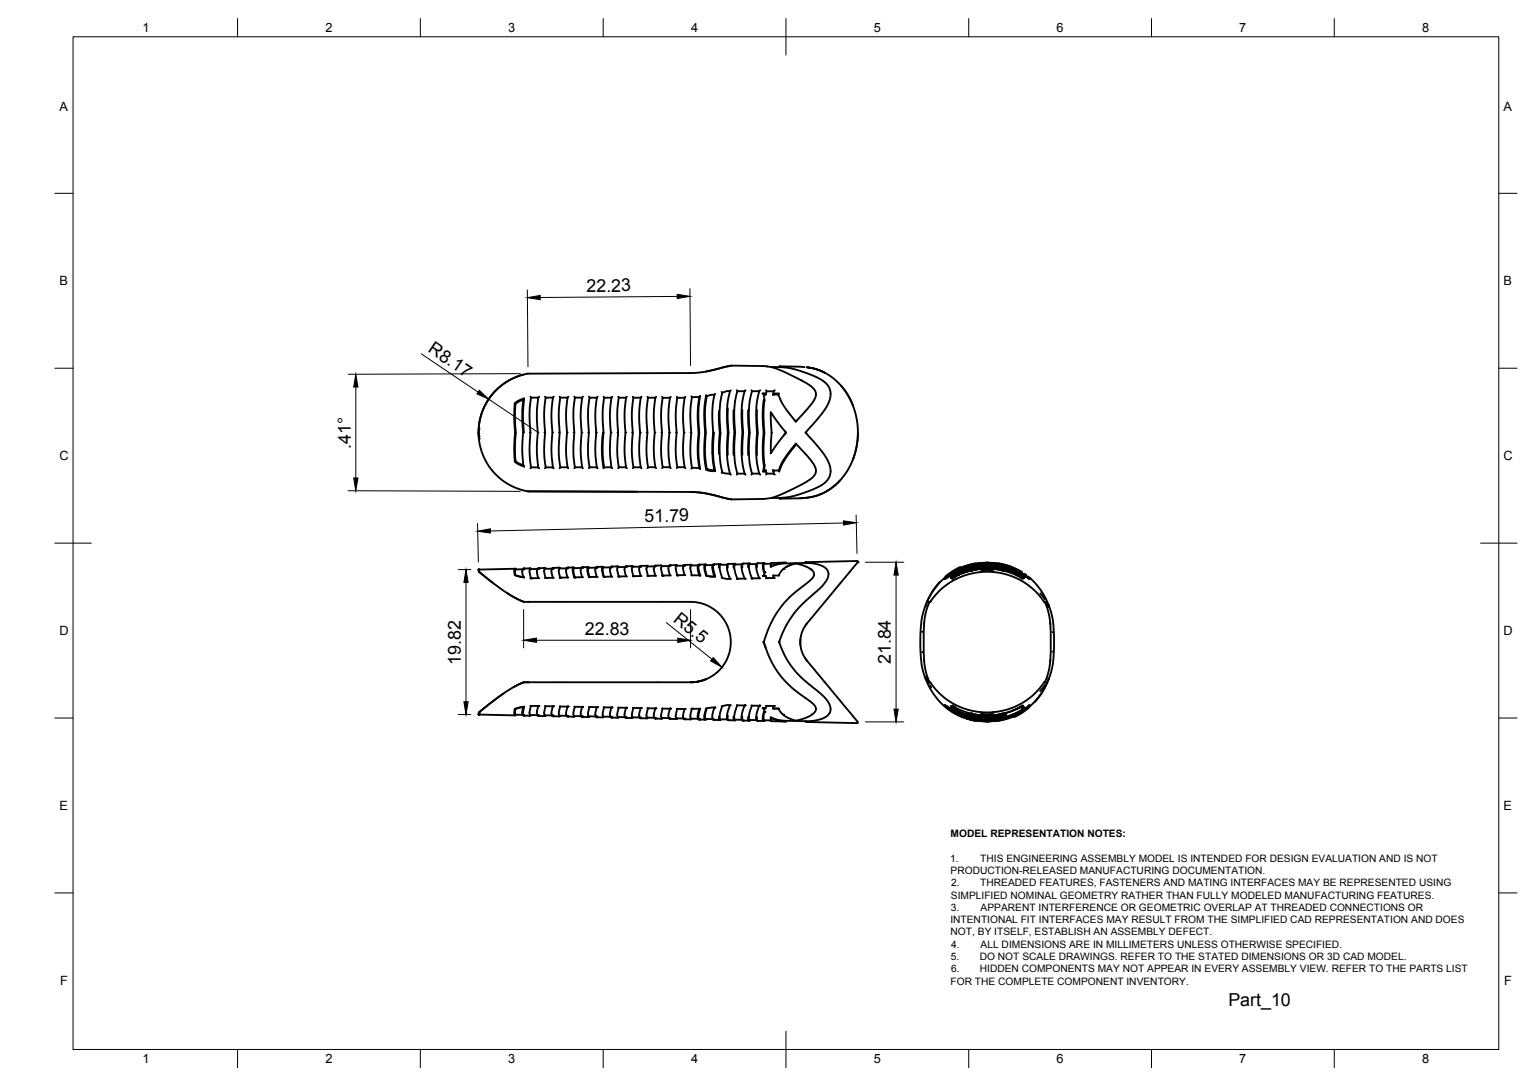
ISO-10303-21;
HEADER;
/* Generated by software containing ST-Developer
 * from STEP Tools, Inc. (www.steptools.com) 
 */

FILE_DESCRIPTION(
/* description */ ('STEP AP242 Edition 2'),
/* implementation_level */ '2;1');

FILE_NAME(
/* name */ 'Part_10.step',
/* time_stamp */ '2026-10-06T10:11:12-07:00',
/* author */ (''),
/* organization */ (''),
/* preprocessor_version */ 'ST-DEVELOPER v20.2',
/* originating_system */ 'Autodesk Translation Framework v15.15.0.0',
/* authorisation */ '');

FILE_SCHEMA (('AUTOMOTIVE_DESIGN { 1 0 10303 214 3 1 1 }'));
ENDSEC;

DATA;
#10=MECHANICAL_DESIGN_GEOMETRIC_PRESENTATION_REPRESENTATION('',(#1786),#54580);
#71=ELLIPSE('',#18547,0.0043287679400298,0.000195921240702569);
#131=CONICAL_SURFACE('',#18530,0.00265391324380841,1.37712278252772);
#132=CONICAL_SURFACE('',#18588,3.48610109958525E-5,0.141830950521549);
#133=CONICAL_SURFACE('',#18589,3.48394090574724E-5,0.141829837312193);
#134=CONICAL_SURFACE('',#18592,3.48609373749775E-5,0.141830787231043);
#135=CONICAL_SURFACE('',#18599,3.48393253777631E-5,0.141829687868949);
#136=CONICAL_SURFACE('',#18616,0.0026288792428795,1.38153808164484);
#137=CONICAL_SURFACE('',#18636,0.00265359345896356,1.37715118560564);
#138=CONICAL_SURFACE('',#18637,0.00263026865692114,1.38147192931234);
#139=CONICAL_SURFACE('',#18655,0.00614051900660571,0.733182632957209);
#140=CONICAL_SURFACE('',#18656,0.00592688725800199,0.772003379135275);
#143=SPHERICAL_SURFACE('',#18577,0.0001);
#144=SPHERICAL_SURFACE('',#18591,0.0001);
#145=SPHERICAL_SURFACE('',#18594,0.0001);
#146=SPHERICAL_SURFACE('',#18598,0.0001);
#147=SPHERICAL_SURFACE('',#18605,0.0001);
#148=SPHERICAL_SURFACE('',#18609,0.0001);
#192=TOROIDAL_SURFACE('',#18561,43.0172655815845,43.0171612476028);
#193=TOROIDAL_SURFACE('',#18562,43.0192266270189,43.0191222943202);
#194=TOROIDAL_SURFACE('',#18565,0.00931146593211752,9.99931797011151E-5);
#195=TOROIDAL_SURFACE('',#18566,0.00931142924739271,9.99898356076873E-5);
#196=TOROIDAL_SURFACE('',#18569,43.0172619393224,43.0171576053291);
#197=TOROIDAL_SURFACE('',#18572,43.0192273884314,43.0191230557219);
#198=TOROIDAL_SURFACE('',#18575,0.00408904168337188,9.99937992667749E-5);
#199=TOROIDAL_SURFACE('',#18576,0.00408904168282665,9.99937992622037E-5);
#200=TOROIDAL_SURFACE('',#18579,0.00806904972011834,0.0001);
#201=TOROIDAL_SURFACE('',#18596,0.00806904972011834,0.0001);
#202=TOROIDAL_SURFACE('',#18607,0.00806904972011834,0.0001);
#203=TOROIDAL_SURFACE('',#18610,0.00408913544960028,0.000100040268464404);
#204=TOROIDAL_SURFACE('',#18615,0.0040891354500689,0.000100040268460989);
#205=TOROIDAL_SURFACE('',#18659,0.00836123117893049,0.00010366855176599);
#206=TOROIDAL_SURFACE('',#18684,0.00815612470458011,0.000103667398436053);
#207=TOROIDAL_SURFACE('',#18687,0.00871025103595541,0.000103662944645038);
#208=TOROIDAL_SURFACE('',#18688,0.00850695260093233,0.000103538344715324);
#209=TOROIDAL_SURFACE('',#18689,0.00871017740815006,0.000103662875721332);
#210=TOROIDAL_SURFACE('',#18690,0.00836086459677531,0.00010366849218277);
#211=TOROIDAL_SURFACE('',#18717,0.00815633290592581,0.00010366728866353);
#212=TOROIDAL_SURFACE('',#18720,0.00864670349933223,0.000103665652215068);
#213=TOROIDAL_SURFACE('',#18721,0.00850751186664759,0.00010353842958418);
#214=TOROIDAL_SURFACE('',#18722,0.00867809676383051,0.000103667225081647);
#215=TOROIDAL_SURFACE('',#18723,0.000528332315378602,0.000103512489509189);
#216=TOROIDAL_SURFACE('',#18724,0.00917182682012945,9.99999869507318E-5);
#217=TOROIDAL_SURFACE('',#18725,0.0040475617622906,9.99881997863187E-5);
#218=TOROIDAL_SURFACE('',#18727,0.00904061800886142,0.000100004225353136);
#219=TOROIDAL_SURFACE('',#18728,0.00360779826836622,9.99961776029768E-5);
#220=TOROIDAL_SURFACE('',#18729,0.0052330922254768,9.99920638411154E-5);
#221=TOROIDAL_SURFACE('',#18730,0.000732704479508413,0.000103581963632023);
#222=TOROIDAL_SURFACE('',#18731,0.0091590450963941,9.99999843261172E-5);
#223=TOROIDAL_SURFACE('',#18733,0.00915567105502713,9.99999896646458E-5);
#224=TOROIDAL_SURFACE('',#18734,0.00389212279884052,9.99966861379351E-5);
#225=TOROIDAL_SURFACE('',#18735,0.00357438694091518,9.99963100583166E-5);
#226=TOROIDAL_SURFACE('',#18736,0.00915654585560002,9.9999989426787E-5);
#227=TOROIDAL_SURFACE('',#18738,0.009161034600788,9.9999985180343E-5);
#228=TOROIDAL_SURFACE('',#18739,0.000584574123278554,0.000103503607413102);
#229=TOROIDAL_SURFACE('',#18740,0.00392317197798013,9.99876820615925E-5);
#230=TOROIDAL_SURFACE('',#18741,0.00339615673268595,9.99957943856544E-5);
#231=TOROIDAL_SURFACE('',#18742,0.00916833013124114,9.99999895548281E-5);
#232=TOROIDAL_SURFACE('',#18744,0.00475797702577389,9.99904037368119E-5);
#233=TOROIDAL_SURFACE('',#18745,0.00917126548676907,9.99999867155255E-5);
#234=TOROIDAL_SURFACE('',#18746,0.00060192390944549,0.000103561614538704);
#325=B_SPLINE_SURFACE_WITH_KNOTS('',3,3,((#25845,#25846,#25847,#25848),
(#25849,#25850,#25851,#25852),(#25853,#25854,#25855,#25856),(#25857,#25858,
#25859,#25860),(#25861,#25862,#25863,#25864),(#25865,#25866,#25867,#25868),
(#25869,#25870,#25871,#25872),(#25873,#25874,#25875,#25876),(#25877,#25878,
#25879,#25880),(#25881,#25882,#25883,#25884),(#25885,#25886,#25887,#25888),
(#25889,#25890,#25891,#25892),(#25893,#25894,#25895,#25896),(#25897,#25898,
#25899,#25900),(#25901,#25902,#25903,#25904),(#25905,#25906,#25907,#25908),
(#25909,#25910,#25911,#25912),(#25913,#25914,#25915,#25916),(#25917,#25918,
#25919,#25920),(#25921,#25922,#25923,#25924),(#25925,#25926,#25927,#25928),
(#25929,#25930,#25931,#25932),(#25933,#25934,#25935,#25936),(#25937,#25938,
#25939,#25940),(#25941,#25942,#25943,#25944),(#25945,#25946,#25947,#25948),
(#25949,#25950,#25951,#25952),(#25953,#25954,#25955,#25956),(#25957,#25958,
#25959,#25960),(#25961,#25962,#25963,#25964),(#25965,#25966,#25967,#25968),
(#25969,#25970,#25971,#25972),(#25973,#25974,#25975,#25976),(#25977,#25978,
#25979,#25980),(#25981,#25982,#25983,#25984),(#25985,#25986,#25987,#25988),
(#25989,#25990,#25991,#25992),(#25993,#25994,#25995,#25996),(#25997,#25998,
#25999,#26000)),.UNSPECIFIED.,.T.,.F.,.F.,(4,1,1,1,1,1,1,1,1,1,1,1,1,1,
1,1,1,1,1,1,1,1,1,1,1,1,1,1,1,1,1,1,1,1,1,1,4),(4,4),(-1.,-0.9921875,-0.984375,
-0.96875,-0.9375,-0.921875,-0.90625,-0.875,-0.84375,-0.8125,-0.78125,-0.75,
-0.6875,-0.625,-0.59375,-0.5625,-0.53125,-0.515625,-0.5,-0.4921875,-0.484375,
-0.46875,-0.4375,-0.421875,-0.40625,-0.375,-0.34375,-0.3125,-0.28125,-0.25,
-0.1875,-0.125,-0.09375,-0.0625,-0.03125,-0.015625,0.),(0.0970446199077052,
0.967246564070376),.UNSPECIFIED.);
#326=B_SPLINE_SURFACE_WITH_KNOTS('',3,1,((#26093,#26094),(#26095,#26096),
(#26097,#26098),(#26099,#26100),(#26101,#26102),(#26103,#26104),(#26105,
#26106),(#26107,#26108),(#26109,#26110),(#26111,#26112),(#26113,#26114),
(#26115,#26116),(#26117,#26118),(#26119,#26120),(#26121,#26122),(#26123,
#26124),(#26125,#26126),(#26127,#26128),(#26129,#26130),(#26131,#26132),
(#26133,#26134),(#26135,#26136),(#26137,#26138),(#26139,#26140),(#26141,
#26142),(#26143,#26144),(#26145,#26146),(#26147,#26148),(#26149,#26150),
(#26151,#26152),(#26153,#26154),(#26155,#26156)),.UNSPECIFIED.,.T.,.F.,
 .F.,(4,1,2,1,1,1,1,1,1,1,2,1,1,1,2,1,1,1,1,1,1,1,3,1,4),(2,2),(-0.962123410396902,
-0.943185115595354,-0.924246820793805,-0.871215968194179,-0.818185115594553,
-0.765154262994927,-0.712123410395301,-0.659092557795675,-0.606061705196049,
-0.553030852596423,-0.499999999996798,-0.481061705196237,-0.462123410395676,
-0.443185115595116,-0.424246820794555,-0.371215968195236,-0.318185115595916,
-0.265154262996597,-0.212123410397278,-0.159092557797958,-0.106061705198639,
-0.0530308525993189,0.,0.0189382948015488,0.0378765896030977),(0.785837404066612,
0.964086943478034),.UNSPECIFIED.);
#327=B_SPLINE_SURFACE_WITH_KNOTS('',3,1,((#26801,#26802),(#26803,#26804),
(#26805,#26806),(#26807,#26808),(#26809,#26810),(#26811,#26812),(#26813,
#26814),(#26815,#26816),(#26817,#26818),(#26819,#26820),(#26821,#26822),
(#26823,#26824),(#26825,#26826),(#26827,#26828),(#26829,#26830),(#26831,
#26832),(#26833,#26834),(#26835,#26836),(#26837,#26838),(#26839,#26840),
(#26841,#26842),(#26843,#26844),(#26845,#26846),(#26847,#26848),(#26849,
#26850),(#26851,#26852),(#26853,#26854),(#26855,#26856),(#26857,#26858),
(#26859,#26860),(#26861,#26862),(#26863,#26864),(#26865,#26866)),
 .UNSPECIFIED.,.T.,.F.,.F.,(4,1,1,1,1,3,1,1,1,2,1,1,1,1,1,1,1,2,1,1,1,2,
1,1,1,4),(2,2),(-0.237377771779514,-0.212123410397278,-0.159092557797958,
-0.106061705198639,-0.0530308525993189,0.,0.0189382948015488,0.0378765896030977,
0.0568148844046463,0.0757531792061952,0.128784031805821,0.181814884405447,
0.234845737005073,0.287876589604699,0.340907442204325,0.393938294803951,
0.446969147403577,0.500000000003202,0.518938294803763,0.537876589604324,
0.556814884404884,0.575753179205445,0.628784031804764,0.681814884404084,
0.734845737003403,0.762622228220486),(0.0953842576150604,0.872111738883991),
 .UNSPECIFIED.);
#328=B_SPLINE_SURFACE_WITH_KNOTS('',3,3,((#29129,#29130,#29131,#29132),
(#29133,#29134,#29135,#29136),(#29137,#29138,#29139,#29140),(#29141,#29142,
#29143,#29144),(#29145,#29146,#29147,#29148),(#29149,#29150,#29151,#29152),
(#29153,#29154,#29155,#29156),(#29157,#29158,#29159,#29160),(#29161,#29162,
#29163,#29164),(#29165,#29166,#29167,#29168),(#29169,#29170,#29171,#29172),
(#29173,#29174,#29175,#29176),(#29177,#29178,#29179,#29180),(#29181,#29182,
#29183,#29184),(#29185,#29186,#29187,#29188),(#29189,#29190,#29191,#29192),
(#29193,#29194,#29195,#29196),(#29197,#29198,#29199,#29200),(#29201,#29202,
#29203,#29204),(#29205,#29206,#29207,#29208),(#29209,#29210,#29211,#29212),
(#29213,#29214,#29215,#29216),(#29217,#29218,#29219,#29220),(#29221,#29222,
#29223,#29224),(#29225,#29226,#29227,#29228),(#29229,#29230,#29231,#29232),
(#29233,#29234,#29235,#29236),(#29237,#29238,#29239,#29240),(#29241,#29242,
#29243,#29244),(#29245,#29246,#29247,#29248),(#29249,#29250,#29251,#29252),
(#29253,#29254,#29255,#29256),(#29257,#29258,#29259,#29260),(#29261,#29262,
#29263,#29264),(#29265,#29266,#29267,#29268)),.UNSPECIFIED.,.T.,.F.,.F.,
(4,1,1,1,1,1,1,1,1,1,1,1,1,1,1,1,1,1,1,1,1,1,1,1,1,1,1,1,1,1,1,1,4),(4,
4),(-1.,-0.984375,-0.96875,-0.9375,-0.921875,-0.90625,-0.875,-0.84375,-0.8125,
-0.75,-0.6875,-0.625,-0.59375,-0.5625,-0.53125,-0.515625,-0.5,-0.484375,
-0.46875,-0.4375,-0.421875,-0.40625,-0.375,-0.34375,-0.3125,-0.25,-0.1875,
-0.125,-0.09375,-0.0625,-0.03125,-0.015625,0.),(0.748401658952503,0.903433079647334),
 .UNSPECIFIED.);
#329=B_SPLINE_SURFACE_WITH_KNOTS('',3,3,((#30017,#30018,#30019,#30020),
(#30021,#30022,#30023,#30024),(#30025,#30026,#30027,#30028),(#30029,#30030,
#30031,#30032),(#30033,#30034,#30035,#30036),(#30037,#30038,#30039,#30040),
(#30041,#30042,#30043,#30044),(#30045,#30046,#30047,#30048),(#30049,#30050,
#30051,#30052),(#30053,#30054,#30055,#30056),(#30057,#30058,#30059,#30060),
(#30061,#30062,#30063,#30064),(#30065,#30066,#30067,#30068),(#30069,#30070,
#30071,#30072),(#30073,#30074,#30075,#30076),(#30077,#30078,#30079,#30080),
(#30081,#30082,#30083,#30084),(#30085,#30086,#30087,#30088),(#30089,#30090,
#30091,#30092),(#30093,#30094,#30095,#30096),(#30097,#30098,#30099,#30100),
(#30101,#30102,#30103,#30104),(#30105,#30106,#30107,#30108),(#30109,#30110,
#30111,#30112),(#30113,#30114,#30115,#30116),(#30117,#30118,#30119,#30120),
(#30121,#30122,#30123,#30124),(#30125,#30126,#30127,#30128),(#30129,#30130,
#30131,#30132),(#30133,#30134,#30135,#30136),(#30137,#30138,#30139,#30140),
(#30141,#30142,#30143,#30144),(#30145,#30146,#30147,#30148),(#30149,#30150,
#30151,#30152),(#30153,#30154,#30155,#30156)),.UNSPECIFIED.,.T.,.F.,.F.,
(4,1,1,1,1,1,1,1,1,1,1,1,1,1,1,1,1,1,1,1,1,1,1,1,1,1,1,1,1,1,1,1,4),(4,
4),(1.,1.015625,1.03125,1.0625,1.078125,1.09375,1.125,1.15625,1.1875,1.25,
1.3125,1.375,1.40625,1.4375,1.46875,1.484375,1.5,1.515625,1.53125,1.5625,
1.578125,1.59375,1.625,1.65625,1.6875,1.75,1.8125,1.875,1.90625,1.9375,
1.96875,1.984375,2.),(0.748401658952503,0.903433079647334),
 .UNSPECIFIED.);
#330=B_SPLINE_SURFACE_WITH_KNOTS('',3,1,((#30336,#30337),(#30338,#30339),
(#30340,#30341),(#30342,#30343),(#30344,#30345),(#30346,#30347),(#30348,
#30349),(#30350,#30351),(#30352,#30353),(#30354,#30355),(#30356,#30357),
(#30358,#30359),(#30360,#30361),(#30362,#30363),(#30364,#30365),(#30366,
#30367),(#30368,#30369),(#30370,#30371),(#30372,#30373),(#30374,#30375),
(#30376,#30377),(#30378,#30379),(#30380,#30381),(#30382,#30383),(#30384,
#30385),(#30386,#30387),(#30388,#30389),(#30390,#30391),(#30392,#30393),
(#30394,#30395)),.UNSPECIFIED.,.T.,.F.,.F.,(4,1,1,1,2,1,1,1,1,1,1,1,2,1,
1,1,2,1,1,1,1,1,1,1,4),(2,2),(1.,1.01893829480155,1.0378765896031,1.05681488440465,
1.0757531792062,1.12878403180582,1.18181488440545,1.23484573700507,1.2878765896047,
1.34090744220433,1.39393829480395,1.44696914740358,1.5000000000032,1.51893829480376,
1.53787658960432,1.55681488440488,1.57575317920544,1.62878403180476,1.68181488440408,
1.7348457370034,1.78787658960272,1.84090744220204,1.89393829480136,1.94696914740068,
2.),(0.0953842576150604,0.872111738883991),.UNSPECIFIED.);
#331=B_SPLINE_SURFACE_WITH_KNOTS('',3,1,((#34950,#34951),(#34952,#34953),
(#34954,#34955),(#34956,#34957),(#34958,#34959),(#34960,#34961),(#34962,
#34963),(#34964,#34965),(#34966,#34967),(#34968,#34969),(#34970,#34971),
(#34972,#34973),(#34974,#34975),(#34976,#34977),(#34978,#34979),(#34980,
#34981),(#34982,#34983),(#34984,#34985),(#34986,#34987),(#34988,#34989),
(#34990,#34991),(#34992,#34993),(#34994,#34995),(#34996,#34997),(#34998,
#34999),(#35000,#35001),(#35002,#35003),(#35004,#35005),(#35006,#35007),
(#35008,#35009)),.UNSPECIFIED.,.T.,.F.,.F.,(4,1,1,1,2,1,1,1,1,1,1,1,2,1,
1,1,2,1,1,1,1,1,1,1,4),(2,2),(1.,1.01893829480155,1.0378765896031,1.05681488440465,
1.0757531792062,1.12878403180582,1.18181488440545,1.23484573700507,1.2878765896047,
1.34090744220433,1.39393829480395,1.44696914740358,1.5000000000032,1.51893829480376,
1.53787658960432,1.55681488440488,1.57575317920544,1.62878403180476,1.68181488440408,
1.7348457370034,1.78787658960272,1.84090744220204,1.89393829480136,1.94696914740068,
2.),(0.785837404066612,0.964086943478034),.UNSPECIFIED.);
#332=B_SPLINE_SURFACE_WITH_KNOTS('',1,3,((#35025,#35026,#35027,#35028,#35029,
#35030,#35031,#35032,#35033,#35034,#35035,#35036,#35037,#35038,#35039,#35040,
#35041,#35042,#35043,#35044),(#35045,#35046,#35047,#35048,#35049,#35050,
#35051,#35052,#35053,#35054,#35055,#35056,#35057,#35058,#35059,#35060,#35061,
#35062,#35063,#35064),(#35065,#35066,#35067,#35068,#35069,#35070,#35071,
#35072,#35073,#35074,#35075,#35076,#35077,#35078,#35079,#35080,#35081,#35082,
#35083,#35084)),.UNSPECIFIED.,.F.,.F.,.F.,(2,1,2),(4,2,2,2,2,2,2,2,2,4),
(0.,1.,1.005),(0.999268187708551,0.99938964839267,0.999511718705164,0.999633789017659,
0.999694824173906,0.999755859330153,0.999877929642648,0.999908447220771,
0.999938964798895,0.999999999955142),.UNSPECIFIED.);
#333=B_SPLINE_SURFACE_WITH_KNOTS('',3,3,((#35229,#35230,#35231,#35232),
(#35233,#35234,#35235,#35236),(#35237,#35238,#35239,#35240),(#35241,#35242,
#35243,#35244),(#35245,#35246,#35247,#35248),(#35249,#35250,#35251,#35252),
(#35253,#35254,#35255,#35256),(#35257,#35258,#35259,#35260),(#35261,#35262,
#35263,#35264),(#35265,#35266,#35267,#35268),(#35269,#35270,#35271,#35272),
(#35273,#35274,#35275,#35276),(#35277,#35278,#35279,#35280),(#35281,#35282,
#35283,#35284),(#35285,#35286,#35287,#35288),(#35289,#35290,#35291,#35292),
(#35293,#35294,#35295,#35296),(#35297,#35298,#35299,#35300),(#35301,#35302,
#35303,#35304),(#35305,#35306,#35307,#35308),(#35309,#35310,#35311,#35312),
(#35313,#35314,#35315,#35316),(#35317,#35318,#35319,#35320),(#35321,#35322,
#35323,#35324),(#35325,#35326,#35327,#35328),(#35329,#35330,#35331,#35332),
(#35333,#35334,#35335,#35336),(#35337,#35338,#35339,#35340),(#35341,#35342,
#35343,#35344),(#35345,#35346,#35347,#35348),(#35349,#35350,#35351,#35352),
(#35353,#35354,#35355,#35356),(#35357,#35358,#35359,#35360),(#35361,#35362,
#35363,#35364),(#35365,#35366,#35367,#35368),(#35369,#35370,#35371,#35372),
(#35373,#35374,#35375,#35376),(#35377,#35378,#35379,#35380),(#35381,#35382,
#35383,#35384)),.UNSPECIFIED.,.T.,.F.,.F.,(4,1,1,1,1,1,1,1,1,1,1,1,1,1,
1,1,1,1,1,1,1,1,1,1,1,1,1,1,1,1,1,1,1,1,1,1,4),(4,4),(0.,0.0078125,0.015625,
0.03125,0.0625,0.078125,0.09375,0.125,0.15625,0.1875,0.21875,0.25,0.3125,
0.375,0.40625,0.4375,0.46875,0.484375,0.5,0.5078125,0.515625,0.53125,0.5625,
0.578125,0.59375,0.625,0.65625,0.6875,0.71875,0.75,0.8125,0.875,0.90625,
0.9375,0.96875,0.984375,1.),(0.0970446199077052,0.967246564070376),
 .UNSPECIFIED.);
#334=B_SPLINE_SURFACE_WITH_KNOTS('',3,3,((#37152,#37153,#37154,#37155),
(#37156,#37157,#37158,#37159),(#37160,#37161,#37162,#37163),(#37164,#37165,
#37166,#37167),(#37168,#37169,#37170,#37171),(#37172,#37173,#37174,#37175),
(#37176,#37177,#37178,#37179),(#37180,#37181,#37182,#37183),(#37184,#37185,
#37186,#37187),(#37188,#37189,#37190,#37191),(#37192,#37193,#37194,#37195),
(#37196,#37197,#37198,#37199),(#37200,#37201,#37202,#37203),(#37204,#37205,
#37206,#37207),(#37208,#37209,#37210,#37211),(#37212,#37213,#37214,#37215),
(#37216,#37217,#37218,#37219),(#37220,#37221,#37222,#37223),(#37224,#37225,
#37226,#37227),(#37228,#37229,#37230,#37231),(#37232,#37233,#37234,#37235),
(#37236,#37237,#37238,#37239),(#37240,#37241,#37242,#37243),(#37244,#37245,
#37246,#37247),(#37248,#37249,#37250,#37251),(#37252,#37253,#37254,#37255),
(#37256,#37257,#37258,#37259),(#37260,#37261,#37262,#37263),(#37264,#37265,
#37266,#37267),(#37268,#37269,#37270,#37271),(#37272,#37273,#37274,#37275),
(#37276,#37277,#37278,#37279),(#37280,#37281,#37282,#37283),(#37284,#37285,
#37286,#37287),(#37288,#37289,#37290,#37291)),.UNSPECIFIED.,.T.,.F.,.F.,
(4,1,1,1,1,1,1,1,1,1,1,1,1,1,1,1,1,1,1,1,1,1,1,1,1,1,1,1,1,1,1,1,4),(4,
4),(0.,0.015625,0.03125,0.0625,0.078125,0.09375,0.125,0.15625,0.1875,0.25,
0.3125,0.375,0.40625,0.4375,0.46875,0.484375,0.5,0.515625,0.53125,0.5625,
0.578125,0.59375,0.625,0.65625,0.6875,0.75,0.8125,0.875,0.90625,0.9375,
0.96875,0.984375,1.),(0.748401658952503,0.903433079647334),
 .UNSPECIFIED.);
#335=B_SPLINE_SURFACE_WITH_KNOTS('',3,3,((#44797,#44798,#44799,#44800,#44801),
(#44802,#44803,#44804,#44805,#44806),(#44807,#44808,#44809,#44810,#44811),
(#44812,#44813,#44814,#44815,#44816),(#44817,#44818,#44819,#44820,#44821),
(#44822,#44823,#44824,#44825,#44826),(#44827,#44828,#44829,#44830,#44831),
(#44832,#44833,#44834,#44835,#44836),(#44837,#44838,#44839,#44840,#44841)),
 .UNSPECIFIED.,.F.,.F.,.F.,(4,1,1,1,1,1,4),(4,1,4),(0.00214678110273797,
0.00328311417485291,0.00393151580676355,0.00522831907058484,0.00652512233440613,
0.00717352396631677,0.00830134515056596),(-0.00760700162757571,0.496196499186212,
1.0043667759093),.UNSPECIFIED.);
#336=B_SPLINE_SURFACE_WITH_KNOTS('',3,3,((#44958,#44959,#44960,#44961,#44962),
(#44963,#44964,#44965,#44966,#44967),(#44968,#44969,#44970,#44971,#44972),
(#44973,#44974,#44975,#44976,#44977),(#44978,#44979,#44980,#44981,#44982),
(#44983,#44984,#44985,#44986,#44987),(#44988,#44989,#44990,#44991,#44992),
(#44993,#44994,#44995,#44996,#44997),(#44998,#44999,#45000,#45001,#45002)),
 .UNSPECIFIED.,.F.,.F.,.F.,(4,1,1,1,1,1,4),(4,1,4),(0.0021509040335451,
0.00328755319845632,0.00393613508633228,0.0052332988620842,0.00653046263783612,
0.00717904452571208,0.0083071902285716),(-0.00767667710147584,0.496161661449262,
1.00435471660804),.UNSPECIFIED.);
#365=B_SPLINE_CURVE_WITH_KNOTS('',3,(#26003,#26004,#26005,#26006),
 .UNSPECIFIED.,.F.,.F.,(4,4),(0.668250521172189,0.843615509259931),
 .UNSPECIFIED.);
#366=B_SPLINE_CURVE_WITH_KNOTS('',3,(#26008,#26009,#26010,#26011,#26012,
#26013,#26014,#26015,#26016,#26017,#26018,#26019,#26020,#26021,#26022,#26023,
#26024,#26025,#26026),.UNSPECIFIED.,.F.,.F.,(4,3,3,3,3,3,4),(0.0111833063008374,
0.0121008630969431,0.0122880406507484,0.0132009415603016,0.0135642406067081,
0.0154010984870185,0.0176012552434354),.UNSPECIFIED.);
#367=B_SPLINE_CURVE_WITH_KNOTS('',3,(#26028,#26029,#26030,#26031,#26032,
#26033,#26034,#26035,#26036,#26037,#26038,#26039,#26040,#26041,#26042,#26043,
#26044,#26045,#26046,#26047,#26048,#26049,#26050,#26051,#26052,#26053,#26054,
#26055),.UNSPECIFIED.,.F.,.F.,(4,3,3,3,3,3,3,3,3,4),(1.06517613933674E-8,
0.0625,0.125,0.15625,0.1875,0.25,0.375,0.5,0.75,0.99999998854857),
 .UNSPECIFIED.);
#368=B_SPLINE_CURVE_WITH_KNOTS('',3,(#26057,#26058,#26059,#26060,#26061,
#26062,#26063),.UNSPECIFIED.,.F.,.F.,(4,1,1,1,4),(2.92983445734476E-17,
0.00266695458268161,0.00533390916536319,0.00800086374804478,0.0106678183307264),
 .UNSPECIFIED.);
#369=B_SPLINE_CURVE_WITH_KNOTS('',3,(#26065,#26066,#26067,#26068),
 .UNSPECIFIED.,.F.,.F.,(4,4),(0.102324395314902,0.960851822466372),
 .UNSPECIFIED.);
#370=B_SPLINE_CURVE_WITH_KNOTS('',3,(#26070,#26071,#26072,#26073,#26074,
#26075,#26076,#26077,#26078,#26079,#26080,#26081,#26082,#26083,#26084,#26085,
#26086,#26087,#26088,#26089,#26090,#26091),.UNSPECIFIED.,.F.,.F.,(4,3,3,
3,3,3,3,4),(0.0158713903754465,0.0168306242499723,0.0187006936110803,0.0205707629721883,
0.0224303222343527,0.0224408323332963,0.0261809710555123,0.0299211047587188),
 .UNSPECIFIED.);
#371=B_SPLINE_CURVE_WITH_KNOTS('',1,(#26159,#26160),.UNSPECIFIED.,.F.,.F.,
(2,2),(-0.843561641779046,-0.803664345351663),.UNSPECIFIED.);
#372=B_SPLINE_CURVE_WITH_KNOTS('',3,(#26162,#26163,#26164,#26165),
 .UNSPECIFIED.,.F.,.F.,(4,4),(0.,0.0677982128913682),.UNSPECIFIED.);
#373=B_SPLINE_CURVE_WITH_KNOTS('',3,(#26167,#26168,#26169,#26170,#26171,
#26172,#26173,#26174,#26175,#26176,#26177,#26178,#26179,#26180,#26181,#26182,
#26183,#26184,#26185,#26186,#26187,#26188,#26189,#26190,#26191,#26192,#26193,
#26194,#26195,#26196,#26197,#26198,#26199,#26200,#26201,#26202,#26203,#26204,
#26205,#26206,#26207,#26208,#26209,#26210,#26211,#26212,#26213,#26214,#26215,
#26216,#26217,#26218,#26219,#26220,#26221,#26222,#26223,#26224,#26225,#26226,
#26227,#26228,#26229,#26230,#26231,#26232,#26233,#26234,#26235,#26236,#26237,
#26238,#26239,#26240,#26241,#26242,#26243,#26244,#26245,#26246,#26247,#26248,
#26249,#26250,#26251,#26252,#26253,#26254,#26255,#26256,#26257,#26258,#26259,
#26260,#26261,#26262,#26263,#26264,#26265,#26266,#26267,#26268,#26269,#26270,
#26271,#26272,#26273,#26274,#26275,#26276,#26277,#26278,#26279,#26280,#26281,
#26282,#26283,#26284,#26285,#26286,#26287,#26288,#26289,#26290,#26291,#26292,
#26293,#26294,#26295,#26296,#26297,#26298,#26299,#26300,#26301,#26302,#26303,
#26304,#26305,#26306,#26307,#26308,#26309,#26310,#26311,#26312,#26313,#26314,
#26315,#26316,#26317,#26318,#26319,#26320,#26321,#26322,#26323,#26324,#26325,
#26326,#26327,#26328,#26329,#26330,#26331,#26332,#26333,#26334,#26335,#26336,
#26337,#26338,#26339,#26340,#26341,#26342,#26343,#26344,#26345,#26346,#26347,
#26348,#26349,#26350),.UNSPECIFIED.,.F.,.F.,(4,3,3,3,3,3,3,3,3,3,3,3,3,
3,3,3,3,3,3,3,3,3,3,3,3,3,3,3,3,3,3,3,3,3,3,3,3,3,3,3,3,3,3,3,3,3,3,3,3,
3,3,3,3,3,3,3,3,3,3,3,3,4),(2.23112281381123E-7,0.03125,0.046875,0.0546875,
0.0625,0.0703125,0.078125,0.09375,0.109375,0.125,0.128101322996236,0.140625,
0.15625,0.171875,0.1875,0.203125,0.21875,0.234375,0.25,0.261882944458568,
0.265625,0.28125,0.3125,0.34375,0.359375,0.375,0.385783882951856,0.390625,
0.40625,0.4375,0.5,0.50039038538168,0.5625,0.59375,0.609375,0.614591279201434,
0.625,0.640625,0.65625,0.6875,0.71875,0.734375,0.73855596574661,0.75,0.765625,
0.78125,0.796875,0.8125,0.828125,0.84375,0.859375,0.872372445270951,0.875,
0.890625,0.90625,0.921875,0.9296875,0.9375,0.9453125,0.953125,0.96875,0.999999779165919),
 .UNSPECIFIED.);
#374=B_SPLINE_CURVE_WITH_KNOTS('',3,(#26352,#26353,#26354,#26355,#26356),
 .UNSPECIFIED.,.F.,.F.,(4,1,4),(0.,0.5,1.),.UNSPECIFIED.);
#375=B_SPLINE_CURVE_WITH_KNOTS('',3,(#26358,#26359,#26360,#26361,#26362,
#26363,#26364,#26365,#26366,#26367,#26368,#26369,#26370,#26371,#26372,#26373,
#26374,#26375,#26376,#26377,#26378,#26379,#26380,#26381,#26382,#26383,#26384,
#26385,#26386,#26387,#26388,#26389,#26390,#26391,#26392,#26393,#26394,#26395,
#26396,#26397,#26398,#26399,#26400,#26401,#26402,#26403,#26404,#26405,#26406,
#26407,#26408,#26409,#26410,#26411,#26412,#26413,#26414,#26415,#26416,#26417,
#26418,#26419,#26420,#26421,#26422,#26423,#26424,#26425,#26426,#26427,#26428,
#26429,#26430,#26431,#26432,#26433,#26434,#26435,#26436,#26437,#26438,#26439,
#26440,#26441,#26442,#26443,#26444,#26445,#26446,#26447,#26448,#26449,#26450,
#26451,#26452,#26453,#26454,#26455,#26456,#26457,#26458,#26459,#26460,#26461,
#26462,#26463,#26464,#26465,#26466,#26467,#26468,#26469,#26470,#26471,#26472,
#26473,#26474,#26475,#26476,#26477,#26478,#26479,#26480,#26481,#26482,#26483,
#26484,#26485,#26486,#26487,#26488,#26489,#26490,#26491,#26492,#26493,#26494,
#26495,#26496,#26497,#26498,#26499,#26500,#26501,#26502,#26503,#26504,#26505,
#26506,#26507,#26508,#26509,#26510,#26511,#26512,#26513,#26514,#26515,#26516,
#26517,#26518,#26519,#26520,#26521,#26522,#26523,#26524,#26525,#26526,#26527,
#26528,#26529,#26530,#26531,#26532,#26533,#26534,#26535,#26536,#26537,#26538,
#26539,#26540,#26541),.UNSPECIFIED.,.F.,.F.,(4,3,3,3,3,3,3,3,3,3,3,3,3,
3,3,3,3,3,3,3,3,3,3,3,3,3,3,3,3,3,3,3,3,3,3,3,3,3,3,3,3,3,3,3,3,3,3,3,3,
3,3,3,3,3,3,3,3,3,3,3,3,4),(2.23106010072049E-7,0.03125,0.046875,0.0546875,
0.0625,0.0703125,0.078125,0.09375,0.109375,0.125,0.128101110916128,0.140625,
0.15625,0.171875,0.1875,0.203125,0.21875,0.234375,0.25,0.261882369249052,
0.265625,0.28125,0.3125,0.34375,0.359375,0.375,0.385783798958653,0.390625,
0.40625,0.4375,0.5,0.500390522344446,0.5625,0.59375,0.609375,0.614591477860909,
0.625,0.640625,0.65625,0.6875,0.71875,0.734375,0.738556592284746,0.75,0.765625,
0.78125,0.796875,0.8125,0.828125,0.84375,0.859375,0.872372659350468,0.875,
0.890625,0.90625,0.921875,0.9296875,0.9375,0.9453125,0.953125,0.96875,0.999999779172077),
 .UNSPECIFIED.);
#376=B_SPLINE_CURVE_WITH_KNOTS('',3,(#26543,#26544,#26545,#26546),
 .UNSPECIFIED.,.F.,.F.,(4,4),(0.499948130219197,1.),.UNSPECIFIED.);
#377=B_SPLINE_CURVE_WITH_KNOTS('',1,(#26548,#26549),.UNSPECIFIED.,.F.,.F.,
(2,2),(-0.831634677873798,-0.786894219517676),.UNSPECIFIED.);
#378=B_SPLINE_CURVE_WITH_KNOTS('',3,(#26551,#26552,#26553,#26554,#26555,
#26556,#26557,#26558,#26559,#26560,#26561,#26562,#26563,#26564,#26565,#26566,
#26567,#26568,#26569,#26570,#26571,#26572,#26573,#26574,#26575,#26576,#26577,
#26578,#26579,#26580,#26581,#26582,#26583,#26584,#26585,#26586,#26587,#26588,
#26589),.UNSPECIFIED.,.F.,.F.,(4,1,1,1,1,1,1,1,1,1,1,1,1,1,1,1,1,1,1,1,
1,1,1,1,1,1,1,1,1,1,1,1,1,1,1,1,4),(0.,0.015625,0.03125,0.046875,0.0625,
0.09375,0.125,0.15625,0.1875,0.25,0.28125,0.296875,0.3125,0.328125,0.34375,
0.359375,0.3671875,0.37109375,0.375,0.37890625,0.3828125,0.390625,0.3984375,
0.40625,0.4140625,0.421875,0.4296875,0.4375,0.4453125,0.453125,0.46875,
0.484375,0.5,0.515625,0.53125,0.5625,0.625),.UNSPECIFIED.);
#379=B_SPLINE_CURVE_WITH_KNOTS('',3,(#26591,#26592,#26593,#26594,#26595,
#26596,#26597,#26598,#26599,#26600,#26601,#26602,#26603,#26604,#26605,#26606,
#26607,#26608,#26609,#26610,#26611,#26612),.UNSPECIFIED.,.F.,.F.,(4,1,1,
1,1,1,1,1,1,1,1,1,1,1,1,1,1,1,1,4),(0.625,0.6875,0.71875,0.75,0.78125,0.796875,
0.8125,0.828125,0.84375,0.859375,0.875,0.890625,0.90625,0.921875,0.9296875,
0.9375,0.9453125,0.953125,0.96875,1.),.UNSPECIFIED.);
#380=B_SPLINE_CURVE_WITH_KNOTS('',3,(#26614,#26615,#26616,#26617,#26618,
#26619,#26620,#26621,#26622,#26623,#26624,#26625,#26626,#26627,#26628,#26629,
#26630,#26631,#26632,#26633,#26634,#26635,#26636,#26637,#26638,#26639,#26640,
#26641,#26642,#26643,#26644,#26645,#26646,#26647,#26648,#26649,#26650,#26651,
#26652,#26653,#26654,#26655,#26656,#26657,#26658,#26659,#26660,#26661,#26662,
#26663,#26664,#26665,#26666,#26667,#26668,#26669,#26670,#26671,#26672,#26673,
#26674,#26675,#26676,#26677),.UNSPECIFIED.,.F.,.F.,(4,1,1,1,1,1,1,1,1,1,
1,1,1,1,1,1,1,1,1,1,1,1,1,1,1,1,1,1,1,1,1,1,1,1,1,1,1,1,1,1,1,1,1,1,1,1,
1,1,1,1,1,1,1,1,1,1,1,1,1,1,1,4),(1.77187976368624E-6,0.03125,0.046875,
0.0546875,0.0625,0.0703125,0.078125,0.09375,0.109375,0.125,0.140625,0.15625,
0.171875,0.1875,0.203125,0.21875,0.234375,0.25,0.265625,0.28125,0.3125,
0.375,0.40625,0.4375,0.46875,0.484375,0.5,0.515625,0.53125,0.546875,0.5546875,
0.5625,0.5703125,0.578125,0.59375,0.6015625,0.609375,0.6171875,0.62109375,
0.625,0.62890625,0.6328125,0.640625,0.65625,0.671875,0.6875,0.703125,0.71875,
0.75,0.8125,0.84375,0.859375,0.875,0.90625,0.921875,0.9375,0.953125,0.9609375,
0.96875,0.9765625,0.984375,0.999999998713145),.UNSPECIFIED.);
#381=B_SPLINE_CURVE_WITH_KNOTS('',3,(#26679,#26680,#26681,#26682,#26683,
#26684,#26685,#26686,#26687,#26688,#26689,#26690),.UNSPECIFIED.,.F.,.F.,
(4,1,1,1,1,1,1,1,1,4),(0.,0.015625,0.0234375,0.03125,0.0390625,0.046875,
0.0625,0.078125,0.09375,0.124710011167853),.UNSPECIFIED.);
#382=B_SPLINE_CURVE_WITH_KNOTS('',3,(#26692,#26693,#26694,#26695,#26696,
#26697,#26698,#26699,#26700,#26701,#26702,#26703,#26704,#26705,#26706,#26707,
#26708,#26709,#26710,#26711,#26712,#26713,#26714,#26715,#26716,#26717,#26718,
#26719,#26720,#26721,#26722,#26723,#26724,#26725,#26726,#26727,#26728,#26729,
#26730,#26731),.UNSPECIFIED.,.F.,.F.,(4,1,1,1,1,1,1,1,1,1,1,1,1,1,1,1,1,
1,1,1,1,1,1,1,1,1,1,1,1,1,1,1,1,1,1,1,1,4),(0.124710011167853,0.125,0.15625,
0.1875,0.21875,0.25,0.28125,0.296875,0.3125,0.328125,0.34375,0.359375,0.3671875,
0.375,0.3828125,0.390625,0.40625,0.4140625,0.421875,0.4296875,0.43359375,
0.4375,0.44140625,0.4453125,0.453125,0.4609375,0.46875,0.484375,0.5,0.515625,
0.53125,0.5625,0.59375,0.625,0.6875,0.71875,0.75,0.756387532860041),
 .UNSPECIFIED.);
#383=B_SPLINE_CURVE_WITH_KNOTS('',3,(#26733,#26734,#26735,#26736,#26737,
#26738,#26739,#26740,#26741,#26742,#26743,#26744,#26745,#26746,#26747,#26748,
#26749,#26750,#26751),.UNSPECIFIED.,.F.,.F.,(4,1,1,1,1,1,1,1,1,1,1,1,1,
1,1,1,4),(0.756387532860041,0.78125,0.796875,0.8125,0.828125,0.84375,0.859375,
0.875,0.890625,0.90625,0.921875,0.9296875,0.9375,0.9453125,0.953125,0.96875,
1.),.UNSPECIFIED.);
#384=B_SPLINE_CURVE_WITH_KNOTS('',3,(#26752,#26753,#26754,#26755,#26756,
#26757,#26758,#26759,#26760,#26761,#26762,#26763,#26764,#26765,#26766,#26767,
#26768,#26769,#26770,#26771,#26772,#26773,#26774,#26775,#26776,#26777,#26778,
#26779,#26780,#26781,#26782,#26783,#26784,#26785,#26786,#26787,#26788,#26789,
#26790,#26791,#26792,#26793,#26794,#26795,#26796,#26797,#26798,#26799,#26800),
 .UNSPECIFIED.,.F.,.F.,(4,1,1,1,1,1,1,1,1,1,1,1,1,1,1,1,1,1,1,1,1,1,1,1,
1,1,1,1,1,1,1,1,1,1,1,1,1,1,1,1,1,1,1,1,1,1,4),(5.26782351439448E-6,0.03125,
0.0625,0.09375,0.109375,0.125,0.140625,0.15625,0.171875,0.1875,0.203125,
0.21875,0.25,0.28125,0.3125,0.375,0.40625,0.4375,0.46875,0.484375,0.5,0.515625,
0.5234375,0.53125,0.5390625,0.546875,0.5546875,0.55859375,0.5625,0.56640625,
0.5703125,0.578125,0.5859375,0.59375,0.609375,0.6171875,0.625,0.6328125,
0.640625,0.65625,0.671875,0.6875,0.703125,0.71875,0.75,0.8125,0.867768400737492),
 .UNSPECIFIED.);
#385=B_SPLINE_CURVE_WITH_KNOTS('',1,(#26869,#26870),.UNSPECIFIED.,.F.,.F.,
(2,2),(-0.762686810518316,-0.668179912465779),.UNSPECIFIED.);
#386=B_SPLINE_CURVE_WITH_KNOTS('',3,(#26872,#26873,#26874,#26875,#26876,
#26877,#26878,#26879,#26880,#26881,#26882,#26883,#26884,#26885,#26886,#26887,
#26888,#26889,#26890,#26891,#26892,#26893,#26894,#26895,#26896,#26897,#26898,
#26899,#26900,#26901,#26902,#26903,#26904,#26905,#26906,#26907,#26908,#26909,
#26910,#26911,#26912,#26913),.UNSPECIFIED.,.F.,.F.,(4,1,1,1,1,1,1,1,1,1,
1,1,1,1,1,1,1,1,1,1,1,1,1,1,1,1,1,1,1,1,1,1,1,1,1,1,1,1,1,4),(0.142413158676735,
0.1875,0.25,0.3125,0.34375,0.375,0.40625,0.4375,0.46875,0.484375,0.5,0.515625,
0.53125,0.5625,0.578125,0.59375,0.609375,0.625,0.640625,0.65625,0.671875,
0.6875,0.703125,0.71875,0.75,0.765625,0.78125,0.796875,0.8125,0.828125,
0.84375,0.859375,0.875,0.890625,0.90625,0.921875,0.9375,0.953125,0.96875,
1.),.UNSPECIFIED.);
#387=B_SPLINE_CURVE_WITH_KNOTS('',3,(#26915,#26916,#26917,#26918,#26919,
#26920,#26921,#26922,#26923,#26924,#26925,#26926,#26927,#26928,#26929,#26930,
#26931,#26932,#26933,#26934,#26935,#26936,#26937,#26938,#26939,#26940,#26941,
#26942),.UNSPECIFIED.,.F.,.F.,(4,3,3,3,3,3,3,3,3,4),(0.,0.0625,0.125,0.1875,
0.25,0.3125,0.375,0.4375,0.475532550545482,0.483433722321772),
 .UNSPECIFIED.);
#388=B_SPLINE_CURVE_WITH_KNOTS('',3,(#26944,#26945,#26946,#26947,#26948,
#26949,#26950,#26951,#26952,#26953,#26954,#26955,#26956,#26957,#26958,#26959,
#26960,#26961,#26962,#26963,#26964,#26965,#26966,#26967,#26968,#26969,#26970,
#26971,#26972,#26973,#26974,#26975,#26976,#26977),.UNSPECIFIED.,.F.,.F.,
(4,3,3,3,3,3,3,3,3,3,3,4),(0.483433722321772,0.5,0.5625,0.625,0.6875,0.75,
0.8125,0.84375,0.875,0.90625,0.9375,0.999990394166022),.UNSPECIFIED.);
#389=B_SPLINE_CURVE_WITH_KNOTS('',3,(#26979,#26980,#26981,#26982,#26983,
#26984,#26985,#26986,#26987,#26988,#26989,#26990,#26991,#26992,#26993,#26994,
#26995,#26996,#26997,#26998,#26999,#27000,#27001,#27002,#27003),
 .UNSPECIFIED.,.F.,.F.,(4,3,3,3,3,3,3,3,4),(3.51665398735729E-9,0.125,0.25,
0.375,0.5,0.5625,0.625,0.75,0.99894251312119),.UNSPECIFIED.);
#390=B_SPLINE_CURVE_WITH_KNOTS('',3,(#27009,#27010,#27011,#27012,#27013,
#27014,#27015,#27016,#27017,#27018),.UNSPECIFIED.,.F.,.F.,(4,3,3,4),(0.,
0.25,0.5,1.),.UNSPECIFIED.);
#391=B_SPLINE_CURVE_WITH_KNOTS('',3,(#27020,#27021,#27022,#27023,#27024,
#27025,#27026),.UNSPECIFIED.,.F.,.F.,(4,3,4),(0.0269518367147259,0.5,1.),
 .UNSPECIFIED.);
#392=B_SPLINE_CURVE_WITH_KNOTS('',3,(#27028,#27029,#27030,#27031),
 .UNSPECIFIED.,.F.,.F.,(4,4),(0.,0.0269518367147259),.UNSPECIFIED.);
#393=B_SPLINE_CURVE_WITH_KNOTS('',3,(#27033,#27034,#27035,#27036,#27037,
#27038,#27039,#27040,#27041,#27042,#27043,#27044,#27045,#27046,#27047,#27048,
#27049,#27050,#27051,#27052,#27053,#27054,#27055,#27056,#27057,#27058,#27059,
#27060),.UNSPECIFIED.,.F.,.F.,(4,3,3,3,3,3,3,3,3,4),(0.,0.25,0.375,0.5,
0.5625,0.625,0.6875,0.75,0.875,1.),.UNSPECIFIED.);
#394=B_SPLINE_CURVE_WITH_KNOTS('',3,(#27062,#27063,#27064,#27065,#27066,
#27067,#27068,#27069,#27070,#27071,#27072,#27073,#27074),.UNSPECIFIED.,
 .F.,.F.,(4,3,3,3,4),(0.,0.125,0.25,0.270263701077272,0.364903448065341),
 .UNSPECIFIED.);
#395=B_SPLINE_CURVE_WITH_KNOTS('',3,(#27076,#27077,#27078,#27079,#27080,
#27081,#27082,#27083,#27084,#27085,#27086,#27087,#27088,#27089,#27090,#27091,
#27092,#27093,#27094,#27095,#27096,#27097),.UNSPECIFIED.,.F.,.F.,(4,3,3,
3,3,3,3,4),(0.364903448065341,0.5,0.625,0.6875,0.75,0.8125,0.875,1.),
 .UNSPECIFIED.);
#396=B_SPLINE_CURVE_WITH_KNOTS('',3,(#27099,#27100,#27101,#27102,#27103,
#27104,#27105,#27106,#27107,#27108,#27109,#27110,#27111,#27112,#27113,#27114),
 .UNSPECIFIED.,.F.,.F.,(4,3,3,3,3,4),(8.50485119671489E-5,0.125,0.1875,
0.25,0.3125,0.339613136872108),.UNSPECIFIED.);
#397=B_SPLINE_CURVE_WITH_KNOTS('',1,(#27116,#27117),.UNSPECIFIED.,.F.,.F.,
(2,2),(-0.747935545358406,-0.734608691980728),.UNSPECIFIED.);
#398=B_SPLINE_CURVE_WITH_KNOTS('',3,(#27119,#27120,#27121,#27122,#27123,
#27124,#27125,#27126,#27127,#27128),.UNSPECIFIED.,.F.,.F.,(4,1,1,1,1,1,
1,4),(0.742143863244383,0.75,0.8125,0.84375,0.875,0.90625,0.9375,1.),
 .UNSPECIFIED.);
#399=B_SPLINE_CURVE_WITH_KNOTS('',3,(#27130,#27131,#27132,#27133,#27134,
#27135,#27136,#27137,#27138,#27139,#27140),.UNSPECIFIED.,.F.,.F.,(4,1,1,
1,1,1,1,1,4),(2.19745662600075E-7,0.0625,0.09375,0.125,0.15625,0.1875,0.25,
0.375,0.499885453205276),.UNSPECIFIED.);
#400=B_SPLINE_CURVE_WITH_KNOTS('',3,(#27142,#27143,#27144,#27145,#27146,
#27147,#27148,#27149,#27150,#27151,#27152,#27153),.UNSPECIFIED.,.F.,.F.,
(4,1,1,1,1,1,1,1,1,4),(0.5,0.625,0.6875,0.75,0.8125,0.84375,0.875,0.90625,
0.9375,0.999977328601928),.UNSPECIFIED.);
#401=B_SPLINE_CURVE_WITH_KNOTS('',3,(#27157,#27158,#27159,#27160,#27161,
#27162,#27163,#27164,#27165,#27166,#27167,#27168),.UNSPECIFIED.,.F.,.F.,
(4,1,1,1,1,1,1,1,1,4),(0.,0.0625,0.09375,0.125,0.15625,0.1875,0.25,0.3125,
0.375,0.5),.UNSPECIFIED.);
#402=B_SPLINE_CURVE_WITH_KNOTS('',3,(#27170,#27171,#27172,#27173,#27174,
#27175,#27176,#27177,#27178,#27179,#27180),.UNSPECIFIED.,.F.,.F.,(4,1,1,
1,1,1,1,1,4),(0.5,0.625,0.75,0.8125,0.84375,0.875,0.90625,0.9375,1.),
 .UNSPECIFIED.);
#403=B_SPLINE_CURVE_WITH_KNOTS('',3,(#27182,#27183,#27184,#27185,#27186,
#27187,#27188,#27189,#27190,#27191),.UNSPECIFIED.,.F.,.F.,(4,1,1,1,1,1,
1,4),(7.21673521508086E-6,0.0625,0.09375,0.125,0.15625,0.1875,0.25,0.257506245398161),
 .UNSPECIFIED.);
#404=B_SPLINE_CURVE_WITH_KNOTS('',1,(#27193,#27194),.UNSPECIFIED.,.F.,.F.,
(2,2),(-0.714609893047583,-0.701287175823169),.UNSPECIFIED.);
#405=B_SPLINE_CURVE_WITH_KNOTS('',3,(#27196,#27197,#27198,#27199,#27200,
#27201,#27202,#27203,#27204,#27205),.UNSPECIFIED.,.F.,.F.,(4,1,1,1,1,1,
1,4),(0.742719765959379,0.75,0.8125,0.84375,0.875,0.90625,0.9375,1.),
 .UNSPECIFIED.);
#406=B_SPLINE_CURVE_WITH_KNOTS('',3,(#27207,#27208,#27209,#27210,#27211,
#27212,#27213,#27214,#27215,#27216,#27217),.UNSPECIFIED.,.F.,.F.,(4,1,1,
1,1,1,1,1,4),(2.44735148634498E-7,0.0625,0.09375,0.125,0.15625,0.1875,0.25,
0.375,0.499888365983082),.UNSPECIFIED.);
#407=B_SPLINE_CURVE_WITH_KNOTS('',3,(#27219,#27220,#27221,#27222,#27223,
#27224,#27225,#27226,#27227,#27228,#27229,#27230),.UNSPECIFIED.,.F.,.F.,
(4,1,1,1,1,1,1,1,1,4),(0.5,0.625,0.6875,0.75,0.8125,0.84375,0.875,0.90625,
0.9375,1.),.UNSPECIFIED.);
#408=B_SPLINE_CURVE_WITH_KNOTS('',3,(#27234,#27235,#27236,#27237,#27238,
#27239,#27240,#27241,#27242,#27243,#27244,#27245),.UNSPECIFIED.,.F.,.F.,
(4,1,1,1,1,1,1,1,1,4),(0.,0.0625,0.09375,0.125,0.15625,0.1875,0.25,0.3125,
0.375,0.5),.UNSPECIFIED.);
#409=B_SPLINE_CURVE_WITH_KNOTS('',3,(#27247,#27248,#27249,#27250,#27251,
#27252,#27253,#27254,#27255,#27256,#27257),.UNSPECIFIED.,.F.,.F.,(4,1,1,
1,1,1,1,1,4),(0.5,0.625,0.75,0.8125,0.84375,0.875,0.90625,0.9375,1.),
 .UNSPECIFIED.);
#410=B_SPLINE_CURVE_WITH_KNOTS('',3,(#27259,#27260,#27261,#27262,#27263,
#27264,#27265,#27266,#27267,#27268),.UNSPECIFIED.,.F.,.F.,(4,1,1,1,1,1,
1,4),(6.46805633295331E-6,0.0625,0.09375,0.125,0.15625,0.1875,0.25,0.256944255797255),
 .UNSPECIFIED.);
#411=B_SPLINE_CURVE_WITH_KNOTS('',1,(#27270,#27271),.UNSPECIFIED.,.F.,.F.,
(2,2),(-0.681288387796028,-0.667963314640389),.UNSPECIFIED.);
#412=B_SPLINE_CURVE_WITH_KNOTS('',3,(#27273,#27274,#27275,#27276,#27277,
#27278,#27279,#27280,#27281,#27282),.UNSPECIFIED.,.F.,.F.,(4,1,1,1,1,1,
1,4),(0.743178274051315,0.75,0.8125,0.84375,0.875,0.90625,0.9375,1.),
 .UNSPECIFIED.);
#413=B_SPLINE_CURVE_WITH_KNOTS('',3,(#27284,#27285,#27286,#27287,#27288,
#27289,#27290,#27291,#27292,#27293,#27294),.UNSPECIFIED.,.F.,.F.,(4,1,1,
1,1,1,1,1,4),(1.8821041512382E-7,0.0625,0.09375,0.125,0.15625,0.1875,0.25,
0.375,0.499902076873613),.UNSPECIFIED.);
#414=B_SPLINE_CURVE_WITH_KNOTS('',3,(#27296,#27297,#27298,#27299,#27300,
#27301,#27302,#27303,#27304,#27305,#27306,#27307),.UNSPECIFIED.,.F.,.F.,
(4,1,1,1,1,1,1,1,1,4),(0.5,0.625,0.6875,0.75,0.8125,0.84375,0.875,0.90625,
0.9375,1.),.UNSPECIFIED.);
#415=B_SPLINE_CURVE_WITH_KNOTS('',3,(#27309,#27310,#27311,#27312,#27313,
#27314,#27315,#27316,#27317,#27318,#27319,#27320,#27321,#27322,#27323,#27324,
#27325,#27326,#27327,#27328,#27329,#27330,#27331,#27332,#27333,#27334,#27335,
#27336,#27337,#27338,#27339),.UNSPECIFIED.,.F.,.F.,(4,3,3,3,3,3,3,3,3,3,
4),(0.000195514036727322,0.0625,0.125,0.1875,0.25,0.375,0.5,0.625,0.75,
0.875,0.999997646068875),.UNSPECIFIED.);
#416=B_SPLINE_CURVE_WITH_KNOTS('',3,(#27341,#27342,#27343,#27344,#27345,
#27346,#27347,#27348,#27349,#27350,#27351,#27352,#27353),.UNSPECIFIED.,
 .F.,.F.,(4,1,1,1,1,1,1,1,1,1,4),(0.,0.0625,0.09375,0.125,0.15625,0.1875,
0.25,0.3125,0.375,0.5,0.500672802403104),.UNSPECIFIED.);
#417=B_SPLINE_CURVE_WITH_KNOTS('',3,(#27355,#27356,#27357,#27358,#27359,
#27360,#27361,#27362,#27363,#27364,#27365),.UNSPECIFIED.,.F.,.F.,(4,1,1,
1,1,1,1,1,4),(0.500672802403104,0.625,0.75,0.8125,0.84375,0.875,0.90625,
0.9375,0.999999779246756),.UNSPECIFIED.);
#418=B_SPLINE_CURVE_WITH_KNOTS('',3,(#27367,#27368,#27369,#27370,#27371,
#27372,#27373,#27374,#27375,#27376),.UNSPECIFIED.,.F.,.F.,(4,1,1,1,1,1,
1,4),(0.,0.0625,0.09375,0.125,0.15625,0.1875,0.25,0.271066582727647),
 .UNSPECIFIED.);
#419=B_SPLINE_CURVE_WITH_KNOTS('',1,(#27378,#27379),.UNSPECIFIED.,.F.,.F.,
(2,2),(-0.647962203600483,-0.634635368538325),.UNSPECIFIED.);
#420=B_SPLINE_CURVE_WITH_KNOTS('',3,(#27381,#27382,#27383,#27384,#27385,
#27386,#27387,#27388,#27389,#27390),.UNSPECIFIED.,.F.,.F.,(4,1,1,1,1,1,
1,4),(0.71355566892686,0.75,0.8125,0.84375,0.875,0.90625,0.9375,1.),
 .UNSPECIFIED.);
#421=B_SPLINE_CURVE_WITH_KNOTS('',3,(#27392,#27393,#27394,#27395),
 .UNSPECIFIED.,.F.,.F.,(4,4),(0.951039109725656,0.999996744713042),
 .UNSPECIFIED.);
#422=B_SPLINE_CURVE_WITH_KNOTS('',3,(#27397,#27398,#27399,#27400,#27401,
#27402,#27403,#27404,#27405,#27406,#27407,#27408,#27409,#27410,#27411,#27412,
#27413,#27414,#27415,#27416,#27417,#27418,#27419,#27420,#27421,#27422,#27423,
#27424),.UNSPECIFIED.,.F.,.F.,(4,3,3,3,3,3,3,3,3,4),(0.584078652551858,
0.59375,0.625,0.6875,0.71875,0.75,0.78125,0.8125,0.875,0.951039109725656),
 .UNSPECIFIED.);
#423=B_SPLINE_CURVE_WITH_KNOTS('',3,(#27426,#27427,#27428,#27429,#27430,
#27431,#27432,#27433,#27434,#27435,#27436,#27437,#27438,#27439,#27440,#27441,
#27442,#27443,#27444,#27445,#27446,#27447,#27448,#27449,#27450,#27451,#27452,
#27453,#27454,#27455,#27456,#27457,#27458,#27459,#27460,#27461,#27462,#27463,
#27464,#27465,#27466,#27467,#27468,#27469,#27470,#27471,#27472,#27473,#27474),
 .UNSPECIFIED.,.F.,.F.,(4,3,3,3,3,3,3,3,3,3,3,3,3,3,3,3,4),(0.125,0.15625,
0.1875,0.21875,0.25,0.3125,0.375,0.40625,0.434649092523259,0.4375,0.46875,
0.484375,0.5,0.515625,0.53125,0.5625,0.584078652551858),.UNSPECIFIED.);
#424=B_SPLINE_CURVE_WITH_KNOTS('',3,(#27476,#27477,#27478,#27479,#27480,
#27481,#27482),.UNSPECIFIED.,.F.,.F.,(4,3,4),(1.0214071444072E-5,0.0625,
0.125),.UNSPECIFIED.);
#425=B_SPLINE_CURVE_WITH_KNOTS('',3,(#27484,#27485,#27486,#27487,#27488,
#27489,#27490,#27491),.UNSPECIFIED.,.F.,.F.,(4,1,1,1,1,4),(7.73334121881107E-5,
0.0625,0.125,0.25,0.375,0.499602040488809),.UNSPECIFIED.);
#426=B_SPLINE_CURVE_WITH_KNOTS('',3,(#27493,#27494,#27495,#27496,#27497,
#27498,#27499),.UNSPECIFIED.,.F.,.F.,(4,1,1,1,4),(0.5,0.625,0.75,0.875,
0.999994675291189),.UNSPECIFIED.);
#427=B_SPLINE_CURVE_WITH_KNOTS('',3,(#27501,#27502,#27503,#27504,#27505,
#27506,#27507,#27508,#27509,#27510,#27511,#27512,#27513,#27514,#27515,#27516,
#27517,#27518,#27519,#27520,#27521,#27522,#27523,#27524,#27525,#27526,#27527,
#27528),.UNSPECIFIED.,.F.,.F.,(4,3,3,3,3,3,3,3,3,4),(0.,0.0625,0.09375,
0.125,0.15625,0.1875,0.25,0.375,0.5,0.500630475285163),.UNSPECIFIED.);
#428=B_SPLINE_CURVE_WITH_KNOTS('',3,(#27530,#27531,#27532,#27533,#27534,
#27535,#27536,#27537,#27538,#27539,#27540,#27541,#27542,#27543,#27544,#27545,
#27546,#27547,#27548,#27549,#27550,#27551,#27552,#27553,#27554),
 .UNSPECIFIED.,.F.,.F.,(4,3,3,3,3,3,3,3,4),(0.500630475285163,0.625,0.6875,
0.71875,0.75,0.78125,0.8125,0.875,0.999999745637335),.UNSPECIFIED.);
#429=B_SPLINE_CURVE_WITH_KNOTS('',3,(#27556,#27557,#27558,#27559,#27560,
#27561,#27562,#27563,#27564,#27565,#27566,#27567,#27568,#27569,#27570,#27571,
#27572,#27573,#27574),.UNSPECIFIED.,.F.,.F.,(4,3,3,3,3,3,4),(0.,0.125,0.1875,
0.21875,0.25,0.28125,0.295540353636982),.UNSPECIFIED.);
#430=B_SPLINE_CURVE_WITH_KNOTS('',1,(#27576,#27577),.UNSPECIFIED.,.F.,.F.,
(2,2),(-0.614701012907286,-0.601354554659112),.UNSPECIFIED.);
#431=B_SPLINE_CURVE_WITH_KNOTS('',3,(#27579,#27580,#27581,#27582,#27583,
#27584,#27585,#27586,#27587,#27588,#27589,#27590,#27591,#27592,#27593,#27594,
#27595,#27596,#27597),.UNSPECIFIED.,.F.,.F.,(4,3,3,3,3,3,4),(0.699974107082008,
0.71875,0.75,0.78125,0.8125,0.875,0.999999882359552),.UNSPECIFIED.);
#432=B_SPLINE_CURVE_WITH_KNOTS('',3,(#27599,#27600,#27601,#27602,#27603,
#27604,#27605,#27606,#27607,#27608,#27609,#27610,#27611,#27612,#27613,#27614,
#27615,#27616,#27617,#27618,#27619,#27620,#27621,#27622,#27623),
 .UNSPECIFIED.,.F.,.F.,(4,3,3,3,3,3,3,3,4),(0.,0.125,0.1875,0.21875,0.25,
0.28125,0.3125,0.375,0.5),.UNSPECIFIED.);
#433=B_SPLINE_CURVE_WITH_KNOTS('',3,(#27625,#27626,#27627,#27628,#27629,
#27630,#27631,#27632,#27633,#27634,#27635,#27636,#27637,#27638,#27639,#27640,
#27641,#27642,#27643,#27644,#27645,#27646,#27647,#27648,#27649,#27650,#27651,
#27652),.UNSPECIFIED.,.F.,.F.,(4,3,3,3,3,3,3,3,3,4),(0.5,0.625,0.636099191630217,
0.75,0.8125,0.84375,0.875,0.90625,0.9375,1.),.UNSPECIFIED.);
#434=B_SPLINE_CURVE_WITH_KNOTS('',3,(#27656,#27657,#27658,#27659,#27660,
#27661,#27662,#27663,#27664,#27665,#27666,#27667,#27668,#27669,#27670,#27671,
#27672,#27673,#27674),.UNSPECIFIED.,.F.,.F.,(4,1,1,1,1,1,1,1,1,1,1,1,1,
1,1,1,4),(0.,0.0625,0.09375,0.125,0.15625,0.1875,0.25,0.375,0.5,0.625,0.6875,
0.71875,0.75,0.78125,0.8125,0.875,0.9999997812994),.UNSPECIFIED.);
#435=B_SPLINE_CURVE_WITH_KNOTS('',3,(#27676,#27677,#27678,#27679,#27680,
#27681,#27682,#27683,#27684),.UNSPECIFIED.,.F.,.F.,(4,1,1,1,1,1,4),(0.,
0.125,0.1875,0.21875,0.25,0.28125,0.302671489156909),.UNSPECIFIED.);
#436=B_SPLINE_CURVE_WITH_KNOTS('',1,(#27686,#27687),.UNSPECIFIED.,.F.,.F.,
(2,2),(-0.581356766185651,-0.567943718980148),.UNSPECIFIED.);
#437=B_SPLINE_CURVE_WITH_KNOTS('',3,(#27689,#27690,#27691,#27692,#27693,
#27694,#27695,#27696,#27697,#27698,#27699,#27700,#27701,#27702,#27703,#27704,
#27705,#27706,#27707,#27708,#27709,#27710),.UNSPECIFIED.,.F.,.F.,(4,3,3,
3,3,3,3,4),(0.690961556714303,0.75,0.8125,0.84375,0.875,0.90625,0.9375,
1.),.UNSPECIFIED.);
#438=B_SPLINE_CURVE_WITH_KNOTS('',3,(#27712,#27713,#27714,#27715,#27716,
#27717,#27718,#27719,#27720,#27721,#27722,#27723,#27724,#27725,#27726,#27727,
#27728,#27729,#27730,#27731,#27732,#27733,#27734,#27735,#27736,#27737,#27738,
#27739,#27740,#27741,#27742,#27743,#27744,#27745,#27746,#27747,#27748,#27749,
#27750,#27751,#27752,#27753,#27754,#27755,#27756,#27757,#27758,#27759,#27760,
#27761,#27762,#27763,#27764,#27765,#27766,#27767,#27768,#27769),
 .UNSPECIFIED.,.F.,.F.,(4,3,3,3,3,3,3,3,3,3,3,3,3,3,3,3,3,3,3,4),(8.74756603760378E-8,
0.0625,0.09375,0.125,0.15625,0.1875,0.25,0.3125,0.375,0.5,0.625,0.653701494884754,
0.6875,0.75,0.8125,0.84375,0.875,0.90625,0.9375,0.999999836811042),
 .UNSPECIFIED.);
#439=B_SPLINE_CURVE_WITH_KNOTS('',3,(#27773,#27774,#27775,#27776,#27777,
#27778,#27779,#27780,#27781,#27782,#27783,#27784,#27785,#27786,#27787,#27788,
#27789,#27790,#27791,#27792,#27793),.UNSPECIFIED.,.F.,.F.,(4,1,1,1,1,1,
1,1,1,1,1,1,1,1,1,1,1,1,4),(2.76904502469975E-7,0.0625,0.09375,0.125,0.15625,
0.1875,0.25,0.3125,0.375,0.5,0.625,0.6875,0.75,0.8125,0.84375,0.875,0.90625,
0.9375,0.999999617215634),.UNSPECIFIED.);
#440=B_SPLINE_CURVE_WITH_KNOTS('',3,(#27795,#27796,#27797,#27798,#27799,
#27800,#27801,#27802,#27803,#27804),.UNSPECIFIED.,.F.,.F.,(4,1,1,1,1,1,
1,4),(0.,0.0625,0.09375,0.125,0.15625,0.1875,0.25,0.308404661026527),
 .UNSPECIFIED.);
#441=B_SPLINE_CURVE_WITH_KNOTS('',1,(#27806,#27807),.UNSPECIFIED.,.F.,.F.,
(2,2),(-0.547952025403732,-0.534632217745046),.UNSPECIFIED.);
#442=B_SPLINE_CURVE_WITH_KNOTS('',3,(#27809,#27810,#27811,#27812,#27813,
#27814,#27815,#27816,#27817,#27818,#27819,#27820,#27821,#27822,#27823,#27824,
#27825,#27826,#27827,#27828,#27829,#27830),.UNSPECIFIED.,.F.,.F.,(4,3,3,
3,3,3,3,4),(0.691764098829342,0.75,0.8125,0.84375,0.875,0.90625,0.9375,
1.),.UNSPECIFIED.);
#443=B_SPLINE_CURVE_WITH_KNOTS('',3,(#27832,#27833,#27834,#27835,#27836,
#27837,#27838,#27839,#27840,#27841,#27842,#27843,#27844,#27845,#27846,#27847,
#27848,#27849,#27850,#27851,#27852,#27853,#27854,#27855,#27856,#27857,#27858,
#27859,#27860,#27861,#27862,#27863,#27864,#27865,#27866,#27867,#27868,#27869,
#27870,#27871,#27872,#27873,#27874,#27875,#27876,#27877,#27878,#27879,#27880,
#27881,#27882,#27883,#27884,#27885,#27886,#27887,#27888,#27889),
 .UNSPECIFIED.,.F.,.F.,(4,3,3,3,3,3,3,3,3,3,3,3,3,3,3,3,3,3,3,4),(6.60130104707959E-8,
0.0625,0.09375,0.125,0.15625,0.1875,0.25,0.3125,0.375,0.5,0.625,0.651822706730315,
0.6875,0.75,0.8125,0.84375,0.875,0.90625,0.9375,0.999999831175229),
 .UNSPECIFIED.);
#444=B_SPLINE_CURVE_WITH_KNOTS('',3,(#27893,#27894,#27895,#27896,#27897,
#27898,#27899,#27900,#27901,#27902,#27903,#27904,#27905,#27906,#27907,#27908,
#27909,#27910,#27911,#27912,#27913),.UNSPECIFIED.,.F.,.F.,(4,1,1,1,1,1,
1,1,1,1,1,1,1,1,1,1,1,1,4),(2.85246569633639E-7,0.0625,0.09375,0.125,0.15625,
0.1875,0.25,0.3125,0.375,0.5,0.625,0.6875,0.75,0.8125,0.84375,0.875,0.90625,
0.9375,0.999999654885251),.UNSPECIFIED.);
#445=B_SPLINE_CURVE_WITH_KNOTS('',3,(#27915,#27916,#27917,#27918,#27919,
#27920,#27921,#27922,#27923,#27924),.UNSPECIFIED.,.F.,.F.,(4,1,1,1,1,1,
1,4),(0.,0.0625,0.09375,0.125,0.15625,0.1875,0.25,0.307485444826301),
 .UNSPECIFIED.);
#446=B_SPLINE_CURVE_WITH_KNOTS('',1,(#27926,#27927),.UNSPECIFIED.,.F.,.F.,
(2,2),(-0.514641034236103,-0.501321659607129),.UNSPECIFIED.);
#447=B_SPLINE_CURVE_WITH_KNOTS('',3,(#27929,#27930,#27931,#27932,#27933,
#27934,#27935,#27936,#27937,#27938),.UNSPECIFIED.,.F.,.F.,(4,1,1,1,1,1,
1,4),(0.692733007429323,0.75,0.8125,0.84375,0.875,0.90625,0.9375,1.),
 .UNSPECIFIED.);
#448=B_SPLINE_CURVE_WITH_KNOTS('',3,(#27940,#27941,#27942,#27943,#27944,
#27945,#27946,#27947,#27948,#27949,#27950,#27951,#27952,#27953,#27954,#27955,
#27956,#27957,#27958,#27959,#27960,#27961,#27962,#27963,#27964,#27965,#27966,
#27967,#27968,#27969,#27970,#27971,#27972,#27973,#27974,#27975,#27976,#27977,
#27978,#27979,#27980,#27981,#27982,#27983,#27984,#27985,#27986,#27987,#27988,
#27989,#27990,#27991,#27992,#27993,#27994,#27995,#27996,#27997),
 .UNSPECIFIED.,.F.,.F.,(4,3,3,3,3,3,3,3,3,3,3,3,3,3,3,3,3,3,3,4),(3.79295315668372E-8,
0.0625,0.09375,0.125,0.15625,0.1875,0.25,0.3125,0.375,0.5,0.625,0.64975298249665,
0.6875,0.75,0.8125,0.84375,0.875,0.90625,0.9375,0.999999823692408),
 .UNSPECIFIED.);
#449=B_SPLINE_CURVE_WITH_KNOTS('',3,(#28001,#28002,#28003,#28004,#28005,
#28006,#28007,#28008,#28009,#28010,#28011,#28012,#28013,#28014,#28015,#28016,
#28017,#28018,#28019,#28020,#28021),.UNSPECIFIED.,.F.,.F.,(4,1,1,1,1,1,
1,1,1,1,1,1,1,1,1,1,1,1,4),(2.85268618544073E-7,0.0625,0.09375,0.125,0.15625,
0.1875,0.25,0.3125,0.375,0.5,0.625,0.6875,0.75,0.8125,0.84375,0.875,0.90625,
0.9375,0.999999714317637),.UNSPECIFIED.);
#450=B_SPLINE_CURVE_WITH_KNOTS('',3,(#28023,#28024,#28025,#28026,#28027,
#28028,#28029,#28030,#28031,#28032),.UNSPECIFIED.,.F.,.F.,(4,1,1,1,1,1,
1,4),(0.,0.0625,0.09375,0.125,0.15625,0.1875,0.25,0.306675627321796),
 .UNSPECIFIED.);
#451=B_SPLINE_CURVE_WITH_KNOTS('',1,(#28034,#28035),.UNSPECIFIED.,.F.,.F.,
(2,2),(-0.481330907823224,-0.468014532967897),.UNSPECIFIED.);
#452=B_SPLINE_CURVE_WITH_KNOTS('',3,(#28037,#28038,#28039,#28040,#28041,
#28042,#28043,#28044,#28045,#28046),.UNSPECIFIED.,.F.,.F.,(4,1,1,1,1,1,
1,4),(0.693739351488113,0.75,0.8125,0.84375,0.875,0.90625,0.9375,1.),
 .UNSPECIFIED.);
#453=B_SPLINE_CURVE_WITH_KNOTS('',3,(#28048,#28049,#28050,#28051,#28052,
#28053,#28054,#28055,#28056,#28057,#28058,#28059,#28060,#28061,#28062,#28063,
#28064,#28065,#28066,#28067,#28068,#28069,#28070,#28071,#28072,#28073,#28074,
#28075,#28076,#28077,#28078,#28079,#28080,#28081,#28082,#28083,#28084,#28085,
#28086,#28087,#28088,#28089,#28090,#28091,#28092,#28093,#28094,#28095,#28096,
#28097,#28098,#28099,#28100,#28101,#28102,#28103,#28104,#28105),
 .UNSPECIFIED.,.F.,.F.,(4,3,3,3,3,3,3,3,3,3,3,3,3,3,3,3,3,3,3,4),(2.59941942783721E-8,
0.0625,0.09375,0.125,0.15625,0.1875,0.25,0.3125,0.375,0.5,0.625,0.647786928436969,
0.6875,0.75,0.8125,0.84375,0.875,0.90625,0.9375,0.999999815530093),
 .UNSPECIFIED.);
#454=B_SPLINE_CURVE_WITH_KNOTS('',3,(#28109,#28110,#28111,#28112,#28113,
#28114,#28115,#28116,#28117,#28118,#28119,#28120,#28121,#28122,#28123,#28124,
#28125,#28126,#28127,#28128,#28129),.UNSPECIFIED.,.F.,.F.,(4,1,1,1,1,1,
1,1,1,1,1,1,1,1,1,1,1,1,4),(2.82907565420154E-7,0.0625,0.09375,0.125,0.15625,
0.1875,0.25,0.3125,0.375,0.5,0.625,0.6875,0.75,0.8125,0.84375,0.875,0.90625,
0.9375,0.99999978184527),.UNSPECIFIED.);
#455=B_SPLINE_CURVE_WITH_KNOTS('',3,(#28131,#28132,#28133,#28134,#28135,
#28136,#28137,#28138,#28139,#28140),.UNSPECIFIED.,.F.,.F.,(4,1,1,1,1,1,
1,4),(0.,0.0625,0.09375,0.125,0.15625,0.1875,0.25,0.305513267453618),
 .UNSPECIFIED.);
#456=B_SPLINE_CURVE_WITH_KNOTS('',1,(#28142,#28143),.UNSPECIFIED.,.F.,.F.,
(2,2),(-0.448026172671341,-0.434710029955949),.UNSPECIFIED.);
#457=B_SPLINE_CURVE_WITH_KNOTS('',3,(#28145,#28146,#28147,#28148,#28149,
#28150,#28151,#28152,#28153,#28154),.UNSPECIFIED.,.F.,.F.,(4,1,1,1,1,1,
1,4),(0.69476673108169,0.75,0.8125,0.84375,0.875,0.90625,0.9375,1.),
 .UNSPECIFIED.);
#458=B_SPLINE_CURVE_WITH_KNOTS('',3,(#28156,#28157,#28158,#28159,#28160,
#28161,#28162,#28163,#28164,#28165,#28166,#28167,#28168,#28169,#28170,#28171,
#28172,#28173,#28174,#28175,#28176),.UNSPECIFIED.,.F.,.F.,(4,1,1,1,1,1,
1,1,1,1,1,1,1,1,1,1,1,1,4),(1.10928375193975E-8,0.0625,0.09375,0.125,0.15625,
0.1875,0.25,0.3125,0.375,0.5,0.625,0.6875,0.75,0.8125,0.84375,0.875,0.90625,
0.9375,0.999999806606368),.UNSPECIFIED.);
#459=B_SPLINE_CURVE_WITH_KNOTS('',3,(#28180,#28181,#28182,#28183,#28184,
#28185,#28186,#28187,#28188,#28189,#28190,#28191,#28192,#28193,#28194,#28195,
#28196,#28197,#28198,#28199,#28200),.UNSPECIFIED.,.F.,.F.,(4,1,1,1,1,1,
1,1,1,1,1,1,1,1,1,1,1,1,4),(2.78980747991976E-7,0.0625,0.09375,0.125,0.15625,
0.1875,0.25,0.3125,0.375,0.5,0.625,0.6875,0.75,0.8125,0.84375,0.875,0.90625,
0.9375,0.99999982218199),.UNSPECIFIED.);
#460=B_SPLINE_CURVE_WITH_KNOTS('',3,(#28202,#28203,#28204,#28205,#28206,
#28207,#28208,#28209,#28210,#28211),.UNSPECIFIED.,.F.,.F.,(4,1,1,1,1,1,
1,4),(0.,0.0625,0.09375,0.125,0.15625,0.1875,0.25,0.304441335563685),
 .UNSPECIFIED.);
#461=B_SPLINE_CURVE_WITH_KNOTS('',1,(#28213,#28214),.UNSPECIFIED.,.F.,.F.,
(2,2),(-0.414721936888564,-0.401409886337017),.UNSPECIFIED.);
#462=B_SPLINE_CURVE_WITH_KNOTS('',3,(#28216,#28217,#28218,#28219,#28220,
#28221,#28222,#28223,#28224,#28225,#28226,#28227,#28228,#28229,#28230,#28231),
 .UNSPECIFIED.,.F.,.F.,(4,3,3,3,3,4),(0.694959544378405,0.75,0.8125,0.84375,
0.875,0.999999985529887),.UNSPECIFIED.);
#463=B_SPLINE_CURVE_WITH_KNOTS('',3,(#28233,#28234,#28235,#28236,#28237,
#28238,#28239,#28240,#28241,#28242,#28243,#28244,#28245,#28246,#28247,#28248,
#28249,#28250,#28251,#28252,#28253),.UNSPECIFIED.,.F.,.F.,(4,1,1,1,1,1,
1,1,1,1,1,1,1,1,1,1,1,1,4),(0.,0.0625,0.09375,0.125,0.15625,0.1875,0.25,
0.3125,0.375,0.5,0.625,0.6875,0.75,0.8125,0.84375,0.875,0.90625,0.9375,
0.99999979724297),.UNSPECIFIED.);
#464=B_SPLINE_CURVE_WITH_KNOTS('',3,(#28257,#28258,#28259,#28260,#28261,
#28262),.UNSPECIFIED.,.F.,.F.,(4,2,4),(-0.386843013885963,-0.22816224008248,
-0.000106862707127469),.UNSPECIFIED.);
#465=B_SPLINE_CURVE_WITH_KNOTS('',3,(#28264,#28265,#28266,#28267,#28268,
#28269,#28270,#28271,#28272),.UNSPECIFIED.,.F.,.F.,(4,1,1,1,1,1,4),(0.,
0.125,0.1875,0.21875,0.25,0.28125,0.302853998408664),.UNSPECIFIED.);
#466=B_SPLINE_CURVE_WITH_KNOTS('',1,(#28274,#28275),.UNSPECIFIED.,.F.,.F.,
(2,2),(-0.38141833719901,-0.368114143248423),.UNSPECIFIED.);
#467=B_SPLINE_CURVE_WITH_KNOTS('',3,(#28277,#28278,#28279,#28280,#28281,
#28282,#28283,#28284,#28285,#28286,#28287,#28288,#28289,#28290,#28291,#28292,
#28293,#28294,#28295),.UNSPECIFIED.,.F.,.F.,(4,3,3,3,3,3,4),(0.697655525115426,
0.71875,0.75,0.78125,0.8125,0.875,1.),.UNSPECIFIED.);
#468=B_SPLINE_CURVE_WITH_KNOTS('',3,(#28297,#28298,#28299,#28300,#28301,
#28302,#28303,#28304,#28305,#28306,#28307,#28308,#28309,#28310,#28311,#28312,
#28313,#28314,#28315,#28316,#28317,#28318,#28319,#28320,#28321,#28322,#28323,
#28324,#28325,#28326,#28327,#28328,#28329,#28330,#28331,#28332,#28333,#28334,
#28335,#28336,#28337,#28338,#28339,#28340,#28341,#28342,#28343,#28344,#28345,
#28346,#28347,#28348),.UNSPECIFIED.,.F.,.F.,(4,3,3,3,3,3,3,3,3,3,3,3,3,
3,3,3,3,4),(3.40252582782886E-8,0.125,0.1875,0.21875,0.25,0.28125,0.3125,
0.375,0.5,0.625,0.641085058040362,0.75,0.8125,0.84375,0.875,0.90625,0.9375,
0.999999822300934),.UNSPECIFIED.);
#469=B_SPLINE_CURVE_WITH_KNOTS('',3,(#28352,#28353,#28354,#28355,#28356,
#28357,#28358,#28359,#28360,#28361,#28362,#28363,#28364,#28365,#28366,#28367,
#28368,#28369,#28370,#28371,#28372,#28373,#28374,#28375,#28376,#28377,#28378,
#28379,#28380,#28381,#28382,#28383,#28384,#28385,#28386,#28387,#28388,#28389,
#28390,#28391,#28392,#28393,#28394,#28395,#28396,#28397,#28398,#28399,#28400,
#28401,#28402,#28403),.UNSPECIFIED.,.F.,.F.,(4,3,3,3,3,3,3,3,3,3,3,3,3,
3,3,3,3,4),(0.,0.0625,0.09375,0.125,0.15625,0.1875,0.25,0.360119793928473,
0.375,0.5,0.625,0.6875,0.71875,0.75,0.78125,0.8125,0.875,1.),
 .UNSPECIFIED.);
#470=B_SPLINE_CURVE_WITH_KNOTS('',3,(#28405,#28406,#28407,#28408,#28409,
#28410,#28411,#28412,#28413),.UNSPECIFIED.,.F.,.F.,(4,1,1,1,1,1,4),(0.,
0.125,0.1875,0.21875,0.25,0.28125,0.301839172550323),.UNSPECIFIED.);
#471=B_SPLINE_CURVE_WITH_KNOTS('',1,(#28415,#28416),.UNSPECIFIED.,.F.,.F.,
(2,2),(-0.348122442733603,-0.334802618107589),.UNSPECIFIED.);
#472=B_SPLINE_CURVE_WITH_KNOTS('',3,(#28418,#28419,#28420,#28421,#28422,
#28423,#28424,#28425,#28426,#28427,#28428,#28429,#28430,#28431,#28432,#28433,
#28434,#28435,#28436),.UNSPECIFIED.,.F.,.F.,(4,3,3,3,3,3,4),(0.698643471576761,
0.71875,0.75,0.78125,0.8125,0.875,1.),.UNSPECIFIED.);
#473=B_SPLINE_CURVE_WITH_KNOTS('',3,(#28438,#28439,#28440,#28441,#28442,
#28443,#28444,#28445,#28446,#28447,#28448,#28449,#28450,#28451,#28452,#28453,
#28454,#28455,#28456,#28457,#28458,#28459,#28460,#28461,#28462,#28463,#28464,
#28465,#28466,#28467,#28468,#28469,#28470,#28471,#28472,#28473,#28474,#28475,
#28476,#28477,#28478,#28479,#28480,#28481,#28482,#28483,#28484,#28485,#28486,
#28487,#28488,#28489),.UNSPECIFIED.,.F.,.F.,(4,3,3,3,3,3,3,3,3,3,3,3,3,
3,3,3,3,4),(6.90927897239085E-8,0.125,0.1875,0.21875,0.25,0.28125,0.3125,
0.375,0.5,0.625,0.639344739454029,0.75,0.8125,0.84375,0.875,0.90625,0.9375,
0.999999825004712),.UNSPECIFIED.);
#474=B_SPLINE_CURVE_WITH_KNOTS('',3,(#28493,#28494,#28495,#28496,#28497,
#28498,#28499,#28500,#28501,#28502,#28503,#28504,#28505,#28506,#28507,#28508,
#28509,#28510,#28511,#28512,#28513,#28514,#28515,#28516,#28517,#28518,#28519,
#28520,#28521,#28522,#28523,#28524,#28525,#28526,#28527,#28528,#28529,#28530,
#28531,#28532,#28533,#28534,#28535,#28536,#28537,#28538,#28539,#28540,#28541,
#28542,#28543,#28544),.UNSPECIFIED.,.F.,.F.,(4,3,3,3,3,3,3,3,3,3,3,3,3,
3,3,3,3,4),(1.74218079178612E-7,0.0625,0.09375,0.125,0.15625,0.1875,0.25,
0.361910921352633,0.375,0.5,0.625,0.6875,0.71875,0.75,0.78125,0.8125,0.875,
1.),.UNSPECIFIED.);
#475=B_SPLINE_CURVE_WITH_KNOTS('',3,(#28546,#28547,#28548,#28549,#28550,
#28551,#28552,#28553,#28554),.UNSPECIFIED.,.F.,.F.,(4,1,1,1,1,1,4),(0.,
0.125,0.1875,0.21875,0.25,0.28125,0.300810905459472),.UNSPECIFIED.);
#476=B_SPLINE_CURVE_WITH_KNOTS('',1,(#28556,#28557),.UNSPECIFIED.,.F.,.F.,
(2,2),(-0.314810126318466,-0.30149018112365),.UNSPECIFIED.);
#477=B_SPLINE_CURVE_WITH_KNOTS('',3,(#28559,#28560,#28561,#28562,#28563,
#28564,#28565,#28566,#28567,#28568,#28569,#28570,#28571,#28572,#28573,#28574,
#28575,#28576,#28577),.UNSPECIFIED.,.F.,.F.,(4,3,3,3,3,3,4),(0.699678783356034,
0.71875,0.75,0.78125,0.8125,0.875,1.),.UNSPECIFIED.);
#478=B_SPLINE_CURVE_WITH_KNOTS('',3,(#28579,#28580,#28581,#28582,#28583,
#28584,#28585,#28586,#28587,#28588,#28589,#28590,#28591,#28592,#28593,#28594,
#28595,#28596,#28597,#28598,#28599,#28600,#28601,#28602,#28603,#28604,#28605,
#28606,#28607,#28608,#28609,#28610,#28611,#28612,#28613,#28614,#28615,#28616,
#28617,#28618,#28619,#28620,#28621,#28622,#28623,#28624,#28625,#28626,#28627,
#28628,#28629,#28630),.UNSPECIFIED.,.F.,.F.,(4,3,3,3,3,3,3,3,3,3,3,3,3,
3,3,3,3,4),(7.65381569237967E-8,0.125,0.1875,0.21875,0.25,0.28125,0.3125,
0.375,0.5,0.625,0.637564576525894,0.75,0.8125,0.84375,0.875,0.90625,0.9375,
0.999999824573213),.UNSPECIFIED.);
#479=B_SPLINE_CURVE_WITH_KNOTS('',3,(#28634,#28635,#28636,#28637,#28638,
#28639,#28640,#28641,#28642,#28643,#28644,#28645,#28646,#28647,#28648,#28649,
#28650,#28651,#28652),.UNSPECIFIED.,.F.,.F.,(4,1,1,1,1,1,1,1,1,1,1,1,1,
1,1,1,4),(2.68538809727287E-7,0.0625,0.09375,0.125,0.15625,0.1875,0.25,
0.375,0.5,0.625,0.6875,0.71875,0.75,0.78125,0.8125,0.875,1.),
 .UNSPECIFIED.);
#480=B_SPLINE_CURVE_WITH_KNOTS('',3,(#28654,#28655,#28656,#28657,#28658,
#28659,#28660,#28661,#28662),.UNSPECIFIED.,.F.,.F.,(4,1,1,1,1,1,4),(1.72862727219145E-8,
0.125,0.1875,0.21875,0.25,0.28125,0.299787333569703),.UNSPECIFIED.);
#481=B_SPLINE_CURVE_WITH_KNOTS('',1,(#28664,#28665),.UNSPECIFIED.,.F.,.F.,
(2,2),(-0.281497700229318,-0.268175969207313),.UNSPECIFIED.);
#482=B_SPLINE_CURVE_WITH_KNOTS('',3,(#28667,#28668,#28669,#28670,#28671,
#28672,#28673,#28674,#28675,#28676,#28677,#28678,#28679,#28680,#28681,#28682,
#28683,#28684,#28685),.UNSPECIFIED.,.F.,.F.,(4,3,3,3,3,3,4),(0.700679367798627,
0.71875,0.75,0.78125,0.8125,0.875,0.999999976169426),.UNSPECIFIED.);
#483=B_SPLINE_CURVE_WITH_KNOTS('',3,(#28687,#28688,#28689,#28690,#28691,
#28692,#28693,#28694,#28695,#28696,#28697,#28698,#28699,#28700,#28701,#28702,
#28703,#28704,#28705,#28706,#28707,#28708,#28709,#28710,#28711,#28712,#28713,
#28714,#28715,#28716,#28717,#28718,#28719,#28720,#28721,#28722,#28723,#28724,
#28725,#28726,#28727,#28728,#28729,#28730,#28731,#28732,#28733,#28734,#28735,
#28736,#28737,#28738),.UNSPECIFIED.,.F.,.F.,(4,3,3,3,3,3,3,3,3,3,3,3,3,
3,3,3,3,4),(0.,0.125,0.1875,0.21875,0.25,0.28125,0.3125,0.375,0.5,0.625,
0.635605727697318,0.75,0.8125,0.84375,0.875,0.90625,0.9375,0.999999821937738),
 .UNSPECIFIED.);
#484=B_SPLINE_CURVE_WITH_KNOTS('',3,(#28742,#28743,#28744,#28745,#28746,
#28747,#28748,#28749,#28750,#28751,#28752,#28753,#28754,#28755,#28756,#28757,
#28758,#28759,#28760),.UNSPECIFIED.,.F.,.F.,(4,1,1,1,1,1,1,1,1,1,1,1,1,
1,1,1,4),(0.,0.0625,0.09375,0.125,0.15625,0.1875,0.25,0.375,0.5,0.625,0.6875,
0.71875,0.75,0.78125,0.8125,0.875,1.),.UNSPECIFIED.);
#485=B_SPLINE_CURVE_WITH_KNOTS('',3,(#28762,#28763,#28764,#28765,#28766,
#28767,#28768,#28769,#28770),.UNSPECIFIED.,.F.,.F.,(4,1,1,1,1,1,4),(4.65545680163139E-9,
0.125,0.1875,0.21875,0.25,0.28125,0.298831604432797),.UNSPECIFIED.);
#486=B_SPLINE_CURVE_WITH_KNOTS('',1,(#28772,#28773),.UNSPECIFIED.,.F.,.F.,
(2,2),(-0.24818047819294,-0.234857897987038),.UNSPECIFIED.);
#487=B_SPLINE_CURVE_WITH_KNOTS('',3,(#28775,#28776,#28777,#28778,#28779,
#28780,#28781,#28782,#28783,#28784,#28785,#28786,#28787,#28788,#28789,#28790,
#28791,#28792,#28793),.UNSPECIFIED.,.F.,.F.,(4,3,3,3,3,3,4),(0.701590233395244,
0.71875,0.75,0.78125,0.8125,0.875,0.99999997963134),.UNSPECIFIED.);
#488=B_SPLINE_CURVE_WITH_KNOTS('',3,(#28795,#28796,#28797,#28798,#28799,
#28800,#28801,#28802,#28803,#28804,#28805,#28806,#28807,#28808,#28809,#28810,
#28811,#28812,#28813,#28814,#28815,#28816,#28817,#28818,#28819,#28820,#28821,
#28822,#28823,#28824,#28825,#28826,#28827,#28828,#28829,#28830,#28831,#28832,
#28833,#28834,#28835,#28836,#28837,#28838,#28839,#28840,#28841,#28842,#28843,
#28844,#28845,#28846),.UNSPECIFIED.,.F.,.F.,(4,3,3,3,3,3,3,3,3,3,3,3,3,
3,3,3,3,4),(0.,0.125,0.1875,0.21875,0.25,0.28125,0.3125,0.375,0.5,0.625,
0.633652818087256,0.75,0.8125,0.84375,0.875,0.90625,0.9375,0.99999982127163),
 .UNSPECIFIED.);
#489=B_SPLINE_CURVE_WITH_KNOTS('',3,(#28850,#28851,#28852,#28853,#28854,
#28855,#28856,#28857,#28858,#28859,#28860,#28861,#28862,#28863,#28864,#28865,
#28866,#28867,#28868),.UNSPECIFIED.,.F.,.F.,(4,1,1,1,1,1,1,1,1,1,1,1,1,
1,1,1,4),(2.60020861133173E-7,0.0625,0.09375,0.125,0.15625,0.1875,0.25,
0.375,0.5,0.625,0.6875,0.71875,0.75,0.78125,0.8125,0.875,0.999999902697824),
 .UNSPECIFIED.);
#490=B_SPLINE_CURVE_WITH_KNOTS('',3,(#28870,#28871,#28872,#28873,#28874,
#28875,#28876,#28877,#28878),.UNSPECIFIED.,.F.,.F.,(4,1,1,1,1,1,4),(0.,
0.125,0.1875,0.21875,0.25,0.28125,0.298021461655708),.UNSPECIFIED.);
#491=B_SPLINE_CURVE_WITH_KNOTS('',1,(#28880,#28881),.UNSPECIFIED.,.F.,.F.,
(2,2),(-0.214862684454297,-0.201578551331348),.UNSPECIFIED.);
#492=B_SPLINE_CURVE_WITH_KNOTS('',3,(#28883,#28884,#28885,#28886,#28887,
#28888,#28889,#28890,#28891,#28892,#28893,#28894,#28895,#28896,#28897,#28898,
#28899,#28900,#28901),.UNSPECIFIED.,.F.,.F.,(4,3,3,3,3,3,4),(0.0574863041974119,
0.125,0.1875,0.21875,0.25,0.28125,0.293194800091934),.UNSPECIFIED.);
#493=B_SPLINE_CURVE_WITH_KNOTS('',3,(#28903,#28904,#28905,#28906),
 .UNSPECIFIED.,.F.,.F.,(4,4),(6.86640626528075E-6,0.0574863041974119),
 .UNSPECIFIED.);
#494=B_SPLINE_CURVE_WITH_KNOTS('',3,(#28908,#28909,#28910,#28911,#28912,
#28913,#28914,#28915,#28916,#28917,#28918,#28919,#28920,#28921,#28922,#28923,
#28924,#28925,#28926,#28927,#28928,#28929,#28930,#28931,#28932,#28933,#28934,
#28935,#28936,#28937,#28938,#28939,#28940,#28941,#28942,#28943,#28944,#28945,
#28946,#28947,#28948,#28949,#28950,#28951,#28952,#28953,#28954,#28955,#28956,
#28957,#28958,#28959),.UNSPECIFIED.,.F.,.F.,(4,3,3,3,3,3,3,3,3,3,3,3,3,
3,3,3,3,4),(0.,0.125,0.1875,0.21875,0.25,0.28125,0.3125,0.375,0.5,0.625,
0.66804399378711,0.75,0.8125,0.84375,0.875,0.90625,0.9375,0.999999677104164),
 .UNSPECIFIED.);
#495=B_SPLINE_CURVE_WITH_KNOTS('',3,(#28961,#28962,#28963,#28964,#28965,
#28966,#28967,#28968,#28969),.UNSPECIFIED.,.F.,.F.,(4,1,1,1,1,1,4),(0.,
0.125,0.1875,0.25,0.3125,0.375,0.499188038144574),.UNSPECIFIED.);
#496=B_SPLINE_CURVE_WITH_KNOTS('',3,(#28971,#28972,#28973,#28974,#28975,
#28976,#28977,#28978,#28979),.UNSPECIFIED.,.F.,.F.,(4,1,1,1,1,1,4),(0.499188038144574,
0.5,0.625,0.75,0.875,0.9375,0.998196008235996),.UNSPECIFIED.);
#497=B_SPLINE_CURVE_WITH_KNOTS('',3,(#28981,#28982,#28983,#28984,#28985,
#28986,#28987,#28988,#28989,#28990,#28991,#28992,#28993,#28994,#28995,#28996,
#28997,#28998,#28999,#29000,#29001,#29002,#29003,#29004,#29005,#29006,#29007,
#29008,#29009,#29010,#29011,#29012,#29013,#29014,#29015,#29016,#29017,#29018,
#29019,#29020,#29021,#29022,#29023,#29024,#29025,#29026,#29027,#29028,#29029),
 .UNSPECIFIED.,.F.,.F.,(4,3,3,3,3,3,3,3,3,3,3,3,3,3,3,3,4),(0.,0.125,0.1875,
0.21875,0.25,0.28125,0.3125,0.375,0.4375,0.5,0.5625,0.625,0.6875,0.75,0.809462341510482,
0.875,1.),.UNSPECIFIED.);
#498=B_SPLINE_CURVE_WITH_KNOTS('',3,(#29031,#29032,#29033,#29034,#29035,
#29036,#29037,#29038,#29039,#29040,#29041,#29042,#29043,#29044,#29045,#29046,
#29047,#29048,#29049,#29050,#29051,#29052),.UNSPECIFIED.,.F.,.F.,(4,3,3,
3,3,3,3,4),(0.626108993264048,0.6875,0.71875,0.75,0.78125,0.8125,0.875,
0.999993195039302),.UNSPECIFIED.);
#499=B_SPLINE_CURVE_WITH_KNOTS('',1,(#29054,#29055),.UNSPECIFIED.,.F.,.F.,
(2,2),(-0.181505671215862,-0.1040158100396),.UNSPECIFIED.);
#500=B_SPLINE_CURVE_WITH_KNOTS('',3,(#29057,#29058,#29059,#29060),
 .UNSPECIFIED.,.F.,.F.,(4,4),(0.915239918615735,1.),.UNSPECIFIED.);
#501=B_SPLINE_CURVE_WITH_KNOTS('',3,(#29062,#29063,#29064,#29065),
 .UNSPECIFIED.,.F.,.F.,(4,4),(0.75,1.),.UNSPECIFIED.);
#502=B_SPLINE_CURVE_WITH_KNOTS('',3,(#29067,#29068,#29069,#29070,#29071,
#29072,#29073,#29074,#29075,#29076,#29077,#29078,#29079),.UNSPECIFIED.,
 .F.,.F.,(4,3,3,3,4),(6.7281280280231E-5,0.25,0.375,0.5,0.75),
 .UNSPECIFIED.);
#503=B_SPLINE_CURVE_WITH_KNOTS('',3,(#29081,#29082,#29083,#29084),
 .UNSPECIFIED.,.F.,.F.,(4,4),(0.380644930253737,0.999995028027359),
 .UNSPECIFIED.);
#504=B_SPLINE_CURVE_WITH_KNOTS('',3,(#29086,#29087,#29088,#29089),
 .UNSPECIFIED.,.F.,.F.,(4,4),(0.,0.380644930253737),.UNSPECIFIED.);
#505=B_SPLINE_CURVE_WITH_KNOTS('',3,(#29091,#29092,#29093,#29094,#29095,
#29096,#29097,#29098,#29099,#29100,#29101,#29102,#29103,#29104,#29105,#29106,
#29107),.UNSPECIFIED.,.F.,.F.,(4,1,1,1,1,1,1,1,1,1,1,1,1,1,4),(0.,0.125,
0.1875,0.25,0.3125,0.375,0.4375,0.5,0.625,0.6875,0.75,0.8125,0.875,0.9375,
0.999999571178552),.UNSPECIFIED.);
#506=B_SPLINE_CURVE_WITH_KNOTS('',3,(#29109,#29110,#29111,#29112),
 .UNSPECIFIED.,.F.,.F.,(4,4),(0.,1.),.UNSPECIFIED.);
#507=B_SPLINE_CURVE_WITH_KNOTS('',3,(#29113,#29114,#29115,#29116,#29117,
#29118,#29119,#29120,#29121,#29122,#29123,#29124,#29125,#29126,#29127,#29128),
 .UNSPECIFIED.,.F.,.F.,(4,3,3,3,3,4),(0.,0.0575860235571798,0.125,0.25,
0.3125,0.364118167489102),.UNSPECIFIED.);
#508=B_SPLINE_CURVE_WITH_KNOTS('',3,(#29271,#29272,#29273,#29274),
 .UNSPECIFIED.,.F.,.F.,(4,4),(-0.801761649289337,-0.764530975504951),
 .UNSPECIFIED.);
#509=B_SPLINE_CURVE_WITH_KNOTS('',3,(#29276,#29277,#29278,#29279,#29280,
#29281,#29282,#29283,#29284,#29285,#29286,#29287,#29288,#29289,#29290,#29291,
#29292,#29293,#29294,#29295,#29296,#29297,#29298,#29299,#29300,#29301,#29302,
#29303,#29304,#29305,#29306,#29307,#29308,#29309,#29310,#29311,#29312,#29313,
#29314,#29315,#29316,#29317,#29318,#29319,#29320,#29321,#29322,#29323,#29324,
#29325,#29326,#29327,#29328,#29329,#29330),.UNSPECIFIED.,.F.,.F.,(4,3,3,
3,3,3,3,3,3,3,3,3,3,3,3,3,3,3,4),(3.7275728618467E-8,0.00213268712132415,
0.00241015582328363,0.00361523373492544,0.00482031164656725,0.00602538955820906,
0.00666926365661724,0.00723046746985087,0.00843554538149267,0.00883404960601883,
0.00964062329313448,0.0108457012047763,0.0115672277245366,0.0120507791164181,
0.0143099259775042,0.0144609349397017,0.0155427936599299,0.0156660128513435,
0.0167172049195214),.UNSPECIFIED.);
#510=B_SPLINE_CURVE_WITH_KNOTS('',3,(#29332,#29333,#29334,#29335,#29336,
#29337,#29338,#29339,#29340,#29341,#29342,#29343,#29344,#29345,#29346,#29347,
#29348,#29349),.UNSPECIFIED.,.F.,.F.,(4,2,2,2,2,2,2,2,4),(0.,0.125,0.25,
0.375,0.5,0.625,0.75,0.875,1.),.UNSPECIFIED.);
#511=B_SPLINE_CURVE_WITH_KNOTS('',3,(#29351,#29352,#29353,#29354,#29355,
#29356,#29357,#29358,#29359,#29360,#29361,#29362,#29363,#29364,#29365,#29366,
#29367,#29368,#29369,#29370,#29371,#29372,#29373,#29374,#29375,#29376,#29377,
#29378,#29379,#29380,#29381,#29382,#29383,#29384,#29385,#29386,#29387,#29388,
#29389,#29390,#29391,#29392,#29393,#29394,#29395,#29396,#29397,#29398,#29399,
#29400,#29401,#29402,#29403,#29404,#29405,#29406,#29407,#29408,#29409,#29410,
#29411,#29412,#29413,#29414,#29415,#29416,#29417,#29418,#29419,#29420),
 .UNSPECIFIED.,.F.,.F.,(4,3,3,3,3,3,3,3,3,3,3,3,3,3,3,3,3,3,3,3,3,3,3,4),
(1.08058869667645E-7,0.000426646628827551,0.00122648046975059,0.00145211381056247,
0.0024529609387835,0.00255429073838069,0.00367944140781642,0.00374167552846414,
0.00490592187684933,0.0050104433434355,0.00735888281491516,0.0079238714718458,
0.00858536328394808,0.00981184375298099,0.010715819001823,0.0110383242220139,
0.0122648046910468,0.0128618444900144,0.0134912851600797,0.0147177656291127,
0.0159442460981456,0.0171707265671785,0.0174912668652558,0.0196236713267414),
 .UNSPECIFIED.);
#512=B_SPLINE_CURVE_WITH_KNOTS('',3,(#29422,#29423,#29424,#29425,#29426,
#29427,#29428,#29429,#29430,#29431,#29432,#29433,#29434,#29435,#29436,#29437,
#29438,#29439,#29440,#29441,#29442,#29443,#29444,#29445,#29446,#29447,#29448,
#29449,#29450,#29451,#29452,#29453,#29454,#29455,#29456,#29457,#29458,#29459,
#29460,#29461),.UNSPECIFIED.,.F.,.F.,(4,3,3,3,3,3,3,3,3,3,3,3,3,4),(0.0138309084487971,
0.0141209324226746,0.0144279092144626,0.0147348860062506,0.0147783505908347,
0.0153488395898266,0.0158093047775086,0.0158956420001989,0.0159765831464712,
0.0160205263564273,0.0171907003405545,0.0172599467341181,0.0178046539241305,
0.019646491834798),.UNSPECIFIED.);
#513=B_SPLINE_CURVE_WITH_KNOTS('',3,(#29463,#29464,#29465,#29466),
 .UNSPECIFIED.,.F.,.F.,(4,4),(-0.900360708476172,-0.86499516359624),
 .UNSPECIFIED.);
#514=B_SPLINE_CURVE_WITH_KNOTS('',3,(#29468,#29469,#29470,#29471,#29472,
#29473,#29474),.UNSPECIFIED.,.F.,.F.,(4,1,1,1,4),(3.72393009463586E-10,
0.00112032596633615,0.00224065181164156,0.00336097765694698,0.00404745390640756),
 .UNSPECIFIED.);
#515=B_SPLINE_CURVE_WITH_KNOTS('',3,(#29476,#29477,#29478,#29479,#29480,
#29481,#29482,#29483,#29484,#29485,#29486,#29487,#29488,#29489,#29490,#29491,
#29492,#29493,#29494,#29495,#29496,#29497,#29498,#29499,#29500,#29501,#29502,
#29503,#29504,#29505,#29506,#29507,#29508,#29509),.UNSPECIFIED.,.F.,.F.,
(4,3,3,3,3,3,3,3,3,3,3,4),(1.56135529065312E-9,0.000149014693064497,0.000707813936974023,
0.00112691336990617,0.00118870219951449,0.00128407565725572,0.0023842116687026,
0.00241586779852081,0.00298026419553942,0.00357631672237625,0.00364795327462914,
0.00380005432105398),.UNSPECIFIED.);
#516=B_SPLINE_CURVE_WITH_KNOTS('',3,(#29511,#29512,#29513,#29514),
 .UNSPECIFIED.,.F.,.F.,(4,4),(-0.788485824448602,-0.75173722881735),
 .UNSPECIFIED.);
#517=B_SPLINE_CURVE_WITH_KNOTS('',3,(#29516,#29517,#29518,#29519,#29520,
#29521,#29522,#29523,#29524,#29525),.UNSPECIFIED.,.F.,.F.,(4,3,3,4),(3.52393154467455E-8,
0.00220719129062706,0.00226386756700581,0.00462327622956672),
 .UNSPECIFIED.);
#518=B_SPLINE_CURVE_WITH_KNOTS('',3,(#29527,#29528,#29529,#29530,#29531,
#29532,#29533,#29534,#29535,#29536),.UNSPECIFIED.,.F.,.F.,(4,3,3,4),(7.932060984575E-15,
0.00157881831260296,0.00235387237808879,0.00470771557316006),
 .UNSPECIFIED.);
#519=B_SPLINE_CURVE_WITH_KNOTS('',3,(#29538,#29539,#29540,#29541,#29542,
#29543,#29544,#29545),.UNSPECIFIED.,.F.,.F.,(4,2,2,4),(7.02291898378891E-6,
0.0451293601147105,0.0692682469770136,0.0896084138988641),.UNSPECIFIED.);
#520=B_SPLINE_CURVE_WITH_KNOTS('',3,(#29547,#29548,#29549,#29550,#29551,
#29552),.UNSPECIFIED.,.F.,.F.,(4,2,4),(0.00040201242378087,0.0139583175638981,
0.0275208583776574),.UNSPECIFIED.);
#521=B_SPLINE_CURVE_WITH_KNOTS('',3,(#29554,#29555,#29556,#29557,#29558,
#29559),.UNSPECIFIED.,.F.,.F.,(4,2,4),(6.53624102621552E-6,0.0289149570250049,
0.0574752936489782),.UNSPECIFIED.);
#522=B_SPLINE_CURVE_WITH_KNOTS('',3,(#29561,#29562,#29563,#29564,#29565,
#29566),.UNSPECIFIED.,.F.,.F.,(4,2,4),(-0.100164676307967,-0.0501603860011391,
-0.000310269947608522),.UNSPECIFIED.);
#523=B_SPLINE_CURVE_WITH_KNOTS('',3,(#29568,#29569,#29570,#29571,#29572,
#29573),.UNSPECIFIED.,.F.,.F.,(4,2,4),(0.000156968191344601,0.0294034008226515,
0.0586209359117642),.UNSPECIFIED.);
#524=B_SPLINE_CURVE_WITH_KNOTS('',3,(#29575,#29576,#29577,#29578,#29579,
#29580),.UNSPECIFIED.,.F.,.F.,(4,2,4),(5.32014841871761E-5,0.0390048636397492,
0.0777949467112503),.UNSPECIFIED.);
#525=B_SPLINE_CURVE_WITH_KNOTS('',3,(#29582,#29583,#29584,#29585,#29586,
#29587,#29588,#29589,#29590,#29591,#29592,#29593,#29594),.UNSPECIFIED.,
 .F.,.F.,(4,3,3,3,4),(8.67361737988404E-19,7.42016414987991E-5,0.00236271426147704,
0.00354407139221556,0.00472542852295408),.UNSPECIFIED.);
#526=B_SPLINE_CURVE_WITH_KNOTS('',3,(#29596,#29597,#29598,#29599,#29600,
#29601,#29602,#29603,#29604,#29605,#29606,#29607,#29608,#29609,#29610,#29611,
#29612,#29613,#29614,#29615,#29616,#29617,#29618,#29619,#29620,#29621,#29622,
#29623,#29624,#29625,#29626,#29627,#29628,#29629,#29630,#29631,#29632,#29633,
#29634,#29635,#29636,#29637,#29638,#29639,#29640,#29641,#29642,#29643,#29644,
#29645,#29646,#29647,#29648,#29649,#29650,#29651,#29652,#29653,#29654,#29655,
#29656,#29657,#29658,#29659,#29660,#29661,#29662,#29663,#29664,#29665,#29666,
#29667,#29668),.UNSPECIFIED.,.F.,.F.,(4,3,3,3,3,3,3,3,3,3,3,3,3,3,3,3,3,
3,3,3,3,3,3,3,4),(0.,7.75161947677991E-5,0.00111757680617575,0.00223515361235151,
0.00335273041852726,0.00391151882161514,0.00447030722470301,0.00499947827886225,
0.00502909562779089,0.00558788403087876,0.00670546083705452,0.00745503820642138,
0.00782303764323027,0.00894061444940602,0.0104502859150961,0.0111757680617575,
0.0130679753464858,0.013410921674109,0.0142514928999412,0.0145284984802848,
0.0153723205684816,0.0156460752864605,0.0164339145851788,0.0174532669379536,
0.017881228898812),.UNSPECIFIED.);
#527=B_SPLINE_CURVE_WITH_KNOTS('',3,(#29670,#29671,#29672,#29673,#29674,
#29675,#29676,#29677,#29678,#29679,#29680,#29681,#29682,#29683,#29684,#29685,
#29686,#29687,#29688,#29689,#29690,#29691,#29692,#29693,#29694,#29695,#29696,
#29697,#29698,#29699,#29700,#29701,#29702,#29703,#29704,#29705,#29706,#29707,
#29708,#29709,#29710,#29711,#29712,#29713,#29714,#29715,#29716,#29717,#29718,
#29719,#29720,#29721,#29722,#29723,#29724,#29725,#29726,#29727,#29728,#29729,
#29730,#29731,#29732,#29733),.UNSPECIFIED.,.F.,.F.,(4,3,3,3,3,3,3,3,3,3,
3,3,3,3,3,3,3,3,3,3,3,4),(0.,0.00158828845524716,0.0021893200599713,0.00264594734442174,
0.00328398008995695,0.00375597387774578,0.0043786401199426,0.00615520482571866,
0.0065679601799139,0.0087572802398852,0.0088668805883462,0.00985194026987085,
0.0109466002998565,0.011634371002562,0.0120412603298422,0.012588590344835,
0.0131359203598278,0.0142305803898135,0.0153252404197991,0.016220768789973,
0.0164199004497848,0.0175145604797704),.UNSPECIFIED.);
#528=B_SPLINE_CURVE_WITH_KNOTS('',3,(#29735,#29736,#29737,#29738,#29739,
#29740,#29741,#29742,#29743,#29744,#29745,#29746,#29747,#29748,#29749,#29750,
#29751,#29752,#29753,#29754,#29755,#29756,#29757,#29758,#29759,#29760,#29761,
#29762,#29763,#29764,#29765,#29766,#29767,#29768,#29769,#29770,#29771),
 .UNSPECIFIED.,.F.,.F.,(4,3,3,3,3,3,3,3,3,3,3,3,4),(0.,0.000297867429863575,
0.000744668574658938,0.000968069147056619,0.00110064938673372,0.0011914697194543,
0.00178720457918146,0.00193613829411324,0.00234224251489775,0.00238293943890861,
0.00297867429863576,0.00359302587272938,0.00476587887781721),
 .UNSPECIFIED.);
#529=B_SPLINE_CURVE_WITH_KNOTS('',3,(#29773,#29774,#29775,#29776,#29777,
#29778),.UNSPECIFIED.,.F.,.F.,(4,2,4),(0.000112668959181985,0.0394878781786619,
0.0787740170229608),.UNSPECIFIED.);
#530=B_SPLINE_CURVE_WITH_KNOTS('',3,(#29782,#29783,#29784,#29785,#29786,
#29787),.UNSPECIFIED.,.F.,.F.,(4,2,4),(4.69002654761246E-6,0.050001342311006,
0.0999913387878795),.UNSPECIFIED.);
#531=B_SPLINE_CURVE_WITH_KNOTS('',3,(#29791,#29792,#29793,#29794,#29795,
#29796),.UNSPECIFIED.,.F.,.F.,(4,2,4),(0.000695999025172847,0.013935683082129,
0.0269158957041709),.UNSPECIFIED.);
#532=B_SPLINE_CURVE_WITH_KNOTS('',3,(#29798,#29799,#29800,#29801,#29802,
#29803,#29804,#29805),.UNSPECIFIED.,.F.,.F.,(4,2,2,4),(4.60554727665049E-5,
0.0201218316749581,0.0440109401186668,0.0887346835144923),.UNSPECIFIED.);
#533=B_SPLINE_CURVE_WITH_KNOTS('',3,(#29807,#29808,#29809,#29810,#29811,
#29812,#29813),.UNSPECIFIED.,.F.,.F.,(4,3,4),(3.18003771205116E-15,0.0023582377455569,
0.00470691707255086),.UNSPECIFIED.);
#534=B_SPLINE_CURVE_WITH_KNOTS('',3,(#29815,#29816,#29817,#29818,#29819,
#29820,#29821,#29822,#29823,#29824),.UNSPECIFIED.,.F.,.F.,(4,3,3,4),(3.44289573972157E-8,
0.00232495486867497,0.00307076742172914,0.00464990715460391),
 .UNSPECIFIED.);
#535=B_SPLINE_CURVE_WITH_KNOTS('',3,(#29826,#29827,#29828,#29829,#29830,
#29831,#29832,#29833),.UNSPECIFIED.,.F.,.F.,(4,2,2,4),(6.42183317534942E-6,
0.04781967269061,0.0732367945616579,0.0950553531959799),.UNSPECIFIED.);
#536=B_SPLINE_CURVE_WITH_KNOTS('',3,(#29835,#29836,#29837,#29838,#29839,
#29840),.UNSPECIFIED.,.F.,.F.,(4,2,4),(0.000374884371361637,0.0150232472508783,
0.0297168549388432),.UNSPECIFIED.);
#537=B_SPLINE_CURVE_WITH_KNOTS('',3,(#29842,#29843,#29844,#29845,#29846,
#29847),.UNSPECIFIED.,.F.,.F.,(4,2,4),(6.13317120454564E-6,0.0290789797557169,
0.0578659870050568),.UNSPECIFIED.);
#538=B_SPLINE_CURVE_WITH_KNOTS('',3,(#29849,#29850,#29851,#29852,#29853,
#29854),.UNSPECIFIED.,.F.,.F.,(4,2,4),(1.00018224971625E-5,0.0500087821938493,
0.10001293618161),.UNSPECIFIED.);
#539=B_SPLINE_CURVE_WITH_KNOTS('',3,(#29856,#29857,#29858,#29859,#29860,
#29861),.UNSPECIFIED.,.F.,.F.,(4,2,4),(7.53330920655929E-6,0.0293896381172448,
0.0587097736963051),.UNSPECIFIED.);
#540=B_SPLINE_CURVE_WITH_KNOTS('',3,(#29863,#29864,#29865,#29866,#29867,
#29868),.UNSPECIFIED.,.F.,.F.,(4,2,4),(8.20230271009787E-5,0.0377809065926269,
0.0755399468969054),.UNSPECIFIED.);
#541=B_SPLINE_CURVE_WITH_KNOTS('',3,(#29870,#29871,#29872,#29873,#29874,
#29875),.UNSPECIFIED.,.F.,.F.,(4,1,1,4),(0.,0.00119697920627212,0.00239395841254424,
0.00478791682508848),.UNSPECIFIED.);
#542=B_SPLINE_CURVE_WITH_KNOTS('',3,(#29876,#29877,#29878,#29879,#29880,
#29881,#29882,#29883,#29884,#29885,#29886,#29887,#29888,#29889,#29890,#29891),
 .UNSPECIFIED.,.F.,.F.,(4,1,1,1,1,1,1,1,1,1,1,1,1,4),(0.00248265578786311,
0.00329931417081839,0.00439908556096978,0.00659862834127257,0.00879817112157535,
0.00989794251172675,0.0109977139018781,0.0120974852920295,0.0126473709871052,
0.0131972566821809,0.0142970280723323,0.0153967994624837,0.0164965708526351,
0.0175963422427865),.UNSPECIFIED.);
#543=B_SPLINE_CURVE_WITH_KNOTS('',3,(#29894,#29895,#29896,#29897,#29898,
#29899),.UNSPECIFIED.,.F.,.F.,(4,2,4),(-0.351103621180421,-0.184658836618039,
-0.000144336259837594),.UNSPECIFIED.);
#544=B_SPLINE_CURVE_WITH_KNOTS('',3,(#29901,#29902,#29903,#29904,#29905,
#29906,#29907,#29908),.UNSPECIFIED.,.F.,.F.,(4,2,2,4),(0.00013573500535706,
0.152913187988002,0.221936523531357,0.281794792544631),.UNSPECIFIED.);
#545=B_SPLINE_CURVE_WITH_KNOTS('',3,(#29910,#29911,#29912,#29913,#29914,
#29915,#29916,#29917),.UNSPECIFIED.,.F.,.F.,(4,2,2,4),(8.16139213976878E-5,
0.0601010912620195,0.129621118816494,0.284198839020368),.UNSPECIFIED.);
#546=B_SPLINE_CURVE_WITH_KNOTS('',3,(#29918,#29919,#29920,#29921,#29922,
#29923,#29924,#29925,#29926,#29927,#29928,#29929,#29930,#29931,#29932,#29933,
#29934,#29935,#29936,#29937,#29938,#29939,#29940,#29941,#29942,#29943,#29944,
#29945,#29946,#29947,#29948,#29949,#29950,#29951,#29952,#29953,#29954,#29955,
#29956,#29957,#29958,#29959,#29960,#29961,#29962,#29963,#29964,#29965,#29966,
#29967,#29968,#29969,#29970,#29971,#29972,#29973,#29974,#29975,#29976,#29977,
#29978,#29979,#29980,#29981,#29982,#29983,#29984),.UNSPECIFIED.,.F.,.F.,
(4,3,3,3,3,3,3,3,3,3,3,3,3,3,3,3,3,3,3,3,3,3,4),(0.,0.000109920237579343,
0.00061591770973852,0.000934322019424417,0.000985847130789734,0.00103415192269472,
0.00119683823187687,0.00172622571154797,0.00175872380126949,0.0019699967952482,
0.00219840475158686,0.00236328510795588,0.00243542026386732,0.0025030469725343,
0.00272120378944146,0.00286687736586743,0.00301024728753664,0.00304119051135285,
0.00326384744503781,0.00339064752378839,0.00345404756316369,0.00348574758285133,
0.00351744760253898),.UNSPECIFIED.);
#547=B_SPLINE_CURVE_WITH_KNOTS('',3,(#29987,#29988,#29989,#29990,#29991,
#29992,#29993,#29994),.UNSPECIFIED.,.F.,.F.,(4,2,2,4),(0.,0.0594485370103995,
0.128200922849087,0.28027816230381),.UNSPECIFIED.);
#548=B_SPLINE_CURVE_WITH_KNOTS('',3,(#29996,#29997,#29998,#29999,#30000,
#30001),.UNSPECIFIED.,.F.,.F.,(4,2,4),(-0.353460855213146,-0.168401493160792,
0.),.UNSPECIFIED.);
#549=B_SPLINE_CURVE_WITH_KNOTS('',3,(#30003,#30004,#30005,#30006,#30007,
#30008),.UNSPECIFIED.,.F.,.F.,(4,2,4),(-0.35246001194512,-0.169875343850794,
-8.95159592229078E-7),.UNSPECIFIED.);
#550=B_SPLINE_CURVE_WITH_KNOTS('',3,(#30009,#30010,#30011,#30012,#30013,
#30014,#30015,#30016),.UNSPECIFIED.,.F.,.F.,(4,2,2,4),(0.000136900112796742,
0.156887006623476,0.227547774409115,0.288714197538024),.UNSPECIFIED.);
#551=B_SPLINE_CURVE_WITH_KNOTS('',3,(#30158,#30159,#30160,#30161,#30162),
 .UNSPECIFIED.,.F.,.F.,(4,1,4),(3.64204572566108E-13,0.00219954278066699,
0.00248265578786311),.UNSPECIFIED.);
#552=B_SPLINE_CURVE_WITH_KNOTS('',3,(#30163,#30164,#30165,#30166,#30167,
#30168,#30169,#30170,#30171,#30172,#30173,#30174,#30175,#30176),
 .UNSPECIFIED.,.F.,.F.,(4,1,1,1,1,1,1,1,1,1,1,4),(0.00404745390640756,0.00448130350225239,
0.0050414664249051,0.00560162934755781,0.00672195519286322,0.00784228103816864,
0.00896260688347405,0.0112032585740849,0.0134439102646957,0.0145642361100011,
0.0156845619553065,0.0179252136459174),.UNSPECIFIED.);
#553=B_SPLINE_CURVE_WITH_KNOTS('',3,(#30178,#30179,#30180,#30181,#30182,
#30183,#30184,#30185,#30186,#30187,#30188,#30189,#30190,#30191,#30192,#30193,
#30194,#30195,#30196,#30197,#30198,#30199,#30200,#30201,#30202,#30203,#30204,
#30205,#30206,#30207,#30208,#30209,#30210,#30211,#30212,#30213,#30214,#30215,
#30216,#30217,#30218,#30219,#30220,#30221,#30222,#30223,#30224,#30225,#30226,
#30227,#30228,#30229,#30230,#30231,#30232,#30233,#30234,#30235,#30236,#30237,
#30238,#30239,#30240,#30241,#30242,#30243,#30244,#30245,#30246,#30247,#30248,
#30249,#30250,#30251,#30252,#30253,#30254,#30255,#30256,#30257,#30258,#30259,
#30260,#30261,#30262,#30263,#30264,#30265,#30266,#30267,#30268,#30269,#30270,
#30271,#30272,#30273,#30274,#30275,#30276,#30277,#30278,#30279,#30280,#30281,
#30282,#30283,#30284,#30285,#30286),.UNSPECIFIED.,.F.,.F.,(4,3,3,3,3,3,
3,3,3,3,3,3,3,3,3,3,3,3,3,3,3,3,3,3,3,3,3,3,3,3,3,3,3,3,3,3,4),(4.26881478763691E-13,
0.000306976792214876,0.00112686428044965,0.00122790716757886,0.00138139556347286,
0.00191860494910184,0.00218720964191634,0.00238136727005047,0.00245581433473083,
0.0036439705098947,0.0036837215018828,0.00429767508545879,0.00489317856768551,
0.00491162866903478,0.00613953583618676,0.00675348941976274,0.00736744300333873,
0.00739256586998839,0.00798139658691471,0.0085953501704907,0.00863787380293649,
0.00920930375406668,0.00982325733764267,0.00986608700714022,0.0104372109212186,
0.0110511645047946,0.0110965072788747,0.0113581412965826,0.0118186064842646,
0.0122790716719466,0.0123256390264983,0.0128930252555226,0.0132000020473106,
0.0133534904432046,0.0135069788390986,0.0135490258016012,0.0138309084487971),
 .UNSPECIFIED.);
#554=B_SPLINE_CURVE_WITH_KNOTS('',3,(#30287,#30288,#30289,#30290,#30291,
#30292,#30293,#30294,#30295,#30296,#30297,#30298,#30299,#30300,#30301,#30302),
 .UNSPECIFIED.,.F.,.F.,(4,3,3,3,3,4),(0.0167172049195214,0.0168710907629853,
0.0178203760382903,0.0180761686746271,0.0188523687683586,0.019281246586269),
 .UNSPECIFIED.);
#555=B_SPLINE_CURVE_WITH_KNOTS('',3,(#30306,#30307,#30308,#30309,#30310,
#30311),.UNSPECIFIED.,.F.,.F.,(4,2,4),(-1.66978451121418,-1.49281136073648,
-1.33992830231631),.UNSPECIFIED.);
#556=B_SPLINE_CURVE_WITH_KNOTS('',3,(#30313,#30314,#30315,#30316,#30317,
#30318,#30319,#30320,#30321,#30322,#30323,#30324),.UNSPECIFIED.,.F.,.F.,
(4,1,1,1,1,1,1,1,1,4),(0.,0.25,0.375,0.5,0.625,0.6875,0.75,0.8125,0.875,
1.),.UNSPECIFIED.);
#557=B_SPLINE_CURVE_WITH_KNOTS('',3,(#30326,#30327,#30328,#30329),
 .UNSPECIFIED.,.F.,.F.,(4,4),(2.50930273678697,2.78682786773594),
 .UNSPECIFIED.);
#558=B_SPLINE_CURVE_WITH_KNOTS('',3,(#30330,#30331,#30332,#30333,#30334,
#30335),.UNSPECIFIED.,.F.,.F.,(4,2,4),(2.77504169139609,2.7756154298488,
3.04976295261124),.UNSPECIFIED.);
#559=B_SPLINE_CURVE_WITH_KNOTS('',3,(#30397,#30398,#30399,#30400,#30401,
#30402,#30403,#30404,#30405,#30406,#30407,#30408,#30409,#30410,#30411,#30412,
#30413,#30414,#30415,#30416,#30417,#30418,#30419,#30420,#30421,#30422,#30423,
#30424,#30425,#30426,#30427,#30428,#30429,#30430),.UNSPECIFIED.,.F.,.F.,
(4,3,3,3,3,3,3,3,3,3,3,4),(0.364118167489102,0.375,0.434093352847254,0.5,
0.56610957647016,0.625,0.635973158026349,0.6875,0.75,0.875,0.942536907276119,
1.),.UNSPECIFIED.);
#560=B_SPLINE_CURVE_WITH_KNOTS('',3,(#30432,#30433,#30434,#30435),
 .UNSPECIFIED.,.F.,.F.,(4,4),(0.,1.),.UNSPECIFIED.);
#561=B_SPLINE_CURVE_WITH_KNOTS('',3,(#30437,#30438,#30439,#30440,#30441,
#30442,#30443,#30444,#30445,#30446,#30447,#30448,#30449,#30450,#30451,#30452,
#30453),.UNSPECIFIED.,.F.,.F.,(4,1,1,1,1,1,1,1,1,1,1,1,1,1,4),(3.19570811666715E-7,
0.0625,0.125,0.1875,0.25,0.3125,0.375,0.5,0.5625,0.625,0.6875,0.75,0.8125,
0.875,1.),.UNSPECIFIED.);
#562=B_SPLINE_CURVE_WITH_KNOTS('',3,(#30455,#30456,#30457,#30458),
 .UNSPECIFIED.,.F.,.F.,(4,4),(0.75,1.),.UNSPECIFIED.);
#563=B_SPLINE_CURVE_WITH_KNOTS('',3,(#30460,#30461,#30462,#30463,#30464,
#30465,#30466,#30467,#30468,#30469,#30470,#30471,#30472),.UNSPECIFIED.,
 .F.,.F.,(4,3,3,3,4),(6.9291577602274E-5,0.25,0.375,0.5,0.75),
 .UNSPECIFIED.);
#564=B_SPLINE_CURVE_WITH_KNOTS('',3,(#30474,#30475,#30476,#30477),
 .UNSPECIFIED.,.F.,.F.,(4,4),(0.380639039903466,0.999995038571591),
 .UNSPECIFIED.);
#565=B_SPLINE_CURVE_WITH_KNOTS('',3,(#30479,#30480,#30481,#30482),
 .UNSPECIFIED.,.F.,.F.,(4,4),(0.,0.380639039903466),.UNSPECIFIED.);
#566=B_SPLINE_CURVE_WITH_KNOTS('',3,(#30484,#30485,#30486,#30487,#30488,
#30489,#30490,#30491,#30492,#30493,#30494,#30495,#30496,#30497,#30498,#30499,
#30500),.UNSPECIFIED.,.F.,.F.,(4,1,1,1,1,1,1,1,1,1,1,1,1,1,4),(0.,0.125,
0.1875,0.25,0.3125,0.375,0.4375,0.5,0.625,0.6875,0.75,0.8125,0.875,0.9375,
0.999999754494977),.UNSPECIFIED.);
#567=B_SPLINE_CURVE_WITH_KNOTS('',3,(#30502,#30503,#30504,#30505),
 .UNSPECIFIED.,.F.,.F.,(4,4),(0.,1.),.UNSPECIFIED.);
#568=B_SPLINE_CURVE_WITH_KNOTS('',3,(#30507,#30508,#30509,#30510,#30511,
#30512,#30513,#30514,#30515,#30516,#30517,#30518,#30519),.UNSPECIFIED.,
 .F.,.F.,(4,1,1,1,1,1,1,1,1,1,4),(0.,0.125,0.25,0.3125,0.375,0.5,0.625,
0.6875,0.75,0.875,1.),.UNSPECIFIED.);
#569=B_SPLINE_CURVE_WITH_KNOTS('',3,(#30521,#30522,#30523,#30524),
 .UNSPECIFIED.,.F.,.F.,(4,4),(0.,1.),.UNSPECIFIED.);
#570=B_SPLINE_CURVE_WITH_KNOTS('',3,(#30525,#30526,#30527,#30528,#30529,
#30530,#30531,#30532,#30533,#30534,#30535,#30536,#30537,#30538,#30539,#30540,
#30541),.UNSPECIFIED.,.F.,.F.,(4,1,1,1,1,1,1,1,1,1,1,1,1,1,4),(4.29717416154947E-7,
0.0625,0.125,0.1875,0.25,0.3125,0.375,0.5,0.5625,0.625,0.6875,0.75,0.8125,
0.875,0.915239918615735),.UNSPECIFIED.);
#571=B_SPLINE_CURVE_WITH_KNOTS('',3,(#30543,#30544,#30545,#30546,#30547,
#30548,#30549,#30550,#30551,#30552,#30553,#30554,#30555,#30556,#30557,#30558,
#30559,#30560,#30561,#30562,#30563,#30564,#30565,#30566,#30567,#30568,#30569,
#30570,#30571,#30572,#30573,#30574,#30575,#30576),.UNSPECIFIED.,.F.,.F.,
(4,3,3,3,3,3,3,3,3,3,3,4),(0.,0.125,0.1875,0.214870088595688,0.25,0.3125,
0.375,0.4375,0.5,0.5625,0.625,0.626108993264048),.UNSPECIFIED.);
#572=B_SPLINE_CURVE_WITH_KNOTS('',3,(#30578,#30579,#30580,#30581,#30582,
#30583,#30584,#30585),.UNSPECIFIED.,.F.,.F.,(4,1,1,1,1,4),(1.26755486773303E-5,
0.0625,0.125,0.25,0.375,0.5),.UNSPECIFIED.);
#573=B_SPLINE_CURVE_WITH_KNOTS('',3,(#30587,#30588,#30589,#30590,#30591,
#30592,#30593,#30594,#30595),.UNSPECIFIED.,.F.,.F.,(4,1,1,1,1,1,4),(0.500407782941687,
0.625,0.6875,0.75,0.8125,0.875,0.998506616626188),.UNSPECIFIED.);
#574=B_SPLINE_CURVE_WITH_KNOTS('',3,(#30597,#30598,#30599,#30600,#30601,
#30602,#30603,#30604,#30605,#30606,#30607,#30608,#30609,#30610,#30611,#30612),
 .UNSPECIFIED.,.F.,.F.,(4,3,3,3,3,4),(0.658192818009893,0.6875,0.71693403423044,
0.75,0.875,0.997625654344755),.UNSPECIFIED.);
#575=B_SPLINE_CURVE_WITH_KNOTS('',3,(#30614,#30615,#30616,#30617,#30618,
#30619,#30620,#30621,#30622,#30623,#30624,#30625,#30626,#30627,#30628,#30629,
#30630,#30631,#30632),.UNSPECIFIED.,.F.,.F.,(4,3,3,3,3,3,4),(0.39947571826055,
0.4375,0.5,0.53125,0.5625,0.625,0.658192818009893),.UNSPECIFIED.);
#576=B_SPLINE_CURVE_WITH_KNOTS('',3,(#30633,#30634,#30635,#30636,#30637,
#30638,#30639,#30640,#30641,#30642),.UNSPECIFIED.,.F.,.F.,(4,3,3,4),(0.293194800091934,
0.3125,0.375,0.39947571826055),.UNSPECIFIED.);
#577=B_SPLINE_CURVE_WITH_KNOTS('',3,(#30644,#30645,#30646,#30647,#30648,
#30649,#30650,#30651,#30652,#30653,#30654,#30655,#30656,#30657),
 .UNSPECIFIED.,.F.,.F.,(4,1,1,1,1,1,1,1,1,1,1,4),(0.298021461655708,0.3125,
0.375,0.5,0.625,0.75,0.8125,0.84375,0.875,0.90625,0.9375,1.),
 .UNSPECIFIED.);
#578=B_SPLINE_CURVE_WITH_KNOTS('',3,(#30660,#30661,#30662,#30663,#30664,
#30665,#30666,#30667,#30668,#30669,#30670,#30671,#30672,#30673,#30674,#30675,
#30676,#30677,#30678,#30679,#30680,#30681,#30682,#30683,#30684,#30685,#30686,
#30687,#30688,#30689,#30690,#30691,#30692,#30693,#30694,#30695,#30696),
 .UNSPECIFIED.,.F.,.F.,(4,3,3,3,3,3,3,3,3,3,3,3,4),(2.62189710416264E-7,
0.0625,0.09375,0.125,0.15625,0.1875,0.25,0.367359141751235,0.375,0.5,0.625,
0.6875,0.701590233395244),.UNSPECIFIED.);
#579=B_SPLINE_CURVE_WITH_KNOTS('',3,(#30698,#30699,#30700,#30701,#30702,
#30703,#30704,#30705,#30706,#30707,#30708,#30709,#30710,#30711),
 .UNSPECIFIED.,.F.,.F.,(4,1,1,1,1,1,1,1,1,1,1,4),(0.298831604432797,0.3125,
0.375,0.5,0.625,0.75,0.8125,0.84375,0.875,0.90625,0.9375,1.),
 .UNSPECIFIED.);
#580=B_SPLINE_CURVE_WITH_KNOTS('',3,(#30714,#30715,#30716,#30717,#30718,
#30719,#30720,#30721,#30722,#30723,#30724,#30725,#30726,#30727,#30728,#30729,
#30730,#30731,#30732,#30733,#30734,#30735,#30736,#30737,#30738,#30739,#30740,
#30741,#30742,#30743,#30744,#30745,#30746,#30747,#30748,#30749,#30750),
 .UNSPECIFIED.,.F.,.F.,(4,3,3,3,3,3,3,3,3,3,3,3,4),(2.66010736456726E-7,
0.0625,0.09375,0.125,0.15625,0.1875,0.25,0.365514712737838,0.375,0.5,0.625,
0.6875,0.700679367798627),.UNSPECIFIED.);
#581=B_SPLINE_CURVE_WITH_KNOTS('',3,(#30752,#30753,#30754,#30755,#30756,
#30757,#30758,#30759,#30760,#30761,#30762,#30763,#30764,#30765),
 .UNSPECIFIED.,.F.,.F.,(4,1,1,1,1,1,1,1,1,1,1,4),(0.299787333569703,0.3125,
0.375,0.5,0.625,0.75,0.8125,0.84375,0.875,0.90625,0.9375,1.),
 .UNSPECIFIED.);
#582=B_SPLINE_CURVE_WITH_KNOTS('',3,(#30768,#30769,#30770,#30771,#30772,
#30773,#30774,#30775,#30776,#30777,#30778,#30779,#30780,#30781,#30782,#30783,
#30784,#30785,#30786,#30787,#30788,#30789,#30790,#30791,#30792,#30793,#30794,
#30795,#30796,#30797,#30798,#30799,#30800,#30801,#30802,#30803,#30804),
 .UNSPECIFIED.,.F.,.F.,(4,3,3,3,3,3,3,3,3,3,3,3,4),(2.75012543287525E-7,
0.0625,0.09375,0.125,0.15625,0.1875,0.25,0.363598682235725,0.375,0.5,0.625,
0.6875,0.699678783356034),.UNSPECIFIED.);
#583=B_SPLINE_CURVE_WITH_KNOTS('',3,(#30806,#30807,#30808,#30809,#30810,
#30811,#30812,#30813,#30814,#30815,#30816,#30817,#30818,#30819),
 .UNSPECIFIED.,.F.,.F.,(4,1,1,1,1,1,1,1,1,1,1,4),(0.300810905459472,0.3125,
0.375,0.5,0.625,0.75,0.8125,0.84375,0.875,0.90625,0.9375,1.),
 .UNSPECIFIED.);
#584=B_SPLINE_CURVE_WITH_KNOTS('',3,(#30822,#30823,#30824,#30825,#30826,
#30827,#30828,#30829,#30830,#30831,#30832,#30833,#30834,#30835,#30836,#30837,
#30838,#30839,#30840,#30841,#30842,#30843,#30844,#30845,#30846,#30847,#30848,
#30849,#30850,#30851,#30852,#30853,#30854,#30855,#30856,#30857,#30858),
 .UNSPECIFIED.,.F.,.F.,(4,3,3,3,3,3,3,3,3,3,3,3,4),(2.7737565455879E-7,
0.0625,0.09375,0.125,0.15625,0.1875,0.25,0.361643443501042,0.375,0.5,0.625,
0.6875,0.698643471576761),.UNSPECIFIED.);
#585=B_SPLINE_CURVE_WITH_KNOTS('',3,(#30860,#30861,#30862,#30863,#30864,
#30865,#30866,#30867,#30868,#30869,#30870,#30871,#30872,#30873),
 .UNSPECIFIED.,.F.,.F.,(4,1,1,1,1,1,1,1,1,1,1,4),(0.301839172550323,0.3125,
0.375,0.5,0.625,0.75,0.8125,0.84375,0.875,0.90625,0.9375,1.),
 .UNSPECIFIED.);
#586=B_SPLINE_CURVE_WITH_KNOTS('',3,(#30876,#30877,#30878,#30879,#30880,
#30881,#30882,#30883,#30884,#30885,#30886,#30887,#30888,#30889,#30890,#30891,
#30892,#30893,#30894,#30895,#30896,#30897,#30898,#30899,#30900,#30901,#30902,
#30903,#30904,#30905,#30906,#30907,#30908,#30909,#30910,#30911,#30912),
 .UNSPECIFIED.,.F.,.F.,(4,3,3,3,3,3,3,3,3,3,3,3,4),(2.80962005521138E-7,
0.0625,0.09375,0.125,0.15625,0.1875,0.25,0.359695004612115,0.375,0.5,0.625,
0.6875,0.697655525115426),.UNSPECIFIED.);
#587=B_SPLINE_CURVE_WITH_KNOTS('',3,(#30914,#30915,#30916,#30917,#30918,
#30919,#30920,#30921,#30922,#30923,#30924,#30925,#30926,#30927),
 .UNSPECIFIED.,.F.,.F.,(4,1,1,1,1,1,1,1,1,1,1,4),(0.302853998408664,0.3125,
0.375,0.5,0.625,0.75,0.8125,0.84375,0.875,0.90625,0.9375,1.),
 .UNSPECIFIED.);
#588=B_SPLINE_CURVE_WITH_KNOTS('',3,(#30930,#30931,#30932,#30933,#30934,
#30935,#30936,#30937,#30938,#30939,#30940,#30941,#30942,#30943,#30944,#30945,
#30946,#30947,#30948,#30949,#30950,#30951,#30952,#30953,#30954,#30955,#30956,
#30957,#30958,#30959,#30960,#30961,#30962,#30963),.UNSPECIFIED.,.F.,.F.,
(4,3,3,3,3,3,3,3,3,3,3,4),(2.873516990008E-7,0.0625,0.09375,0.125,0.15625,
0.1875,0.25,0.357103578474147,0.375,0.5,0.625,0.694959544378405),
 .UNSPECIFIED.);
#589=B_SPLINE_CURVE_WITH_KNOTS('',3,(#30965,#30966,#30967,#30968,#30969,
#30970,#30971,#30972,#30973,#30974,#30975,#30976,#30977,#30978,#30979),
 .UNSPECIFIED.,.F.,.F.,(4,1,1,1,1,1,1,1,1,1,1,1,4),(0.304441335563685,0.3125,
0.375,0.5,0.625,0.6875,0.75,0.8125,0.84375,0.875,0.90625,0.9375,1.),
 .UNSPECIFIED.);
#590=B_SPLINE_CURVE_WITH_KNOTS('',3,(#30982,#30983,#30984,#30985,#30986,
#30987,#30988,#30989,#30990,#30991,#30992,#30993,#30994,#30995,#30996),
 .UNSPECIFIED.,.F.,.F.,(4,1,1,1,1,1,1,1,1,1,1,1,4),(2.84937768142854E-7,
0.0625,0.09375,0.125,0.15625,0.1875,0.25,0.3125,0.375,0.5,0.625,0.6875,
0.69476673108169),.UNSPECIFIED.);
#591=B_SPLINE_CURVE_WITH_KNOTS('',3,(#30998,#30999,#31000,#31001,#31002,
#31003,#31004,#31005,#31006,#31007,#31008,#31009,#31010,#31011,#31012),
 .UNSPECIFIED.,.F.,.F.,(4,1,1,1,1,1,1,1,1,1,1,1,4),(0.305513267453618,0.3125,
0.375,0.5,0.625,0.6875,0.75,0.8125,0.84375,0.875,0.90625,0.9375,1.),
 .UNSPECIFIED.);
#592=B_SPLINE_CURVE_WITH_KNOTS('',3,(#31015,#31016,#31017,#31018,#31019,
#31020,#31021,#31022,#31023,#31024,#31025,#31026,#31027,#31028,#31029),
 .UNSPECIFIED.,.F.,.F.,(4,1,1,1,1,1,1,1,1,1,1,1,4),(2.86307819456861E-7,
0.0625,0.09375,0.125,0.15625,0.1875,0.25,0.3125,0.375,0.5,0.625,0.6875,
0.693739351488113),.UNSPECIFIED.);
#593=B_SPLINE_CURVE_WITH_KNOTS('',3,(#31031,#31032,#31033,#31034,#31035,
#31036,#31037,#31038,#31039,#31040,#31041,#31042,#31043,#31044,#31045),
 .UNSPECIFIED.,.F.,.F.,(4,1,1,1,1,1,1,1,1,1,1,1,4),(0.306675627321796,0.3125,
0.375,0.5,0.625,0.6875,0.75,0.8125,0.84375,0.875,0.90625,0.9375,1.),
 .UNSPECIFIED.);
#594=B_SPLINE_CURVE_WITH_KNOTS('',3,(#31048,#31049,#31050,#31051,#31052,
#31053,#31054,#31055,#31056,#31057,#31058,#31059,#31060,#31061,#31062),
 .UNSPECIFIED.,.F.,.F.,(4,1,1,1,1,1,1,1,1,1,1,1,4),(2.94206060623265E-7,
0.0625,0.09375,0.125,0.15625,0.1875,0.25,0.3125,0.375,0.5,0.625,0.6875,
0.692733007429323),.UNSPECIFIED.);
#595=B_SPLINE_CURVE_WITH_KNOTS('',3,(#31064,#31065,#31066,#31067,#31068,
#31069,#31070,#31071,#31072,#31073,#31074,#31075,#31076,#31077,#31078),
 .UNSPECIFIED.,.F.,.F.,(4,1,1,1,1,1,1,1,1,1,1,1,4),(0.307485444826301,0.3125,
0.375,0.5,0.625,0.6875,0.75,0.8125,0.84375,0.875,0.90625,0.9375,1.),
 .UNSPECIFIED.);
#596=B_SPLINE_CURVE_WITH_KNOTS('',3,(#31081,#31082,#31083,#31084,#31085,
#31086,#31087,#31088,#31089,#31090,#31091,#31092,#31093,#31094,#31095,#31096,
#31097,#31098,#31099,#31100,#31101,#31102,#31103,#31104,#31105,#31106,#31107,
#31108,#31109,#31110,#31111,#31112,#31113,#31114,#31115,#31116,#31117,#31118,
#31119,#31120),.UNSPECIFIED.,.F.,.F.,(4,3,3,3,3,3,3,3,3,3,3,3,3,4),(3.05038783548285E-7,
0.0625,0.09375,0.125,0.15625,0.1875,0.25,0.3125,0.348312622039473,0.375,
0.5,0.625,0.6875,0.691764098829342),.UNSPECIFIED.);
#597=B_SPLINE_CURVE_WITH_KNOTS('',3,(#31122,#31123,#31124,#31125,#31126,
#31127,#31128,#31129,#31130,#31131,#31132,#31133,#31134,#31135,#31136),
 .UNSPECIFIED.,.F.,.F.,(4,1,1,1,1,1,1,1,1,1,1,1,4),(0.308404661026527,0.3125,
0.375,0.5,0.625,0.6875,0.75,0.8125,0.84375,0.875,0.90625,0.9375,1.),
 .UNSPECIFIED.);
#598=B_SPLINE_CURVE_WITH_KNOTS('',3,(#31139,#31140,#31141,#31142,#31143,
#31144,#31145,#31146,#31147,#31148,#31149,#31150,#31151,#31152,#31153,#31154,
#31155,#31156,#31157,#31158,#31159,#31160,#31161,#31162,#31163,#31164,#31165,
#31166,#31167,#31168,#31169,#31170,#31171,#31172,#31173,#31174,#31175,#31176,
#31177,#31178),.UNSPECIFIED.,.F.,.F.,(4,3,3,3,3,3,3,3,3,3,3,3,3,4),(2.88155531850153E-7,
0.0625,0.09375,0.125,0.15625,0.1875,0.25,0.3125,0.346342722159355,0.375,
0.5,0.625,0.6875,0.690961556714303),.UNSPECIFIED.);
#599=B_SPLINE_CURVE_WITH_KNOTS('',3,(#31180,#31181,#31182,#31183,#31184,
#31185,#31186,#31187,#31188,#31189,#31190,#31191,#31192,#31193),
 .UNSPECIFIED.,.F.,.F.,(4,1,1,1,1,1,1,1,1,1,1,4),(0.302671489156909,0.3125,
0.375,0.5,0.625,0.75,0.8125,0.84375,0.875,0.90625,0.9375,1.),
 .UNSPECIFIED.);
#600=B_SPLINE_CURVE_WITH_KNOTS('',3,(#31197,#31198,#31199,#31200,#31201,
#31202,#31203,#31204,#31205,#31206,#31207,#31208,#31209,#31210,#31211,#31212,
#31213,#31214,#31215,#31216,#31217,#31218,#31219,#31220,#31221,#31222,#31223,
#31224),.UNSPECIFIED.,.F.,.F.,(4,3,3,3,3,3,3,3,3,4),(0.,0.0625,0.09375,
0.125,0.15625,0.1875,0.25,0.364633141489333,0.375,0.499908337236844),
 .UNSPECIFIED.);
#601=B_SPLINE_CURVE_WITH_KNOTS('',3,(#31225,#31226,#31227,#31228,#31229,
#31230,#31231,#31232,#31233,#31234),.UNSPECIFIED.,.F.,.F.,(4,3,3,4),(0.5,
0.625,0.6875,0.699974107082008),.UNSPECIFIED.);
#602=B_SPLINE_CURVE_WITH_KNOTS('',3,(#31236,#31237,#31238,#31239,#31240,
#31241,#31242,#31243,#31244,#31245),.UNSPECIFIED.,.F.,.F.,(4,3,3,4),(0.295540353636982,
0.3125,0.375,0.5),.UNSPECIFIED.);
#603=B_SPLINE_CURVE_WITH_KNOTS('',3,(#31247,#31248,#31249,#31250,#31251,
#31252,#31253,#31254,#31255,#31256,#31257,#31258,#31259,#31260,#31261,#31262,
#31263,#31264,#31265,#31266,#31267,#31268,#31269,#31270,#31271),
 .UNSPECIFIED.,.F.,.F.,(4,3,3,3,3,3,3,3,4),(0.500189461797682,0.625,0.75,
0.8125,0.84375,0.875,0.90625,0.9375,0.999997786243782),.UNSPECIFIED.);
#604=B_SPLINE_CURVE_WITH_KNOTS('',3,(#31273,#31274,#31275,#31276,#31277,
#31278,#31279,#31280),.UNSPECIFIED.,.F.,.F.,(4,1,1,1,1,4),(0.,0.0625,0.125,
0.25,0.375,0.5),.UNSPECIFIED.);
#605=B_SPLINE_CURVE_WITH_KNOTS('',3,(#31282,#31283,#31284,#31285,#31286,
#31287,#31288,#31289,#31290),.UNSPECIFIED.,.F.,.F.,(4,1,1,1,1,1,4),(0.500434798583671,
0.625,0.6875,0.75,0.8125,0.875,0.999998086846501),.UNSPECIFIED.);
#606=B_SPLINE_CURVE_WITH_KNOTS('',3,(#31291,#31292,#31293,#31294,#31295,
#31296,#31297,#31298,#31299,#31300,#31301,#31302,#31303),.UNSPECIFIED.,
 .F.,.F.,(4,1,1,1,1,1,1,1,1,1,4),(0.,0.0625,0.09375,0.125,0.15625,0.1875,
0.25,0.375,0.5,0.625,0.71355566892686),.UNSPECIFIED.);
#607=B_SPLINE_CURVE_WITH_KNOTS('',3,(#31305,#31306,#31307,#31308,#31309),
 .UNSPECIFIED.,.F.,.F.,(4,1,4),(0.271066582727647,0.375,0.4994045688759),
 .UNSPECIFIED.);
#608=B_SPLINE_CURVE_WITH_KNOTS('',3,(#31311,#31312,#31313,#31314,#31315,
#31316,#31317,#31318,#31319,#31320,#31321,#31322),.UNSPECIFIED.,.F.,.F.,
(4,1,1,1,1,1,1,1,1,4),(0.4994045688759,0.5,0.625,0.75,0.8125,0.84375,0.875,
0.90625,0.9375,1.),.UNSPECIFIED.);
#609=B_SPLINE_CURVE_WITH_KNOTS('',3,(#31324,#31325,#31326,#31327,#31328,
#31329,#31330,#31331,#31332,#31333,#31334,#31335,#31336,#31337,#31338,#31339,
#31340,#31341,#31342,#31343,#31344,#31345,#31346,#31347,#31348,#31349,#31350,
#31351,#31352,#31353,#31354),.UNSPECIFIED.,.F.,.F.,(4,3,3,3,3,3,3,3,3,3,
4),(1.20911684619388E-6,0.125,0.25,0.375,0.5,0.625,0.6875,0.75,0.8125,0.875,
0.999824037442535),.UNSPECIFIED.);
#610=B_SPLINE_CURVE_WITH_KNOTS('',3,(#31356,#31357,#31358,#31359,#31360,
#31361,#31362,#31363,#31364,#31365,#31366,#31367),.UNSPECIFIED.,.F.,.F.,
(4,1,1,1,1,1,1,1,1,4),(1.15789001547902E-5,0.0625,0.09375,0.125,0.15625,
0.1875,0.25,0.3125,0.375,0.463468292977054),.UNSPECIFIED.);
#611=B_SPLINE_CURVE_WITH_KNOTS('',3,(#31368,#31369,#31370,#31371,#31372,
#31373),.UNSPECIFIED.,.F.,.F.,(4,1,1,4),(0.463468292977054,0.5,0.625,0.743178274051315),
 .UNSPECIFIED.);
#612=B_SPLINE_CURVE_WITH_KNOTS('',3,(#31375,#31376,#31377,#31378,#31379),
 .UNSPECIFIED.,.F.,.F.,(4,1,4),(0.256944255797255,0.375,0.499319773304833),
 .UNSPECIFIED.);
#613=B_SPLINE_CURVE_WITH_KNOTS('',3,(#31381,#31382,#31383,#31384,#31385,
#31386,#31387,#31388,#31389,#31390,#31391,#31392,#31393),.UNSPECIFIED.,
 .F.,.F.,(4,1,1,1,1,1,1,1,1,1,4),(0.499319773304833,0.5,0.625,0.6875,0.75,
0.8125,0.84375,0.875,0.90625,0.9375,1.),.UNSPECIFIED.);
#614=B_SPLINE_CURVE_WITH_KNOTS('',3,(#31397,#31398,#31399,#31400,#31401,
#31402,#31403,#31404,#31405,#31406,#31407,#31408),.UNSPECIFIED.,.F.,.F.,
(4,1,1,1,1,1,1,1,1,4),(0.,0.0625,0.09375,0.125,0.15625,0.1875,0.25,0.3125,
0.375,0.5),.UNSPECIFIED.);
#615=B_SPLINE_CURVE_WITH_KNOTS('',3,(#31409,#31410,#31411,#31412,#31413),
 .UNSPECIFIED.,.F.,.F.,(4,1,4),(0.5,0.625,0.742719765959379),
 .UNSPECIFIED.);
#616=B_SPLINE_CURVE_WITH_KNOTS('',3,(#31415,#31416,#31417,#31418,#31419),
 .UNSPECIFIED.,.F.,.F.,(4,1,4),(0.257506245398161,0.375,0.499318574492738),
 .UNSPECIFIED.);
#617=B_SPLINE_CURVE_WITH_KNOTS('',3,(#31421,#31422,#31423,#31424,#31425,
#31426,#31427,#31428,#31429,#31430,#31431,#31432,#31433),.UNSPECIFIED.,
 .F.,.F.,(4,1,1,1,1,1,1,1,1,1,4),(0.499318574492738,0.5,0.625,0.6875,0.75,
0.8125,0.84375,0.875,0.90625,0.9375,1.),.UNSPECIFIED.);
#618=B_SPLINE_CURVE_WITH_KNOTS('',3,(#31437,#31438,#31439,#31440,#31441,
#31442,#31443,#31444,#31445,#31446,#31447,#31448),.UNSPECIFIED.,.F.,.F.,
(4,1,1,1,1,1,1,1,1,4),(0.,0.0625,0.09375,0.125,0.15625,0.1875,0.25,0.3125,
0.375,0.5),.UNSPECIFIED.);
#619=B_SPLINE_CURVE_WITH_KNOTS('',3,(#31449,#31450,#31451,#31452,#31453),
 .UNSPECIFIED.,.F.,.F.,(4,1,4),(0.5,0.625,0.742143863244383),
 .UNSPECIFIED.);
#620=B_SPLINE_CURVE_WITH_KNOTS('',3,(#31455,#31456,#31457,#31458,#31459,
#31460,#31461),.UNSPECIFIED.,.F.,.F.,(4,3,4),(0.339613136872108,0.375,0.499997657275256),
 .UNSPECIFIED.);
#621=B_SPLINE_CURVE_WITH_KNOTS('',3,(#31463,#31464,#31465,#31466,#31467,
#31468,#31469,#31470,#31471,#31472,#31473,#31474,#31475,#31476,#31477,#31478),
 .UNSPECIFIED.,.F.,.F.,(4,3,3,3,3,4),(0.5,0.625,0.718785408996563,0.75,
0.875,1.),.UNSPECIFIED.);
#622=B_SPLINE_CURVE_WITH_KNOTS('',3,(#31480,#31481,#31482,#31483,#31484,
#31485,#31486,#31487,#31488,#31489,#31490,#31491,#31492,#31493,#31494,#31495,
#31496,#31497,#31498,#31499,#31500,#31501,#31502,#31503,#31504),
 .UNSPECIFIED.,.F.,.F.,(4,3,3,3,3,3,3,3,4),(0.125,0.25,0.3125,0.375,0.4375,
0.5,0.625,0.75,1.),.UNSPECIFIED.);
#623=B_SPLINE_CURVE_WITH_KNOTS('',3,(#31506,#31507,#31508,#31509),
 .UNSPECIFIED.,.F.,.F.,(4,4),(9.19960507825898E-5,0.125),.UNSPECIFIED.);
#624=B_SPLINE_CURVE_WITH_KNOTS('',3,(#31511,#31512,#31513,#31514,#31515,
#31516,#31517),.UNSPECIFIED.,.F.,.F.,(4,3,4),(4.03926038141589E-9,0.621738318522071,
0.999999432402183),.UNSPECIFIED.);
#625=B_SPLINE_CURVE_WITH_KNOTS('',3,(#31519,#31520,#31521,#31522,#31523,
#31524,#31525,#31526,#31527,#31528,#31529,#31530,#31531,#31532,#31533,#31534),
 .UNSPECIFIED.,.F.,.F.,(4,3,3,3,3,4),(0.,0.25,0.5,0.625,0.75,0.999999984180473),
 .UNSPECIFIED.);
#626=B_SPLINE_CURVE_WITH_KNOTS('',3,(#31540,#31541,#31542,#31543,#31544,
#31545,#31546,#31547,#31548,#31549,#31550,#31551,#31552,#31553,#31554,#31555,
#31556,#31557,#31558,#31559,#31560,#31561,#31562,#31563,#31564,#31565,#31566,
#31567),.UNSPECIFIED.,.F.,.F.,(4,3,3,3,3,3,3,3,3,4),(0.,0.25,0.375,0.5,
0.625,0.6875,0.75,0.8125,0.875,0.999999996427379),.UNSPECIFIED.);
#627=B_SPLINE_CURVE_WITH_KNOTS('',3,(#31569,#31570,#31571,#31572,#31573,
#31574,#31575,#31576,#31577,#31578,#31579,#31580,#31581,#31582,#31583,#31584,
#31585,#31586,#31587,#31588,#31589,#31590),.UNSPECIFIED.,.F.,.F.,(4,3,3,
3,3,3,3,4),(5.11212140420089E-8,0.0625,0.09375,0.125,0.15625,0.1875,0.25,
0.251514333796608),.UNSPECIFIED.);
#628=B_SPLINE_CURVE_WITH_KNOTS('',3,(#31592,#31593,#31594,#31595,#31596,
#31597,#31598,#31599,#31600,#31601,#31602,#31603,#31604,#31605,#31606,#31607),
 .UNSPECIFIED.,.F.,.F.,(4,3,3,3,3,4),(0.251514333796608,0.3125,0.375,0.4375,
0.5,0.508539107283651),.UNSPECIFIED.);
#629=B_SPLINE_CURVE_WITH_KNOTS('',3,(#31609,#31610,#31611,#31612,#31613,
#31614,#31615,#31616,#31617,#31618,#31619,#31620,#31621,#31622,#31623,#31624),
 .UNSPECIFIED.,.F.,.F.,(4,3,3,3,3,4),(0.508539107283651,0.5275897246703,
0.625,0.75,0.875,1.),.UNSPECIFIED.);
#630=B_SPLINE_CURVE_WITH_KNOTS('',3,(#31626,#31627,#31628,#31629,#31630,
#31631,#31632,#31633,#31634,#31635,#31636,#31637,#31638,#31639,#31640,#31641,
#31642,#31643,#31644,#31645,#31646,#31647,#31648,#31649,#31650,#31651,#31652,
#31653,#31654,#31655,#31656,#31657,#31658,#31659,#31660,#31661,#31662,#31663,
#31664,#31665,#31666,#31667,#31668,#31669,#31670,#31671,#31672,#31673,#31674,
#31675,#31676,#31677,#31678,#31679,#31680,#31681,#31682,#31683,#31684,#31685,
#31686,#31687,#31688,#31689,#31690,#31691,#31692,#31693,#31694,#31695,#31696,
#31697,#31698,#31699,#31700,#31701,#31702,#31703,#31704,#31705,#31706,#31707,
#31708,#31709,#31710,#31711,#31712,#31713,#31714,#31715,#31716,#31717,#31718,
#31719,#31720,#31721,#31722,#31723,#31724,#31725,#31726,#31727,#31728,#31729,
#31730,#31731,#31732,#31733,#31734,#31735,#31736,#31737,#31738,#31739,#31740,
#31741,#31742,#31743,#31744,#31745,#31746,#31747,#31748,#31749,#31750,#31751,
#31752,#31753,#31754,#31755,#31756,#31757,#31758,#31759,#31760,#31761,#31762,
#31763,#31764,#31765,#31766,#31767,#31768,#31769,#31770,#31771,#31772,#31773,
#31774,#31775,#31776,#31777,#31778,#31779,#31780,#31781,#31782,#31783,#31784,
#31785),.UNSPECIFIED.,.F.,.F.,(4,3,3,3,3,3,3,3,3,3,3,3,3,3,3,3,3,3,3,3,
3,3,3,3,3,3,3,3,3,3,3,3,3,3,3,3,3,3,3,3,3,3,3,3,3,3,3,3,3,3,3,3,3,4),(0.,
0.03125,0.046875,0.0546875,0.0625,0.0703125,0.078125,0.09375,0.109375,0.125,
0.134813898918915,0.140625,0.15625,0.171875,0.1875,0.203125,0.21875,0.234375,
0.25,0.28125,0.296875,0.3125,0.328125,0.34375,0.356926011470558,0.359375,
0.375,0.390625,0.40625,0.421875,0.4375,0.46875,0.5,0.53125,0.5625,0.59375,
0.625,0.626999867348899,0.6875,0.75,0.8125,0.84375,0.855575696034116,0.875,
0.90625,0.921875,0.929958125829058,0.9375,0.953125,0.9609375,0.96875,0.9765625,
0.984375,0.999999930559409),.UNSPECIFIED.);
#631=B_SPLINE_CURVE_WITH_KNOTS('',3,(#31787,#31788,#31789,#31790,#31791,
#31792,#31793,#31794,#31795,#31796,#31797,#31798,#31799,#31800,#31801,#31802,
#31803,#31804,#31805,#31806,#31807,#31808,#31809,#31810,#31811,#31812,#31813,
#31814,#31815,#31816,#31817,#31818,#31819,#31820,#31821,#31822,#31823,#31824,
#31825,#31826,#31827,#31828,#31829,#31830,#31831,#31832,#31833,#31834,#31835,
#31836,#31837,#31838,#31839),.UNSPECIFIED.,.F.,.F.,(4,1,1,1,1,1,1,1,1,1,
1,1,1,1,1,1,1,1,1,1,1,1,1,1,1,1,1,1,1,1,1,1,1,1,1,1,1,1,1,1,1,1,1,1,1,1,
1,1,1,1,4),(2.33524176194205E-8,0.015625,0.0234375,0.03125,0.0390625,0.046875,
0.0625,0.078125,0.09375,0.125,0.15625,0.1875,0.25,0.3125,0.375,0.40625,
0.4375,0.46875,0.484375,0.5,0.515625,0.53125,0.5625,0.578125,0.59375,0.609375,
0.625,0.640625,0.65625,0.671875,0.6875,0.703125,0.71875,0.75,0.765625,0.78125,
0.796875,0.8125,0.828125,0.84375,0.859375,0.875,0.890625,0.90625,0.921875,
0.9296875,0.9375,0.9453125,0.953125,0.96875,1.),.UNSPECIFIED.);
#632=B_SPLINE_CURVE_WITH_KNOTS('',3,(#31841,#31842,#31843,#31844,#31845,
#31846,#31847,#31848,#31849,#31850,#31851,#31852,#31853,#31854,#31855,#31856),
 .UNSPECIFIED.,.F.,.F.,(4,3,3,3,3,4),(0.,0.125,0.25,0.375,0.4375,0.461967251686174),
 .UNSPECIFIED.);
#633=B_SPLINE_CURVE_WITH_KNOTS('',3,(#31858,#31859,#31860,#31861,#31862,
#31863,#31864,#31865,#31866,#31867,#31868,#31869,#31870,#31871,#31872,#31873),
 .UNSPECIFIED.,.F.,.F.,(4,3,3,3,3,4),(0.461967251686174,0.5,0.5625,0.625,
0.6875,0.748603143222001),.UNSPECIFIED.);
#634=B_SPLINE_CURVE_WITH_KNOTS('',3,(#31875,#31876,#31877,#31878,#31879,
#31880,#31881,#31882,#31883,#31884,#31885,#31886,#31887,#31888,#31889,#31890,
#31891,#31892,#31893,#31894,#31895,#31896),.UNSPECIFIED.,.F.,.F.,(4,3,3,
3,3,3,3,4),(0.748603143222001,0.75,0.8125,0.84375,0.875,0.90625,0.9375,
0.999999927233155),.UNSPECIFIED.);
#635=B_SPLINE_CURVE_WITH_KNOTS('',3,(#31898,#31899,#31900,#31901,#31902,
#31903,#31904,#31905,#31906),.UNSPECIFIED.,.F.,.F.,(4,1,1,1,1,1,4),(0.,
0.125,0.25,0.5,0.625,0.75,1.),.UNSPECIFIED.);
#636=B_SPLINE_CURVE_WITH_KNOTS('',3,(#31914,#31915,#31916,#31917,#31918,
#31919,#31920),.UNSPECIFIED.,.F.,.F.,(4,3,4),(0.028486178614514,0.5,1.),
 .UNSPECIFIED.);
#637=B_SPLINE_CURVE_WITH_KNOTS('',3,(#31922,#31923,#31924,#31925),
 .UNSPECIFIED.,.F.,.F.,(4,4),(0.,0.028486178614514),.UNSPECIFIED.);
#638=B_SPLINE_CURVE_WITH_KNOTS('',3,(#31927,#31928,#31929,#31930),
 .UNSPECIFIED.,.F.,.F.,(4,4),(0.875,1.),.UNSPECIFIED.);
#639=B_SPLINE_CURVE_WITH_KNOTS('',3,(#31932,#31933,#31934,#31935,#31936,
#31937,#31938,#31939,#31940,#31941,#31942,#31943,#31944,#31945,#31946,#31947,
#31948,#31949,#31950,#31951,#31952,#31953,#31954,#31955,#31956),
 .UNSPECIFIED.,.F.,.F.,(4,3,3,3,3,3,3,3,4),(0.,0.25,0.375,0.5,0.5625,0.625,
0.6875,0.75,0.875),.UNSPECIFIED.);
#640=B_SPLINE_CURVE_WITH_KNOTS('',3,(#31958,#31959,#31960,#31961,#31962,
#31963,#31964,#31965,#31966,#31967,#31968,#31969,#31970),.UNSPECIFIED.,
 .F.,.F.,(4,3,3,3,4),(0.,0.125,0.25,0.279719843926451,0.375),
 .UNSPECIFIED.);
#641=B_SPLINE_CURVE_WITH_KNOTS('',3,(#31972,#31973,#31974,#31975,#31976,
#31977,#31978,#31979,#31980,#31981,#31982,#31983,#31984,#31985,#31986,#31987,
#31988,#31989,#31990,#31991,#31992,#31993),.UNSPECIFIED.,.F.,.F.,(4,3,3,
3,3,3,3,4),(0.375,0.5,0.625,0.6875,0.75,0.8125,0.875,1.),.UNSPECIFIED.);
#642=B_SPLINE_CURVE_WITH_KNOTS('',3,(#31995,#31996,#31997,#31998,#31999,
#32000,#32001,#32002,#32003,#32004,#32005,#32006,#32007,#32008,#32009,#32010,
#32011,#32012,#32013),.UNSPECIFIED.,.F.,.F.,(4,3,3,3,3,3,4),(8.04807277738882E-5,
0.125,0.1875,0.25,0.3125,0.375,0.5),.UNSPECIFIED.);
#643=B_SPLINE_CURVE_WITH_KNOTS('',3,(#32015,#32016,#32017,#32018,#32019,
#32020,#32021,#32022,#32023,#32024,#32025,#32026,#32027),.UNSPECIFIED.,
 .F.,.F.,(4,3,3,3,4),(0.500165768693434,0.732349597796809,0.75,0.875,1.),
 .UNSPECIFIED.);
#644=B_SPLINE_CURVE_WITH_KNOTS('',3,(#32029,#32030,#32031,#32032,#32033,
#32034,#32035,#32036,#32037,#32038,#32039,#32040,#32041,#32042,#32043,#32044,
#32045,#32046,#32047,#32048,#32049,#32050,#32051,#32052,#32053,#32054,#32055,
#32056),.UNSPECIFIED.,.F.,.F.,(4,3,3,3,3,3,3,3,3,4),(1.05884092999222E-5,
0.125,0.25,0.3125,0.375,0.4375,0.5,0.625,0.75,1.),.UNSPECIFIED.);
#645=B_SPLINE_CURVE_WITH_KNOTS('',3,(#32058,#32059,#32060,#32061,#32062,
#32063,#32064),.UNSPECIFIED.,.F.,.F.,(4,3,4),(0.,0.5,0.999998285932114),
 .UNSPECIFIED.);
#646=B_SPLINE_CURVE_WITH_KNOTS('',3,(#32066,#32067,#32068,#32069,#32070,
#32071,#32072,#32073,#32074,#32075),.UNSPECIFIED.,.F.,.F.,(4,3,3,4),(0.,
0.5,0.75,1.),.UNSPECIFIED.);
#647=B_SPLINE_CURVE_WITH_KNOTS('',3,(#32081,#32082,#32083,#32084,#32085,
#32086,#32087),.UNSPECIFIED.,.F.,.F.,(4,3,4),(9.24712860392496E-13,0.5,
1.),.UNSPECIFIED.);
#648=B_SPLINE_CURVE_WITH_KNOTS('',3,(#32089,#32090,#32091,#32092,#32093,
#32094,#32095,#32096,#32097,#32098,#32099,#32100,#32101,#32102,#32103,#32104,
#32105,#32106,#32107),.UNSPECIFIED.,.F.,.F.,(4,1,1,1,1,1,1,1,1,1,1,1,1,
1,1,1,4),(0.000133962196229911,0.0625,0.09375,0.125,0.15625,0.1875,0.25,
0.375,0.4375,0.5,0.5625,0.625,0.6875,0.75,0.8125,0.875,1.),
 .UNSPECIFIED.);
#649=B_SPLINE_CURVE_WITH_KNOTS('',3,(#32109,#32110,#32111,#32112,#32113,
#32114,#32115,#32116,#32117,#32118,#32119,#32120,#32121,#32122,#32123,#32124,
#32125,#32126,#32127,#32128,#32129,#32130,#32131,#32132,#32133,#32134,#32135,
#32136,#32137,#32138,#32139,#32140,#32141,#32142,#32143,#32144,#32145,#32146,
#32147,#32148,#32149,#32150,#32151,#32152,#32153,#32154,#32155,#32156,#32157,
#32158,#32159,#32160,#32161,#32162,#32163,#32164,#32165,#32166,#32167,#32168,
#32169,#32170,#32171,#32172,#32173,#32174,#32175,#32176,#32177,#32178,#32179,
#32180,#32181,#32182,#32183,#32184,#32185,#32186,#32187,#32188,#32189,#32190,
#32191,#32192,#32193,#32194,#32195,#32196,#32197,#32198,#32199,#32200,#32201,
#32202,#32203,#32204,#32205,#32206,#32207,#32208,#32209,#32210,#32211,#32212,
#32213,#32214,#32215,#32216,#32217,#32218,#32219,#32220,#32221,#32222,#32223,
#32224,#32225,#32226,#32227,#32228,#32229,#32230,#32231,#32232,#32233,#32234,
#32235,#32236,#32237,#32238,#32239,#32240,#32241,#32242,#32243,#32244,#32245,
#32246,#32247,#32248,#32249,#32250,#32251,#32252,#32253,#32254,#32255,#32256,
#32257,#32258,#32259,#32260,#32261,#32262,#32263,#32264,#32265,#32266,#32267,
#32268,#32269,#32270,#32271),.UNSPECIFIED.,.F.,.F.,(4,3,3,3,3,3,3,3,3,3,
3,3,3,3,3,3,3,3,3,3,3,3,3,3,3,3,3,3,3,3,3,3,3,3,3,3,3,3,3,3,3,3,3,3,3,3,
3,3,3,3,3,3,3,3,4),(0.,0.03125,0.046875,0.0546875,0.0625,0.0703125,0.078125,
0.09375,0.109375,0.125,0.132706893319552,0.140625,0.15625,0.171875,0.1875,
0.203125,0.21875,0.234375,0.25,0.28125,0.296875,0.3125,0.328125,0.34375,
0.354656215967293,0.359375,0.375,0.390625,0.40625,0.421875,0.4375,0.453125,
0.46875,0.484375,0.5,0.53125,0.5625,0.59375,0.625,0.627549721648294,0.65625,
0.6875,0.75,0.8125,0.84375,0.85684618431259,0.875,0.90625,0.921875,0.930906239968274,
0.9375,0.953125,0.96875,0.984375,0.999999864466775),.UNSPECIFIED.);
#650=B_SPLINE_CURVE_WITH_KNOTS('',3,(#32272,#32273,#32274,#32275,#32276,
#32277,#32278,#32279,#32280,#32281,#32282),.UNSPECIFIED.,.F.,.F.,(4,1,1,
1,1,1,1,1,4),(6.13123545891853E-8,0.015625,0.03125,0.046875,0.0625,0.078125,
0.09375,0.125,0.142413158676735),.UNSPECIFIED.);
#651=B_SPLINE_CURVE_WITH_KNOTS('',3,(#32287,#32288,#32289,#32290,#32291,
#32292),.UNSPECIFIED.,.F.,.F.,(4,2,4),(-0.386868606697558,-0.228081755753299,
-0.000106832852268002),.UNSPECIFIED.);
#652=B_SPLINE_CURVE_WITH_KNOTS('',3,(#32294,#32295,#32296,#32297,#32298,
#32299,#32300,#32301,#32302,#32303,#32304,#32305,#32306,#32307,#32308,#32309,
#32310,#32311,#32312),.UNSPECIFIED.,.F.,.F.,(4,1,1,1,1,1,1,1,1,1,1,1,1,
1,1,1,4),(0.,0.125,0.1875,0.21875,0.25,0.28125,0.3125,0.375,0.5,0.625,0.75,
0.8125,0.84375,0.875,0.90625,0.9375,1.),.UNSPECIFIED.);
#653=B_SPLINE_CURVE_WITH_KNOTS('',3,(#32316,#32317,#32318,#32319,#32320,
#32321,#32322,#32323,#32324,#32325,#32326,#32327,#32328,#32329,#32330,#32331,
#32332,#32333,#32334,#32335,#32336,#32337,#32338,#32339,#32340,#32341,#32342,
#32343,#32344,#32345,#32346,#32347,#32348,#32349,#32350,#32351,#32352,#32353,
#32354,#32355,#32356,#32357,#32358,#32359,#32360,#32361),.UNSPECIFIED.,
 .F.,.F.,(4,3,3,3,3,3,3,3,3,3,3,3,3,3,3,4),(2.87286426861497E-7,0.0625,
0.09375,0.125,0.15625,0.1875,0.25,0.357099507040325,0.375,0.5,0.625,0.75,
0.8125,0.84375,0.875,0.999999985631448),.UNSPECIFIED.);
#654=B_SPLINE_CURVE_WITH_KNOTS('',3,(#32362,#32363,#32364,#32365,#32366,
#32367,#32368,#32369,#32370,#32371,#32372,#32373,#32374,#32375,#32376,#32377,
#32378,#32379,#32380,#32381,#32382),.UNSPECIFIED.,.F.,.F.,(4,1,1,1,1,1,
1,1,1,1,1,1,1,1,1,1,1,1,4),(0.,0.0625,0.09375,0.125,0.15625,0.1875,0.25,
0.3125,0.375,0.5,0.625,0.6875,0.75,0.8125,0.84375,0.875,0.90625,0.9375,
0.999999797571635),.UNSPECIFIED.);
#655=B_SPLINE_CURVE_WITH_KNOTS('',3,(#32387,#32388,#32389,#32390,#32391,
#32392,#32393,#32394,#32395,#32396,#32397,#32398,#32399,#32400,#32401,#32402,
#32403,#32404,#32405,#32406,#32407),.UNSPECIFIED.,.F.,.F.,(4,1,1,1,1,1,
1,1,1,1,1,1,1,1,1,1,1,1,4),(2.78773030124088E-7,0.0625,0.09375,0.125,0.15625,
0.1875,0.25,0.3125,0.375,0.5,0.625,0.6875,0.75,0.8125,0.84375,0.875,0.90625,
0.9375,0.999999822301832),.UNSPECIFIED.);
#656=B_SPLINE_CURVE_WITH_KNOTS('',3,(#32409,#32410,#32411,#32412,#32413,
#32414,#32415,#32416,#32417,#32418,#32419,#32420,#32421,#32422,#32423,#32424,
#32425,#32426,#32427,#32428,#32429),.UNSPECIFIED.,.F.,.F.,(4,1,1,1,1,1,
1,1,1,1,1,1,1,1,1,1,1,1,4),(0.,0.0625,0.09375,0.125,0.15625,0.1875,0.25,
0.3125,0.375,0.5,0.625,0.6875,0.75,0.8125,0.84375,0.875,0.90625,0.9375,
1.),.UNSPECIFIED.);
#657=B_SPLINE_CURVE_WITH_KNOTS('',3,(#32433,#32434,#32435,#32436,#32437,
#32438,#32439,#32440,#32441,#32442,#32443,#32444,#32445,#32446,#32447,#32448,
#32449,#32450,#32451,#32452,#32453),.UNSPECIFIED.,.F.,.F.,(4,1,1,1,1,1,
1,1,1,1,1,1,1,1,1,1,1,1,4),(2.8501534152819E-7,0.0625,0.09375,0.125,0.15625,
0.1875,0.25,0.3125,0.375,0.5,0.625,0.6875,0.75,0.8125,0.84375,0.875,0.90625,
0.9375,1.),.UNSPECIFIED.);
#658=B_SPLINE_CURVE_WITH_KNOTS('',3,(#32454,#32455,#32456,#32457,#32458,
#32459,#32460,#32461,#32462,#32463,#32464,#32465,#32466,#32467,#32468,#32469,
#32470,#32471,#32472,#32473,#32474),.UNSPECIFIED.,.F.,.F.,(4,1,1,1,1,1,
1,1,1,1,1,1,1,1,1,1,1,1,4),(1.11184293768699E-8,0.0625,0.09375,0.125,0.15625,
0.1875,0.25,0.3125,0.375,0.5,0.625,0.6875,0.75,0.8125,0.84375,0.875,0.90625,
0.9375,0.999999806772229),.UNSPECIFIED.);
#659=B_SPLINE_CURVE_WITH_KNOTS('',3,(#32479,#32480,#32481,#32482,#32483,
#32484,#32485,#32486,#32487,#32488,#32489,#32490,#32491,#32492,#32493,#32494,
#32495,#32496,#32497,#32498,#32499),.UNSPECIFIED.,.F.,.F.,(4,1,1,1,1,1,
1,1,1,1,1,1,1,1,1,1,1,1,4),(2.82686142298943E-7,0.0625,0.09375,0.125,0.15625,
0.1875,0.25,0.3125,0.375,0.5,0.625,0.6875,0.75,0.8125,0.84375,0.875,0.90625,
0.9375,0.999999781697572),.UNSPECIFIED.);
#660=B_SPLINE_CURVE_WITH_KNOTS('',3,(#32501,#32502,#32503,#32504,#32505,
#32506,#32507,#32508,#32509,#32510,#32511,#32512,#32513,#32514,#32515,#32516,
#32517,#32518,#32519,#32520,#32521),.UNSPECIFIED.,.F.,.F.,(4,1,1,1,1,1,
1,1,1,1,1,1,1,1,1,1,1,1,4),(0.,0.0625,0.09375,0.125,0.15625,0.1875,0.25,
0.3125,0.375,0.5,0.625,0.6875,0.75,0.8125,0.84375,0.875,0.90625,0.9375,
1.),.UNSPECIFIED.);
#661=B_SPLINE_CURVE_WITH_KNOTS('',3,(#32525,#32526,#32527,#32528,#32529,
#32530,#32531,#32532,#32533,#32534,#32535,#32536,#32537,#32538,#32539,#32540,
#32541,#32542,#32543,#32544,#32545),.UNSPECIFIED.,.F.,.F.,(4,1,1,1,1,1,
1,1,1,1,1,1,1,1,1,1,1,1,4),(2.86446402154255E-7,0.0625,0.09375,0.125,0.15625,
0.1875,0.25,0.3125,0.375,0.5,0.625,0.6875,0.75,0.8125,0.84375,0.875,0.90625,
0.9375,1.),.UNSPECIFIED.);
#662=B_SPLINE_CURVE_WITH_KNOTS('',3,(#32546,#32547,#32548,#32549,#32550,
#32551,#32552,#32553,#32554,#32555,#32556,#32557,#32558,#32559,#32560,#32561,
#32562,#32563,#32564,#32565,#32566,#32567,#32568,#32569,#32570,#32571,#32572,
#32573,#32574,#32575,#32576,#32577,#32578,#32579,#32580,#32581,#32582,#32583,
#32584,#32585,#32586,#32587,#32588,#32589,#32590,#32591,#32592,#32593,#32594,
#32595,#32596,#32597,#32598,#32599,#32600,#32601,#32602,#32603),
 .UNSPECIFIED.,.F.,.F.,(4,3,3,3,3,3,3,3,3,3,3,3,3,3,3,3,3,3,3,4),(2.61184801452757E-8,
0.0625,0.09375,0.125,0.15625,0.1875,0.25,0.3125,0.375,0.5,0.625,0.647792304041325,
0.6875,0.75,0.8125,0.84375,0.875,0.90625,0.9375,0.999999815671741),
 .UNSPECIFIED.);
#663=B_SPLINE_CURVE_WITH_KNOTS('',3,(#32608,#32609,#32610,#32611,#32612,
#32613,#32614,#32615,#32616,#32617,#32618,#32619,#32620,#32621,#32622,#32623,
#32624,#32625,#32626,#32627,#32628),.UNSPECIFIED.,.F.,.F.,(4,1,1,1,1,1,
1,1,1,1,1,1,1,1,1,1,1,1,4),(2.84967473049237E-7,0.0625,0.09375,0.125,0.15625,
0.1875,0.25,0.3125,0.375,0.5,0.625,0.6875,0.75,0.8125,0.84375,0.875,0.90625,
0.9375,0.999999714401756),.UNSPECIFIED.);
#664=B_SPLINE_CURVE_WITH_KNOTS('',3,(#32630,#32631,#32632,#32633,#32634,
#32635,#32636,#32637,#32638,#32639,#32640,#32641,#32642,#32643,#32644,#32645,
#32646,#32647,#32648,#32649,#32650),.UNSPECIFIED.,.F.,.F.,(4,1,1,1,1,1,
1,1,1,1,1,1,1,1,1,1,1,1,4),(0.,0.0625,0.09375,0.125,0.15625,0.1875,0.25,
0.3125,0.375,0.5,0.625,0.6875,0.75,0.8125,0.84375,0.875,0.90625,0.9375,
1.),.UNSPECIFIED.);
#665=B_SPLINE_CURVE_WITH_KNOTS('',3,(#32654,#32655,#32656,#32657,#32658,
#32659,#32660,#32661,#32662,#32663,#32664,#32665,#32666,#32667,#32668,#32669,
#32670,#32671,#32672,#32673,#32674),.UNSPECIFIED.,.F.,.F.,(4,1,1,1,1,1,
1,1,1,1,1,1,1,1,1,1,1,1,4),(2.94403525435868E-7,0.0625,0.09375,0.125,0.15625,
0.1875,0.25,0.3125,0.375,0.5,0.625,0.6875,0.75,0.8125,0.84375,0.875,0.90625,
0.9375,1.),.UNSPECIFIED.);
#666=B_SPLINE_CURVE_WITH_KNOTS('',3,(#32675,#32676,#32677,#32678,#32679,
#32680,#32681,#32682,#32683,#32684,#32685,#32686,#32687,#32688,#32689,#32690,
#32691,#32692,#32693,#32694,#32695,#32696,#32697,#32698,#32699,#32700,#32701,
#32702,#32703,#32704,#32705,#32706,#32707,#32708,#32709,#32710,#32711,#32712,
#32713,#32714,#32715,#32716,#32717,#32718,#32719,#32720,#32721,#32722,#32723,
#32724,#32725,#32726,#32727,#32728,#32729,#32730,#32731,#32732),
 .UNSPECIFIED.,.F.,.F.,(4,3,3,3,3,3,3,3,3,3,3,3,3,3,3,3,3,3,3,4),(3.81813237642607E-8,
0.0625,0.09375,0.125,0.15625,0.1875,0.25,0.3125,0.375,0.5,0.625,0.649759799039456,
0.6875,0.75,0.8125,0.84375,0.875,0.90625,0.9375,0.999999823797946),
 .UNSPECIFIED.);
#667=B_SPLINE_CURVE_WITH_KNOTS('',3,(#32737,#32738,#32739,#32740,#32741,
#32742,#32743,#32744,#32745,#32746,#32747,#32748,#32749,#32750,#32751,#32752,
#32753,#32754,#32755),.UNSPECIFIED.,.F.,.F.,(4,1,1,1,1,1,1,1,1,1,1,1,1,
1,1,1,4),(2.60222887639683E-7,0.0625,0.09375,0.125,0.15625,0.1875,0.25,
0.375,0.5,0.625,0.6875,0.71875,0.75,0.78125,0.8125,0.875,0.999999892515785),
 .UNSPECIFIED.);
#668=B_SPLINE_CURVE_WITH_KNOTS('',3,(#32757,#32758,#32759,#32760,#32761,
#32762,#32763,#32764,#32765,#32766,#32767,#32768,#32769,#32770,#32771,#32772,
#32773,#32774,#32775),.UNSPECIFIED.,.F.,.F.,(4,1,1,1,1,1,1,1,1,1,1,1,1,
1,1,1,4),(0.,0.125,0.1875,0.21875,0.25,0.28125,0.3125,0.375,0.5,0.625,0.75,
0.8125,0.84375,0.875,0.90625,0.9375,1.),.UNSPECIFIED.);
#669=B_SPLINE_CURVE_WITH_KNOTS('',3,(#32779,#32780,#32781,#32782,#32783,
#32784,#32785,#32786,#32787,#32788,#32789,#32790,#32791,#32792,#32793,#32794,
#32795,#32796,#32797,#32798,#32799,#32800,#32801,#32802,#32803,#32804,#32805,
#32806,#32807,#32808,#32809,#32810,#32811,#32812,#32813,#32814,#32815,#32816,
#32817,#32818,#32819,#32820,#32821,#32822,#32823,#32824,#32825,#32826,#32827,
#32828,#32829,#32830),.UNSPECIFIED.,.F.,.F.,(4,3,3,3,3,3,3,3,3,3,3,3,3,
3,3,3,3,4),(2.63017244894725E-7,0.0625,0.09375,0.125,0.15625,0.1875,0.25,
0.367332392673666,0.375,0.5,0.625,0.6875,0.71875,0.75,0.78125,0.8125,0.875,
0.99999998868207),.UNSPECIFIED.);
#670=B_SPLINE_CURVE_WITH_KNOTS('',3,(#32831,#32832,#32833,#32834,#32835,
#32836,#32837,#32838,#32839,#32840,#32841,#32842,#32843,#32844,#32845,#32846,
#32847,#32848,#32849,#32850,#32851,#32852,#32853,#32854,#32855,#32856,#32857,
#32858,#32859,#32860,#32861,#32862,#32863,#32864,#32865,#32866,#32867,#32868,
#32869,#32870,#32871,#32872,#32873,#32874,#32875,#32876,#32877,#32878,#32879,
#32880,#32881,#32882),.UNSPECIFIED.,.F.,.F.,(4,3,3,3,3,3,3,3,3,3,3,3,3,
3,3,3,3,4),(0.,0.125,0.1875,0.21875,0.25,0.28125,0.3125,0.375,0.5,0.625,
0.633637925900044,0.75,0.8125,0.84375,0.875,0.90625,0.9375,0.99999982150407),
 .UNSPECIFIED.);
#671=B_SPLINE_CURVE_WITH_KNOTS('',3,(#32887,#32888,#32889,#32890,#32891,
#32892,#32893,#32894,#32895,#32896,#32897,#32898,#32899,#32900,#32901,#32902,
#32903,#32904,#32905,#32906,#32907),.UNSPECIFIED.,.F.,.F.,(4,1,1,1,1,1,
1,1,1,1,1,1,1,1,1,1,1,1,4),(2.76569125747373E-7,0.0625,0.09375,0.125,0.15625,
0.1875,0.25,0.3125,0.375,0.5,0.625,0.6875,0.75,0.8125,0.84375,0.875,0.90625,
0.9375,0.999999617070618),.UNSPECIFIED.);
#672=B_SPLINE_CURVE_WITH_KNOTS('',3,(#32909,#32910,#32911,#32912,#32913,
#32914,#32915,#32916,#32917,#32918,#32919,#32920,#32921,#32922,#32923,#32924,
#32925,#32926,#32927,#32928,#32929),.UNSPECIFIED.,.F.,.F.,(4,1,1,1,1,1,
1,1,1,1,1,1,1,1,1,1,1,1,4),(0.,0.0625,0.09375,0.125,0.15625,0.1875,0.25,
0.3125,0.375,0.5,0.625,0.6875,0.75,0.8125,0.84375,0.875,0.90625,0.9375,
1.),.UNSPECIFIED.);
#673=B_SPLINE_CURVE_WITH_KNOTS('',3,(#32933,#32934,#32935,#32936,#32937,
#32938,#32939,#32940,#32941,#32942,#32943,#32944,#32945,#32946,#32947,#32948,
#32949,#32950,#32951,#32952,#32953,#32954,#32955,#32956,#32957,#32958,#32959,
#32960,#32961,#32962,#32963,#32964,#32965,#32966,#32967,#32968,#32969,#32970,
#32971,#32972,#32973,#32974,#32975,#32976,#32977,#32978,#32979,#32980,#32981,
#32982,#32983,#32984,#32985,#32986,#32987,#32988,#32989,#32990),
 .UNSPECIFIED.,.F.,.F.,(4,3,3,3,3,3,3,3,3,3,3,3,3,3,3,3,3,3,3,4),(2.8836184248057E-7,
0.0625,0.09375,0.125,0.15625,0.1875,0.25,0.3125,0.34633842624939,0.375,
0.5,0.625,0.6875,0.75,0.8125,0.84375,0.875,0.90625,0.9375,1.),
 .UNSPECIFIED.);
#674=B_SPLINE_CURVE_WITH_KNOTS('',3,(#32991,#32992,#32993,#32994,#32995,
#32996,#32997,#32998,#32999,#33000,#33001,#33002,#33003,#33004,#33005,#33006,
#33007,#33008,#33009,#33010,#33011,#33012,#33013,#33014,#33015,#33016,#33017,
#33018,#33019,#33020,#33021,#33022,#33023,#33024,#33025,#33026,#33027,#33028,
#33029,#33030,#33031,#33032,#33033,#33034,#33035,#33036,#33037,#33038,#33039,
#33040,#33041,#33042,#33043,#33044,#33045,#33046,#33047,#33048),
 .UNSPECIFIED.,.F.,.F.,(4,3,3,3,3,3,3,3,3,3,3,3,3,3,3,3,3,3,3,4),(8.75906255719806E-8,
0.0625,0.09375,0.125,0.15625,0.1875,0.25,0.3125,0.375,0.5,0.625,0.653697969502116,
0.6875,0.75,0.8125,0.84375,0.875,0.90625,0.9375,0.999999836937693),
 .UNSPECIFIED.);
#675=B_SPLINE_CURVE_WITH_KNOTS('',3,(#33053,#33054,#33055,#33056,#33057,
#33058,#33059,#33060,#33061,#33062,#33063,#33064),.UNSPECIFIED.,.F.,.F.,
(4,1,1,1,1,1,1,1,1,4),(0.,0.0625,0.09375,0.125,0.15625,0.1875,0.25,0.3125,
0.375,0.5),.UNSPECIFIED.);
#676=B_SPLINE_CURVE_WITH_KNOTS('',3,(#33066,#33067,#33068,#33069,#33070,
#33071,#33072,#33073,#33074,#33075,#33076),.UNSPECIFIED.,.F.,.F.,(4,1,1,
1,1,1,1,1,4),(0.5,0.625,0.75,0.8125,0.84375,0.875,0.90625,0.9375,1.),
 .UNSPECIFIED.);
#677=B_SPLINE_CURVE_WITH_KNOTS('',3,(#33078,#33079,#33080,#33081,#33082,
#33083,#33084,#33085,#33086,#33087,#33088),.UNSPECIFIED.,.F.,.F.,(4,1,1,
1,1,1,1,1,4),(7.15869646362667E-6,0.0625,0.09375,0.125,0.15625,0.1875,0.25,
0.375,0.499318743160308),.UNSPECIFIED.);
#678=B_SPLINE_CURVE_WITH_KNOTS('',3,(#33090,#33091,#33092,#33093,#33094,
#33095,#33096,#33097,#33098,#33099,#33100,#33101,#33102),.UNSPECIFIED.,
 .F.,.F.,(4,1,1,1,1,1,1,1,1,1,4),(0.499318743160308,0.5,0.625,0.6875,0.75,
0.8125,0.84375,0.875,0.90625,0.9375,1.),.UNSPECIFIED.);
#679=B_SPLINE_CURVE_WITH_KNOTS('',3,(#33106,#33107,#33108,#33109,#33110,
#33111,#33112,#33113,#33114,#33115,#33116,#33117),.UNSPECIFIED.,.F.,.F.,
(4,1,1,1,1,1,1,1,1,4),(0.,0.0625,0.09375,0.125,0.15625,0.1875,0.25,0.3125,
0.375,0.5),.UNSPECIFIED.);
#680=B_SPLINE_CURVE_WITH_KNOTS('',3,(#33119,#33120,#33121,#33122,#33123,
#33124,#33125,#33126,#33127,#33128,#33129),.UNSPECIFIED.,.F.,.F.,(4,1,1,
1,1,1,1,1,4),(0.5,0.625,0.75,0.8125,0.84375,0.875,0.90625,0.9375,1.),
 .UNSPECIFIED.);
#681=B_SPLINE_CURVE_WITH_KNOTS('',3,(#33131,#33132,#33133,#33134,#33135,
#33136,#33137,#33138,#33139,#33140,#33141),.UNSPECIFIED.,.F.,.F.,(4,1,1,
1,1,1,1,1,4),(2.21677758325209E-7,0.0625,0.09375,0.125,0.15625,0.1875,0.25,
0.375,0.499882005198117),.UNSPECIFIED.);
#682=B_SPLINE_CURVE_WITH_KNOTS('',3,(#33142,#33143,#33144,#33145,#33146,
#33147,#33148,#33149,#33150,#33151,#33152,#33153),.UNSPECIFIED.,.F.,.F.,
(4,1,1,1,1,1,1,1,1,4),(0.5,0.625,0.6875,0.75,0.8125,0.84375,0.875,0.90625,
0.9375,0.999977373123454),.UNSPECIFIED.);
#683=B_SPLINE_CURVE_WITH_KNOTS('',3,(#33158,#33159,#33160,#33161,#33162,
#33163,#33164,#33165,#33166,#33167,#33168,#33169,#33170,#33171,#33172,#33173,
#33174,#33175,#33176,#33177,#33178),.UNSPECIFIED.,.F.,.F.,(4,1,1,1,1,1,
1,1,1,1,1,1,1,1,1,1,1,1,4),(2.84936194355119E-7,0.0625,0.09375,0.125,0.15625,
0.1875,0.25,0.3125,0.375,0.5,0.625,0.6875,0.75,0.8125,0.84375,0.875,0.90625,
0.9375,0.999999655061917),.UNSPECIFIED.);
#684=B_SPLINE_CURVE_WITH_KNOTS('',3,(#33180,#33181,#33182,#33183,#33184,
#33185,#33186,#33187,#33188,#33189,#33190,#33191,#33192,#33193,#33194,#33195,
#33196,#33197,#33198,#33199,#33200),.UNSPECIFIED.,.F.,.F.,(4,1,1,1,1,1,
1,1,1,1,1,1,1,1,1,1,1,1,4),(0.,0.0625,0.09375,0.125,0.15625,0.1875,0.25,
0.3125,0.375,0.5,0.625,0.6875,0.75,0.8125,0.84375,0.875,0.90625,0.9375,
1.),.UNSPECIFIED.);
#685=B_SPLINE_CURVE_WITH_KNOTS('',3,(#33204,#33205,#33206,#33207,#33208,
#33209,#33210,#33211,#33212,#33213,#33214,#33215,#33216,#33217,#33218,#33219,
#33220,#33221,#33222,#33223,#33224,#33225,#33226,#33227,#33228,#33229,#33230,
#33231,#33232,#33233,#33234,#33235,#33236,#33237,#33238,#33239,#33240,#33241,
#33242,#33243,#33244,#33245,#33246,#33247,#33248,#33249,#33250,#33251,#33252,
#33253,#33254,#33255,#33256,#33257,#33258,#33259,#33260,#33261),
 .UNSPECIFIED.,.F.,.F.,(4,3,3,3,3,3,3,3,3,3,3,3,3,3,3,3,3,3,3,4),(3.05273049617562E-7,
0.0625,0.09375,0.125,0.15625,0.1875,0.25,0.3125,0.348322390156725,0.375,
0.5,0.625,0.6875,0.75,0.8125,0.84375,0.875,0.90625,0.9375,1.),
 .UNSPECIFIED.);
#686=B_SPLINE_CURVE_WITH_KNOTS('',3,(#33262,#33263,#33264,#33265,#33266,
#33267,#33268,#33269,#33270,#33271,#33272,#33273,#33274,#33275,#33276,#33277,
#33278,#33279,#33280,#33281,#33282,#33283,#33284,#33285,#33286,#33287,#33288,
#33289,#33290,#33291,#33292,#33293,#33294,#33295,#33296,#33297,#33298,#33299,
#33300,#33301,#33302,#33303,#33304,#33305,#33306,#33307,#33308,#33309,#33310,
#33311,#33312,#33313,#33314,#33315,#33316,#33317,#33318,#33319),
 .UNSPECIFIED.,.F.,.F.,(4,3,3,3,3,3,3,3,3,3,3,3,3,3,3,3,3,3,3,4),(6.62097895526065E-8,
0.0625,0.09375,0.125,0.15625,0.1875,0.25,0.3125,0.375,0.5,0.625,0.651832350452469,
0.6875,0.75,0.8125,0.84375,0.875,0.90625,0.9375,0.9999998312716),
 .UNSPECIFIED.);
#687=B_SPLINE_CURVE_WITH_KNOTS('',3,(#33324,#33325,#33326,#33327,#33328,
#33329,#33330,#33331,#33332,#33333,#33334,#33335,#33336,#33337,#33338,#33339,
#33340,#33341,#33342),.UNSPECIFIED.,.F.,.F.,(4,1,1,1,1,1,1,1,1,1,1,1,1,
1,1,1,4),(2.75587839344889E-7,0.0625,0.09375,0.125,0.15625,0.1875,0.25,
0.375,0.5,0.625,0.6875,0.71875,0.75,0.78125,0.8125,0.875,0.999999959370797),
 .UNSPECIFIED.);
#688=B_SPLINE_CURVE_WITH_KNOTS('',3,(#33344,#33345,#33346,#33347,#33348,
#33349,#33350,#33351,#33352,#33353,#33354,#33355,#33356,#33357,#33358,#33359,
#33360,#33361,#33362),.UNSPECIFIED.,.F.,.F.,(4,1,1,1,1,1,1,1,1,1,1,1,1,
1,1,1,4),(0.,0.125,0.1875,0.21875,0.25,0.28125,0.3125,0.375,0.5,0.625,0.75,
0.8125,0.84375,0.875,0.90625,0.9375,1.),.UNSPECIFIED.);
#689=B_SPLINE_CURVE_WITH_KNOTS('',3,(#33366,#33367,#33368,#33369,#33370,
#33371,#33372,#33373,#33374,#33375,#33376,#33377,#33378,#33379,#33380,#33381,
#33382,#33383,#33384,#33385,#33386,#33387,#33388,#33389,#33390,#33391,#33392,
#33393,#33394,#33395,#33396,#33397,#33398,#33399,#33400,#33401,#33402,#33403,
#33404,#33405,#33406,#33407,#33408,#33409,#33410,#33411,#33412,#33413,#33414,
#33415,#33416,#33417),.UNSPECIFIED.,.F.,.F.,(4,3,3,3,3,3,3,3,3,3,3,3,3,
3,3,3,3,4),(2.808774569524E-7,0.0625,0.09375,0.125,0.15625,0.1875,0.25,
0.35969017869594,0.375,0.5,0.625,0.6875,0.71875,0.75,0.78125,0.8125,0.875,
1.),.UNSPECIFIED.);
#690=B_SPLINE_CURVE_WITH_KNOTS('',3,(#33418,#33419,#33420,#33421,#33422,
#33423,#33424,#33425,#33426,#33427,#33428,#33429,#33430,#33431,#33432,#33433,
#33434,#33435,#33436,#33437,#33438,#33439,#33440,#33441,#33442,#33443,#33444,
#33445,#33446,#33447,#33448,#33449,#33450,#33451,#33452,#33453,#33454,#33455,
#33456,#33457,#33458,#33459,#33460,#33461,#33462,#33463,#33464,#33465,#33466,
#33467,#33468,#33469),.UNSPECIFIED.,.F.,.F.,(4,3,3,3,3,3,3,3,3,3,3,3,3,
3,3,3,3,4),(3.41422460553818E-8,0.125,0.1875,0.21875,0.25,0.28125,0.3125,
0.375,0.5,0.625,0.641077554901531,0.75,0.8125,0.84375,0.875,0.90625,0.9375,
0.999999822593873),.UNSPECIFIED.);
#691=B_SPLINE_CURVE_WITH_KNOTS('',3,(#33474,#33475,#33476,#33477,#33478,
#33479,#33480,#33481,#33482,#33483,#33484,#33485,#33486,#33487,#33488,#33489,
#33490,#33491,#33492),.UNSPECIFIED.,.F.,.F.,(4,1,1,1,1,1,1,1,1,1,1,1,1,
1,1,1,4),(2.80445484236532E-7,0.0625,0.09375,0.125,0.15625,0.1875,0.25,
0.375,0.5,0.625,0.6875,0.71875,0.75,0.78125,0.8125,0.875,0.999999987809309),
 .UNSPECIFIED.);
#692=B_SPLINE_CURVE_WITH_KNOTS('',3,(#33494,#33495,#33496,#33497,#33498,
#33499,#33500,#33501,#33502,#33503,#33504,#33505,#33506,#33507,#33508,#33509,
#33510,#33511,#33512),.UNSPECIFIED.,.F.,.F.,(4,1,1,1,1,1,1,1,1,1,1,1,1,
1,1,1,4),(0.,0.125,0.1875,0.21875,0.25,0.28125,0.3125,0.375,0.5,0.625,0.75,
0.8125,0.84375,0.875,0.90625,0.9375,1.),.UNSPECIFIED.);
#693=B_SPLINE_CURVE_WITH_KNOTS('',3,(#33516,#33517,#33518,#33519,#33520,
#33521,#33522,#33523,#33524,#33525,#33526,#33527,#33528,#33529,#33530,#33531,
#33532,#33533,#33534,#33535,#33536,#33537,#33538,#33539,#33540,#33541,#33542,
#33543,#33544,#33545,#33546,#33547,#33548,#33549,#33550,#33551,#33552,#33553,
#33554,#33555,#33556,#33557,#33558,#33559,#33560,#33561,#33562,#33563,#33564,
#33565,#33566,#33567),.UNSPECIFIED.,.F.,.F.,(4,3,3,3,3,3,3,3,3,3,3,3,3,
3,3,3,3,4),(2.77199665841602E-7,0.0625,0.09375,0.125,0.15625,0.1875,0.25,
0.361636464506202,0.375,0.5,0.625,0.6875,0.71875,0.75,0.78125,0.8125,0.875,
1.),.UNSPECIFIED.);
#694=B_SPLINE_CURVE_WITH_KNOTS('',3,(#33568,#33569,#33570,#33571,#33572,
#33573,#33574,#33575,#33576,#33577,#33578,#33579,#33580,#33581,#33582,#33583,
#33584,#33585,#33586,#33587,#33588,#33589,#33590,#33591,#33592,#33593,#33594,
#33595,#33596,#33597,#33598,#33599,#33600,#33601,#33602,#33603,#33604,#33605,
#33606,#33607,#33608,#33609,#33610,#33611,#33612,#33613,#33614,#33615,#33616,
#33617,#33618,#33619),.UNSPECIFIED.,.F.,.F.,(4,3,3,3,3,3,3,3,3,3,3,3,3,
3,3,3,3,4),(6.91571290081694E-8,0.125,0.1875,0.21875,0.25,0.28125,0.3125,
0.375,0.5,0.625,0.639335759650785,0.75,0.8125,0.84375,0.875,0.90625,0.9375,
0.999999825283333),.UNSPECIFIED.);
#695=B_SPLINE_CURVE_WITH_KNOTS('',3,(#33624,#33625,#33626,#33627,#33628,
#33629,#33630,#33631,#33632,#33633,#33634,#33635,#33636,#33637,#33638,#33639,
#33640,#33641,#33642),.UNSPECIFIED.,.F.,.F.,(4,1,1,1,1,1,1,1,1,1,1,1,1,
1,1,1,4),(2.6847278418118E-7,0.0625,0.09375,0.125,0.15625,0.1875,0.25,0.375,
0.5,0.625,0.6875,0.71875,0.75,0.78125,0.8125,0.875,1.),.UNSPECIFIED.);
#696=B_SPLINE_CURVE_WITH_KNOTS('',3,(#33644,#33645,#33646,#33647,#33648,
#33649,#33650,#33651,#33652,#33653,#33654,#33655,#33656,#33657,#33658,#33659,
#33660,#33661,#33662),.UNSPECIFIED.,.F.,.F.,(4,1,1,1,1,1,1,1,1,1,1,1,1,
1,1,1,4),(1.72418419787525E-8,0.125,0.1875,0.21875,0.25,0.28125,0.3125,
0.375,0.5,0.625,0.75,0.8125,0.84375,0.875,0.90625,0.9375,1.),
 .UNSPECIFIED.);
#697=B_SPLINE_CURVE_WITH_KNOTS('',3,(#33666,#33667,#33668,#33669,#33670,
#33671,#33672,#33673,#33674,#33675,#33676,#33677,#33678,#33679,#33680,#33681,
#33682,#33683,#33684,#33685,#33686,#33687,#33688,#33689,#33690,#33691,#33692,
#33693,#33694,#33695,#33696,#33697,#33698,#33699,#33700,#33701,#33702,#33703,
#33704,#33705,#33706,#33707,#33708,#33709,#33710,#33711,#33712,#33713,#33714,
#33715,#33716,#33717),.UNSPECIFIED.,.F.,.F.,(4,3,3,3,3,3,3,3,3,3,3,3,3,
3,3,3,3,4),(2.74314204166858E-7,0.0625,0.09375,0.125,0.15625,0.1875,0.25,
0.36358849545573,0.375,0.5,0.625,0.6875,0.71875,0.75,0.78125,0.8125,0.875,
1.),.UNSPECIFIED.);
#698=B_SPLINE_CURVE_WITH_KNOTS('',3,(#33718,#33719,#33720,#33721,#33722,
#33723,#33724,#33725,#33726,#33727,#33728,#33729,#33730,#33731,#33732,#33733,
#33734,#33735,#33736,#33737,#33738,#33739,#33740,#33741,#33742,#33743,#33744,
#33745,#33746,#33747,#33748,#33749,#33750,#33751,#33752,#33753,#33754,#33755,
#33756,#33757,#33758,#33759,#33760,#33761,#33762,#33763,#33764,#33765,#33766,
#33767,#33768,#33769),.UNSPECIFIED.,.F.,.F.,(4,3,3,3,3,3,3,3,3,3,3,3,3,
3,3,3,3,4),(7.63260218006573E-8,0.125,0.1875,0.21875,0.25,0.28125,0.3125,
0.375,0.5,0.625,0.637553797507691,0.75,0.8125,0.84375,0.875,0.90625,0.9375,
0.999999824822769),.UNSPECIFIED.);
#699=B_SPLINE_CURVE_WITH_KNOTS('',3,(#33774,#33775,#33776,#33777,#33778,
#33779,#33780,#33781,#33782,#33783,#33784,#33785,#33786,#33787,#33788,#33789,
#33790,#33791,#33792),.UNSPECIFIED.,.F.,.F.,(4,1,1,1,1,1,1,1,1,1,1,1,1,
1,1,1,4),(0.,0.0625,0.09375,0.125,0.15625,0.1875,0.25,0.375,0.5,0.625,0.6875,
0.71875,0.75,0.78125,0.8125,0.875,1.),.UNSPECIFIED.);
#700=B_SPLINE_CURVE_WITH_KNOTS('',3,(#33794,#33795,#33796,#33797,#33798,
#33799,#33800,#33801,#33802,#33803,#33804,#33805,#33806,#33807,#33808,#33809,
#33810,#33811,#33812),.UNSPECIFIED.,.F.,.F.,(4,1,1,1,1,1,1,1,1,1,1,1,1,
1,1,1,4),(2.65886426353366E-9,0.125,0.1875,0.21875,0.25,0.28125,0.3125,
0.375,0.5,0.625,0.75,0.8125,0.84375,0.875,0.90625,0.9375,1.),
 .UNSPECIFIED.);
#701=B_SPLINE_CURVE_WITH_KNOTS('',3,(#33816,#33817,#33818,#33819,#33820,
#33821,#33822,#33823,#33824,#33825,#33826,#33827,#33828,#33829,#33830,#33831,
#33832,#33833,#33834,#33835,#33836,#33837,#33838,#33839,#33840,#33841,#33842,
#33843,#33844,#33845,#33846,#33847,#33848,#33849,#33850,#33851,#33852,#33853,
#33854,#33855,#33856,#33857,#33858,#33859,#33860,#33861,#33862,#33863,#33864,
#33865,#33866,#33867),.UNSPECIFIED.,.F.,.F.,(4,3,3,3,3,3,3,3,3,3,3,3,3,
3,3,3,3,4),(2.63361468193179E-7,0.0625,0.09375,0.125,0.15625,0.1875,0.25,
0.365500799027569,0.375,0.5,0.625,0.6875,0.71875,0.75,0.78125,0.8125,0.875,
0.99999997625737),.UNSPECIFIED.);
#702=B_SPLINE_CURVE_WITH_KNOTS('',3,(#33868,#33869,#33870,#33871,#33872,
#33873,#33874,#33875,#33876,#33877,#33878,#33879,#33880,#33881,#33882,#33883,
#33884,#33885,#33886,#33887,#33888,#33889,#33890,#33891,#33892,#33893,#33894,
#33895,#33896,#33897,#33898,#33899,#33900,#33901,#33902,#33903,#33904,#33905,
#33906,#33907,#33908,#33909,#33910,#33911,#33912,#33913,#33914,#33915,#33916,
#33917,#33918,#33919),.UNSPECIFIED.,.F.,.F.,(4,3,3,3,3,3,3,3,3,3,3,3,3,
3,3,3,3,4),(0.,0.125,0.1875,0.21875,0.25,0.28125,0.3125,0.375,0.5,0.625,
0.635593203482249,0.75,0.8125,0.84375,0.875,0.90625,0.9375,0.999999822175548),
 .UNSPECIFIED.);
#703=B_SPLINE_CURVE_WITH_KNOTS('',3,(#33924,#33925,#33926,#33927,#33928,
#33929,#33930,#33931,#33932,#33933,#33934,#33935),.UNSPECIFIED.,.F.,.F.,
(4,1,1,1,1,1,1,1,1,4),(0.,0.0625,0.09375,0.125,0.15625,0.1875,0.25,0.3125,
0.375,0.5),.UNSPECIFIED.);
#704=B_SPLINE_CURVE_WITH_KNOTS('',3,(#33937,#33938,#33939,#33940,#33941,
#33942,#33943,#33944,#33945,#33946,#33947),.UNSPECIFIED.,.F.,.F.,(4,1,1,
1,1,1,1,1,4),(0.5,0.625,0.75,0.8125,0.84375,0.875,0.90625,0.9375,1.),
 .UNSPECIFIED.);
#705=B_SPLINE_CURVE_WITH_KNOTS('',3,(#33949,#33950,#33951,#33952,#33953,
#33954,#33955,#33956,#33957,#33958,#33959),.UNSPECIFIED.,.F.,.F.,(4,1,1,
1,1,1,1,1,4),(6.38525460793569E-6,0.0625,0.09375,0.125,0.15625,0.1875,0.25,
0.375,0.499319982454846),.UNSPECIFIED.);
#706=B_SPLINE_CURVE_WITH_KNOTS('',3,(#33961,#33962,#33963,#33964,#33965,
#33966,#33967,#33968,#33969,#33970,#33971,#33972,#33973),.UNSPECIFIED.,
 .F.,.F.,(4,1,1,1,1,1,1,1,1,1,4),(0.499319982454846,0.5,0.625,0.6875,0.75,
0.8125,0.84375,0.875,0.90625,0.9375,1.),.UNSPECIFIED.);
#707=B_SPLINE_CURVE_WITH_KNOTS('',3,(#33977,#33978,#33979,#33980,#33981,
#33982,#33983,#33984,#33985,#33986,#33987,#33988),.UNSPECIFIED.,.F.,.F.,
(4,1,1,1,1,1,1,1,1,4),(0.,0.0625,0.09375,0.125,0.15625,0.1875,0.25,0.3125,
0.375,0.5),.UNSPECIFIED.);
#708=B_SPLINE_CURVE_WITH_KNOTS('',3,(#33990,#33991,#33992,#33993,#33994,
#33995,#33996,#33997,#33998,#33999,#34000),.UNSPECIFIED.,.F.,.F.,(4,1,1,
1,1,1,1,1,4),(0.5,0.625,0.75,0.8125,0.84375,0.875,0.90625,0.9375,1.),
 .UNSPECIFIED.);
#709=B_SPLINE_CURVE_WITH_KNOTS('',3,(#34002,#34003,#34004,#34005,#34006,
#34007,#34008,#34009,#34010,#34011,#34012),.UNSPECIFIED.,.F.,.F.,(4,1,1,
1,1,1,1,1,4),(2.4708654656939E-7,0.0625,0.09375,0.125,0.15625,0.1875,0.25,
0.375,0.499884707955717),.UNSPECIFIED.);
#710=B_SPLINE_CURVE_WITH_KNOTS('',3,(#34013,#34014,#34015,#34016,#34017,
#34018,#34019,#34020,#34021,#34022,#34023,#34024),.UNSPECIFIED.,.F.,.F.,
(4,1,1,1,1,1,1,1,1,4),(0.5,0.625,0.6875,0.75,0.8125,0.84375,0.875,0.90625,
0.9375,0.999978109235681),.UNSPECIFIED.);
#711=B_SPLINE_CURVE_WITH_KNOTS('',3,(#34027,#34028,#34029,#34030,#34031,
#34032,#34033,#34034,#34035,#34036,#34037,#34038,#34039,#34040,#34041,#34042,
#34043,#34044,#34045,#34046,#34047,#34048,#34049,#34050,#34051,#34052,#34053,
#34054,#34055,#34056,#34057),.UNSPECIFIED.,.F.,.F.,(4,3,3,3,3,3,3,3,3,3,
4),(0.000176563406958893,0.125,0.1875,0.25,0.3125,0.375,0.5,0.625,0.75,
0.875,0.999998995305369),.UNSPECIFIED.);
#712=B_SPLINE_CURVE_WITH_KNOTS('',3,(#34059,#34060,#34061,#34062,#34063,
#34064,#34065,#34066,#34067,#34068,#34069,#34070,#34071),.UNSPECIFIED.,
 .F.,.F.,(4,1,1,1,1,1,1,1,1,1,4),(1.66911490650295E-8,0.0625,0.09375,0.125,
0.15625,0.1875,0.25,0.3125,0.375,0.5,0.500683333035046),.UNSPECIFIED.);
#713=B_SPLINE_CURVE_WITH_KNOTS('',3,(#34073,#34074,#34075,#34076,#34077,
#34078,#34079,#34080,#34081,#34082,#34083),.UNSPECIFIED.,.F.,.F.,(4,1,1,
1,1,1,1,1,4),(0.500683333035046,0.625,0.75,0.8125,0.84375,0.875,0.90625,
0.9375,0.999999813866294),.UNSPECIFIED.);
#714=B_SPLINE_CURVE_WITH_KNOTS('',3,(#34085,#34086,#34087,#34088,#34089,
#34090,#34091,#34092,#34093,#34094,#34095),.UNSPECIFIED.,.F.,.F.,(4,1,1,
1,1,1,1,1,4),(0.,0.0625,0.09375,0.125,0.15625,0.1875,0.25,0.375,0.499405889061093),
 .UNSPECIFIED.);
#715=B_SPLINE_CURVE_WITH_KNOTS('',3,(#34097,#34098,#34099,#34100,#34101,
#34102,#34103,#34104,#34105,#34106,#34107,#34108),.UNSPECIFIED.,.F.,.F.,
(4,1,1,1,1,1,1,1,1,4),(0.499405889061093,0.5,0.625,0.75,0.8125,0.84375,
0.875,0.90625,0.9375,1.),.UNSPECIFIED.);
#716=B_SPLINE_CURVE_WITH_KNOTS('',3,(#34110,#34111,#34112,#34113,#34114,
#34115,#34116,#34117,#34118,#34119,#34120,#34121,#34122,#34123,#34124,#34125,
#34126,#34127,#34128,#34129,#34130,#34131,#34132,#34133,#34134,#34135,#34136,
#34137,#34138,#34139,#34140),.UNSPECIFIED.,.F.,.F.,(4,3,3,3,3,3,3,3,3,3,
4),(3.42300885912184E-6,0.125,0.25,0.375,0.5,0.625,0.75,0.8125,0.875,0.9375,
0.999842771045948),.UNSPECIFIED.);
#717=B_SPLINE_CURVE_WITH_KNOTS('',3,(#34142,#34143,#34144,#34145,#34146,
#34147,#34148,#34149,#34150,#34151,#34152,#34153),.UNSPECIFIED.,.F.,.F.,
(4,1,1,1,1,1,1,1,1,4),(0.,0.0625,0.09375,0.125,0.15625,0.1875,0.25,0.3125,
0.375,0.461683849721955),.UNSPECIFIED.);
#718=B_SPLINE_CURVE_WITH_KNOTS('',3,(#34155,#34156,#34157,#34158,#34159,
#34160,#34161,#34162,#34163,#34164,#34165,#34166),.UNSPECIFIED.,.F.,.F.,
(4,1,1,1,1,1,1,1,1,4),(0.461683849721955,0.5,0.625,0.75,0.8125,0.84375,
0.875,0.90625,0.9375,1.),.UNSPECIFIED.);
#719=B_SPLINE_CURVE_WITH_KNOTS('',3,(#34168,#34169,#34170,#34171,#34172,
#34173,#34174,#34175,#34176,#34177,#34178),.UNSPECIFIED.,.F.,.F.,(4,1,1,
1,1,1,1,1,4),(2.44966122427333E-7,0.0625,0.09375,0.125,0.15625,0.1875,0.25,
0.375,0.499887143451556),.UNSPECIFIED.);
#720=B_SPLINE_CURVE_WITH_KNOTS('',3,(#34179,#34180,#34181,#34182,#34183,
#34184,#34185,#34186,#34187,#34188,#34189,#34190),.UNSPECIFIED.,.F.,.F.,
(4,1,1,1,1,1,1,1,1,4),(0.5,0.625,0.6875,0.75,0.8125,0.84375,0.875,0.90625,
0.9375,0.999988315055417),.UNSPECIFIED.);
#721=B_SPLINE_CURVE_WITH_KNOTS('',3,(#34193,#34194,#34195,#34196,#34197,
#34198,#34199,#34200,#34201),.UNSPECIFIED.,.F.,.F.,(4,1,1,1,1,1,4),(0.00162491627968111,
0.125,0.1875,0.25,0.3125,0.375,0.499422005584456),.UNSPECIFIED.);
#722=B_SPLINE_CURVE_WITH_KNOTS('',3,(#34203,#34204,#34205,#34206,#34207,
#34208,#34209,#34210),.UNSPECIFIED.,.F.,.F.,(4,1,1,1,1,4),(0.5,0.625,0.75,
0.875,0.9375,1.),.UNSPECIFIED.);
#723=B_SPLINE_CURVE_WITH_KNOTS('',3,(#34212,#34213,#34214,#34215,#34216,
#34217,#34218,#34219,#34220,#34221,#34222,#34223,#34224,#34225,#34226,#34227,
#34228,#34229,#34230,#34231,#34232,#34233,#34234,#34235,#34236,#34237,#34238,
#34239,#34240,#34241,#34242),.UNSPECIFIED.,.F.,.F.,(4,3,3,3,3,3,3,3,3,3,
4),(2.03685100085616E-6,0.0625,0.09375,0.125,0.15625,0.1875,0.25,0.373077890397942,
0.375,0.5,0.500627296921563),.UNSPECIFIED.);
#724=B_SPLINE_CURVE_WITH_KNOTS('',3,(#34244,#34245,#34246,#34247,#34248,
#34249,#34250,#34251,#34252,#34253,#34254,#34255,#34256,#34257,#34258,#34259,
#34260,#34261,#34262,#34263,#34264,#34265,#34266,#34267,#34268),
 .UNSPECIFIED.,.F.,.F.,(4,3,3,3,3,3,3,3,4),(0.500627296921563,0.625,0.6875,
0.71875,0.75,0.78125,0.8125,0.875,0.999999762981869),.UNSPECIFIED.);
#725=B_SPLINE_CURVE_WITH_KNOTS('',3,(#34270,#34271,#34272,#34273,#34274,
#34275,#34276,#34277,#34278,#34279,#34280,#34281,#34282,#34283,#34284,#34285,
#34286,#34287,#34288,#34289,#34290,#34291,#34292,#34293,#34294,#34295,#34296,
#34297),.UNSPECIFIED.,.F.,.F.,(4,3,3,3,3,3,3,3,3,4),(0.,0.125,0.1875,0.21875,
0.25,0.28125,0.3125,0.375,0.5,0.500193349382862),.UNSPECIFIED.);
#726=B_SPLINE_CURVE_WITH_KNOTS('',3,(#34299,#34300,#34301,#34302,#34303,
#34304,#34305,#34306,#34307,#34308,#34309,#34310,#34311,#34312,#34313,#34314,
#34315,#34316,#34317,#34318,#34319,#34320,#34321,#34322,#34323),
 .UNSPECIFIED.,.F.,.F.,(4,3,3,3,3,3,3,3,4),(0.500193349382862,0.625,0.75,
0.8125,0.84375,0.875,0.90625,0.9375,1.),.UNSPECIFIED.);
#727=B_SPLINE_CURVE_WITH_KNOTS('',3,(#34325,#34326,#34327,#34328,#34329,
#34330,#34331,#34332,#34333,#34334,#34335,#34336,#34337,#34338,#34339,#34340,
#34341,#34342,#34343,#34344,#34345,#34346,#34347,#34348,#34349,#34350,#34351,
#34352),.UNSPECIFIED.,.F.,.F.,(4,3,3,3,3,3,3,3,3,4),(3.81246354337078E-6,
0.125,0.25,0.375,0.5,0.625,0.75,0.875,0.9375,0.999998611687521),
 .UNSPECIFIED.);
#728=B_SPLINE_CURVE_WITH_KNOTS('',3,(#34354,#34355,#34356,#34357,#34358,
#34359,#34360,#34361,#34362,#34363,#34364,#34365,#34366,#34367,#34368,#34369,
#34370,#34371,#34372),.UNSPECIFIED.,.F.,.F.,(4,1,1,1,1,1,1,1,1,1,1,1,1,
1,1,1,4),(0.,0.0625,0.09375,0.125,0.15625,0.1875,0.25,0.375,0.5,0.625,0.75,
0.8125,0.84375,0.875,0.90625,0.9375,1.),.UNSPECIFIED.);
#729=B_SPLINE_CURVE_WITH_KNOTS('',3,(#34374,#34375,#34376,#34377),
 .UNSPECIFIED.,.F.,.F.,(4,4),(0.951680478228109,0.999996857021366),
 .UNSPECIFIED.);
#730=B_SPLINE_CURVE_WITH_KNOTS('',3,(#34379,#34380,#34381,#34382,#34383,
#34384,#34385,#34386,#34387,#34388,#34389,#34390,#34391,#34392,#34393,#34394,
#34395,#34396,#34397,#34398,#34399,#34400,#34401,#34402,#34403,#34404,#34405,
#34406),.UNSPECIFIED.,.F.,.F.,(4,3,3,3,3,3,3,3,3,4),(0.583516228419036,
0.59375,0.625,0.6875,0.71875,0.75,0.78125,0.8125,0.875,0.951680478228109),
 .UNSPECIFIED.);
#731=B_SPLINE_CURVE_WITH_KNOTS('',3,(#34408,#34409,#34410,#34411,#34412,
#34413,#34414,#34415,#34416,#34417,#34418,#34419,#34420,#34421,#34422,#34423,
#34424,#34425,#34426,#34427,#34428,#34429,#34430,#34431,#34432,#34433,#34434,
#34435,#34436,#34437,#34438,#34439,#34440,#34441,#34442,#34443,#34444,#34445,
#34446,#34447,#34448,#34449,#34450,#34451,#34452,#34453,#34454,#34455,#34456,
#34457,#34458,#34459,#34460,#34461,#34462,#34463,#34464,#34465),
 .UNSPECIFIED.,.F.,.F.,(4,3,3,3,3,3,3,3,3,3,3,3,3,3,3,3,3,3,3,4),(0.1328125,
0.140625,0.15625,0.171875,0.1875,0.203125,0.21875,0.25,0.28125,0.3125,0.375,
0.435752721141823,0.4375,0.46875,0.484375,0.5,0.515625,0.53125,0.5625,0.583516228419036),
 .UNSPECIFIED.);
#732=B_SPLINE_CURVE_WITH_KNOTS('',3,(#34466,#34467,#34468,#34469,#34470,
#34471,#34472,#34473,#34474,#34475,#34476,#34477,#34478,#34479,#34480,#34481),
 .UNSPECIFIED.,.F.,.F.,(4,3,3,3,3,4),(0.00169583748688586,0.0625,0.09375,
0.109375,0.125,0.1328125),.UNSPECIFIED.);
#733=B_SPLINE_CURVE_WITH_KNOTS('',3,(#34486,#34487,#34488,#34489,#34490,
#34491,#34492,#34493,#34494,#34495,#34496,#34497,#34498,#34499,#34500,#34501,
#34502,#34503,#34504),.UNSPECIFIED.,.F.,.F.,(4,1,1,1,1,1,1,1,1,1,1,1,1,
1,1,1,4),(0.,0.0625,0.09375,0.125,0.15625,0.1875,0.25,0.375,0.5,0.625,0.6875,
0.71875,0.75,0.78125,0.8125,0.875,0.999999781104463),.UNSPECIFIED.);
#734=B_SPLINE_CURVE_WITH_KNOTS('',3,(#34506,#34507,#34508,#34509,#34510,
#34511,#34512,#34513,#34514,#34515,#34516,#34517,#34518,#34519,#34520,#34521,
#34522,#34523,#34524),.UNSPECIFIED.,.F.,.F.,(4,1,1,1,1,1,1,1,1,1,1,1,1,
1,1,1,4),(0.,0.125,0.1875,0.21875,0.25,0.28125,0.3125,0.375,0.5,0.625,0.75,
0.8125,0.84375,0.875,0.90625,0.9375,1.),.UNSPECIFIED.);
#735=B_SPLINE_CURVE_WITH_KNOTS('',3,(#34528,#34529,#34530,#34531,#34532,
#34533,#34534,#34535,#34536,#34537,#34538,#34539,#34540,#34541,#34542,#34543,
#34544,#34545,#34546,#34547,#34548,#34549,#34550,#34551,#34552,#34553,#34554,
#34555),.UNSPECIFIED.,.F.,.F.,(4,3,3,3,3,3,3,3,3,4),(0.,0.0625,0.09375,
0.125,0.15625,0.1875,0.25,0.364624833230614,0.375,0.499908883353168),
 .UNSPECIFIED.);
#736=B_SPLINE_CURVE_WITH_KNOTS('',3,(#34557,#34558,#34559,#34560,#34561,
#34562,#34563,#34564,#34565,#34566,#34567,#34568,#34569,#34570,#34571,#34572,
#34573,#34574,#34575,#34576,#34577,#34578,#34579,#34580,#34581),
 .UNSPECIFIED.,.F.,.F.,(4,3,3,3,3,3,3,3,4),(0.5,0.625,0.6875,0.71875,0.75,
0.78125,0.8125,0.875,0.999999882722085),.UNSPECIFIED.);
#737=B_SPLINE_CURVE_WITH_KNOTS('',3,(#34583,#34584,#34585,#34586,#34587,
#34588,#34589,#34590,#34591,#34592,#34593,#34594,#34595,#34596,#34597,#34598,
#34599,#34600,#34601,#34602,#34603,#34604,#34605,#34606,#34607),
 .UNSPECIFIED.,.F.,.F.,(4,3,3,3,3,3,3,3,4),(0.,0.125,0.1875,0.21875,0.25,
0.28125,0.3125,0.375,0.5),.UNSPECIFIED.);
#738=B_SPLINE_CURVE_WITH_KNOTS('',3,(#34608,#34609,#34610,#34611,#34612,
#34613,#34614,#34615,#34616,#34617,#34618,#34619,#34620,#34621,#34622,#34623,
#34624,#34625,#34626,#34627,#34628,#34629,#34630,#34631,#34632,#34633,#34634,
#34635),.UNSPECIFIED.,.F.,.F.,(4,3,3,3,3,3,3,3,3,4),(0.5,0.625,0.636092397936151,
0.75,0.8125,0.84375,0.875,0.90625,0.9375,1.),.UNSPECIFIED.);
#739=B_SPLINE_CURVE_WITH_KNOTS('',3,(#34638,#34639,#34640,#34641,#34642,
#34643,#34644,#34645,#34646,#34647,#34648,#34649,#34650,#34651,#34652,#34653,
#34654,#34655,#34656,#34657,#34658,#34659,#34660,#34661,#34662,#34663,#34664,
#34665,#34666,#34667,#34668,#34669,#34670,#34671,#34672,#34673,#34674,#34675,
#34676,#34677,#34678,#34679,#34680,#34681,#34682,#34683,#34684,#34685,#34686,
#34687,#34688,#34689,#34690,#34691,#34692,#34693,#34694,#34695,#34696,#34697,
#34698,#34699,#34700,#34701,#34702,#34703,#34704,#34705,#34706,#34707,#34708,
#34709,#34710,#34711,#34712,#34713,#34714,#34715,#34716,#34717,#34718,#34719,
#34720,#34721,#34722,#34723,#34724,#34725,#34726,#34727,#34728,#34729,#34730,
#34731),.UNSPECIFIED.,.F.,.F.,(4,3,3,3,3,3,3,3,3,3,3,3,3,3,3,3,3,3,3,3,
3,3,3,3,3,3,3,3,3,3,3,4),(3.86564741912649E-6,0.0625,0.125,0.1875,0.211937941253132,
0.21875,0.234375,0.25,0.2578125,0.26171875,0.265625,0.28125,0.3125,0.34375,
0.359375,0.375,0.390625,0.40625,0.4375,0.46875,0.5,0.515625,0.53125,0.5625,
0.625,0.6875,0.71875,0.75,0.78125,0.8125,0.875,1.),.UNSPECIFIED.);
#740=B_SPLINE_CURVE_WITH_KNOTS('',3,(#34733,#34734,#34735,#34736,#34737,
#34738,#34739,#34740),.UNSPECIFIED.,.F.,.F.,(4,1,1,1,1,4),(3.28844511523668E-5,
0.0625,0.125,0.25,0.375,0.5),.UNSPECIFIED.);
#741=B_SPLINE_CURVE_WITH_KNOTS('',3,(#34742,#34743,#34744,#34745,#34746,
#34747,#34748,#34749,#34750),.UNSPECIFIED.,.F.,.F.,(4,1,1,1,1,1,4),(0.500408394295939,
0.625,0.6875,0.75,0.8125,0.875,0.99850331800662),.UNSPECIFIED.);
#742=B_SPLINE_CURVE_WITH_KNOTS('',3,(#34752,#34753,#34754,#34755,#34756,
#34757,#34758,#34759,#34760,#34761,#34762,#34763,#34764,#34765,#34766,#34767),
 .UNSPECIFIED.,.F.,.F.,(4,3,3,3,3,4),(0.658287225766538,0.6875,0.716881056108036,
0.75,0.875,0.997623466937086),.UNSPECIFIED.);
#743=B_SPLINE_CURVE_WITH_KNOTS('',3,(#34769,#34770,#34771,#34772,#34773,
#34774,#34775,#34776,#34777,#34778,#34779,#34780,#34781,#34782,#34783,#34784,
#34785,#34786,#34787),.UNSPECIFIED.,.F.,.F.,(4,3,3,3,3,3,4),(0.399644838371795,
0.4375,0.5,0.53125,0.5625,0.625,0.658287225766538),.UNSPECIFIED.);
#744=B_SPLINE_CURVE_WITH_KNOTS('',3,(#34789,#34790,#34791,#34792,#34793,
#34794,#34795,#34796,#34797,#34798,#34799,#34800,#34801,#34802,#34803,#34804,
#34805,#34806,#34807,#34808,#34809,#34810,#34811,#34812,#34813),
 .UNSPECIFIED.,.F.,.F.,(4,3,3,3,3,3,3,3,4),(0.057546946328656,0.125,0.1875,
0.21875,0.25,0.28125,0.3125,0.375,0.399644838371795),.UNSPECIFIED.);
#745=B_SPLINE_CURVE_WITH_KNOTS('',3,(#34815,#34816,#34817,#34818),
 .UNSPECIFIED.,.F.,.F.,(4,4),(6.88941806839869E-6,0.057546946328656),
 .UNSPECIFIED.);
#746=B_SPLINE_CURVE_WITH_KNOTS('',3,(#34820,#34821,#34822,#34823,#34824,
#34825,#34826,#34827,#34828,#34829,#34830,#34831,#34832,#34833,#34834,#34835,
#34836,#34837,#34838,#34839,#34840,#34841,#34842,#34843,#34844,#34845,#34846,
#34847,#34848,#34849,#34850,#34851,#34852,#34853,#34854,#34855,#34856,#34857,
#34858,#34859,#34860,#34861,#34862,#34863,#34864,#34865,#34866,#34867,#34868,
#34869,#34870,#34871),.UNSPECIFIED.,.F.,.F.,(4,3,3,3,3,3,3,3,3,3,3,3,3,
3,3,3,3,4),(0.,0.125,0.1875,0.21875,0.25,0.28125,0.3125,0.375,0.5,0.625,
0.668027506996217,0.75,0.8125,0.84375,0.875,0.90625,0.9375,0.999999676766783),
 .UNSPECIFIED.);
#747=B_SPLINE_CURVE_WITH_KNOTS('',3,(#34873,#34874,#34875,#34876,#34877,
#34878,#34879,#34880,#34881),.UNSPECIFIED.,.F.,.F.,(4,1,1,1,1,1,4),(0.,
0.125,0.1875,0.25,0.3125,0.375,0.499188734755095),.UNSPECIFIED.);
#748=B_SPLINE_CURVE_WITH_KNOTS('',3,(#34883,#34884,#34885,#34886,#34887,
#34888,#34889,#34890,#34891),.UNSPECIFIED.,.F.,.F.,(4,1,1,1,1,1,4),(0.499188734755095,
0.5,0.625,0.75,0.875,0.9375,0.998149180837463),.UNSPECIFIED.);
#749=B_SPLINE_CURVE_WITH_KNOTS('',3,(#34892,#34893,#34894,#34895,#34896,
#34897,#34898,#34899,#34900,#34901,#34902,#34903,#34904,#34905,#34906,#34907,
#34908,#34909,#34910,#34911,#34912,#34913,#34914,#34915,#34916,#34917,#34918,
#34919,#34920,#34921,#34922,#34923,#34924,#34925,#34926,#34927,#34928,#34929,
#34930,#34931,#34932,#34933,#34934,#34935,#34936,#34937,#34938,#34939,#34940,
#34941,#34942,#34943,#34944,#34945,#34946,#34947,#34948,#34949),
 .UNSPECIFIED.,.F.,.F.,(4,3,3,3,3,3,3,3,3,3,3,3,3,3,3,3,3,3,3,4),(0.,0.125,
0.1875,0.21875,0.25,0.28125,0.3125,0.375,0.4375,0.5,0.5625,0.625,0.6875,
0.71875,0.75,0.78125,0.790010298169663,0.8125,0.875,1.),.UNSPECIFIED.);
#750=B_SPLINE_CURVE_WITH_KNOTS('',3,(#35010,#35011,#35012,#35013,#35014,
#35015,#35016,#35017,#35018,#35019,#35020),.UNSPECIFIED.,.F.,.F.,(4,1,1,
1,1,1,1,1,4),(0.867768400737492,0.875,0.90625,0.9375,0.953125,0.96875,0.9765625,
0.984375,1.),.UNSPECIFIED.);
#751=B_SPLINE_CURVE_WITH_KNOTS('',3,(#35021,#35022,#35023,#35024),
 .UNSPECIFIED.,.F.,.F.,(4,4),(0.0677982128913682,0.499948130219197),
 .UNSPECIFIED.);
#752=B_SPLINE_CURVE_WITH_KNOTS('',3,(#35097,#35098,#35099,#35100),
 .UNSPECIFIED.,.F.,.F.,(4,4),(6.03873264751521,6.05787500817515),
 .UNSPECIFIED.);
#753=B_SPLINE_CURVE_WITH_KNOTS('',3,(#35102,#35103,#35104,#35105,#35106,
#35107),.UNSPECIFIED.,.F.,.F.,(4,2,4),(2.5354357802791,2.79846665434659,
2.96491518441833),.UNSPECIFIED.);
#754=B_SPLINE_CURVE_WITH_KNOTS('',3,(#35108,#35109,#35110,#35111),
 .UNSPECIFIED.,.F.,.F.,(4,4),(-0.165387428475329,-0.162180666309789),
 .UNSPECIFIED.);
#755=B_SPLINE_CURVE_WITH_KNOTS('',3,(#35114,#35115,#35116,#35117,#35118,
#35119),.UNSPECIFIED.,.F.,.F.,(4,2,4),(-2.47763566945841,-2.35421341597794,
-2.20494366203894),.UNSPECIFIED.);
#756=B_SPLINE_CURVE_WITH_KNOTS('',3,(#35120,#35121,#35122,#35123),
 .UNSPECIFIED.,.F.,.F.,(4,4),(-10.5382550693381,-10.5290312685128),
 .UNSPECIFIED.);
#757=B_SPLINE_CURVE_WITH_KNOTS('',3,(#35127,#35128,#35129,#35130),
 .UNSPECIFIED.,.F.,.F.,(4,4),(0.,1.),.UNSPECIFIED.);
#758=B_SPLINE_CURVE_WITH_KNOTS('',3,(#35134,#35135,#35136,#35137),
 .UNSPECIFIED.,.F.,.F.,(4,4),(0.,0.502010271881345),.UNSPECIFIED.);
#759=B_SPLINE_CURVE_WITH_KNOTS('',3,(#35139,#35140,#35141,#35142),
 .UNSPECIFIED.,.F.,.F.,(4,4),(0.502010271881345,0.999999999999999),
 .UNSPECIFIED.);
#760=B_SPLINE_CURVE_WITH_KNOTS('',3,(#35149,#35150,#35151,#35152),
 .UNSPECIFIED.,.F.,.F.,(4,4),(0.,0.497989729516545),.UNSPECIFIED.);
#761=B_SPLINE_CURVE_WITH_KNOTS('',3,(#35154,#35155,#35156,#35157),
 .UNSPECIFIED.,.F.,.F.,(4,4),(0.497989729516545,1.),.UNSPECIFIED.);
#762=B_SPLINE_CURVE_WITH_KNOTS('',3,(#35160,#35161,#35162,#35163),
 .UNSPECIFIED.,.F.,.F.,(4,4),(0.,1.),.UNSPECIFIED.);
#763=B_SPLINE_CURVE_WITH_KNOTS('',3,(#35169,#35170,#35171,#35172),
 .UNSPECIFIED.,.F.,.F.,(4,4),(0.,0.501026353593291),.UNSPECIFIED.);
#764=B_SPLINE_CURVE_WITH_KNOTS('',3,(#35174,#35175,#35176,#35177),
 .UNSPECIFIED.,.F.,.F.,(4,4),(0.501026353593291,1.),.UNSPECIFIED.);
#765=B_SPLINE_CURVE_WITH_KNOTS('',3,(#35179,#35180,#35181,#35182,#35183,
#35184,#35185,#35186,#35187,#35188,#35189,#35190),.UNSPECIFIED.,.F.,.F.,
(4,2,2,2,2,4),(1.5151239072314E-5,0.0118829596669569,0.0177755711303306,
0.0198524710636481,0.0207583312220325,0.0215368218022216),.UNSPECIFIED.);
#766=B_SPLINE_CURVE_WITH_KNOTS('',3,(#35191,#35192,#35193,#35194),
 .UNSPECIFIED.,.F.,.F.,(4,4),(0.,1.),.UNSPECIFIED.);
#767=B_SPLINE_CURVE_WITH_KNOTS('',3,(#35198,#35199,#35200,#35201),
 .UNSPECIFIED.,.F.,.F.,(4,4),(0.,1.),.UNSPECIFIED.);
#768=B_SPLINE_CURVE_WITH_KNOTS('',3,(#35205,#35206,#35207,#35208),
 .UNSPECIFIED.,.F.,.F.,(4,4),(0.,0.502010320052747),.UNSPECIFIED.);
#769=B_SPLINE_CURVE_WITH_KNOTS('',3,(#35210,#35211,#35212,#35213),
 .UNSPECIFIED.,.F.,.F.,(4,4),(0.502010320052747,1.),.UNSPECIFIED.);
#770=B_SPLINE_CURVE_WITH_KNOTS('',3,(#35217,#35218,#35219,#35220,#35221,
#35222,#35223,#35224),.UNSPECIFIED.,.F.,.F.,(4,2,2,4),(-3.01857335434641,
-3.01637328016506,-2.78274428831762,-2.67485962322313),.UNSPECIFIED.);
#771=B_SPLINE_CURVE_WITH_KNOTS('',3,(#35225,#35226,#35227,#35228),
 .UNSPECIFIED.,.F.,.F.,(4,4),(-0.274599042102008,-0.00061961661749236),
 .UNSPECIFIED.);
#772=B_SPLINE_CURVE_WITH_KNOTS('',3,(#35388,#35389,#35390,#35391,#35392,
#35393,#35394,#35395,#35396,#35397,#35398,#35399,#35400,#35401,#35402,#35403,
#35404,#35405,#35406,#35407,#35408,#35409),.UNSPECIFIED.,.F.,.F.,(4,3,3,
3,3,3,3,4),(5.10562847884237E-9,0.00374014353849567,0.00748028707699134,
0.00749196373323959,0.00935035884623917,0.011220430615487,0.0130905023847349,
0.0149605741539827),.UNSPECIFIED.);
#773=B_SPLINE_CURVE_WITH_KNOTS('',3,(#35411,#35412,#35413,#35414,#35415,
#35416,#35417,#35418,#35419,#35420,#35421,#35422,#35423,#35424,#35425,#35426,
#35427,#35428,#35429,#35430,#35431,#35432),.UNSPECIFIED.,.F.,.F.,(4,3,3,
3,3,3,3,4),(0.0149612645537521,0.0168306459232305,0.0187007176924783,0.0205707894617261,
0.0224303512848831,0.022440861230974,0.0261810047694697,0.0299211432894142),
 .UNSPECIFIED.);
#774=B_SPLINE_CURVE_WITH_KNOTS('',3,(#35435,#35436,#35437,#35438,#35439,
#35440,#35441,#35442,#35443,#35444,#35445,#35446,#35447,#35448,#35449,#35450,
#35451,#35452,#35453,#35454,#35455,#35456,#35457,#35458,#35459),
 .UNSPECIFIED.,.F.,.F.,(4,3,3,3,3,3,3,3,4),(5.10602741926278E-9,0.00374013872221605,
0.0074802774444321,0.00749195384150005,0.00935034680554015,0.0112204161666482,
0.0130904855277562,0.0149605548888642,0.0158713903754465),.UNSPECIFIED.);
#775=B_SPLINE_CURVE_WITH_KNOTS('',3,(#35463,#35464,#35465,#35466,#35467,
#35468,#35469),.UNSPECIFIED.,.F.,.F.,(4,1,1,1,4),(1.7347234759768E-18,0.00269008839466431,
0.00538017678932861,0.00807026518399292,0.0107603535786572),
 .UNSPECIFIED.);
#776=B_SPLINE_CURVE_WITH_KNOTS('',3,(#35471,#35472,#35473,#35474,#35475,
#35476,#35477,#35478,#35479,#35480,#35481,#35482,#35483,#35484,#35485,#35486,
#35487,#35488,#35489,#35490,#35491,#35492,#35493,#35494,#35495,#35496,#35497,
#35498,#35499,#35500,#35501,#35502,#35503,#35504,#35505,#35506,#35507,#35508,
#35509,#35510),.UNSPECIFIED.,.F.,.F.,(4,3,3,3,3,3,3,3,3,3,3,3,3,4),(1.10894064381892E-8,
0.125,0.25,0.3125,0.375,0.4375,0.46875,0.5,0.53125,0.5625,0.625,0.75,0.875,
0.999999989312939),.UNSPECIFIED.);
#777=B_SPLINE_CURVE_WITH_KNOTS('',3,(#35512,#35513,#35514,#35515,#35516,
#35517,#35518,#35519,#35520,#35521,#35522,#35523,#35524,#35525,#35526,#35527,
#35528,#35529,#35530,#35531,#35532,#35533,#35534,#35535,#35536,#35537,#35538,
#35539,#35540,#35541,#35542,#35543,#35544,#35545,#35546,#35547,#35548,#35549,
#35550,#35551,#35552,#35553,#35554,#35555,#35556,#35557,#35558,#35559,#35560,
#35561,#35562,#35563,#35564,#35565,#35566,#35567,#35568,#35569,#35570,#35571,
#35572),.UNSPECIFIED.,.F.,.F.,(4,3,3,3,3,3,3,3,3,3,3,3,3,3,3,3,3,3,3,3,
4),(1.70073241358158E-10,0.00197446710728151,0.00220015688427838,0.00440031376855676,
0.00512931019723391,0.00550039221069595,0.00625356878405253,0.00660047065283514,
0.00728477966928603,0.00880062753711352,0.00920071084948763,0.0101615955899537,
0.0106616073838042,0.0110007844213919,0.011183305887491,0.0121008628635311,
0.0122880395709336,0.0132009413056703,0.0135642393762939,0.0154010981899487,
0.0176012549038037),.UNSPECIFIED.);
#778=B_SPLINE_CURVE_WITH_KNOTS('',3,(#35574,#35575,#35576,#35577,#35578,
#35579,#35580,#35581,#35582,#35583,#35584,#35585,#35586,#35587,#35588,#35589,
#35590,#35591,#35592,#35593,#35594,#35595,#35596,#35597,#35598,#35599,#35600,
#35601),.UNSPECIFIED.,.F.,.F.,(4,3,3,3,3,3,3,3,3,4),(1.06497082191348E-8,
0.0625,0.125,0.15625,0.1875,0.25,0.375,0.5,0.75,0.999999988547865),
 .UNSPECIFIED.);
#779=B_SPLINE_CURVE_WITH_KNOTS('',3,(#35603,#35604,#35605,#35606,#35607,
#35608,#35609),.UNSPECIFIED.,.F.,.F.,(4,1,1,1,4),(3.33360433782453E-17,
0.00266695541805129,0.00533391083610256,0.00800086625415382,0.0106678216722051),
 .UNSPECIFIED.);
#780=B_SPLINE_CURVE_WITH_KNOTS('',3,(#35613,#35614,#35615,#35616,#35617,
#35618,#35619),.UNSPECIFIED.,.F.,.F.,(4,1,1,1,4),(2.43480042509997E-17,
0.00269008902712854,0.00538017805425706,0.00807026708138558,0.0107603561085141),
 .UNSPECIFIED.);
#781=B_SPLINE_CURVE_WITH_KNOTS('',3,(#35621,#35622,#35623,#35624,#35625,
#35626,#35627,#35628,#35629,#35630,#35631,#35632,#35633,#35634,#35635,#35636,
#35637,#35638,#35639,#35640,#35641,#35642,#35643,#35644,#35645,#35646,#35647,
#35648,#35649,#35650,#35651,#35652,#35653,#35654,#35655,#35656,#35657,#35658,
#35659,#35660),.UNSPECIFIED.,.F.,.F.,(4,3,3,3,3,3,3,3,3,3,3,3,3,4),(1.10899779061613E-8,
0.125,0.25,0.3125,0.375,0.4375,0.46875,0.5,0.53125,0.5625,0.625,0.75,0.875,
0.999999989362077),.UNSPECIFIED.);
#782=B_SPLINE_CURVE_WITH_KNOTS('',3,(#35661,#35662,#35663,#35664,#35665,
#35666,#35667,#35668,#35669,#35670,#35671,#35672,#35673,#35674,#35675,#35676,
#35677,#35678,#35679,#35680,#35681,#35682,#35683,#35684,#35685,#35686,#35687,
#35688,#35689,#35690,#35691,#35692,#35693,#35694,#35695,#35696,#35697,#35698,
#35699,#35700,#35701,#35702,#35703),.UNSPECIFIED.,.F.,.F.,(4,3,3,3,3,3,
3,3,3,3,3,3,3,3,4),(1.70091092863581E-10,0.00197446788219035,0.00220015692671693,
0.00440031385343386,0.00512931098783657,0.00550039231679233,0.00625356907264106,
0.00660047078015079,0.00728477985782865,0.00880062770686772,0.00920071115763201,
0.01016159594726,0.0106616077611924,0.0110007846335847,0.0111833063008374),
 .UNSPECIFIED.);
#783=B_SPLINE_CURVE_WITH_KNOTS('',3,(#35706,#35707,#35708,#35709),
 .UNSPECIFIED.,.F.,.F.,(4,4),(6.55458962298397E-7,1.),.UNSPECIFIED.);
#784=B_SPLINE_CURVE_WITH_KNOTS('',3,(#35711,#35712,#35713,#35714),
 .UNSPECIFIED.,.F.,.F.,(4,4),(3.49092837846564E-8,0.000279639041028945),
 .UNSPECIFIED.);
#785=B_SPLINE_CURVE_WITH_KNOTS('',3,(#35716,#35717,#35718,#35719,#35720,
#35721,#35722,#35723,#35724,#35725),.UNSPECIFIED.,.F.,.F.,(4,2,2,2,4),(5.89420191983957E-6,
0.000303437783884664,0.000632488927968499,0.00143564842888828,0.00301213449051446),
 .UNSPECIFIED.);
#786=B_SPLINE_CURVE_WITH_KNOTS('',3,(#35727,#35728,#35729,#35730),
 .UNSPECIFIED.,.F.,.F.,(4,4),(5.05038109498685E-5,0.999936832443628),
 .UNSPECIFIED.);
#787=B_SPLINE_CURVE_WITH_KNOTS('',3,(#35732,#35733,#35734,#35735,#35736,
#35737,#35738,#35739,#35740,#35741),.UNSPECIFIED.,.F.,.F.,(4,2,2,2,4),(-0.0032145494986627,
-0.00295256209228294,-0.0026513848523457,-0.00194290947785501,-1.68534414557259E-6),
 .UNSPECIFIED.);
#788=B_SPLINE_CURVE_WITH_KNOTS('',3,(#35743,#35744,#35745,#35746),
 .UNSPECIFIED.,.F.,.F.,(4,4),(2.31286388414311E-11,0.000279603602071489),
 .UNSPECIFIED.);
#789=B_SPLINE_CURVE_WITH_KNOTS('',3,(#35747,#35748,#35749,#35750),
 .UNSPECIFIED.,.F.,.F.,(4,4),(0.,1.),.UNSPECIFIED.);
#790=B_SPLINE_CURVE_WITH_KNOTS('',3,(#35753,#35754,#35755,#35756,#35757,
#35758,#35759,#35760,#35761,#35762,#35763,#35764,#35765,#35766,#35767,#35768,
#35769,#35770,#35771,#35772,#35773,#35774,#35775,#35776,#35777,#35778,#35779,
#35780),.UNSPECIFIED.,.F.,.F.,(4,3,3,3,3,3,3,3,3,4),(0.,0.00219009522320418,
0.00438019044640836,0.00547523805801045,0.00657028566961254,0.00876038089281672,
0.0109504761160209,0.012045523727623,0.0131405713392251,0.0146411293071528),
 .UNSPECIFIED.);
#791=B_SPLINE_CURVE_WITH_KNOTS('',3,(#35781,#35782,#35783,#35784,#35785,
#35786,#35787),.UNSPECIFIED.,.F.,.F.,(4,3,4),(0.0146411293071528,0.0153306665624293,
0.0175207617856334),.UNSPECIFIED.);
#792=B_SPLINE_CURVE_WITH_KNOTS('',3,(#35789,#35790,#35791,#35792),
 .UNSPECIFIED.,.F.,.F.,(4,4),(4.55973828920902E-10,0.00219012841858902),
 .UNSPECIFIED.);
#793=B_SPLINE_CURVE_WITH_KNOTS('',3,(#35793,#35794,#35795,#35796,#35797,
#35798,#35799,#35800,#35801,#35802,#35803,#35804,#35805,#35806,#35807,#35808,
#35809,#35810,#35811,#35812,#35813,#35814,#35815,#35816,#35817,#35818,#35819,
#35820),.UNSPECIFIED.,.F.,.F.,(4,3,3,3,3,3,3,3,3,4),(0.00219035076041224,
0.00438070152082448,0.00547587690103059,0.00657105228123671,0.00876140304164895,
0.0109517538020612,0.0120469291822673,0.0131421045624734,0.0153324553228857,
0.0175228056278763),.UNSPECIFIED.);
#794=B_SPLINE_CURVE_WITH_KNOTS('',3,(#35823,#35824,#35825,#35826,#35827,
#35828,#35829,#35830,#35831,#35832,#35833,#35834,#35835,#35836,#35837,#35838,
#35839,#35840,#35841,#35842,#35843,#35844,#35845,#35846,#35847,#35848,#35849,
#35850),.UNSPECIFIED.,.F.,.F.,(4,3,3,3,3,3,3,3,3,4),(0.,0.00219009519209258,
0.00438019038418515,0.00547523798023144,0.00657028557627773,0.0087603807683703,
0.0109504759604629,0.0120455235565092,0.0131405711525555,0.0146411150843174),
 .UNSPECIFIED.);
#795=B_SPLINE_CURVE_WITH_KNOTS('',3,(#35851,#35852,#35853,#35854,#35855,
#35856,#35857),.UNSPECIFIED.,.F.,.F.,(4,3,4),(0.0146411150843174,0.015330666344648,
0.0175207615367406),.UNSPECIFIED.);
#796=B_SPLINE_CURVE_WITH_KNOTS('',3,(#35859,#35860,#35861,#35862),
 .UNSPECIFIED.,.F.,.F.,(4,4),(4.55959294391392E-10,0.00219012846087483),
 .UNSPECIFIED.);
#797=B_SPLINE_CURVE_WITH_KNOTS('',3,(#35863,#35864,#35865,#35866,#35867,
#35868,#35869,#35870,#35871,#35872,#35873,#35874,#35875,#35876,#35877,#35878,
#35879,#35880,#35881,#35882,#35883,#35884,#35885,#35886,#35887,#35888,#35889,
#35890),.UNSPECIFIED.,.F.,.F.,(4,3,3,3,3,3,3,3,3,4),(0.00219035079403417,
0.00438070158806835,0.00547587698508544,0.00657105238210252,0.0087614031761367,
0.0109517539701709,0.012046929367188,0.013142104764205,0.0153324555582392,
0.0175228058968349),.UNSPECIFIED.);
#798=B_SPLINE_CURVE_WITH_KNOTS('',3,(#35893,#35894,#35895,#35896),
 .UNSPECIFIED.,.F.,.F.,(4,4),(6.67616818609268E-7,1.),.UNSPECIFIED.);
#799=B_SPLINE_CURVE_WITH_KNOTS('',3,(#35898,#35899,#35900,#35901),
 .UNSPECIFIED.,.F.,.F.,(4,4),(3.49092066549658E-8,0.000279639070515748),
 .UNSPECIFIED.);
#800=B_SPLINE_CURVE_WITH_KNOTS('',3,(#35903,#35904,#35905,#35906),
 .UNSPECIFIED.,.F.,.F.,(4,4),(0.00344166019661847,0.00347128806463756),
 .UNSPECIFIED.);
#801=B_SPLINE_CURVE_WITH_KNOTS('',3,(#35908,#35909,#35910,#35911),
 .UNSPECIFIED.,.F.,.F.,(4,4),(7.68669616547862E-6,0.999996430487618),
 .UNSPECIFIED.);
#802=B_SPLINE_CURVE_WITH_KNOTS('',3,(#35915,#35916,#35917,#35918),
 .UNSPECIFIED.,.F.,.F.,(4,4),(2.31289797358325E-11,0.000279603631692585),
 .UNSPECIFIED.);
#803=B_SPLINE_CURVE_WITH_KNOTS('',3,(#35919,#35920,#35921,#35922),
 .UNSPECIFIED.,.F.,.F.,(4,4),(0.,1.),.UNSPECIFIED.);
#804=B_SPLINE_CURVE_WITH_KNOTS('',3,(#35928,#35929,#35930,#35931,#35932),
 .UNSPECIFIED.,.F.,.F.,(4,1,4),(3.90312782094781E-18,0.00385428159543372,
0.00770856319086743),.UNSPECIFIED.);
#805=B_SPLINE_CURVE_WITH_KNOTS('',3,(#35934,#35935,#35936,#35937),
 .UNSPECIFIED.,.F.,.F.,(4,4),(0.00770856319086743,0.0115628447863011),
 .UNSPECIFIED.);
#806=B_SPLINE_CURVE_WITH_KNOTS('',3,(#35939,#35940,#35941,#35942),
 .UNSPECIFIED.,.F.,.F.,(4,4),(0.0115628447863011,0.0154171263817349),
 .UNSPECIFIED.);
#807=B_SPLINE_CURVE_WITH_KNOTS('',3,(#35944,#35945,#35946,#35947,#35948,
#35949,#35950),.UNSPECIFIED.,.F.,.F.,(4,1,1,1,4),(0.0154171263817349,0.0192714079771686,
0.0231256895726023,0.026979971168036,0.0308342527634697),.UNSPECIFIED.);
#808=B_SPLINE_CURVE_WITH_KNOTS('',3,(#35953,#35954,#35955,#35956,#35957,
#35958,#35959,#35960,#35961,#35962,#35963,#35964,#35965,#35966,#35967,#35968,
#35969,#35970,#35971,#35972,#35973,#35974,#35975,#35976,#35977),
 .UNSPECIFIED.,.F.,.F.,(4,3,3,3,3,3,3,3,4),(3.49644694633735E-18,0.0038084153469596,
0.00761683069391923,0.0114252460408789,0.0152336613878385,0.0190420767347981,
0.0228504920817577,0.0266589074287173,0.0304673227756769),.UNSPECIFIED.);
#809=B_SPLINE_CURVE_WITH_KNOTS('',3,(#35980,#35981,#35982,#35983,#35984,
#35985,#35986,#35987,#35988,#35989),.UNSPECIFIED.,.F.,.F.,(4,3,3,4),(4.95617171550503E-9,
0.03125,0.0625,0.09375),.UNSPECIFIED.);
#810=B_SPLINE_CURVE_WITH_KNOTS('',3,(#35991,#35992,#35993,#35994,#35995,
#35996,#35997,#35998,#35999,#36000,#36001,#36002,#36003,#36004,#36005,#36006,
#36007,#36008,#36009),.UNSPECIFIED.,.F.,.F.,(4,3,3,3,3,3,4),(0.09375,0.125,
0.15625,0.1875,0.21875,0.25,0.28125),.UNSPECIFIED.);
#811=B_SPLINE_CURVE_WITH_KNOTS('',3,(#36011,#36012,#36013,#36014,#36015,
#36016,#36017,#36018,#36019,#36020,#36021,#36022,#36023,#36024,#36025,#36026),
 .UNSPECIFIED.,.F.,.F.,(4,3,3,3,3,4),(0.28125,0.3125,0.375,0.5,0.625,0.658880396082507),
 .UNSPECIFIED.);
#812=B_SPLINE_CURVE_WITH_KNOTS('',3,(#36028,#36029,#36030,#36031,#36032,
#36033,#36034,#36035,#36036,#36037,#36038,#36039,#36040,#36041,#36042,#36043,
#36044,#36045,#36046,#36047,#36048,#36049,#36050,#36051,#36052),
 .UNSPECIFIED.,.F.,.F.,(4,3,3,3,3,3,3,3,4),(0.658880396082507,0.6875,0.71875,
0.75,0.78125,0.8125,0.84375,0.875,0.901787328791184),.UNSPECIFIED.);
#813=B_SPLINE_CURVE_WITH_KNOTS('',3,(#36054,#36055,#36056,#36057,#36058,
#36059,#36060,#36061,#36062,#36063,#36064,#36065,#36066),.UNSPECIFIED.,
 .F.,.F.,(4,3,3,3,4),(0.901787328791184,0.90625,0.9375,0.96875,0.999999995039462),
 .UNSPECIFIED.);
#814=B_SPLINE_CURVE_WITH_KNOTS('',3,(#36070,#36071,#36072,#36073,#36074,
#36075,#36076,#36077,#36078,#36079),.UNSPECIFIED.,.F.,.F.,(4,3,3,4),(0.,
0.03125,0.0625,0.078125),.UNSPECIFIED.);
#815=B_SPLINE_CURVE_WITH_KNOTS('',3,(#36081,#36082,#36083,#36084,#36085,
#36086,#36087,#36088,#36089,#36090,#36091,#36092,#36093,#36094,#36095,#36096,
#36097,#36098,#36099,#36100,#36101,#36102),.UNSPECIFIED.,.F.,.F.,(4,3,3,
3,3,3,3,4),(0.078125,0.09375,0.125,0.15625,0.1875,0.21875,0.25,0.28125),
 .UNSPECIFIED.);
#816=B_SPLINE_CURVE_WITH_KNOTS('',3,(#36104,#36105,#36106,#36107,#36108,
#36109,#36110,#36111,#36112,#36113,#36114,#36115,#36116,#36117,#36118,#36119),
 .UNSPECIFIED.,.F.,.F.,(4,3,3,3,3,4),(0.28125,0.3125,0.375,0.5,0.625,0.658099954027992),
 .UNSPECIFIED.);
#817=B_SPLINE_CURVE_WITH_KNOTS('',3,(#36121,#36122,#36123,#36124,#36125,
#36126,#36127,#36128,#36129,#36130,#36131,#36132,#36133,#36134,#36135,#36136,
#36137,#36138,#36139,#36140,#36141,#36142,#36143,#36144,#36145),
 .UNSPECIFIED.,.F.,.F.,(4,3,3,3,3,3,3,3,4),(0.658099954027992,0.6875,0.71875,
0.75,0.78125,0.8125,0.84375,0.875,0.899951537400222),.UNSPECIFIED.);
#818=B_SPLINE_CURVE_WITH_KNOTS('',3,(#36146,#36147,#36148,#36149,#36150,
#36151,#36152,#36153,#36154,#36155,#36156,#36157,#36158,#36159,#36160,#36161),
 .UNSPECIFIED.,.F.,.F.,(4,3,3,3,3,4),(0.899951537400222,0.90625,0.921875,
0.9375,0.96875,1.),.UNSPECIFIED.);
#819=B_SPLINE_CURVE_WITH_KNOTS('',3,(#36167,#36168,#36169,#36170,#36171,
#36172,#36173,#36174,#36175,#36176),.UNSPECIFIED.,.F.,.F.,(4,3,3,4),(4.95657091019873E-9,
0.03125,0.0625,0.09375),.UNSPECIFIED.);
#820=B_SPLINE_CURVE_WITH_KNOTS('',3,(#36178,#36179,#36180,#36181,#36182,
#36183,#36184,#36185,#36186,#36187,#36188,#36189,#36190,#36191,#36192,#36193,
#36194,#36195,#36196),.UNSPECIFIED.,.F.,.F.,(4,3,3,3,3,3,4),(0.09375,0.125,
0.15625,0.1875,0.21875,0.25,0.28125),.UNSPECIFIED.);
#821=B_SPLINE_CURVE_WITH_KNOTS('',3,(#36198,#36199,#36200,#36201,#36202,
#36203,#36204,#36205,#36206,#36207,#36208,#36209,#36210,#36211,#36212,#36213),
 .UNSPECIFIED.,.F.,.F.,(4,3,3,3,3,4),(0.28125,0.3125,0.375,0.5,0.625,0.658881231743818),
 .UNSPECIFIED.);
#822=B_SPLINE_CURVE_WITH_KNOTS('',3,(#36215,#36216,#36217,#36218,#36219,
#36220,#36221,#36222,#36223,#36224,#36225,#36226,#36227,#36228,#36229,#36230,
#36231,#36232,#36233,#36234,#36235,#36236,#36237,#36238,#36239),
 .UNSPECIFIED.,.F.,.F.,(4,3,3,3,3,3,3,3,4),(0.658881231743818,0.6875,0.71875,
0.75,0.78125,0.8125,0.84375,0.875,0.901786418266221),.UNSPECIFIED.);
#823=B_SPLINE_CURVE_WITH_KNOTS('',3,(#36240,#36241,#36242,#36243,#36244,
#36245,#36246,#36247,#36248,#36249,#36250,#36251,#36252),.UNSPECIFIED.,
 .F.,.F.,(4,3,3,3,4),(0.901786418266221,0.90625,0.9375,0.96875,0.999999995039868),
 .UNSPECIFIED.);
#824=B_SPLINE_CURVE_WITH_KNOTS('',3,(#36254,#36255,#36256,#36257,#36258,
#36259,#36260,#36261,#36262,#36263),.UNSPECIFIED.,.F.,.F.,(4,3,3,4),(0.,
0.03125,0.0625,0.078125),.UNSPECIFIED.);
#825=B_SPLINE_CURVE_WITH_KNOTS('',3,(#36265,#36266,#36267,#36268,#36269,
#36270,#36271,#36272,#36273,#36274,#36275,#36276,#36277,#36278,#36279,#36280,
#36281,#36282,#36283,#36284,#36285,#36286),.UNSPECIFIED.,.F.,.F.,(4,3,3,
3,3,3,3,4),(0.078125,0.09375,0.125,0.15625,0.1875,0.21875,0.25,0.28125),
 .UNSPECIFIED.);
#826=B_SPLINE_CURVE_WITH_KNOTS('',3,(#36288,#36289,#36290,#36291,#36292,
#36293,#36294,#36295,#36296,#36297,#36298,#36299,#36300,#36301,#36302,#36303),
 .UNSPECIFIED.,.F.,.F.,(4,3,3,3,3,4),(0.28125,0.3125,0.375,0.5,0.625,0.658099136367619),
 .UNSPECIFIED.);
#827=B_SPLINE_CURVE_WITH_KNOTS('',3,(#36305,#36306,#36307,#36308,#36309,
#36310,#36311,#36312,#36313,#36314,#36315,#36316,#36317,#36318,#36319,#36320,
#36321,#36322,#36323,#36324,#36325,#36326,#36327,#36328,#36329),
 .UNSPECIFIED.,.F.,.F.,(4,3,3,3,3,3,3,3,4),(0.658099136367619,0.6875,0.71875,
0.75,0.78125,0.8125,0.84375,0.875,0.899952381870881),.UNSPECIFIED.);
#828=B_SPLINE_CURVE_WITH_KNOTS('',3,(#36330,#36331,#36332,#36333,#36334,
#36335,#36336,#36337,#36338,#36339,#36340,#36341,#36342,#36343,#36344,#36345),
 .UNSPECIFIED.,.F.,.F.,(4,3,3,3,3,4),(0.899952381870881,0.90625,0.921875,
0.9375,0.96875,1.),.UNSPECIFIED.);
#829=B_SPLINE_CURVE_WITH_KNOTS('',3,(#36348,#36349,#36350,#36351,#36352),
 .UNSPECIFIED.,.F.,.F.,(4,1,4),(2.21134721367331E-18,0.00385428119363376,
0.00770856238726751),.UNSPECIFIED.);
#830=B_SPLINE_CURVE_WITH_KNOTS('',3,(#36354,#36355,#36356,#36357),
 .UNSPECIFIED.,.F.,.F.,(4,4),(0.00770856238726751,0.0115628435809013),
 .UNSPECIFIED.);
#831=B_SPLINE_CURVE_WITH_KNOTS('',3,(#36359,#36360,#36361,#36362),
 .UNSPECIFIED.,.F.,.F.,(4,4),(0.0115628435809013,0.015417124774535),
 .UNSPECIFIED.);
#832=B_SPLINE_CURVE_WITH_KNOTS('',3,(#36363,#36364,#36365,#36366,#36367,
#36368,#36369),.UNSPECIFIED.,.F.,.F.,(4,1,1,1,4),(0.015417124774535,0.0192714059681688,
0.0231256871618025,0.0269799683554363,0.0308342495490701),.UNSPECIFIED.);
#833=B_SPLINE_CURVE_WITH_KNOTS('',3,(#36370,#36371,#36372,#36373,#36374,
#36375,#36376,#36377,#36378,#36379,#36380,#36381,#36382,#36383,#36384,#36385,
#36386,#36387,#36388,#36389,#36390,#36391,#36392,#36393,#36394),
 .UNSPECIFIED.,.F.,.F.,(4,3,3,3,3,3,3,3,4),(3.03576608295941E-18,0.00380841492928532,
0.00761682985857062,0.0114252447878558,0.0152336597171411,0.0190420746464265,
0.0228504895757117,0.026658904504997,0.0304673194342823),.UNSPECIFIED.);
#834=B_SPLINE_CURVE_WITH_KNOTS('',3,(#36397,#36398,#36399,#36400,#36401,
#36402,#36403),.UNSPECIFIED.,.F.,.F.,(4,1,1,1,4),(5.23213817258733E-8,0.0029056070149641,
0.00581121402992687,0.00871682104488963,0.0116224280598524),
 .UNSPECIFIED.);
#835=B_SPLINE_CURVE_WITH_KNOTS('',3,(#36406,#36407,#36408,#36409,#36410,
#36411,#36412,#36413,#36414,#36415,#36416,#36417,#36418,#36419,#36420,#36421,
#36422,#36423,#36424,#36425,#36426,#36427,#36428,#36429,#36430,#36431,#36432,
#36433,#36434,#36435,#36436),.UNSPECIFIED.,.F.,.F.,(4,3,3,3,3,3,3,3,3,3,
4),(0.000307410351405465,0.0030481449392632,0.0030636165255644,0.00441851223319206,
0.00578887952712092,0.00581844748756307,0.00715924682104978,0.00852961411497865,
0.00857611852702666,0.00989998140890752,0.0112703487028364),
 .UNSPECIFIED.);
#836=B_SPLINE_CURVE_WITH_KNOTS('',3,(#36439,#36440,#36441,#36442,#36443,
#36444,#36445),.UNSPECIFIED.,.F.,.F.,(4,1,1,1,4),(3.65940318147201E-17,
0.00281356312006687,0.00562712624013371,0.00844068936020054,0.0112542524802674),
 .UNSPECIFIED.);
#837=B_SPLINE_CURVE_WITH_KNOTS('',3,(#36447,#36448,#36449,#36450,#36451,
#36452,#36453,#36454,#36455,#36456,#36457,#36458,#36459),.UNSPECIFIED.,
 .F.,.F.,(4,3,3,3,4),(0.,0.25,0.5,0.75,0.999991910881764),.UNSPECIFIED.);
#838=B_SPLINE_CURVE_WITH_KNOTS('',3,(#36460,#36461,#36462,#36463,#36464,
#36465,#36466),.UNSPECIFIED.,.F.,.F.,(4,1,1,1,4),(0.000444700170075515,
0.00338593218391437,0.00632716419775323,0.00926839621159208,0.0122095755614429),
 .UNSPECIFIED.);
#839=B_SPLINE_CURVE_WITH_KNOTS('',3,(#36471,#36472,#36473,#36474,#36475,
#36476,#36477),.UNSPECIFIED.,.F.,.F.,(4,1,1,1,4),(1.46628880702953E-15,
0.00294691748194268,0.0058938349638839,0.00884075244582512,0.0117876171100227),
 .UNSPECIFIED.);
#840=B_SPLINE_CURVE_WITH_KNOTS('',3,(#36478,#36479,#36480,#36481,#36482,
#36483,#36484),.UNSPECIFIED.,.F.,.F.,(4,1,1,1,4),(9.42515350988308E-17,
0.00274256564248042,0.00548513128496075,0.00822769692744107,0.0109702625699214),
 .UNSPECIFIED.);
#841=B_SPLINE_CURVE_WITH_KNOTS('',3,(#36487,#36488,#36489,#36490,#36491,
#36492,#36493),.UNSPECIFIED.,.F.,.F.,(4,1,1,1,4),(5.24770762208555E-8,0.0029075980930468,
0.00581519618608887,0.00872279427913093,0.011630392372173),
 .UNSPECIFIED.);
#842=B_SPLINE_CURVE_WITH_KNOTS('',3,(#36496,#36497,#36498,#36499,#36500,
#36501,#36502,#36503,#36504,#36505,#36506,#36507,#36508,#36509,#36510,#36511,
#36512,#36513,#36514,#36515,#36516,#36517,#36518,#36519,#36520,#36521,#36522,
#36523,#36524,#36525,#36526),.UNSPECIFIED.,.F.,.F.,(4,3,3,3,3,3,3,3,3,3,
4),(0.000307411164707473,0.00304814514067886,0.00306361677010575,0.00441851212866456,
0.00578887911665026,0.00581844712117058,0.00715924610463596,0.00852961309262165,
0.00857611755053204,0.00989998008060733,0.011270347068593),
 .UNSPECIFIED.);
#843=B_SPLINE_CURVE_WITH_KNOTS('',3,(#36569,#36570,#36571,#36572,#36573,
#36574,#36575),.UNSPECIFIED.,.F.,.F.,(4,3,4),(1.7082471228229E-5,0.825036313420024,
1.),.UNSPECIFIED.);
#844=B_SPLINE_CURVE_WITH_KNOTS('',3,(#36599,#36600,#36601,#36602,#36603,
#36604),.UNSPECIFIED.,.F.,.F.,(4,2,4),(-0.0126200035614453,-0.00663868323303364,
-1.51764961458753E-5),.UNSPECIFIED.);
#845=B_SPLINE_CURVE_WITH_KNOTS('',3,(#36605,#36606,#36607,#36608,#36609,
#36610,#36611),.UNSPECIFIED.,.F.,.F.,(4,3,4),(0.,0.632718071204813,0.999999748705075),
 .UNSPECIFIED.);
#846=B_SPLINE_CURVE_WITH_KNOTS('',3,(#36634,#36635,#36636,#36637,#36638,
#36639,#36640),.UNSPECIFIED.,.F.,.F.,(4,3,4),(2.03490870871502E-6,0.698513719527809,
1.),.UNSPECIFIED.);
#847=B_SPLINE_CURVE_WITH_KNOTS('',3,(#36642,#36643,#36644,#36645,#36646,
#36647,#36648),.UNSPECIFIED.,.F.,.F.,(4,3,4),(2.56083752551901E-7,0.698445555099148,
0.9999999084914),.UNSPECIFIED.);
#848=B_SPLINE_CURVE_WITH_KNOTS('',3,(#36650,#36651,#36652,#36653,#36654,
#36655,#36656),.UNSPECIFIED.,.F.,.F.,(4,3,4),(4.92776746415909E-7,0.6333331216261,
0.999995687372378),.UNSPECIFIED.);
#849=B_SPLINE_CURVE_WITH_KNOTS('',3,(#36779,#36780,#36781,#36782,#36783,
#36784,#36785),.UNSPECIFIED.,.F.,.F.,(4,3,4),(0.,0.861053093920219,1.),
 .UNSPECIFIED.);
#850=B_SPLINE_CURVE_WITH_KNOTS('',3,(#36786,#36787,#36788,#36789,#36790,
#36791,#36792),.UNSPECIFIED.,.F.,.F.,(4,3,4),(0.,0.861042149630975,1.),
 .UNSPECIFIED.);
#851=B_SPLINE_CURVE_WITH_KNOTS('',3,(#36794,#36795,#36796,#36797,#36798,
#36799,#36800),.UNSPECIFIED.,.F.,.F.,(4,3,4),(0.,0.861053136203872,1.),
 .UNSPECIFIED.);
#852=B_SPLINE_CURVE_WITH_KNOTS('',3,(#36802,#36803,#36804,#36805,#36806,
#36807,#36808),.UNSPECIFIED.,.F.,.F.,(4,3,4),(0.,0.861042192136075,1.),
 .UNSPECIFIED.);
#853=B_SPLINE_CURVE_WITH_KNOTS('',3,(#36913,#36914,#36915,#36916,#36917,
#36918,#36919),.UNSPECIFIED.,.F.,.F.,(4,3,4),(0.,0.730996929438668,1.),
 .UNSPECIFIED.);
#854=B_SPLINE_CURVE_WITH_KNOTS('',3,(#36922,#36923,#36924,#36925,#36926,
#36927,#36928),.UNSPECIFIED.,.F.,.F.,(4,3,4),(0.,0.770155557257018,1.),
 .UNSPECIFIED.);
#855=B_SPLINE_CURVE_WITH_KNOTS('',3,(#36953,#36954,#36955,#36956,#36957,
#36958,#36959),.UNSPECIFIED.,.F.,.F.,(4,3,4),(0.,0.730997037997434,1.),
 .UNSPECIFIED.);
#856=B_SPLINE_CURVE_WITH_KNOTS('',3,(#36988,#36989,#36990,#36991,#36992,
#36993,#36994),.UNSPECIFIED.,.F.,.F.,(4,3,4),(0.,0.770155702463764,1.),
 .UNSPECIFIED.);
#857=B_SPLINE_CURVE_WITH_KNOTS('',3,(#37016,#37017,#37018,#37019),
 .UNSPECIFIED.,.F.,.F.,(4,4),(0.,1.),.UNSPECIFIED.);
#858=B_SPLINE_CURVE_WITH_KNOTS('',3,(#37148,#37149,#37150,#37151),
 .UNSPECIFIED.,.F.,.F.,(4,4),(-0.705935800703831,-0.696391995080821),
 .UNSPECIFIED.);
#859=B_SPLINE_CURVE_WITH_KNOTS('',3,(#37293,#37294,#37295,#37296,#37297,
#37298,#37299,#37300,#37301,#37302),.UNSPECIFIED.,.F.,.F.,(4,3,3,4),(0.00380005432105398,
0.00387434298579466,0.00432138238092229,0.00476842177604991),
 .UNSPECIFIED.);
#860=B_SPLINE_CURVE_WITH_KNOTS('',3,(#37304,#37305,#37306,#37307,#37308,
#37309),.UNSPECIFIED.,.F.,.F.,(4,2,4),(3.88881683081212E-5,0.0373227534595625,
0.0745507150811631),.UNSPECIFIED.);
#861=B_SPLINE_CURVE_WITH_KNOTS('',3,(#37313,#37314,#37315,#37316,#37317,
#37318),.UNSPECIFIED.,.F.,.F.,(4,2,4),(-0.0999913936388849,-0.0500013329569702,
-4.68222846500675E-6),.UNSPECIFIED.);
#862=B_SPLINE_CURVE_WITH_KNOTS('',3,(#37322,#37323,#37324,#37325,#37326,
#37327),.UNSPECIFIED.,.F.,.F.,(4,2,4),(0.000679649455705054,0.0157748102346675,
0.0307661125813358),.UNSPECIFIED.);
#863=B_SPLINE_CURVE_WITH_KNOTS('',3,(#37328,#37329,#37330,#37331,#37332,
#37333),.UNSPECIFIED.,.F.,.F.,(4,2,4),(4.78528932733694E-5,0.047856719715927,
0.0963109409074384),.UNSPECIFIED.);
#864=B_SPLINE_CURVE_WITH_KNOTS('',3,(#37337,#37338,#37339,#37340,#37341,
#37342,#37343,#37344,#37345,#37346,#37347,#37348,#37349,#37350,#37351,#37352,
#37353),.UNSPECIFIED.,.F.,.F.,(4,1,1,1,1,1,1,1,1,1,1,1,1,1,4),(0.,0.125,
0.1875,0.25,0.3125,0.375,0.5,0.625,0.6875,0.71875,0.75,0.78125,0.8125,0.875,
1.),.UNSPECIFIED.);
#865=B_SPLINE_CURVE_WITH_KNOTS('',3,(#37355,#37356,#37357,#37358,#37359,
#37360,#37361,#37362),.UNSPECIFIED.,.F.,.F.,(4,2,2,4),(0.725687494856636,
0.750372622948823,0.818321739027402,0.830322368571011),.UNSPECIFIED.);
#866=B_SPLINE_CURVE_WITH_KNOTS('',3,(#37364,#37365,#37366,#37367),
 .UNSPECIFIED.,.F.,.F.,(4,4),(-1.14929610836797,-1.05359988011008),
 .UNSPECIFIED.);
#867=B_SPLINE_CURVE_WITH_KNOTS('',3,(#37369,#37370,#37371,#37372,#37373,
#37374,#37375,#37376,#37377,#37378,#37379,#37380,#37381,#37382,#37383,#37384,
#37385),.UNSPECIFIED.,.F.,.F.,(4,1,1,1,1,1,1,1,1,1,1,1,1,1,4),(0.,0.125,
0.1875,0.25,0.3125,0.375,0.5,0.625,0.6875,0.71875,0.75,0.78125,0.8125,0.875,
0.999999992807185),.UNSPECIFIED.);
#868=B_SPLINE_CURVE_WITH_KNOTS('',3,(#37387,#37388,#37389,#37390,#37391,
#37392,#37393,#37394,#37395,#37396,#37397,#37398,#37399,#37400,#37401,#37402,
#37403),.UNSPECIFIED.,.F.,.F.,(4,1,1,1,1,1,1,1,1,1,1,1,1,1,4),(4.6260540190425E-9,
0.125,0.1875,0.21875,0.25,0.28125,0.3125,0.375,0.5,0.625,0.6875,0.75,0.8125,
0.875,1.),.UNSPECIFIED.);
#869=B_SPLINE_CURVE_WITH_KNOTS('',3,(#37404,#37405,#37406,#37407),
 .UNSPECIFIED.,.F.,.F.,(4,4),(-1.14869222711582,-1.05773312703723),
 .UNSPECIFIED.);
#870=B_SPLINE_CURVE_WITH_KNOTS('',3,(#37411,#37412,#37413,#37414,#37415,
#37416,#37417,#37418,#37419,#37420,#37421,#37422,#37423,#37424,#37425,#37426,
#37427),.UNSPECIFIED.,.F.,.F.,(4,1,1,1,1,1,1,1,1,1,1,1,1,1,4),(0.,0.125,
0.1875,0.25,0.3125,0.375,0.5,0.625,0.6875,0.71875,0.75,0.78125,0.8125,0.875,
1.),.UNSPECIFIED.);
#871=B_SPLINE_CURVE_WITH_KNOTS('',3,(#37429,#37430,#37431,#37432,#37433,
#37434,#37435,#37436,#37437,#37438,#37439,#37440,#37441,#37442,#37443,#37444,
#37445,#37446,#37447,#37448,#37449),.UNSPECIFIED.,.F.,.F.,(4,1,1,1,1,1,
1,1,1,1,1,1,1,1,1,1,1,1,4),(1.38893867511916E-7,0.03125,0.0625,0.125,0.1875,
0.21875,0.25,0.28125,0.3125,0.375,0.5,0.625,0.6875,0.71875,0.75,0.78125,
0.8125,0.875,1.),.UNSPECIFIED.);
#872=B_SPLINE_CURVE_WITH_KNOTS('',3,(#37451,#37452,#37453,#37454),
 .UNSPECIFIED.,.F.,.F.,(4,4),(-1.13334392424363,-1.03901243078379),
 .UNSPECIFIED.);
#873=B_SPLINE_CURVE_WITH_KNOTS('',3,(#37456,#37457,#37458,#37459,#37460,
#37461,#37462,#37463,#37464,#37465,#37466,#37467,#37468,#37469,#37470,#37471,
#37472),.UNSPECIFIED.,.F.,.F.,(4,1,1,1,1,1,1,1,1,1,1,1,1,1,4),(0.,0.125,
0.1875,0.25,0.3125,0.375,0.5,0.625,0.6875,0.71875,0.75,0.78125,0.8125,0.875,
1.),.UNSPECIFIED.);
#874=B_SPLINE_CURVE_WITH_KNOTS('',3,(#37474,#37475,#37476,#37477,#37478,
#37479,#37480,#37481,#37482,#37483,#37484,#37485,#37486,#37487,#37488,#37489,
#37490,#37491,#37492),.UNSPECIFIED.,.F.,.F.,(4,1,1,1,1,1,1,1,1,1,1,1,1,
1,1,1,4),(0.,0.125,0.1875,0.21875,0.25,0.28125,0.3125,0.375,0.5,0.625,0.6875,
0.71875,0.75,0.78125,0.8125,0.875,1.),.UNSPECIFIED.);
#875=B_SPLINE_CURVE_WITH_KNOTS('',3,(#37493,#37494,#37495,#37496),
 .UNSPECIFIED.,.F.,.F.,(4,4),(-1.14029447472564,-1.04889589827956),
 .UNSPECIFIED.);
#876=B_SPLINE_CURVE_WITH_KNOTS('',3,(#37500,#37501,#37502,#37503,#37504,
#37505,#37506,#37507,#37508,#37509,#37510,#37511,#37512,#37513,#37514,#37515,
#37516,#37517,#37518,#37519,#37520,#37521,#37522,#37523,#37524,#37525,#37526,
#37527,#37528,#37529,#37530,#37531,#37532,#37533,#37534,#37535,#37536,#37537,
#37538,#37539,#37540,#37541,#37542,#37543,#37544,#37545,#37546,#37547,#37548),
 .UNSPECIFIED.,.F.,.F.,(4,3,3,3,3,3,3,3,3,3,3,3,3,3,3,3,4),(0.,0.125,0.1875,
0.21875,0.25,0.28125,0.3125,0.375,0.5,0.625,0.6875,0.71875,0.75,0.78125,
0.8125,0.875,1.),.UNSPECIFIED.);
#877=B_SPLINE_CURVE_WITH_KNOTS('',3,(#37550,#37551,#37552,#37553,#37554,
#37555,#37556,#37557,#37558,#37559,#37560,#37561,#37562,#37563,#37564,#37565,
#37566,#37567,#37568),.UNSPECIFIED.,.F.,.F.,(4,1,1,1,1,1,1,1,1,1,1,1,1,
1,1,1,4),(2.20369844643671E-7,0.125000167295231,0.187500155345571,0.218750149370742,
0.250000143395912,0.281250137421082,0.312500131446253,0.375000119496593,
0.500000095597275,0.625000071697956,0.687500059748297,0.718750053773467,
0.750000047798637,0.781250041823808,0.812500035848978,0.875000023899319,
1.),.UNSPECIFIED.);
#878=B_SPLINE_CURVE_WITH_KNOTS('',3,(#37570,#37571,#37572,#37573),
 .UNSPECIFIED.,.F.,.F.,(4,4),(-1.13396995922952,-1.03919754738596),
 .UNSPECIFIED.);
#879=B_SPLINE_CURVE_WITH_KNOTS('',3,(#37575,#37576,#37577,#37578,#37579,
#37580,#37581,#37582,#37583,#37584,#37585,#37586,#37587,#37588,#37589,#37590,
#37591,#37592,#37593),.UNSPECIFIED.,.F.,.F.,(4,1,1,1,1,1,1,1,1,1,1,1,1,
1,1,1,4),(0.,0.125,0.1875,0.21875,0.25,0.28125,0.3125,0.375,0.5,0.625,0.6875,
0.71875,0.75,0.78125,0.8125,0.875,1.),.UNSPECIFIED.);
#880=B_SPLINE_CURVE_WITH_KNOTS('',3,(#37595,#37596,#37597,#37598,#37599,
#37600,#37601,#37602,#37603,#37604,#37605,#37606,#37607,#37608,#37609,#37610,
#37611,#37612,#37613,#37614,#37615,#37616,#37617,#37618,#37619,#37620,#37621,
#37622,#37623,#37624,#37625,#37626,#37627,#37628,#37629,#37630,#37631,#37632,
#37633,#37634,#37635,#37636,#37637,#37638,#37639,#37640,#37641,#37642,#37643),
 .UNSPECIFIED.,.F.,.F.,(4,3,3,3,3,3,3,3,3,3,3,3,3,3,3,3,4),(3.09854816786387E-7,
0.125000271122965,0.187500251757039,0.218750242074076,0.250000232391113,
0.28125022270815,0.312500213025186,0.37500019365926,0.500000154927408,0.625000116195556,
0.68750009682963,0.718750087146667,0.750000077463704,0.781250067780741,
0.812500058097778,0.875000038731852,1.),.UNSPECIFIED.);
#881=B_SPLINE_CURVE_WITH_KNOTS('',3,(#37644,#37645,#37646,#37647),
 .UNSPECIFIED.,.F.,.F.,(4,4),(-1.13870654772476,-1.04617847256649),
 .UNSPECIFIED.);
#882=B_SPLINE_CURVE_WITH_KNOTS('',3,(#37651,#37652,#37653,#37654,#37655,
#37656,#37657,#37658,#37659,#37660,#37661,#37662,#37663,#37664,#37665,#37666,
#37667,#37668,#37669,#37670,#37671,#37672,#37673,#37674,#37675,#37676,#37677,
#37678,#37679,#37680,#37681,#37682,#37683,#37684,#37685,#37686,#37687,#37688,
#37689,#37690,#37691,#37692,#37693,#37694,#37695,#37696,#37697,#37698,#37699),
 .UNSPECIFIED.,.F.,.F.,(4,3,3,3,3,3,3,3,3,3,3,3,3,3,3,3,4),(0.,0.125,0.1875,
0.21875,0.25,0.28125,0.3125,0.375,0.5,0.625,0.6875,0.71875,0.75,0.78125,
0.8125,0.875,1.),.UNSPECIFIED.);
#883=B_SPLINE_CURVE_WITH_KNOTS('',3,(#37701,#37702,#37703,#37704,#37705,
#37706,#37707,#37708,#37709,#37710,#37711,#37712,#37713,#37714,#37715,#37716,
#37717,#37718,#37719),.UNSPECIFIED.,.F.,.F.,(4,1,1,1,1,1,1,1,1,1,1,1,1,
1,1,1,4),(1.47023832197186E-7,0.125,0.1875,0.21875,0.25,0.28125,0.3125,
0.375,0.5,0.625,0.6875,0.71875,0.75,0.78125,0.8125,0.875,1.),
 .UNSPECIFIED.);
#884=B_SPLINE_CURVE_WITH_KNOTS('',3,(#37721,#37722,#37723,#37724),
 .UNSPECIFIED.,.F.,.F.,(4,4),(-1.13203448436853,-1.03921975837767),
 .UNSPECIFIED.);
#885=B_SPLINE_CURVE_WITH_KNOTS('',3,(#37726,#37727,#37728,#37729,#37730,
#37731,#37732,#37733,#37734,#37735,#37736,#37737,#37738,#37739,#37740,#37741,
#37742,#37743,#37744,#37745,#37746,#37747,#37748,#37749,#37750,#37751,#37752,
#37753,#37754,#37755,#37756,#37757,#37758,#37759,#37760,#37761,#37762,#37763,
#37764,#37765,#37766,#37767,#37768,#37769,#37770,#37771,#37772,#37773,#37774),
 .UNSPECIFIED.,.F.,.F.,(4,3,3,3,3,3,3,3,3,3,3,3,3,3,3,3,4),(0.,0.125,0.1875,
0.21875,0.25,0.28125,0.3125,0.375,0.5,0.625,0.6875,0.71875,0.75,0.78125,
0.8125,0.875,1.),.UNSPECIFIED.);
#886=B_SPLINE_CURVE_WITH_KNOTS('',3,(#37776,#37777,#37778,#37779,#37780,
#37781,#37782,#37783,#37784,#37785,#37786,#37787,#37788,#37789,#37790,#37791,
#37792,#37793,#37794,#37795,#37796,#37797,#37798,#37799,#37800,#37801,#37802,
#37803,#37804,#37805,#37806,#37807,#37808,#37809,#37810,#37811,#37812,#37813,
#37814,#37815,#37816,#37817,#37818,#37819,#37820,#37821,#37822,#37823,#37824,
#37825,#37826,#37827,#37828,#37829,#37830,#37831,#37832,#37833,#37834,#37835,
#37836,#37837,#37838,#37839),.UNSPECIFIED.,.F.,.F.,(4,3,3,3,3,3,3,3,3,3,
3,3,3,3,3,3,3,3,3,3,3,4),(0.,0.0078125,0.015625,0.03125,0.0625,0.09375,
0.125,0.1875,0.21875,0.25,0.28125,0.3125,0.375,0.5,0.625,0.6875,0.71875,
0.75,0.78125,0.8125,0.875,1.),.UNSPECIFIED.);
#887=B_SPLINE_CURVE_WITH_KNOTS('',3,(#37840,#37841,#37842,#37843),
 .UNSPECIFIED.,.F.,.F.,(4,4),(-1.14623761520631,-1.05526208703702),
 .UNSPECIFIED.);
#888=B_SPLINE_CURVE_WITH_KNOTS('',3,(#37847,#37848,#37849,#37850,#37851,
#37852,#37853,#37854,#37855,#37856,#37857,#37858,#37859,#37860,#37861,#37862,
#37863),.UNSPECIFIED.,.F.,.F.,(4,1,1,1,1,1,1,1,1,1,1,1,1,1,4),(0.,0.125,
0.1875,0.25,0.3125,0.375,0.5,0.625,0.6875,0.71875,0.75,0.78125,0.8125,0.875,
1.),.UNSPECIFIED.);
#889=B_SPLINE_CURVE_WITH_KNOTS('',3,(#37865,#37866,#37867,#37868,#37869,
#37870,#37871,#37872,#37873,#37874,#37875,#37876,#37877,#37878,#37879,#37880,
#37881,#37882,#37883,#37884),.UNSPECIFIED.,.F.,.F.,(4,1,1,1,1,1,1,1,1,1,
1,1,1,1,1,1,1,4),(1.32416122177584E-7,0.015625,0.03125,0.0625,0.125,0.1875,
0.21875,0.25,0.28125,0.3125,0.375,0.5,0.625,0.6875,0.75,0.8125,0.875,1.),
 .UNSPECIFIED.);
#890=B_SPLINE_CURVE_WITH_KNOTS('',3,(#37886,#37887,#37888,#37889),
 .UNSPECIFIED.,.F.,.F.,(4,4),(-1.14630381292734,-1.04873232335616),
 .UNSPECIFIED.);
#891=B_SPLINE_CURVE_WITH_KNOTS('',3,(#37891,#37892,#37893,#37894,#37895,
#37896,#37897,#37898,#37899,#37900,#37901,#37902,#37903,#37904,#37905,#37906,
#37907,#37908),.UNSPECIFIED.,.F.,.F.,(4,1,1,1,1,1,1,1,1,1,1,1,1,1,1,4),
(0.,0.125,0.1875,0.25,0.3125,0.375,0.5,0.625,0.6875,0.71875,0.75,0.78125,
0.8125,0.875,0.9375,0.999999980241856),.UNSPECIFIED.);
#892=B_SPLINE_CURVE_WITH_KNOTS('',3,(#37910,#37911,#37912,#37913,#37914,
#37915,#37916,#37917,#37918,#37919,#37920,#37921,#37922,#37923,#37924,#37925,
#37926),.UNSPECIFIED.,.F.,.F.,(4,1,1,1,1,1,1,1,1,1,1,1,1,1,4),(2.27348631753915E-8,
0.125,0.1875,0.21875,0.25,0.28125,0.3125,0.375,0.5,0.625,0.6875,0.75,0.8125,
0.875,1.),.UNSPECIFIED.);
#893=B_SPLINE_CURVE_WITH_KNOTS('',3,(#37927,#37928,#37929,#37930),
 .UNSPECIFIED.,.F.,.F.,(4,4),(-1.13789426893553,-1.04477626914527),
 .UNSPECIFIED.);
#894=B_SPLINE_CURVE_WITH_KNOTS('',3,(#37934,#37935,#37936,#37937,#37938,
#37939,#37940,#37941,#37942,#37943,#37944,#37945,#37946,#37947,#37948,#37949,
#37950,#37951,#37952),.UNSPECIFIED.,.F.,.F.,(4,1,1,1,1,1,1,1,1,1,1,1,1,
1,1,1,4),(0.,0.125,0.1875,0.21875,0.25,0.28125,0.3125,0.375,0.5,0.625,0.6875,
0.71875,0.75,0.78125,0.8125,0.875,1.),.UNSPECIFIED.);
#895=B_SPLINE_CURVE_WITH_KNOTS('',3,(#37954,#37955,#37956,#37957,#37958,
#37959,#37960,#37961,#37962,#37963,#37964,#37965,#37966,#37967,#37968,#37969,
#37970,#37971,#37972,#37973),.UNSPECIFIED.,.F.,.F.,(4,1,1,1,1,1,1,1,1,1,
1,1,1,1,1,1,1,4),(2.05561699507991E-7,0.0625,0.125,0.1875,0.21875,0.25,
0.28125,0.3125,0.375,0.5,0.625,0.6875,0.71875,0.75,0.78125,0.8125,0.875,
1.),.UNSPECIFIED.);
#896=B_SPLINE_CURVE_WITH_KNOTS('',3,(#37975,#37976,#37977,#37978),
 .UNSPECIFIED.,.F.,.F.,(4,4),(-1.138991292616,-1.0479930898435),
 .UNSPECIFIED.);
#897=B_SPLINE_CURVE_WITH_KNOTS('',3,(#37980,#37981,#37982,#37983,#37984,
#37985,#37986,#37987,#37988,#37989,#37990,#37991,#37992,#37993,#37994,#37995,
#37996,#37997,#37998,#37999,#38000,#38001,#38002,#38003,#38004,#38005,#38006,
#38007,#38008,#38009,#38010,#38011,#38012,#38013,#38014,#38015,#38016,#38017,
#38018,#38019,#38020,#38021,#38022,#38023,#38024,#38025,#38026,#38027,#38028,
#38029,#38030,#38031),.UNSPECIFIED.,.F.,.F.,(4,3,3,3,3,3,3,3,3,3,3,3,3,
3,3,3,3,4),(0.,0.125,0.1875,0.21875,0.25,0.28125,0.3125,0.375,0.5,0.625,
0.6875,0.71875,0.75,0.78125,0.8125,0.875,0.9375,1.),.UNSPECIFIED.);
#898=B_SPLINE_CURVE_WITH_KNOTS('',3,(#38033,#38034,#38035,#38036,#38037,
#38038,#38039,#38040,#38041,#38042,#38043,#38044,#38045,#38046,#38047,#38048,
#38049,#38050,#38051,#38052,#38053,#38054,#38055,#38056,#38057,#38058,#38059,
#38060,#38061,#38062,#38063,#38064,#38065,#38066,#38067,#38068,#38069,#38070,
#38071,#38072,#38073,#38074,#38075,#38076,#38077,#38078,#38079,#38080,#38081),
 .UNSPECIFIED.,.F.,.F.,(4,3,3,3,3,3,3,3,3,3,3,3,3,3,3,3,4),(0.,0.125,0.1875,
0.21875,0.25,0.28125,0.3125,0.375,0.5,0.625,0.6875,0.71875,0.75,0.78125,
0.8125,0.875,1.),.UNSPECIFIED.);
#899=B_SPLINE_CURVE_WITH_KNOTS('',3,(#38082,#38083,#38084,#38085),
 .UNSPECIFIED.,.F.,.F.,(4,4),(-1.15404648390436,-1.06229819758988),
 .UNSPECIFIED.);
#900=B_SPLINE_CURVE_WITH_KNOTS('',3,(#38089,#38090,#38091,#38092,#38093,
#38094,#38095,#38096,#38097,#38098,#38099,#38100,#38101,#38102,#38103,#38104,
#38105,#38106),.UNSPECIFIED.,.F.,.F.,(4,1,1,1,1,1,1,1,1,1,1,1,1,1,1,4),
(0.,0.125,0.1875,0.25,0.3125,0.375,0.4375,0.5,0.625,0.6875,0.71875,0.75,
0.78125,0.8125,0.875,1.),.UNSPECIFIED.);
#901=B_SPLINE_CURVE_WITH_KNOTS('',3,(#38108,#38109,#38110,#38111,#38112,
#38113,#38114,#38115,#38116,#38117,#38118,#38119,#38120,#38121,#38122,#38123,
#38124,#38125,#38126,#38127),.UNSPECIFIED.,.F.,.F.,(4,1,1,1,1,1,1,1,1,1,
1,1,1,1,1,1,1,4),(2.17724807565861E-7,0.03125,0.0625,0.125,0.1875,0.21875,
0.25,0.28125,0.3125,0.375,0.5,0.5625,0.625,0.6875,0.75,0.8125,0.875,0.999999262331069),
 .UNSPECIFIED.);
#902=B_SPLINE_CURVE_WITH_KNOTS('',3,(#38129,#38130,#38131,#38132),
 .UNSPECIFIED.,.F.,.F.,(4,4),(-1.14332564091168,-1.05240155346319),
 .UNSPECIFIED.);
#903=B_SPLINE_CURVE_WITH_KNOTS('',3,(#38134,#38135,#38136,#38137,#38138,
#38139,#38140,#38141,#38142,#38143,#38144,#38145,#38146,#38147,#38148,#38149,
#38150,#38151,#38152,#38153),.UNSPECIFIED.,.F.,.F.,(4,1,1,1,1,1,1,1,1,1,
1,1,1,1,1,1,1,4),(0.,0.125,0.1875,0.25,0.3125,0.375,0.4375,0.5,0.625,0.6875,
0.71875,0.75,0.78125,0.8125,0.875,0.9375,0.96875,0.999999826165719),
 .UNSPECIFIED.);
#904=B_SPLINE_CURVE_WITH_KNOTS('',3,(#38155,#38156,#38157,#38158,#38159,
#38160,#38161,#38162,#38163,#38164,#38165,#38166,#38167,#38168,#38169,#38170,
#38171,#38172),.UNSPECIFIED.,.F.,.F.,(4,1,1,1,1,1,1,1,1,1,1,1,1,1,1,4),
(0.,0.125,0.1875,0.21875,0.25,0.28125,0.3125,0.375,0.5,0.5625,0.625,0.6875,
0.75,0.8125,0.875,1.),.UNSPECIFIED.);
#905=B_SPLINE_CURVE_WITH_KNOTS('',3,(#38173,#38174,#38175,#38176),
 .UNSPECIFIED.,.F.,.F.,(4,4),(-1.168912721115,-1.07795603507789),
 .UNSPECIFIED.);
#906=B_SPLINE_CURVE_WITH_KNOTS('',3,(#38180,#38181,#38182,#38183,#38184,
#38185,#38186,#38187,#38188,#38189,#38190,#38191,#38192,#38193,#38194,#38195,
#38196,#38197,#38198),.UNSPECIFIED.,.F.,.F.,(4,1,1,1,1,1,1,1,1,1,1,1,1,
1,1,1,4),(0.,0.125,0.1875,0.21875,0.25,0.28125,0.3125,0.375,0.5,0.625,0.6875,
0.71875,0.75,0.78125,0.8125,0.875,1.),.UNSPECIFIED.);
#907=B_SPLINE_CURVE_WITH_KNOTS('',3,(#38200,#38201,#38202,#38203,#38204,
#38205,#38206,#38207,#38208,#38209,#38210,#38211,#38212,#38213,#38214,#38215,
#38216,#38217,#38218,#38219,#38220,#38221,#38222,#38223),.UNSPECIFIED.,
 .F.,.F.,(4,1,1,1,1,1,1,1,1,1,1,1,1,1,1,1,1,1,1,1,1,4),(1.6543685732775E-6,
0.0078125,0.015625,0.03125,0.0625,0.09375,0.125,0.1875,0.21875,0.25,0.28125,
0.3125,0.375,0.5,0.625,0.6875,0.71875,0.75,0.78125,0.8125,0.875,1.),
 .UNSPECIFIED.);
#908=B_SPLINE_CURVE_WITH_KNOTS('',3,(#38225,#38226,#38227,#38228),
 .UNSPECIFIED.,.F.,.F.,(4,4),(-1.1365411740379,-1.04546711889777),
 .UNSPECIFIED.);
#909=B_SPLINE_CURVE_WITH_KNOTS('',3,(#38230,#38231,#38232,#38233,#38234,
#38235,#38236,#38237,#38238,#38239,#38240,#38241,#38242,#38243,#38244,#38245,
#38246,#38247,#38248,#38249,#38250,#38251,#38252,#38253,#38254,#38255,#38256,
#38257,#38258,#38259,#38260,#38261,#38262,#38263,#38264,#38265,#38266,#38267,
#38268,#38269,#38270,#38271,#38272,#38273,#38274,#38275,#38276,#38277,#38278),
 .UNSPECIFIED.,.F.,.F.,(4,3,3,3,3,3,3,3,3,3,3,3,3,3,3,3,4),(0.,0.125,0.1875,
0.21875,0.25,0.28125,0.3125,0.375,0.5,0.625,0.6875,0.71875,0.75,0.78125,
0.8125,0.875,1.),.UNSPECIFIED.);
#910=B_SPLINE_CURVE_WITH_KNOTS('',3,(#38280,#38281,#38282,#38283,#38284,
#38285,#38286,#38287,#38288,#38289,#38290,#38291,#38292,#38293,#38294,#38295,
#38296,#38297,#38298,#38299,#38300,#38301,#38302,#38303,#38304,#38305,#38306,
#38307,#38308,#38309,#38310,#38311,#38312,#38313,#38314,#38315,#38316,#38317,
#38318,#38319,#38320,#38321,#38322,#38323,#38324,#38325,#38326,#38327,#38328),
 .UNSPECIFIED.,.F.,.F.,(4,3,3,3,3,3,3,3,3,3,3,3,3,3,3,3,4),(0.,0.125,0.1875,
0.21875,0.25,0.28125,0.3125,0.375,0.5,0.625,0.6875,0.71875,0.75,0.78125,
0.8125,0.875,1.),.UNSPECIFIED.);
#911=B_SPLINE_CURVE_WITH_KNOTS('',3,(#38329,#38330,#38331,#38332),
 .UNSPECIFIED.,.F.,.F.,(4,4),(-1.14644022259357,-1.05547256732452),
 .UNSPECIFIED.);
#912=B_SPLINE_CURVE_WITH_KNOTS('',3,(#38336,#38337,#38338,#38339,#38340,
#38341,#38342,#38343,#38344,#38345,#38346,#38347,#38348,#38349,#38350,#38351,
#38352),.UNSPECIFIED.,.F.,.F.,(4,1,1,1,1,1,1,1,1,1,1,1,1,1,4),(0.,0.125,
0.1875,0.25,0.3125,0.375,0.5,0.625,0.6875,0.71875,0.75,0.78125,0.8125,0.875,
1.),.UNSPECIFIED.);
#913=B_SPLINE_CURVE_WITH_KNOTS('',3,(#38354,#38355,#38356,#38357,#38358,
#38359,#38360,#38361,#38362,#38363,#38364,#38365,#38366,#38367,#38368,#38369,
#38370,#38371,#38372,#38373),.UNSPECIFIED.,.F.,.F.,(4,1,1,1,1,1,1,1,1,1,
1,1,1,1,1,1,1,4),(7.22897047608602E-8,0.015625,0.03125,0.0625,0.125,0.1875,
0.21875,0.25,0.28125,0.3125,0.375,0.5,0.625,0.6875,0.75,0.8125,0.875,1.),
 .UNSPECIFIED.);
#914=B_SPLINE_CURVE_WITH_KNOTS('',3,(#38375,#38376,#38377,#38378),
 .UNSPECIFIED.,.F.,.F.,(4,4),(-1.14915858321821,-1.05511789649031),
 .UNSPECIFIED.);
#915=B_SPLINE_CURVE_WITH_KNOTS('',3,(#38380,#38381,#38382,#38383,#38384,
#38385,#38386,#38387,#38388,#38389,#38390,#38391,#38392,#38393,#38394,#38395,
#38396,#38397,#38398),.UNSPECIFIED.,.F.,.F.,(4,1,1,1,1,1,1,1,1,1,1,1,1,
1,1,1,4),(0.,0.125,0.1875,0.25,0.3125,0.375,0.5,0.625,0.6875,0.71875,0.75,
0.78125,0.8125,0.875,0.9375,0.96875,0.999999982337592),.UNSPECIFIED.);
#916=B_SPLINE_CURVE_WITH_KNOTS('',3,(#38400,#38401,#38402,#38403,#38404,
#38405,#38406,#38407,#38408,#38409,#38410,#38411,#38412,#38413,#38414,#38415,
#38416),.UNSPECIFIED.,.F.,.F.,(4,1,1,1,1,1,1,1,1,1,1,1,1,1,4),(1.83406697454463E-8,
0.125,0.1875,0.21875,0.25,0.28125,0.3125,0.375,0.5,0.625,0.6875,0.75,0.8125,
0.875,1.),.UNSPECIFIED.);
#917=B_SPLINE_CURVE_WITH_KNOTS('',3,(#38417,#38418,#38419,#38420),
 .UNSPECIFIED.,.F.,.F.,(4,4),(-1.14293348037966,-1.05189856760605),
 .UNSPECIFIED.);
#918=B_SPLINE_CURVE_WITH_KNOTS('',3,(#38424,#38425,#38426,#38427,#38428,
#38429,#38430,#38431,#38432,#38433,#38434,#38435,#38436,#38437,#38438,#38439,
#38440),.UNSPECIFIED.,.F.,.F.,(4,1,1,1,1,1,1,1,1,1,1,1,1,1,4),(0.,0.125,
0.1875,0.25,0.3125,0.375,0.5,0.625,0.6875,0.71875,0.75,0.78125,0.8125,0.875,
1.),.UNSPECIFIED.);
#919=B_SPLINE_CURVE_WITH_KNOTS('',3,(#38442,#38443,#38444,#38445,#38446,
#38447,#38448,#38449,#38450,#38451,#38452,#38453,#38454,#38455,#38456,#38457,
#38458,#38459,#38460),.UNSPECIFIED.,.F.,.F.,(4,1,1,1,1,1,1,1,1,1,1,1,1,
1,1,1,4),(4.59429913662085E-8,0.03125,0.0625,0.125,0.1875,0.21875,0.25,
0.28125,0.3125,0.375,0.5,0.625,0.6875,0.75,0.8125,0.875,1.),
 .UNSPECIFIED.);
#920=B_SPLINE_CURVE_WITH_KNOTS('',3,(#38462,#38463,#38464,#38465),
 .UNSPECIFIED.,.F.,.F.,(4,4),(-1.1400229377893,-1.04896134555146),
 .UNSPECIFIED.);
#921=B_SPLINE_CURVE_WITH_KNOTS('',3,(#38467,#38468,#38469,#38470,#38471,
#38472,#38473,#38474,#38475,#38476,#38477,#38478,#38479,#38480,#38481,#38482,
#38483,#38484),.UNSPECIFIED.,.F.,.F.,(4,1,1,1,1,1,1,1,1,1,1,1,1,1,1,4),
(0.,0.125,0.1875,0.25,0.3125,0.375,0.5,0.625,0.6875,0.71875,0.75,0.78125,
0.8125,0.875,0.9375,0.999999974036836),.UNSPECIFIED.);
#922=B_SPLINE_CURVE_WITH_KNOTS('',3,(#38486,#38487,#38488,#38489,#38490,
#38491,#38492,#38493,#38494,#38495,#38496,#38497,#38498,#38499,#38500,#38501,
#38502),.UNSPECIFIED.,.F.,.F.,(4,1,1,1,1,1,1,1,1,1,1,1,1,1,4),(1.69179276891372E-8,
0.125,0.1875,0.21875,0.25,0.28125,0.3125,0.375,0.5,0.625,0.6875,0.75,0.8125,
0.875,1.),.UNSPECIFIED.);
#923=B_SPLINE_CURVE_WITH_KNOTS('',3,(#38503,#38504,#38505,#38506),
 .UNSPECIFIED.,.F.,.F.,(4,4),(-1.14119404467057,-1.05000176302202),
 .UNSPECIFIED.);
#924=B_SPLINE_CURVE_WITH_KNOTS('',3,(#38510,#38511,#38512,#38513,#38514,
#38515,#38516,#38517,#38518,#38519,#38520,#38521,#38522,#38523,#38524,#38525,
#38526),.UNSPECIFIED.,.F.,.F.,(4,1,1,1,1,1,1,1,1,1,1,1,1,1,4),(0.,0.125,
0.1875,0.25,0.3125,0.375,0.5,0.625,0.6875,0.71875,0.75,0.78125,0.8125,0.875,
0.9999999591332),.UNSPECIFIED.);
#925=B_SPLINE_CURVE_WITH_KNOTS('',3,(#38528,#38529,#38530,#38531,#38532,
#38533,#38534,#38535,#38536,#38537,#38538,#38539,#38540,#38541,#38542,#38543,
#38544,#38545,#38546,#38547),.UNSPECIFIED.,.F.,.F.,(4,1,1,1,1,1,1,1,1,1,
1,1,1,1,1,1,1,4),(0.,0.015625,0.03125,0.0625,0.125,0.1875,0.21875,0.25,
0.28125,0.3125,0.375,0.5,0.625,0.6875,0.75,0.8125,0.875,1.),
 .UNSPECIFIED.);
#926=B_SPLINE_CURVE_WITH_KNOTS('',3,(#38549,#38550,#38551,#38552),
 .UNSPECIFIED.,.F.,.F.,(4,4),(-1.14875038807723,-1.05593562205532),
 .UNSPECIFIED.);
#927=B_SPLINE_CURVE_WITH_KNOTS('',3,(#38554,#38555,#38556,#38557,#38558,
#38559,#38560,#38561,#38562,#38563,#38564,#38565,#38566,#38567,#38568,#38569,
#38570,#38571,#38572),.UNSPECIFIED.,.F.,.F.,(4,1,1,1,1,1,1,1,1,1,1,1,1,
1,1,1,4),(0.,0.125,0.1875,0.25,0.3125,0.375,0.5,0.625,0.6875,0.71875,0.75,
0.78125,0.8125,0.875,0.9375,0.96875,0.999999969096218),.UNSPECIFIED.);
#928=B_SPLINE_CURVE_WITH_KNOTS('',3,(#38574,#38575,#38576,#38577,#38578,
#38579,#38580,#38581,#38582,#38583,#38584,#38585,#38586,#38587,#38588,#38589,
#38590),.UNSPECIFIED.,.F.,.F.,(4,1,1,1,1,1,1,1,1,1,1,1,1,1,4),(1.69694494032564E-8,
0.125,0.1875,0.21875,0.25,0.28125,0.3125,0.375,0.5,0.625,0.6875,0.75,0.8125,
0.875,1.),.UNSPECIFIED.);
#929=B_SPLINE_CURVE_WITH_KNOTS('',3,(#38591,#38592,#38593,#38594),
 .UNSPECIFIED.,.F.,.F.,(4,4),(-1.14085663885015,-1.04963197175557),
 .UNSPECIFIED.);
#930=B_SPLINE_CURVE_WITH_KNOTS('',3,(#38598,#38599,#38600,#38601,#38602,
#38603,#38604,#38605,#38606,#38607,#38608,#38609,#38610,#38611,#38612,#38613,
#38614),.UNSPECIFIED.,.F.,.F.,(4,1,1,1,1,1,1,1,1,1,1,1,1,1,4),(0.,0.125,
0.1875,0.25,0.3125,0.375,0.5,0.625,0.6875,0.71875,0.75,0.78125,0.8125,0.875,
0.999999967427316),.UNSPECIFIED.);
#931=B_SPLINE_CURVE_WITH_KNOTS('',3,(#38616,#38617,#38618,#38619,#38620,
#38621,#38622,#38623,#38624,#38625,#38626,#38627,#38628,#38629,#38630,#38631,
#38632,#38633,#38634,#38635),.UNSPECIFIED.,.F.,.F.,(4,1,1,1,1,1,1,1,1,1,
1,1,1,1,1,1,1,4),(0.,0.015625,0.03125,0.0625,0.125,0.1875,0.21875,0.25,
0.28125,0.3125,0.375,0.5,0.625,0.6875,0.75,0.8125,0.875,1.),
 .UNSPECIFIED.);
#932=B_SPLINE_CURVE_WITH_KNOTS('',3,(#38637,#38638,#38639,#38640),
 .UNSPECIFIED.,.F.,.F.,(4,4),(-1.14024200034905,-1.04934844889581),
 .UNSPECIFIED.);
#933=B_SPLINE_CURVE_WITH_KNOTS('',3,(#38642,#38643,#38644,#38645,#38646,
#38647,#38648,#38649,#38650,#38651,#38652,#38653,#38654,#38655,#38656,#38657,
#38658,#38659),.UNSPECIFIED.,.F.,.F.,(4,1,1,1,1,1,1,1,1,1,1,1,1,1,1,4),
(0.,0.125,0.1875,0.25,0.3125,0.375,0.5,0.625,0.6875,0.71875,0.75,0.78125,
0.8125,0.875,0.9375,0.99999998105284),.UNSPECIFIED.);
#934=B_SPLINE_CURVE_WITH_KNOTS('',3,(#38661,#38662,#38663,#38664,#38665,
#38666,#38667,#38668,#38669,#38670,#38671,#38672,#38673,#38674,#38675,#38676,
#38677),.UNSPECIFIED.,.F.,.F.,(4,1,1,1,1,1,1,1,1,1,1,1,1,1,4),(2.32949966596595E-8,
0.125,0.1875,0.21875,0.25,0.28125,0.3125,0.375,0.5,0.625,0.6875,0.75,0.8125,
0.875,1.),.UNSPECIFIED.);
#935=B_SPLINE_CURVE_WITH_KNOTS('',3,(#38678,#38679,#38680,#38681),
 .UNSPECIFIED.,.F.,.F.,(4,4),(-1.15396147913084,-1.0581629542817),
 .UNSPECIFIED.);
#936=B_SPLINE_CURVE_WITH_KNOTS('',3,(#38685,#38686,#38687,#38688,#38689,
#38690,#38691,#38692,#38693,#38694,#38695,#38696,#38697,#38698,#38699,#38700,
#38701,#38702),.UNSPECIFIED.,.F.,.F.,(4,1,1,1,1,1,1,1,1,1,1,1,1,1,1,4),
(0.,0.125,0.1875,0.25,0.3125,0.375,0.4375,0.5,0.625,0.6875,0.71875,0.75,
0.78125,0.8125,0.875,1.),.UNSPECIFIED.);
#937=B_SPLINE_CURVE_WITH_KNOTS('',3,(#38704,#38705,#38706,#38707,#38708,
#38709,#38710,#38711,#38712,#38713,#38714,#38715,#38716,#38717,#38718,#38719,
#38720,#38721,#38722,#38723,#38724),.UNSPECIFIED.,.F.,.F.,(4,1,1,1,1,1,
1,1,1,1,1,1,1,1,1,1,1,1,4),(1.76059286925808E-7,0.015625,0.03125,0.0625,
0.125,0.1875,0.21875,0.25,0.28125,0.3125,0.375,0.5,0.5625,0.625,0.6875,
0.75,0.8125,0.875,0.999999334182892),.UNSPECIFIED.);
#938=B_SPLINE_CURVE_WITH_KNOTS('',3,(#38726,#38727,#38728,#38729),
 .UNSPECIFIED.,.F.,.F.,(4,4),(-1.1418971753089,-1.05100194193717),
 .UNSPECIFIED.);
#939=B_SPLINE_CURVE_WITH_KNOTS('',3,(#38731,#38732,#38733,#38734,#38735,
#38736,#38737,#38738,#38739,#38740,#38741,#38742,#38743,#38744,#38745,#38746,
#38747,#38748,#38749,#38750,#38751),.UNSPECIFIED.,.F.,.F.,(4,1,1,1,1,1,
1,1,1,1,1,1,1,1,1,1,1,1,4),(0.,0.125,0.1875,0.25,0.3125,0.375,0.4375,0.5,
0.625,0.6875,0.71875,0.75,0.78125,0.8125,0.875,0.9375,0.96875,0.984375,
0.999999828518404),.UNSPECIFIED.);
#940=B_SPLINE_CURVE_WITH_KNOTS('',3,(#38753,#38754,#38755,#38756,#38757,
#38758,#38759,#38760,#38761,#38762,#38763,#38764,#38765,#38766,#38767,#38768,
#38769,#38770),.UNSPECIFIED.,.F.,.F.,(4,1,1,1,1,1,1,1,1,1,1,1,1,1,1,4),
(0.,0.125,0.1875,0.21875,0.25,0.28125,0.3125,0.375,0.5,0.5625,0.625,0.6875,
0.75,0.8125,0.875,1.),.UNSPECIFIED.);
#941=B_SPLINE_CURVE_WITH_KNOTS('',3,(#38771,#38772,#38773,#38774),
 .UNSPECIFIED.,.F.,.F.,(4,4),(-1.16831528067923,-1.07737821672828),
 .UNSPECIFIED.);
#942=B_SPLINE_CURVE_WITH_KNOTS('',3,(#38778,#38779,#38780,#38781,#38782,
#38783,#38784,#38785,#38786,#38787,#38788,#38789,#38790,#38791,#38792,#38793,
#38794),.UNSPECIFIED.,.F.,.F.,(4,1,1,1,1,1,1,1,1,1,1,1,1,1,4),(0.,0.125,
0.1875,0.25,0.3125,0.375,0.5,0.625,0.6875,0.71875,0.75,0.78125,0.8125,0.875,
1.),.UNSPECIFIED.);
#943=B_SPLINE_CURVE_WITH_KNOTS('',3,(#38796,#38797,#38798,#38799,#38800,
#38801,#38802,#38803,#38804,#38805,#38806,#38807,#38808,#38809,#38810,#38811,
#38812,#38813,#38814,#38815,#38816),.UNSPECIFIED.,.F.,.F.,(4,1,1,1,1,1,
1,1,1,1,1,1,1,1,1,1,1,1,4),(1.86298453241034E-7,0.015625,0.03125,0.0625,
0.125,0.1875,0.21875,0.25,0.28125,0.3125,0.375,0.5,0.5625,0.625,0.6875,
0.75,0.8125,0.875,0.999989495952636),.UNSPECIFIED.);
#944=B_SPLINE_CURVE_WITH_KNOTS('',3,(#38818,#38819,#38820,#38821,#38822,
#38823,#38824,#38825,#38826),.UNSPECIFIED.,.F.,.F.,(4,1,1,1,1,1,4),(4.64451719452503E-7,
0.25000034833879,0.375000290282325,0.50000023222586,0.625000174169395,0.75000011611293,
0.999999973113588),.UNSPECIFIED.);
#945=B_SPLINE_CURVE_WITH_KNOTS('',3,(#38828,#38829,#38830,#38831,#38832,
#38833,#38834,#38835,#38836,#38837,#38838,#38839,#38840,#38841,#38842,#38843,
#38844,#38845,#38846,#38847),.UNSPECIFIED.,.F.,.F.,(4,1,1,1,1,1,1,1,1,1,
1,1,1,1,1,1,1,4),(0.,0.125,0.1875,0.25,0.3125,0.375,0.4375,0.5,0.625,0.6875,
0.71875,0.75,0.78125,0.8125,0.875,0.9375,0.96875,0.999999724320717),
 .UNSPECIFIED.);
#946=B_SPLINE_CURVE_WITH_KNOTS('',3,(#38849,#38850,#38851,#38852,#38853,
#38854,#38855,#38856,#38857,#38858,#38859,#38860,#38861,#38862,#38863,#38864,
#38865,#38866),.UNSPECIFIED.,.F.,.F.,(4,1,1,1,1,1,1,1,1,1,1,1,1,1,1,4),
(0.,0.125,0.1875,0.21875,0.25,0.28125,0.3125,0.375,0.5,0.5625,0.625,0.6875,
0.75,0.8125,0.875,1.),.UNSPECIFIED.);
#947=B_SPLINE_CURVE_WITH_KNOTS('',3,(#38867,#38868,#38869,#38870,#38871,
#38872,#38873,#38874,#38875,#38876,#38877,#38878,#38879,#38880,#38881,#38882,
#38883,#38884,#38885,#38886,#38887,#38888,#38889,#38890,#38891),
 .UNSPECIFIED.,.F.,.F.,(4,3,3,3,3,3,3,3,4),(4.61042881515865E-6,0.181769987194646,
0.249999940419039,0.374999910628558,0.460304714091956,0.499999880838077,
0.624999851047596,0.749999821257116,0.999990442009691),.UNSPECIFIED.);
#948=B_SPLINE_CURVE_WITH_KNOTS('',3,(#38895,#38896,#38897,#38898,#38899,
#38900,#38901,#38902,#38903,#38904,#38905,#38906,#38907,#38908,#38909,#38910,
#38911),.UNSPECIFIED.,.F.,.F.,(4,1,1,1,1,1,1,1,1,1,1,1,1,1,4),(0.,0.125,
0.1875,0.25,0.3125,0.375,0.5,0.625,0.6875,0.71875,0.75,0.78125,0.8125,0.875,
0.99999998679207),.UNSPECIFIED.);
#949=B_SPLINE_CURVE_WITH_KNOTS('',3,(#38913,#38914,#38915,#38916,#38917,
#38918,#38919,#38920,#38921,#38922,#38923,#38924,#38925,#38926,#38927,#38928,
#38929,#38930),.UNSPECIFIED.,.F.,.F.,(4,1,1,1,1,1,1,1,1,1,1,1,1,1,1,4),
(8.65166934464853E-8,0.0625,0.125,0.1875,0.21875,0.25,0.28125,0.3125,0.375,
0.5,0.625,0.6875,0.75,0.8125,0.875,0.999868727025638),.UNSPECIFIED.);
#950=B_SPLINE_CURVE_WITH_KNOTS('',3,(#38932,#38933,#38934,#38935,#38936,
#38937,#38938,#38939,#38940,#38941,#38942,#38943,#38944,#38945,#38946,#38947,
#38948,#38949,#38950,#38951,#38952,#38953),.UNSPECIFIED.,.F.,.F.,(4,3,3,
3,3,3,3,4),(3.21388604215392E-7,0.250000241041453,0.375000200867878,0.500000160694302,
0.522785205722169,0.625000120520727,0.750000080347151,0.994571406786842),
 .UNSPECIFIED.);
#951=B_SPLINE_CURVE_WITH_KNOTS('',3,(#38955,#38956,#38957,#38958,#38959,
#38960,#38961,#38962),.UNSPECIFIED.,.F.,.F.,(4,2,2,4),(0.164816343944014,
0.188483278277886,0.274212380797636,0.359271548700789),.UNSPECIFIED.);
#952=B_SPLINE_CURVE_WITH_KNOTS('',3,(#38964,#38965,#38966,#38967,#38968,
#38969,#38970,#38971,#38972,#38973,#38974,#38975,#38976,#38977,#38978,#38979,
#38980),.UNSPECIFIED.,.F.,.F.,(4,1,1,1,1,1,1,1,1,1,1,1,1,1,4),(0.,0.125,
0.1875,0.21875,0.25,0.28125,0.3125,0.375,0.5,0.625,0.6875,0.75,0.8125,0.875,
0.999914460666039),.UNSPECIFIED.);
#953=B_SPLINE_CURVE_WITH_KNOTS('',3,(#38981,#38982,#38983,#38984,#38985,
#38986,#38987,#38988),.UNSPECIFIED.,.F.,.F.,(4,2,2,4),(0.000134614298568453,
0.0312571106388446,0.0597187154751761,0.108092813562148),.UNSPECIFIED.);
#954=B_SPLINE_CURVE_WITH_KNOTS('',3,(#38992,#38993,#38994,#38995,#38996,
#38997,#38998,#38999,#39000,#39001,#39002,#39003,#39004,#39005,#39006,#39007,
#39008),.UNSPECIFIED.,.F.,.F.,(4,1,1,1,1,1,1,1,1,1,1,1,1,1,4),(0.,0.125,
0.1875,0.25,0.3125,0.375,0.5,0.625,0.6875,0.71875,0.75,0.78125,0.8125,0.875,
1.),.UNSPECIFIED.);
#955=B_SPLINE_CURVE_WITH_KNOTS('',3,(#39010,#39011,#39012,#39013,#39014,
#39015,#39016,#39017,#39018,#39019,#39020,#39021,#39022,#39023,#39024,#39025,
#39026,#39027,#39028,#39029),.UNSPECIFIED.,.F.,.F.,(4,1,1,1,1,1,1,1,1,1,
1,1,1,1,1,1,1,4),(1.54060242968102E-7,0.015625,0.03125,0.0625,0.125,0.1875,
0.21875,0.25,0.28125,0.3125,0.375,0.5,0.625,0.6875,0.75,0.8125,0.875,1.),
 .UNSPECIFIED.);
#956=B_SPLINE_CURVE_WITH_KNOTS('',3,(#39031,#39032,#39033,#39034),
 .UNSPECIFIED.,.F.,.F.,(4,4),(8.88179596710341E-5,1.),.UNSPECIFIED.);
#957=B_SPLINE_CURVE_WITH_KNOTS('',3,(#39036,#39037,#39038,#39039,#39040,
#39041,#39042,#39043,#39044,#39045,#39046,#39047,#39048,#39049,#39050,#39051,
#39052),.UNSPECIFIED.,.F.,.F.,(4,1,1,1,1,1,1,1,1,1,1,1,1,1,4),(0.,0.125,
0.1875,0.25,0.3125,0.375,0.5,0.625,0.6875,0.71875,0.75,0.78125,0.8125,0.875,
0.999999976331826),.UNSPECIFIED.);
#958=B_SPLINE_CURVE_WITH_KNOTS('',3,(#39054,#39055,#39056,#39057,#39058,
#39059,#39060,#39061,#39062,#39063,#39064,#39065,#39066,#39067,#39068,#39069,
#39070),.UNSPECIFIED.,.F.,.F.,(4,1,1,1,1,1,1,1,1,1,1,1,1,1,4),(2.51851931900819E-8,
0.125,0.1875,0.21875,0.25,0.28125,0.3125,0.375,0.5,0.625,0.6875,0.75,0.8125,
0.875,1.),.UNSPECIFIED.);
#959=B_SPLINE_CURVE_WITH_KNOTS('',3,(#39071,#39072,#39073,#39074),
 .UNSPECIFIED.,.F.,.F.,(4,4),(0.,0.999911764093188),.UNSPECIFIED.);
#960=B_SPLINE_CURVE_WITH_KNOTS('',3,(#39078,#39079,#39080,#39081,#39082,
#39083,#39084,#39085),.UNSPECIFIED.,.F.,.F.,(4,2,2,4),(0.194407098287881,
0.199210339160986,0.303119902588705,0.355842009022126),.UNSPECIFIED.);
#961=B_SPLINE_CURVE_WITH_KNOTS('',3,(#39087,#39088,#39089,#39090,#39091,
#39092,#39093,#39094,#39095,#39096,#39097,#39098,#39099,#39100,#39101,#39102,
#39103,#39104,#39105),.UNSPECIFIED.,.F.,.F.,(4,3,3,3,3,3,4),(0.00444962817548656,
0.25,0.375,0.5,0.625,0.75,0.999988823500867),.UNSPECIFIED.);
#962=B_SPLINE_CURVE_WITH_KNOTS('',3,(#39107,#39108,#39109,#39110,#39111,
#39112,#39113,#39114),.UNSPECIFIED.,.F.,.F.,(4,2,2,4),(0.77443684568303,
0.777443693348876,0.895320737726667,0.914820143068275),.UNSPECIFIED.);
#963=B_SPLINE_CURVE_WITH_KNOTS('',3,(#39116,#39117,#39118,#39119,#39120,
#39121),.UNSPECIFIED.,.F.,.F.,(4,2,4),(0.586399068895315,0.598734783294216,
0.63797926634324),.UNSPECIFIED.);
#964=B_SPLINE_CURVE_WITH_KNOTS('',3,(#39123,#39124,#39125,#39126,#39127,
#39128,#39129,#39130,#39131,#39132,#39133,#39134,#39135,#39136,#39137,#39138,
#39139,#39140,#39141),.UNSPECIFIED.,.F.,.F.,(4,3,3,3,3,3,4),(3.45882434345197E-9,
0.25,0.375,0.5,0.625,0.75,1.),.UNSPECIFIED.);
#965=B_SPLINE_CURVE_WITH_KNOTS('',3,(#39142,#39143,#39144,#39145,#39146,
#39147,#39148,#39149,#39150,#39151,#39152,#39153,#39154,#39155,#39156,#39157,
#39158,#39159,#39160,#39161),.UNSPECIFIED.,.F.,.F.,(4,1,1,1,1,1,1,1,1,1,
1,1,1,1,1,1,1,4),(0.,0.125,0.1875,0.25,0.3125,0.375,0.5,0.625,0.6875,0.71875,
0.75,0.78125,0.8125,0.875,0.9375,0.96875,0.984375,0.999999989997333),
 .UNSPECIFIED.);
#966=B_SPLINE_CURVE_WITH_KNOTS('',3,(#39163,#39164,#39165,#39166),
 .UNSPECIFIED.,.F.,.F.,(4,4),(-0.0665009223849787,-0.0568933364251996),
 .UNSPECIFIED.);
#967=B_SPLINE_CURVE_WITH_KNOTS('',3,(#39167,#39168,#39169,#39170),
 .UNSPECIFIED.,.F.,.F.,(4,4),(-10.5474701151172,-10.5382467411489),
 .UNSPECIFIED.);
#968=B_SPLINE_CURVE_WITH_KNOTS('',3,(#39175,#39176,#39177,#39178,#39179,
#39180,#39181,#39182,#39183,#39184,#39185,#39186,#39187,#39188,#39189,#39190,
#39191),.UNSPECIFIED.,.F.,.F.,(4,1,1,1,1,1,1,1,1,1,1,1,1,1,4),(0.,0.125,
0.1875,0.25,0.3125,0.375,0.5,0.625,0.6875,0.71875,0.75,0.78125,0.8125,0.875,
1.),.UNSPECIFIED.);
#969=B_SPLINE_CURVE_WITH_KNOTS('',3,(#39193,#39194,#39195,#39196,#39197,
#39198,#39199,#39200),.UNSPECIFIED.,.F.,.F.,(4,2,2,4),(0.723946350565727,
0.748538685805071,0.816066681444924,0.827939780191109),.UNSPECIFIED.);
#970=B_SPLINE_CURVE_WITH_KNOTS('',3,(#39202,#39203,#39204,#39205),
 .UNSPECIFIED.,.F.,.F.,(4,4),(-1.14947842120138,-1.05363271233087),
 .UNSPECIFIED.);
#971=B_SPLINE_CURVE_WITH_KNOTS('',3,(#39207,#39208,#39209,#39210,#39211,
#39212,#39213,#39214,#39215,#39216,#39217,#39218,#39219,#39220,#39221,#39222,
#39223),.UNSPECIFIED.,.F.,.F.,(4,1,1,1,1,1,1,1,1,1,1,1,1,1,4),(0.,0.125,
0.1875,0.25,0.3125,0.375,0.5,0.625,0.6875,0.71875,0.75,0.78125,0.8125,0.875,
0.999999992783616),.UNSPECIFIED.);
#972=B_SPLINE_CURVE_WITH_KNOTS('',3,(#39225,#39226,#39227,#39228,#39229,
#39230,#39231,#39232,#39233,#39234,#39235,#39236,#39237,#39238,#39239,#39240,
#39241),.UNSPECIFIED.,.F.,.F.,(4,1,1,1,1,1,1,1,1,1,1,1,1,1,4),(4.61532930101729E-9,
0.125,0.1875,0.21875,0.25,0.28125,0.3125,0.375,0.5,0.625,0.6875,0.75,0.8125,
0.875,1.),.UNSPECIFIED.);
#973=B_SPLINE_CURVE_WITH_KNOTS('',3,(#39242,#39243,#39244,#39245),
 .UNSPECIFIED.,.F.,.F.,(4,4),(-1.1486920679677,-1.05773319824162),
 .UNSPECIFIED.);
#974=B_SPLINE_CURVE_WITH_KNOTS('',3,(#39249,#39250,#39251,#39252,#39253,
#39254,#39255,#39256,#39257,#39258,#39259,#39260,#39261,#39262,#39263,#39264,
#39265),.UNSPECIFIED.,.F.,.F.,(4,1,1,1,1,1,1,1,1,1,1,1,1,1,4),(0.,0.125,
0.1875,0.25,0.3125,0.375,0.5,0.625,0.6875,0.71875,0.75,0.78125,0.8125,0.875,
0.999999986938439),.UNSPECIFIED.);
#975=B_SPLINE_CURVE_WITH_KNOTS('',3,(#39267,#39268,#39269,#39270,#39271,
#39272,#39273,#39274,#39275,#39276,#39277,#39278,#39279,#39280,#39281,#39282,
#39283,#39284,#39285),.UNSPECIFIED.,.F.,.F.,(4,1,1,1,1,1,1,1,1,1,1,1,1,
1,1,1,4),(9.72661732996662E-8,0.125,0.1875,0.21875,0.25,0.28125,0.3125,
0.375,0.5,0.625,0.6875,0.71875,0.75,0.78125,0.8125,0.875,1.),
 .UNSPECIFIED.);
#976=B_SPLINE_CURVE_WITH_KNOTS('',3,(#39287,#39288,#39289,#39290),
 .UNSPECIFIED.,.F.,.F.,(4,4),(-1.13349992980958,-1.03925436083094),
 .UNSPECIFIED.);
#977=B_SPLINE_CURVE_WITH_KNOTS('',3,(#39292,#39293,#39294,#39295,#39296,
#39297,#39298,#39299,#39300,#39301,#39302,#39303,#39304,#39305,#39306,#39307,
#39308,#39309,#39310),.UNSPECIFIED.,.F.,.F.,(4,1,1,1,1,1,1,1,1,1,1,1,1,
1,1,1,4),(0.,0.125,0.1875,0.21875,0.25,0.28125,0.3125,0.375,0.5,0.625,0.6875,
0.71875,0.75,0.78125,0.8125,0.875,1.),.UNSPECIFIED.);
#978=B_SPLINE_CURVE_WITH_KNOTS('',3,(#39312,#39313,#39314,#39315,#39316,
#39317,#39318,#39319,#39320,#39321,#39322,#39323,#39324,#39325,#39326,#39327,
#39328),.UNSPECIFIED.,.F.,.F.,(4,1,1,1,1,1,1,1,1,1,1,1,1,1,4),(0.,0.125,
0.1875,0.21875,0.25,0.28125,0.3125,0.375,0.5,0.625,0.6875,0.75,0.8125,0.875,
1.),.UNSPECIFIED.);
#979=B_SPLINE_CURVE_WITH_KNOTS('',3,(#39329,#39330,#39331,#39332),
 .UNSPECIFIED.,.F.,.F.,(4,4),(-1.14030765698104,-1.04891270929124),
 .UNSPECIFIED.);
#980=B_SPLINE_CURVE_WITH_KNOTS('',3,(#39336,#39337,#39338,#39339,#39340,
#39341,#39342,#39343,#39344,#39345,#39346,#39347,#39348,#39349,#39350,#39351,
#39352,#39353,#39354,#39355,#39356,#39357,#39358,#39359,#39360,#39361,#39362,
#39363,#39364,#39365,#39366,#39367,#39368,#39369,#39370,#39371,#39372,#39373,
#39374,#39375,#39376,#39377,#39378,#39379,#39380,#39381,#39382,#39383,#39384),
 .UNSPECIFIED.,.F.,.F.,(4,3,3,3,3,3,3,3,3,3,3,3,3,3,3,3,4),(2.55001903434036E-14,
0.125,0.1875,0.21875,0.25,0.28125,0.3125,0.375,0.5,0.625,0.6875,0.71875,
0.75,0.78125,0.8125,0.875,0.999999987092966),.UNSPECIFIED.);
#981=B_SPLINE_CURVE_WITH_KNOTS('',3,(#39386,#39387,#39388,#39389,#39390,
#39391,#39392,#39393,#39394,#39395,#39396,#39397,#39398,#39399,#39400,#39401,
#39402,#39403,#39404),.UNSPECIFIED.,.F.,.F.,(4,1,1,1,1,1,1,1,1,1,1,1,1,
1,1,1,4),(1.12071241714957E-7,0.125,0.1875,0.21875,0.25,0.28125,0.3125,
0.375,0.5,0.625,0.6875,0.71875,0.75,0.78125,0.8125,0.875,1.),
 .UNSPECIFIED.);
#982=B_SPLINE_CURVE_WITH_KNOTS('',3,(#39406,#39407,#39408,#39409),
 .UNSPECIFIED.,.F.,.F.,(4,4),(-1.13407654678454,-1.03941382788935),
 .UNSPECIFIED.);
#983=B_SPLINE_CURVE_WITH_KNOTS('',3,(#39411,#39412,#39413,#39414,#39415,
#39416,#39417,#39418,#39419,#39420,#39421,#39422,#39423,#39424,#39425,#39426,
#39427,#39428,#39429,#39430,#39431,#39432,#39433,#39434,#39435,#39436,#39437,
#39438,#39439,#39440,#39441,#39442,#39443,#39444,#39445,#39446,#39447,#39448,
#39449,#39450,#39451,#39452,#39453,#39454,#39455,#39456,#39457,#39458,#39459),
 .UNSPECIFIED.,.F.,.F.,(4,3,3,3,3,3,3,3,3,3,3,3,3,3,3,3,4),(0.,0.125,0.1875,
0.21875,0.25,0.28125,0.3125,0.375,0.5,0.625,0.6875,0.71875,0.75,0.78125,
0.8125,0.875,1.),.UNSPECIFIED.);
#984=B_SPLINE_CURVE_WITH_KNOTS('',3,(#39461,#39462,#39463,#39464,#39465,
#39466,#39467,#39468,#39469,#39470,#39471,#39472,#39473,#39474,#39475,#39476,
#39477),.UNSPECIFIED.,.F.,.F.,(4,1,1,1,1,1,1,1,1,1,1,1,1,1,4),(0.,0.125,
0.1875,0.21875,0.25,0.28125,0.3125,0.375,0.5,0.625,0.6875,0.75,0.8125,0.875,
1.),.UNSPECIFIED.);
#985=B_SPLINE_CURVE_WITH_KNOTS('',3,(#39478,#39479,#39480,#39481),
 .UNSPECIFIED.,.F.,.F.,(4,4),(-1.13870206156022,-1.04613000297405),
 .UNSPECIFIED.);
#986=B_SPLINE_CURVE_WITH_KNOTS('',3,(#39485,#39486,#39487,#39488,#39489,
#39490,#39491,#39492,#39493,#39494,#39495,#39496,#39497,#39498,#39499,#39500,
#39501,#39502,#39503,#39504,#39505,#39506,#39507,#39508,#39509,#39510,#39511,
#39512,#39513,#39514,#39515,#39516,#39517,#39518,#39519,#39520,#39521,#39522,
#39523,#39524,#39525,#39526,#39527,#39528,#39529,#39530,#39531,#39532,#39533),
 .UNSPECIFIED.,.F.,.F.,(4,3,3,3,3,3,3,3,3,3,3,3,3,3,3,3,4),(5.88455490193989E-15,
0.125,0.1875,0.21875,0.25,0.28125,0.3125,0.375,0.5,0.625,0.6875,0.71875,
0.75,0.78125,0.8125,0.875,0.99999998726157),.UNSPECIFIED.);
#987=B_SPLINE_CURVE_WITH_KNOTS('',3,(#39535,#39536,#39537,#39538,#39539,
#39540,#39541,#39542,#39543,#39544,#39545,#39546,#39547,#39548,#39549,#39550,
#39551,#39552,#39553),.UNSPECIFIED.,.F.,.F.,(4,1,1,1,1,1,1,1,1,1,1,1,1,
1,1,1,4),(1.40925419990928E-7,0.125,0.1875,0.21875,0.25,0.28125,0.3125,
0.375,0.5,0.625,0.6875,0.71875,0.75,0.78125,0.8125,0.875,1.),
 .UNSPECIFIED.);
#988=B_SPLINE_CURVE_WITH_KNOTS('',3,(#39555,#39556,#39557,#39558),
 .UNSPECIFIED.,.F.,.F.,(4,4),(-1.13230492679919,-1.03947426144326),
 .UNSPECIFIED.);
#989=B_SPLINE_CURVE_WITH_KNOTS('',3,(#39560,#39561,#39562,#39563,#39564,
#39565,#39566,#39567,#39568,#39569,#39570,#39571,#39572,#39573,#39574,#39575,
#39576,#39577,#39578,#39579,#39580,#39581,#39582,#39583,#39584,#39585,#39586,
#39587,#39588,#39589,#39590,#39591,#39592,#39593,#39594,#39595,#39596,#39597,
#39598,#39599,#39600,#39601,#39602,#39603,#39604,#39605,#39606,#39607,#39608),
 .UNSPECIFIED.,.F.,.F.,(4,3,3,3,3,3,3,3,3,3,3,3,3,3,3,3,4),(0.,0.125,0.1875,
0.21875,0.25,0.28125,0.3125,0.375,0.5,0.625,0.6875,0.71875,0.75,0.78125,
0.8125,0.875,1.),.UNSPECIFIED.);
#990=B_SPLINE_CURVE_WITH_KNOTS('',3,(#39610,#39611,#39612,#39613,#39614,
#39615,#39616,#39617,#39618,#39619,#39620,#39621,#39622,#39623,#39624,#39625,
#39626,#39627,#39628,#39629,#39630,#39631,#39632,#39633,#39634,#39635,#39636,
#39637,#39638,#39639,#39640,#39641,#39642,#39643,#39644,#39645,#39646,#39647,
#39648,#39649,#39650,#39651,#39652,#39653,#39654,#39655,#39656,#39657,#39658),
 .UNSPECIFIED.,.F.,.F.,(4,3,3,3,3,3,3,3,3,3,3,3,3,3,3,3,4),(0.,0.125,0.1875,
0.21875,0.25,0.28125,0.3125,0.375,0.5,0.625,0.6875,0.71875,0.75,0.78125,
0.8125,0.875,1.),.UNSPECIFIED.);
#991=B_SPLINE_CURVE_WITH_KNOTS('',3,(#39659,#39660,#39661,#39662),
 .UNSPECIFIED.,.F.,.F.,(4,4),(-1.14623578895171,-1.0552604634692),
 .UNSPECIFIED.);
#992=B_SPLINE_CURVE_WITH_KNOTS('',3,(#39666,#39667,#39668,#39669,#39670,
#39671,#39672,#39673,#39674,#39675,#39676,#39677,#39678,#39679,#39680,#39681,
#39682),.UNSPECIFIED.,.F.,.F.,(4,1,1,1,1,1,1,1,1,1,1,1,1,1,4),(0.,0.125,
0.1875,0.25,0.3125,0.375,0.5,0.625,0.6875,0.71875,0.75,0.78125,0.8125,0.875,
1.),.UNSPECIFIED.);
#993=B_SPLINE_CURVE_WITH_KNOTS('',3,(#39684,#39685,#39686,#39687,#39688,
#39689,#39690,#39691,#39692,#39693,#39694,#39695,#39696,#39697,#39698,#39699,
#39700),.UNSPECIFIED.,.F.,.F.,(4,1,1,1,1,1,1,1,1,1,1,1,1,1,4),(8.0555447065195E-8,
0.125,0.1875,0.21875,0.25,0.28125,0.3125,0.375,0.5,0.625,0.6875,0.75,0.8125,
0.875,1.),.UNSPECIFIED.);
#994=B_SPLINE_CURVE_WITH_KNOTS('',3,(#39702,#39703,#39704,#39705,#39706,
#39707),.UNSPECIFIED.,.F.,.F.,(4,2,4),(-1.14515135463117,-1.06190814579394,
-1.04640883228602),.UNSPECIFIED.);
#995=B_SPLINE_CURVE_WITH_KNOTS('',3,(#39709,#39710,#39711,#39712,#39713,
#39714,#39715,#39716,#39717,#39718,#39719,#39720,#39721,#39722,#39723,#39724,
#39725),.UNSPECIFIED.,.F.,.F.,(4,1,1,1,1,1,1,1,1,1,1,1,1,1,4),(0.,0.125,
0.1875,0.25,0.3125,0.375,0.5,0.625,0.6875,0.71875,0.75,0.78125,0.8125,0.875,
0.999999978936368),.UNSPECIFIED.);
#996=B_SPLINE_CURVE_WITH_KNOTS('',3,(#39727,#39728,#39729,#39730,#39731,
#39732,#39733,#39734,#39735,#39736,#39737,#39738,#39739,#39740,#39741,#39742,
#39743),.UNSPECIFIED.,.F.,.F.,(4,1,1,1,1,1,1,1,1,1,1,1,1,1,4),(2.28361295605953E-8,
0.125,0.1875,0.21875,0.25,0.28125,0.3125,0.375,0.5,0.625,0.6875,0.75,0.8125,
0.875,1.),.UNSPECIFIED.);
#997=B_SPLINE_CURVE_WITH_KNOTS('',3,(#39744,#39745,#39746,#39747),
 .UNSPECIFIED.,.F.,.F.,(4,4),(-1.13911633111086,-1.04475206254057),
 .UNSPECIFIED.);
#998=B_SPLINE_CURVE_WITH_KNOTS('',3,(#39751,#39752,#39753,#39754,#39755,
#39756,#39757,#39758,#39759,#39760,#39761,#39762,#39763,#39764,#39765,#39766,
#39767,#39768,#39769),.UNSPECIFIED.,.F.,.F.,(4,1,1,1,1,1,1,1,1,1,1,1,1,
1,1,1,4),(0.,0.125,0.1875,0.21875,0.25,0.28125,0.3125,0.375,0.5,0.625,0.6875,
0.71875,0.75,0.78125,0.8125,0.875,0.999999987528574),.UNSPECIFIED.);
#999=B_SPLINE_CURVE_WITH_KNOTS('',3,(#39771,#39772,#39773,#39774,#39775,
#39776,#39777,#39778,#39779,#39780,#39781,#39782,#39783,#39784,#39785,#39786,
#39787,#39788,#39789),.UNSPECIFIED.,.F.,.F.,(4,1,1,1,1,1,1,1,1,1,1,1,1,
1,1,1,4),(1.7743161549064E-7,0.125,0.1875,0.21875,0.25,0.28125,0.3125,0.375,
0.5,0.625,0.6875,0.71875,0.75,0.78125,0.8125,0.875,1.),.UNSPECIFIED.);
#1000=B_SPLINE_CURVE_WITH_KNOTS('',3,(#39791,#39792,#39793,#39794),
 .UNSPECIFIED.,.F.,.F.,(4,4),(-1.13925469784202,-1.04825641978528),
 .UNSPECIFIED.);
#1001=B_SPLINE_CURVE_WITH_KNOTS('',3,(#39796,#39797,#39798,#39799,#39800,
#39801,#39802,#39803,#39804,#39805,#39806,#39807,#39808,#39809,#39810,#39811,
#39812,#39813,#39814,#39815,#39816,#39817,#39818,#39819,#39820,#39821,#39822,
#39823,#39824,#39825,#39826,#39827,#39828,#39829,#39830,#39831,#39832,#39833,
#39834,#39835,#39836,#39837,#39838,#39839,#39840,#39841,#39842,#39843,#39844),
 .UNSPECIFIED.,.F.,.F.,(4,3,3,3,3,3,3,3,3,3,3,3,3,3,3,3,4),(0.,0.125,0.1875,
0.21875,0.25,0.28125,0.3125,0.375,0.5,0.625,0.6875,0.71875,0.75,0.78125,
0.8125,0.875,1.),.UNSPECIFIED.);
#1002=B_SPLINE_CURVE_WITH_KNOTS('',3,(#39846,#39847,#39848,#39849,#39850,
#39851,#39852,#39853,#39854,#39855,#39856,#39857,#39858,#39859,#39860,#39861,
#39862,#39863,#39864,#39865,#39866,#39867,#39868,#39869,#39870,#39871,#39872,
#39873,#39874,#39875,#39876,#39877,#39878,#39879,#39880,#39881,#39882,#39883,
#39884,#39885,#39886,#39887,#39888,#39889,#39890,#39891,#39892,#39893,#39894),
 .UNSPECIFIED.,.F.,.F.,(4,3,3,3,3,3,3,3,3,3,3,3,3,3,3,3,4),(0.,0.125,0.1875,
0.21875,0.25,0.28125,0.3125,0.375,0.5,0.625,0.6875,0.71875,0.75,0.78125,
0.8125,0.875,1.),.UNSPECIFIED.);
#1003=B_SPLINE_CURVE_WITH_KNOTS('',3,(#39895,#39896,#39897,#39898),
 .UNSPECIFIED.,.F.,.F.,(4,4),(-1.15381330807476,-1.06213654023606),
 .UNSPECIFIED.);
#1004=B_SPLINE_CURVE_WITH_KNOTS('',3,(#39902,#39903,#39904,#39905,#39906,
#39907,#39908,#39909,#39910,#39911,#39912,#39913,#39914,#39915,#39916,#39917,
#39918,#39919),.UNSPECIFIED.,.F.,.F.,(4,1,1,1,1,1,1,1,1,1,1,1,1,1,1,4),
(0.,0.125,0.1875,0.25,0.3125,0.375,0.4375,0.5,0.625,0.6875,0.71875,0.75,
0.78125,0.8125,0.875,1.),.UNSPECIFIED.);
#1005=B_SPLINE_CURVE_WITH_KNOTS('',3,(#39921,#39922,#39923,#39924,#39925,
#39926,#39927,#39928,#39929,#39930,#39931,#39932,#39933,#39934,#39935,#39936,
#39937,#39938),.UNSPECIFIED.,.F.,.F.,(4,1,1,1,1,1,1,1,1,1,1,1,1,1,1,4),
(1.64962983094098E-7,0.125,0.1875,0.21875,0.25,0.28125,0.3125,0.375,0.5,
0.5625,0.625,0.6875,0.75,0.8125,0.875,0.999999279741807),.UNSPECIFIED.);
#1006=B_SPLINE_CURVE_WITH_KNOTS('',3,(#39940,#39941,#39942,#39943),
 .UNSPECIFIED.,.F.,.F.,(4,4),(-1.14333787758334,-1.05241548175551),
 .UNSPECIFIED.);
#1007=B_SPLINE_CURVE_WITH_KNOTS('',3,(#39945,#39946,#39947,#39948,#39949,
#39950,#39951,#39952,#39953,#39954,#39955,#39956,#39957,#39958,#39959,#39960,
#39961,#39962),.UNSPECIFIED.,.F.,.F.,(4,1,1,1,1,1,1,1,1,1,1,1,1,1,1,4),
(0.,0.125,0.1875,0.25,0.3125,0.375,0.4375,0.5,0.625,0.6875,0.71875,0.75,
0.78125,0.8125,0.875,0.999999803503463),.UNSPECIFIED.);
#1008=B_SPLINE_CURVE_WITH_KNOTS('',3,(#39964,#39965,#39966,#39967,#39968,
#39969,#39970,#39971,#39972,#39973,#39974,#39975,#39976,#39977,#39978,#39979,
#39980,#39981),.UNSPECIFIED.,.F.,.F.,(4,1,1,1,1,1,1,1,1,1,1,1,1,1,1,4),
(0.,0.125,0.1875,0.21875,0.25,0.28125,0.3125,0.375,0.5,0.5625,0.625,0.6875,
0.75,0.8125,0.875,1.),.UNSPECIFIED.);
#1009=B_SPLINE_CURVE_WITH_KNOTS('',3,(#39982,#39983,#39984,#39985),
 .UNSPECIFIED.,.F.,.F.,(4,4),(-1.16836067888312,-1.07743287791435),
 .UNSPECIFIED.);
#1010=B_SPLINE_CURVE_WITH_KNOTS('',3,(#39989,#39990,#39991,#39992,#39993,
#39994,#39995,#39996,#39997,#39998,#39999,#40000,#40001,#40002,#40003,#40004,
#40005,#40006,#40007),.UNSPECIFIED.,.F.,.F.,(4,1,1,1,1,1,1,1,1,1,1,1,1,
1,1,1,4),(0.,0.125,0.1875,0.21875,0.25,0.28125,0.3125,0.375,0.5,0.625,0.6875,
0.71875,0.75,0.78125,0.8125,0.875,1.),.UNSPECIFIED.);
#1011=B_SPLINE_CURVE_WITH_KNOTS('',3,(#40009,#40010,#40011,#40012,#40013,
#40014,#40015,#40016,#40017,#40018,#40019,#40020,#40021,#40022,#40023,#40024,
#40025,#40026,#40027),.UNSPECIFIED.,.F.,.F.,(4,1,1,1,1,1,1,1,1,1,1,1,1,
1,1,1,4),(1.71448431414438E-7,0.125,0.1875,0.21875,0.25,0.28125,0.3125,
0.375,0.5,0.625,0.6875,0.71875,0.75,0.78125,0.8125,0.875,1.),
 .UNSPECIFIED.);
#1012=B_SPLINE_CURVE_WITH_KNOTS('',3,(#40029,#40030,#40031,#40032),
 .UNSPECIFIED.,.F.,.F.,(4,4),(-1.13680001467877,-1.04572530935217),
 .UNSPECIFIED.);
#1013=B_SPLINE_CURVE_WITH_KNOTS('',3,(#40034,#40035,#40036,#40037,#40038,
#40039,#40040,#40041,#40042,#40043,#40044,#40045,#40046,#40047,#40048,#40049,
#40050,#40051,#40052,#40053,#40054,#40055,#40056,#40057,#40058,#40059,#40060,
#40061,#40062,#40063,#40064,#40065,#40066,#40067,#40068,#40069,#40070,#40071,
#40072,#40073,#40074,#40075,#40076,#40077,#40078,#40079,#40080,#40081,#40082),
 .UNSPECIFIED.,.F.,.F.,(4,3,3,3,3,3,3,3,3,3,3,3,3,3,3,3,4),(0.,0.125,0.1875,
0.21875,0.25,0.28125,0.3125,0.375,0.5,0.625,0.6875,0.71875,0.75,0.78125,
0.8125,0.875,1.),.UNSPECIFIED.);
#1014=B_SPLINE_CURVE_WITH_KNOTS('',3,(#40084,#40085,#40086,#40087,#40088,
#40089,#40090,#40091,#40092,#40093,#40094,#40095,#40096,#40097,#40098,#40099,
#40100,#40101,#40102,#40103,#40104,#40105,#40106,#40107,#40108,#40109,#40110,
#40111,#40112,#40113,#40114,#40115,#40116,#40117,#40118,#40119,#40120,#40121,
#40122,#40123,#40124,#40125,#40126,#40127,#40128,#40129,#40130,#40131,#40132),
 .UNSPECIFIED.,.F.,.F.,(4,3,3,3,3,3,3,3,3,3,3,3,3,3,3,3,4),(0.,0.125,0.1875,
0.21875,0.25,0.28125,0.3125,0.375,0.5,0.625,0.6875,0.71875,0.75,0.78125,
0.8125,0.875,1.),.UNSPECIFIED.);
#1015=B_SPLINE_CURVE_WITH_KNOTS('',3,(#40133,#40134,#40135,#40136),
 .UNSPECIFIED.,.F.,.F.,(4,4),(-1.14643591429736,-1.05546845872828),
 .UNSPECIFIED.);
#1016=B_SPLINE_CURVE_WITH_KNOTS('',3,(#40140,#40141,#40142,#40143,#40144,
#40145,#40146,#40147,#40148,#40149,#40150,#40151,#40152,#40153,#40154,#40155,
#40156),.UNSPECIFIED.,.F.,.F.,(4,1,1,1,1,1,1,1,1,1,1,1,1,1,4),(0.,0.125,
0.1875,0.25,0.3125,0.375,0.5,0.625,0.6875,0.71875,0.75,0.78125,0.8125,0.875,
0.999974157502117),.UNSPECIFIED.);
#1017=B_SPLINE_CURVE_WITH_KNOTS('',3,(#40158,#40159,#40160,#40161,#40162,
#40163,#40164,#40165,#40166,#40167,#40168,#40169,#40170,#40171,#40172,#40173,
#40174,#40175,#40176,#40177,#40178,#40179,#40180,#40181,#40182,#40183,#40184,
#40185,#40186,#40187,#40188,#40189,#40190,#40191,#40192,#40193,#40194,#40195,
#40196,#40197,#40198,#40199,#40200,#40201,#40202,#40203,#40204,#40205,#40206,
#40207),.UNSPECIFIED.,.F.,.F.,(4,2,2,2,2,2,2,2,2,2,2,2,2,2,2,2,2,2,2,2,
2,2,2,2,4),(2.4036706065768E-5,0.00977418865733799,0.0213000820686129,0.0228713448821847,
0.0245760487443449,0.028666855265285,0.0419488423804167,0.0819470875054392,
0.0874089326177544,0.116494431563777,0.155248703049381,0.176699028655761,
0.20033104560553,0.250819278402669,0.282215606032038,0.337127383171215,
0.420231565913135,0.422824375704096,0.427853052523601,0.465166977215536,
0.477606564650635,0.485039244387621,0.489575937579279,0.490429017673501,
0.503063262505017),.UNSPECIFIED.);
#1018=B_SPLINE_CURVE_WITH_KNOTS('',3,(#40209,#40210,#40211,#40212),
 .UNSPECIFIED.,.F.,.F.,(4,4),(-1.14946321606806,-1.05524237219014),
 .UNSPECIFIED.);
#1019=B_SPLINE_CURVE_WITH_KNOTS('',3,(#40214,#40215,#40216,#40217,#40218,
#40219,#40220,#40221,#40222,#40223,#40224,#40225,#40226,#40227,#40228,#40229,
#40230),.UNSPECIFIED.,.F.,.F.,(4,1,1,1,1,1,1,1,1,1,1,1,1,1,4),(0.,0.125,
0.1875,0.25,0.3125,0.375,0.5,0.625,0.6875,0.71875,0.75,0.78125,0.8125,0.875,
0.999999978619674),.UNSPECIFIED.);
#1020=B_SPLINE_CURVE_WITH_KNOTS('',3,(#40232,#40233,#40234,#40235,#40236,
#40237,#40238,#40239,#40240,#40241,#40242,#40243,#40244,#40245,#40246,#40247,
#40248),.UNSPECIFIED.,.F.,.F.,(4,1,1,1,1,1,1,1,1,1,1,1,1,1,4),(1.83706666942875E-8,
0.125,0.1875,0.21875,0.25,0.28125,0.3125,0.375,0.5,0.625,0.6875,0.75,0.8125,
0.875,1.),.UNSPECIFIED.);
#1021=B_SPLINE_CURVE_WITH_KNOTS('',3,(#40249,#40250,#40251,#40252),
 .UNSPECIFIED.,.F.,.F.,(4,4),(-1.14299247720633,-1.0519693017081),
 .UNSPECIFIED.);
#1022=B_SPLINE_CURVE_WITH_KNOTS('',3,(#40256,#40257,#40258,#40259,#40260,
#40261,#40262,#40263,#40264,#40265,#40266,#40267,#40268,#40269,#40270,#40271,
#40272),.UNSPECIFIED.,.F.,.F.,(4,1,1,1,1,1,1,1,1,1,1,1,1,1,4),(0.,0.125,
0.1875,0.25,0.3125,0.375,0.5,0.625,0.6875,0.71875,0.75,0.78125,0.8125,0.875,
0.999973904155701),.UNSPECIFIED.);
#1023=B_SPLINE_CURVE_WITH_KNOTS('',3,(#40274,#40275,#40276,#40277,#40278,
#40279,#40280,#40281,#40282,#40283,#40284,#40285,#40286,#40287,#40288,#40289,
#40290,#40291,#40292,#40293,#40294,#40295,#40296,#40297,#40298,#40299,#40300,
#40301,#40302,#40303,#40304,#40305,#40306,#40307,#40308,#40309,#40310,#40311,
#40312,#40313,#40314,#40315,#40316,#40317,#40318,#40319),.UNSPECIFIED.,
 .F.,.F.,(4,2,2,2,2,2,2,2,2,2,2,2,2,2,2,2,2,2,2,2,2,2,4),(2.47988659577903E-5,
0.00978202028211238,0.0213215802168401,0.0228946245359042,0.0246012949911653,
0.0286969595382463,0.0419977049211027,0.0820560797602515,0.0875251626699372,
0.116649382017729,0.155456996931585,0.17693206420461,0.200598959304169,
0.250883813270901,0.282287570163106,0.337211637910956,0.420331994699351,
0.430730860332875,0.466657227821203,0.47845661856984,0.485622048026449,
0.49444503678418,0.503140993568406),.UNSPECIFIED.);
#1024=B_SPLINE_CURVE_WITH_KNOTS('',3,(#40321,#40322,#40323,#40324),
 .UNSPECIFIED.,.F.,.F.,(4,4),(-1.14031632988646,-1.04922087046088),
 .UNSPECIFIED.);
#1025=B_SPLINE_CURVE_WITH_KNOTS('',3,(#40326,#40327,#40328,#40329,#40330,
#40331,#40332,#40333,#40334,#40335,#40336,#40337,#40338,#40339,#40340,#40341,
#40342),.UNSPECIFIED.,.F.,.F.,(4,1,1,1,1,1,1,1,1,1,1,1,1,1,4),(0.,0.125,
0.1875,0.25,0.3125,0.375,0.5,0.625,0.6875,0.71875,0.75,0.78125,0.8125,0.875,
0.999999976967435),.UNSPECIFIED.);
#1026=B_SPLINE_CURVE_WITH_KNOTS('',3,(#40344,#40345,#40346,#40347,#40348,
#40349,#40350,#40351,#40352,#40353,#40354,#40355,#40356,#40357,#40358,#40359,
#40360),.UNSPECIFIED.,.F.,.F.,(4,1,1,1,1,1,1,1,1,1,1,1,1,1,4),(1.69410983812543E-8,
0.125,0.1875,0.21875,0.25,0.28125,0.3125,0.375,0.5,0.625,0.6875,0.75,0.8125,
0.875,1.),.UNSPECIFIED.);
#1027=B_SPLINE_CURVE_WITH_KNOTS('',3,(#40361,#40362,#40363,#40364),
 .UNSPECIFIED.,.F.,.F.,(4,4),(-1.14138748856057,-1.05023984115422),
 .UNSPECIFIED.);
#1028=B_SPLINE_CURVE_WITH_KNOTS('',3,(#40368,#40369,#40370,#40371,#40372,
#40373,#40374,#40375,#40376,#40377,#40378,#40379,#40380,#40381,#40382,#40383,
#40384),.UNSPECIFIED.,.F.,.F.,(4,1,1,1,1,1,1,1,1,1,1,1,1,1,4),(0.,0.125,
0.1875,0.25,0.3125,0.375,0.5,0.625,0.6875,0.71875,0.75,0.78125,0.8125,0.875,
0.999999958992443),.UNSPECIFIED.);
#1029=B_SPLINE_CURVE_WITH_KNOTS('',3,(#40386,#40387,#40388,#40389,#40390,
#40391,#40392,#40393,#40394,#40395,#40396,#40397,#40398,#40399,#40400,#40401,
#40402),.UNSPECIFIED.,.F.,.F.,(4,1,1,1,1,1,1,1,1,1,1,1,1,1,4),(0.,0.125,
0.1875,0.21875,0.25,0.28125,0.3125,0.375,0.5,0.625,0.6875,0.75,0.8125,0.875,
1.),.UNSPECIFIED.);
#1030=B_SPLINE_CURVE_WITH_KNOTS('',3,(#40404,#40405,#40406,#40407),
 .UNSPECIFIED.,.F.,.F.,(4,4),(-1.14907451824135,-1.05612055222212),
 .UNSPECIFIED.);
#1031=B_SPLINE_CURVE_WITH_KNOTS('',3,(#40409,#40410,#40411,#40412,#40413,
#40414,#40415,#40416,#40417,#40418,#40419,#40420,#40421,#40422,#40423,#40424,
#40425),.UNSPECIFIED.,.F.,.F.,(4,1,1,1,1,1,1,1,1,1,1,1,1,1,4),(0.,0.125,
0.1875,0.25,0.3125,0.375,0.5,0.625,0.6875,0.71875,0.75,0.78125,0.8125,0.875,
0.999999976401986),.UNSPECIFIED.);
#1032=B_SPLINE_CURVE_WITH_KNOTS('',3,(#40427,#40428,#40429,#40430,#40431,
#40432,#40433,#40434,#40435,#40436,#40437,#40438,#40439,#40440,#40441,#40442,
#40443),.UNSPECIFIED.,.F.,.F.,(4,1,1,1,1,1,1,1,1,1,1,1,1,1,4),(1.69808900141672E-8,
0.125,0.1875,0.21875,0.25,0.28125,0.3125,0.375,0.5,0.625,0.6875,0.75,0.8125,
0.875,1.),.UNSPECIFIED.);
#1033=B_SPLINE_CURVE_WITH_KNOTS('',3,(#40444,#40445,#40446,#40447),
 .UNSPECIFIED.,.F.,.F.,(4,4),(-1.14206554603712,-1.05097269226909),
 .UNSPECIFIED.);
#1034=B_SPLINE_CURVE_WITH_KNOTS('',3,(#40451,#40452,#40453,#40454,#40455,
#40456,#40457,#40458,#40459,#40460,#40461,#40462,#40463,#40464,#40465,#40466,
#40467),.UNSPECIFIED.,.F.,.F.,(4,1,1,1,1,1,1,1,1,1,1,1,1,1,4),(0.,0.125,
0.1875,0.25,0.3125,0.375,0.5,0.625,0.6875,0.71875,0.75,0.78125,0.8125,0.875,
0.999999966016196),.UNSPECIFIED.);
#1035=B_SPLINE_CURVE_WITH_KNOTS('',3,(#40469,#40470,#40471,#40472,#40473,
#40474,#40475,#40476,#40477,#40478,#40479,#40480,#40481,#40482,#40483,#40484,
#40485),.UNSPECIFIED.,.F.,.F.,(4,1,1,1,1,1,1,1,1,1,1,1,1,1,4),(0.,0.125,
0.1875,0.21875,0.25,0.28125,0.3125,0.375,0.5,0.625,0.6875,0.75,0.8125,0.875,
1.),.UNSPECIFIED.);
#1036=B_SPLINE_CURVE_WITH_KNOTS('',3,(#40487,#40488,#40489,#40490),
 .UNSPECIFIED.,.F.,.F.,(4,4),(-1.14014949111156,-1.04925591765877),
 .UNSPECIFIED.);
#1037=B_SPLINE_CURVE_WITH_KNOTS('',3,(#40492,#40493,#40494,#40495,#40496,
#40497,#40498,#40499,#40500,#40501,#40502,#40503,#40504,#40505,#40506,#40507,
#40508),.UNSPECIFIED.,.F.,.F.,(4,1,1,1,1,1,1,1,1,1,1,1,1,1,4),(0.,0.125,
0.1875,0.25,0.3125,0.375,0.5,0.625,0.6875,0.71875,0.75,0.78125,0.8125,0.875,
0.999999978755288),.UNSPECIFIED.);
#1038=B_SPLINE_CURVE_WITH_KNOTS('',3,(#40510,#40511,#40512,#40513,#40514,
#40515,#40516,#40517,#40518,#40519,#40520,#40521,#40522,#40523,#40524,#40525,
#40526),.UNSPECIFIED.,.F.,.F.,(4,1,1,1,1,1,1,1,1,1,1,1,1,1,4),(2.33180965054172E-8,
0.125,0.1875,0.21875,0.25,0.28125,0.3125,0.375,0.5,0.625,0.6875,0.75,0.8125,
0.875,1.),.UNSPECIFIED.);
#1039=B_SPLINE_CURVE_WITH_KNOTS('',3,(#40527,#40528,#40529,#40530),
 .UNSPECIFIED.,.F.,.F.,(4,4),(-1.14020705449601,-1.04518868540341),
 .UNSPECIFIED.);
#1040=B_SPLINE_CURVE_WITH_KNOTS('',3,(#40534,#40535,#40536,#40537,#40538,
#40539,#40540,#40541,#40542,#40543,#40544,#40545,#40546,#40547,#40548,#40549,
#40550,#40551),.UNSPECIFIED.,.F.,.F.,(4,1,1,1,1,1,1,1,1,1,1,1,1,1,1,4),
(0.,0.125,0.1875,0.25,0.3125,0.375,0.4375,0.5,0.625,0.6875,0.71875,0.75,
0.78125,0.8125,0.875,1.),.UNSPECIFIED.);
#1041=B_SPLINE_CURVE_WITH_KNOTS('',3,(#40553,#40554,#40555,#40556,#40557,
#40558,#40559,#40560,#40561,#40562,#40563,#40564,#40565,#40566,#40567,#40568,
#40569,#40570),.UNSPECIFIED.,.F.,.F.,(4,1,1,1,1,1,1,1,1,1,1,1,1,1,1,4),
(9.65284522368403E-8,0.125,0.1875,0.21875,0.25,0.28125,0.3125,0.375,0.5,
0.5625,0.625,0.6875,0.75,0.8125,0.875,0.999999352149596),.UNSPECIFIED.);
#1042=B_SPLINE_CURVE_WITH_KNOTS('',3,(#40572,#40573,#40574,#40575),
 .UNSPECIFIED.,.F.,.F.,(4,4),(-1.14221789136096,-1.0513242695399),
 .UNSPECIFIED.);
#1043=B_SPLINE_CURVE_WITH_KNOTS('',3,(#40577,#40578,#40579,#40580,#40581,
#40582,#40583,#40584,#40585,#40586,#40587,#40588,#40589,#40590,#40591,#40592,
#40593,#40594),.UNSPECIFIED.,.F.,.F.,(4,1,1,1,1,1,1,1,1,1,1,1,1,1,1,4),
(0.,0.125,0.1875,0.25,0.3125,0.375,0.4375,0.5,0.625,0.6875,0.71875,0.75,
0.78125,0.8125,0.875,0.999999772281826),.UNSPECIFIED.);
#1044=B_SPLINE_CURVE_WITH_KNOTS('',3,(#40596,#40597,#40598,#40599,#40600,
#40601,#40602,#40603,#40604,#40605,#40606,#40607,#40608,#40609,#40610,#40611,
#40612,#40613),.UNSPECIFIED.,.F.,.F.,(4,1,1,1,1,1,1,1,1,1,1,1,1,1,1,4),
(0.,0.125,0.1875,0.21875,0.25,0.28125,0.3125,0.375,0.5,0.5625,0.625,0.6875,
0.75,0.8125,0.875,1.),.UNSPECIFIED.);
#1045=B_SPLINE_CURVE_WITH_KNOTS('',3,(#40614,#40615,#40616,#40617),
 .UNSPECIFIED.,.F.,.F.,(4,4),(-1.16809592630694,-1.07716888491671),
 .UNSPECIFIED.);
#1046=B_SPLINE_CURVE_WITH_KNOTS('',3,(#40621,#40622,#40623,#40624,#40625,
#40626,#40627,#40628,#40629,#40630,#40631,#40632,#40633,#40634,#40635,#40636,
#40637),.UNSPECIFIED.,.F.,.F.,(4,1,1,1,1,1,1,1,1,1,1,1,1,1,4),(1.05070398993036E-5,
0.125,0.1875,0.25,0.3125,0.375,0.5,0.625,0.6875,0.71875,0.75,0.78125,0.8125,
0.875,1.),.UNSPECIFIED.);
#1047=B_SPLINE_CURVE_WITH_KNOTS('',3,(#40639,#40640,#40641,#40642,#40643,
#40644,#40645,#40646,#40647,#40648,#40649,#40650,#40651,#40652,#40653,#40654,
#40655),.UNSPECIFIED.,.F.,.F.,(4,1,1,1,1,1,1,1,1,1,1,1,1,1,4),(1.68482309315291E-7,
0.125,0.1875,0.21875,0.25,0.28125,0.3125,0.375,0.5,0.625,0.6875,0.75,0.8125,
0.875,1.),.UNSPECIFIED.);
#1048=B_SPLINE_CURVE_WITH_KNOTS('',3,(#40657,#40658,#40659,#40660,#40661,
#40662,#40663,#40664,#40665,#40666,#40667,#40668,#40669,#40670,#40671,#40672,
#40673,#40674,#40675,#40676,#40677,#40678,#40679,#40680,#40681),
 .UNSPECIFIED.,.F.,.F.,(4,3,3,3,3,3,3,3,4),(9.0152389462332E-6,0.250000179528252,
0.375000149606877,0.500000119685501,0.539828000683998,0.625000089764126,
0.750000059842751,0.81706191736929,0.999996337578903),.UNSPECIFIED.);
#1049=B_SPLINE_CURVE_WITH_KNOTS('',3,(#40683,#40684,#40685,#40686,#40687,
#40688,#40689,#40690,#40691,#40692,#40693,#40694,#40695,#40696,#40697,#40698,
#40699,#40700),.UNSPECIFIED.,.F.,.F.,(4,1,1,1,1,1,1,1,1,1,1,1,1,1,1,4),
(0.,0.125,0.1875,0.25,0.3125,0.375,0.4375,0.5,0.625,0.6875,0.71875,0.75,
0.78125,0.8125,0.875,0.999999833967708),.UNSPECIFIED.);
#1050=B_SPLINE_CURVE_WITH_KNOTS('',3,(#40702,#40703,#40704,#40705,#40706,
#40707,#40708,#40709,#40710,#40711,#40712,#40713,#40714,#40715,#40716,#40717,
#40718),.UNSPECIFIED.,.F.,.F.,(4,1,1,1,1,1,1,1,1,1,1,1,1,1,4),(0.,0.125,
0.1875,0.21875,0.25,0.28125,0.3125,0.375,0.5,0.625,0.6875,0.75,0.8125,0.875,
1.),.UNSPECIFIED.);
#1051=B_SPLINE_CURVE_WITH_KNOTS('',3,(#40719,#40720,#40721,#40722,#40723,
#40724,#40725,#40726,#40727),.UNSPECIFIED.,.F.,.F.,(4,1,1,1,1,1,4),(5.75355075983042E-8,
0.249999939248312,0.374999908872468,0.499999878496624,0.62499984812078,
0.749999817744936,0.999999756993248),.UNSPECIFIED.);
#1052=B_SPLINE_CURVE_WITH_KNOTS('',3,(#40731,#40732,#40733,#40734,#40735,
#40736,#40737,#40738,#40739,#40740,#40741,#40742,#40743,#40744,#40745,#40746,
#40747),.UNSPECIFIED.,.F.,.F.,(4,1,1,1,1,1,1,1,1,1,1,1,1,1,4),(0.000130637014181663,
0.125,0.1875,0.25,0.3125,0.375,0.5,0.625,0.6875,0.71875,0.75,0.78125,0.8125,
0.875,0.999999986791086),.UNSPECIFIED.);
#1053=B_SPLINE_CURVE_WITH_KNOTS('',3,(#40749,#40750,#40751,#40752,#40753,
#40754,#40755,#40756,#40757,#40758,#40759,#40760,#40761,#40762,#40763,#40764,
#40765,#40766,#40767),.UNSPECIFIED.,.F.,.F.,(4,1,1,1,1,1,1,1,1,1,1,1,1,
1,1,1,4),(7.60606706307879E-8,0.125,0.1875,0.21875,0.25,0.28125,0.3125,
0.375,0.5,0.625,0.6875,0.71875,0.75,0.78125,0.8125,0.875,1.),
 .UNSPECIFIED.);
#1054=B_SPLINE_CURVE_WITH_KNOTS('',3,(#40769,#40770,#40771,#40772,#40773,
#40774),.UNSPECIFIED.,.F.,.F.,(4,2,4),(4.75084510343136E-5,0.0562772365901649,
0.106122687546361),.UNSPECIFIED.);
#1055=B_SPLINE_CURVE_WITH_KNOTS('',3,(#40776,#40777,#40778,#40779,#40780,
#40781,#40782,#40783),.UNSPECIFIED.,.F.,.F.,(4,2,2,4),(0.163849162898279,
0.18750836405779,0.272594094712416,0.355211229604226),.UNSPECIFIED.);
#1056=B_SPLINE_CURVE_WITH_KNOTS('',3,(#40785,#40786,#40787,#40788,#40789,
#40790,#40791,#40792,#40793,#40794,#40795,#40796,#40797,#40798,#40799,#40800,
#40801),.UNSPECIFIED.,.F.,.F.,(4,1,1,1,1,1,1,1,1,1,1,1,1,1,4),(0.,0.125,
0.1875,0.21875,0.25,0.28125,0.3125,0.375,0.5,0.625,0.6875,0.75,0.8125,0.875,
1.),.UNSPECIFIED.);
#1057=B_SPLINE_CURVE_WITH_KNOTS('',3,(#40802,#40803,#40804,#40805,#40806,
#40807,#40808,#40809,#40810,#40811,#40812,#40813,#40814,#40815,#40816,#40817,
#40818,#40819,#40820,#40821,#40822,#40823),.UNSPECIFIED.,.F.,.F.,(4,3,3,
3,3,3,3,4),(1.21073077537255E-7,0.25,0.375,0.477137911585377,0.5,0.625,
0.75,1.),.UNSPECIFIED.);
#1058=B_SPLINE_CURVE_WITH_KNOTS('',3,(#40827,#40828,#40829,#40830,#40831,
#40832,#40833,#40834,#40835,#40836,#40837,#40838,#40839,#40840,#40841,#40842,
#40843),.UNSPECIFIED.,.F.,.F.,(4,1,1,1,1,1,1,1,1,1,1,1,1,1,4),(0.,0.125,
0.1875,0.25,0.3125,0.375,0.5,0.625,0.6875,0.71875,0.75,0.78125,0.8125,0.875,
1.),.UNSPECIFIED.);
#1059=B_SPLINE_CURVE_WITH_KNOTS('',3,(#40845,#40846,#40847,#40848,#40849,
#40850,#40851,#40852,#40853,#40854,#40855,#40856,#40857,#40858,#40859,#40860,
#40861),.UNSPECIFIED.,.F.,.F.,(4,1,1,1,1,1,1,1,1,1,1,1,1,1,4),(9.8229068389049E-8,
0.125,0.1875,0.21875,0.25,0.28125,0.3125,0.375,0.5,0.625,0.6875,0.75,0.8125,
0.875,1.),.UNSPECIFIED.);
#1060=B_SPLINE_CURVE_WITH_KNOTS('',3,(#40863,#40864,#40865,#40866),
 .UNSPECIFIED.,.F.,.F.,(4,4),(8.86637280826242E-5,1.),.UNSPECIFIED.);
#1061=B_SPLINE_CURVE_WITH_KNOTS('',3,(#40868,#40869,#40870,#40871,#40872,
#40873,#40874,#40875,#40876,#40877,#40878,#40879,#40880,#40881,#40882,#40883,
#40884),.UNSPECIFIED.,.F.,.F.,(4,1,1,1,1,1,1,1,1,1,1,1,1,1,4),(0.,0.125,
0.1875,0.25,0.3125,0.375,0.5,0.625,0.6875,0.71875,0.75,0.78125,0.8125,0.875,
0.999999976690837),.UNSPECIFIED.);
#1062=B_SPLINE_CURVE_WITH_KNOTS('',3,(#40886,#40887,#40888,#40889,#40890,
#40891,#40892,#40893,#40894,#40895,#40896,#40897,#40898,#40899,#40900,#40901,
#40902),.UNSPECIFIED.,.F.,.F.,(4,1,1,1,1,1,1,1,1,1,1,1,1,1,4),(2.52343280623569E-8,
0.125,0.1875,0.21875,0.25,0.28125,0.3125,0.375,0.5,0.625,0.6875,0.75,0.8125,
0.875,1.),.UNSPECIFIED.);
#1063=B_SPLINE_CURVE_WITH_KNOTS('',3,(#40903,#40904,#40905,#40906),
 .UNSPECIFIED.,.F.,.F.,(4,4),(0.,0.999911620910334),.UNSPECIFIED.);
#1064=B_SPLINE_CURVE_WITH_KNOTS('',3,(#40910,#40911,#40912,#40913,#40914,
#40915,#40916,#40917,#40918,#40919,#40920,#40921,#40922,#40923,#40924,#40925,
#40926,#40927,#40928),.UNSPECIFIED.,.F.,.F.,(4,3,3,3,3,3,4),(0.,0.25,0.375,
0.5,0.625,0.75,1.),.UNSPECIFIED.);
#1065=B_SPLINE_CURVE_WITH_KNOTS('',3,(#40930,#40931,#40932,#40933,#40934,
#40935,#40936,#40937,#40938,#40939,#40940,#40941,#40942,#40943,#40944,#40945,
#40946),.UNSPECIFIED.,.F.,.F.,(4,1,1,1,1,1,1,1,1,1,1,1,1,1,4),(0.,0.125,
0.1875,0.25,0.3125,0.375,0.5,0.625,0.6875,0.71875,0.75,0.78125,0.8125,0.875,
0.999999985754337),.UNSPECIFIED.);
#1066=B_SPLINE_CURVE_WITH_KNOTS('',3,(#40948,#40949,#40950,#40951,#40952,
#40953,#40954,#40955),.UNSPECIFIED.,.F.,.F.,(4,2,2,4),(0.190745761082819,
0.195318232891979,0.294499389363961,0.344632001218864),.UNSPECIFIED.);
#1067=B_SPLINE_CURVE_WITH_KNOTS('',3,(#40957,#40958,#40959,#40960,#40961,
#40962,#40963,#40964,#40965,#40966,#40967,#40968,#40969,#40970,#40971,#40972,
#40973,#40974,#40975),.UNSPECIFIED.,.F.,.F.,(4,3,3,3,3,3,4),(0.00444335916602599,
0.25,0.375,0.5,0.625,0.75,1.),.UNSPECIFIED.);
#1068=B_SPLINE_CURVE_WITH_KNOTS('',3,(#40977,#40978,#40979,#40980,#40981,
#40982),.UNSPECIFIED.,.F.,.F.,(4,2,4),(0.695401129409354,0.724410509776768,
0.80598859149533),.UNSPECIFIED.);
#1069=B_SPLINE_CURVE_WITH_KNOTS('',3,(#40983,#40984,#40985,#40986,#40987,
#40988),.UNSPECIFIED.,.F.,.F.,(4,2,4),(0.663566354634175,0.697565900531653,
0.775630565396341),.UNSPECIFIED.);
#1070=B_SPLINE_CURVE_WITH_KNOTS('',3,(#41006,#41007,#41008,#41009,#41010,
#41011,#41012,#41013,#41014,#41015,#41016,#41017,#41018,#41019),
 .UNSPECIFIED.,.F.,.F.,(4,2,2,2,2,2,4),(-0.01507830543452,-0.0131185429662993,
-0.0110343515831027,-0.00717762894557236,-0.00331925504980651,-7.55493420441511E-7,
0.000663167325391246),.UNSPECIFIED.);
#1071=B_SPLINE_CURVE_WITH_KNOTS('',3,(#41020,#41021,#41022,#41023,#41024,
#41025,#41026,#41027,#41028,#41029,#41030,#41031,#41032,#41033,#41034),
 .UNSPECIFIED.,.F.,.F.,(4,2,2,2,2,2,1,4),(0.000110379421385148,0.00233264133731716,
0.00497678284857156,0.00924166096140105,0.0134515198447832,0.0196622706603402,
0.0205807311791432,0.0214991916979463),.UNSPECIFIED.);
#1072=B_SPLINE_CURVE_WITH_KNOTS('',3,(#41036,#41037,#41038,#41039,#41040,
#41041,#41042,#41043,#41044,#41045,#41046,#41047,#41048,#41049,#41050),
 .UNSPECIFIED.,.F.,.F.,(4,2,2,2,2,2,1,4),(-0.0107327112951072,-0.00932351786082577,
-0.00775928892532341,-0.00524294687388514,-0.00290996407673086,0.,0.000360584068865346,
0.000721168137730691),.UNSPECIFIED.);
#1073=B_SPLINE_CURVE_WITH_KNOTS('',3,(#41066,#41067,#41068,#41069,#41070,
#41071,#41072,#41073,#41074,#41075,#41076,#41077,#41078,#41079,#41080),
 .UNSPECIFIED.,.F.,.F.,(4,1,2,2,2,2,2,4),(-0.000831847091679277,-0.000415718710644378,
4.09670390521676E-7,0.0033967242603589,0.00614729864505439,0.00905447795736422,
0.0108472486697068,0.0123547719820523),.UNSPECIFIED.);
#1074=B_SPLINE_CURVE_WITH_KNOTS('',3,(#41096,#41097,#41098,#41099,#41100,
#41101,#41102,#41103,#41104,#41105,#41106),.UNSPECIFIED.,.F.,.F.,(4,2,2,
2,1,4),(-0.0100540276238623,-0.00756834425613214,-0.00473757454927083,-0.00188169994745774,
-9.55994444132124E-5,0.),.UNSPECIFIED.);
#1075=B_SPLINE_CURVE_WITH_KNOTS('',3,(#41108,#41109,#41110,#41111,#41112,
#41113,#41114,#41115,#41116,#41117,#41118,#41119,#41120,#41121,#41122,#41123),
 .UNSPECIFIED.,.F.,.F.,(4,2,2,2,2,2,2,4),(0.0109454996995501,0.0121640780030457,
0.0143626163448094,0.0170563730060771,0.0211889870954567,0.0237556002878168,
0.0248641156521573,0.0252222827077722),.UNSPECIFIED.);
#1076=B_SPLINE_CURVE_WITH_KNOTS('',3,(#41140,#41141,#41142,#41143,#41144,
#41145,#41146,#41147,#41148,#41149,#41150,#41151,#41152,#41153),
 .UNSPECIFIED.,.F.,.F.,(4,2,2,2,2,2,4),(-0.0150736213696635,-0.0131145281722507,
-0.0110310296272098,-0.00717567152716654,-0.0033185625050402,-7.27641435771531E-7,
0.000662519455103558),.UNSPECIFIED.);
#1077=B_SPLINE_CURVE_WITH_KNOTS('',3,(#41154,#41155,#41156,#41157,#41158,
#41159,#41160,#41161,#41162,#41163,#41164,#41165,#41166,#41167,#41168),
 .UNSPECIFIED.,.F.,.F.,(4,2,2,2,2,2,1,4),(0.000109277498535426,0.00233122821911415,
0.0049736263892055,0.00923726610637425,0.0133900437988086,0.0195564321408132,
0.0207410647190443,0.0219256972972754),.UNSPECIFIED.);
#1078=B_SPLINE_CURVE_WITH_KNOTS('',3,(#41170,#41171,#41172,#41173,#41174,
#41175,#41176,#41177,#41178,#41179,#41180,#41181,#41182,#41183,#41184),
 .UNSPECIFIED.,.F.,.F.,(4,2,2,2,2,2,1,4),(-0.0111927944725922,-0.00971535165057207,
-0.00807540492660865,-0.00543708380189962,-0.00299063929573346,0.,0.000367166839165872,
0.000734333678331744),.UNSPECIFIED.);
#1079=B_SPLINE_CURVE_WITH_KNOTS('',3,(#41200,#41201,#41202,#41203,#41204,
#41205,#41206,#41207,#41208,#41209,#41210,#41211,#41212,#41213,#41214),
 .UNSPECIFIED.,.F.,.F.,(4,1,2,2,2,2,2,4),(-0.000841606462170108,-0.000420623329405298,
3.59803359512067E-7,0.00341940295621038,0.00619678753011438,0.00913724210812968,
0.010951633465127,0.0124778685491557),.UNSPECIFIED.);
#1080=B_SPLINE_CURVE_WITH_KNOTS('',3,(#41230,#41231,#41232,#41233,#41234,
#41235,#41236,#41237,#41238,#41239,#41240,#41241,#41242,#41243),
 .UNSPECIFIED.,.F.,.F.,(4,2,2,2,2,2,4),(-0.0126310563478074,-0.0110402596235953,
-0.00932700685802013,-0.00615674109370743,-0.00298505983244596,0.,0.000652684360861046),
 .UNSPECIFIED.);
#1081=B_SPLINE_CURVE_WITH_KNOTS('',3,(#41245,#41246,#41247,#41248,#41249,
#41250,#41251,#41252,#41253,#41254,#41255,#41256,#41257,#41258),
 .UNSPECIFIED.,.F.,.F.,(4,2,2,2,2,2,4),(0.,0.00233205662631541,0.00492501613407614,
0.00904723499130749,0.0129234630237897,0.0187564284015468,0.0218496675394978),
 .UNSPECIFIED.);
#1082=B_SPLINE_CURVE_WITH_KNOTS('',3,(#41289,#41290,#41291,#41292,#41293,
#41294,#41295,#41296,#41297,#41298,#41299,#41300,#41301,#41302),
 .UNSPECIFIED.,.F.,.F.,(4,2,2,2,2,2,4),(-0.015067945938605,-0.0131096675981174,
-0.0110270176791167,-0.0071733025740434,-0.00331774097657231,-6.94603856923534E-7,
0.000661736637824425),.UNSPECIFIED.);
#1083=B_SPLINE_CURVE_WITH_KNOTS('',3,(#41303,#41304,#41305,#41306,#41307,
#41308,#41309,#41310,#41311,#41312,#41313,#41314,#41315,#41316),
 .UNSPECIFIED.,.F.,.F.,(4,2,2,2,2,2,4),(0.000108411815062279,0.00233046514898696,
0.00497190484499379,0.00923486963259684,0.0133609629567941,0.0174716316940529,
0.018064453437383),.UNSPECIFIED.);
#1084=B_SPLINE_CURVE_WITH_KNOTS('',3,(#41318,#41319,#41320,#41321,#41322,
#41323,#41324,#41325,#41326,#41327,#41328,#41329,#41330,#41331,#41332),
 .UNSPECIFIED.,.F.,.F.,(4,2,2,2,2,2,1,4),(-0.0112911210319579,-0.00979969372819557,
-0.00814422742212235,-0.00548091191237493,-0.00301110838872929,0.,0.000370911555962369,
0.000741823111924738),.UNSPECIFIED.);
#1085=B_SPLINE_CURVE_WITH_KNOTS('',3,(#41348,#41349,#41350,#41351,#41352,
#41353,#41354,#41355,#41356,#41357,#41358,#41359,#41360,#41361,#41362),
 .UNSPECIFIED.,.F.,.F.,(4,1,2,2,2,2,2,4),(-0.000845952505115191,-0.000422815860888459,
3.20783338272771E-7,0.00342787238279231,0.00621649248522469,0.0091738937142793,
0.0109998757388608,0.0125362536341693),.UNSPECIFIED.);
#1086=B_SPLINE_CURVE_WITH_KNOTS('',3,(#41378,#41379,#41380,#41381,#41382,
#41383,#41384,#41385,#41386,#41387,#41388,#41389,#41390,#41391),
 .UNSPECIFIED.,.F.,.F.,(4,2,2,2,2,2,4),(-0.0122863233744583,-0.0107429899947187,
-0.00908185001333585,-0.00600812479454555,-0.00293295547261242,0.,0.000649621328147838),
 .UNSPECIFIED.);
#1087=B_SPLINE_CURVE_WITH_KNOTS('',3,(#41393,#41394,#41395,#41396,#41397,
#41398,#41399,#41400,#41401,#41402,#41403,#41404,#41405,#41406),
 .UNSPECIFIED.,.F.,.F.,(4,2,2,2,2,2,4),(0.,0.00233208722840324,0.00492509994382487,
0.0090473081885449,0.012910133820222,0.0166890239584757,0.0172660039537804),
 .UNSPECIFIED.);
#1088=B_SPLINE_CURVE_WITH_KNOTS('',3,(#41437,#41438,#41439,#41440,#41441,
#41442,#41443,#41444,#41445,#41446,#41447,#41448,#41449,#41450),
 .UNSPECIFIED.,.F.,.F.,(4,2,2,2,2,2,4),(-0.0150618266103595,-0.0131044294361987,
-0.0110226997841704,-0.00717075164604429,-0.00331686670257359,-6.61750749050491E-7,
0.000660888945518815),.UNSPECIFIED.);
#1089=B_SPLINE_CURVE_WITH_KNOTS('',3,(#41451,#41452,#41453,#41454,#41455,
#41456,#41457,#41458,#41459,#41460,#41461,#41462,#41463,#41464),
 .UNSPECIFIED.,.F.,.F.,(4,2,2,2,2,2,4),(0.000107524573743238,0.00233075355229494,
0.00497250195749481,0.00923570004390666,0.0133716966279069,0.0197477605613191,
0.0233570440188243),.UNSPECIFIED.);
#1090=B_SPLINE_CURVE_WITH_KNOTS('',3,(#41466,#41467,#41468,#41469,#41470,
#41471,#41472,#41473,#41474,#41475,#41476,#41477,#41478,#41479,#41480),
 .UNSPECIFIED.,.F.,.F.,(4,2,2,2,2,2,1,4),(-0.0112689852378272,-0.00978070704858543,
-0.0081286839041701,-0.00547107361921424,-0.00300660551843908,0.,0.000370059615394522,
0.000740119230789043),.UNSPECIFIED.);
#1091=B_SPLINE_CURVE_WITH_KNOTS('',3,(#41496,#41497,#41498,#41499,#41500,
#41501,#41502,#41503,#41504,#41505,#41506,#41507,#41508,#41509,#41510),
 .UNSPECIFIED.,.F.,.F.,(4,1,2,2,2,2,2,4),(-0.000852309778855015,-0.000426014539963934,
2.80698927146807E-7,0.00344207743051125,0.00624846680252986,0.00922991249153885,
0.0110719050982193,0.0126221279026672),.UNSPECIFIED.);
#1092=B_SPLINE_CURVE_WITH_KNOTS('',3,(#41526,#41527,#41528,#41529,#41530,
#41531,#41532,#41533,#41534,#41535,#41536,#41537,#41538,#41539),
 .UNSPECIFIED.,.F.,.F.,(4,2,2,2,2,2,4),(-0.0112537356406148,-0.0098521206422284,
-0.00834440416079227,-0.0055546808585686,-0.0027635731133648,0.,0.000645987732377855),
 .UNSPECIFIED.);
#1093=B_SPLINE_CURVE_WITH_KNOTS('',3,(#41541,#41542,#41543,#41544,#41545,
#41546,#41547,#41548,#41549,#41550,#41551,#41552,#41553,#41554),
 .UNSPECIFIED.,.F.,.F.,(4,2,2,2,2,2,4),(0.,0.0023321032472572,0.0049251475977755,
0.00904732760149453,0.0128912897831174,0.0181134987013173,0.0197352105609782),
 .UNSPECIFIED.);
#1094=B_SPLINE_CURVE_WITH_KNOTS('',3,(#41585,#41586,#41587,#41588,#41589,
#41590,#41591,#41592,#41593,#41594,#41595,#41596,#41597),.UNSPECIFIED.,
 .F.,.F.,(4,2,2,2,2,1,4),(0.,0.00196346055139926,0.00405154240681477,0.00791565834815476,
0.011781209799845,0.0156720041993471,0.0157373755669737),.UNSPECIFIED.);
#1095=B_SPLINE_CURVE_WITH_KNOTS('',3,(#41598,#41599,#41600,#41601,#41602,
#41603,#41604,#41605,#41606,#41607,#41608,#41609,#41610,#41611,#41612),
 .UNSPECIFIED.,.F.,.F.,(4,2,2,2,2,2,1,4),(0.000114739303757549,0.0023334430315381,
0.00497816475940246,0.00924233839267071,0.013514656302117,0.01989139391585,
0.0206513029014127,0.0214112118869755),.UNSPECIFIED.);
#1096=B_SPLINE_CURVE_WITH_KNOTS('',3,(#41614,#41615,#41616,#41617,#41618,
#41619,#41620,#41621,#41622,#41623,#41624,#41625,#41626,#41627,#41628),
 .UNSPECIFIED.,.F.,.F.,(4,2,2,2,2,2,1,4),(-0.0103555407250338,-0.00899996641982785,
-0.00749506887131186,-0.00507443351976568,-0.00283082962523163,-2.71882089498271E-8,
0.000345077207643678,0.000690181603496307),.UNSPECIFIED.);
#1097=B_SPLINE_CURVE_WITH_KNOTS('',3,(#41644,#41645,#41646,#41647,#41648,
#41649,#41650,#41651,#41652,#41653,#41654,#41655,#41656,#41657,#41658),
 .UNSPECIFIED.,.F.,.F.,(4,1,2,2,2,2,2,4),(-0.000788977077809716,-0.000394173563697078,
6.29950415558791E-7,0.00329621038696056,0.00593031022203129,0.00869747301509253,
0.0104000877764451,0.0118299274704398),.UNSPECIFIED.);
#1098=B_SPLINE_CURVE_WITH_KNOTS('',3,(#41674,#41675,#41676,#41677,#41678,
#41679,#41680,#41681,#41682,#41683,#41684,#41685,#41686),.UNSPECIFIED.,
 .F.,.F.,(4,2,2,2,2,1,4),(3.14269389793808E-5,0.0019634367265874,0.00405149149102325,
0.00791568233580109,0.0117813314665308,0.0182072596508539,0.0189955540620671),
 .UNSPECIFIED.);
#1099=B_SPLINE_CURVE_WITH_KNOTS('',3,(#41688,#41689,#41690,#41691,#41692,
#41693,#41694,#41695,#41696,#41697,#41698,#41699,#41700,#41701,#41702),
 .UNSPECIFIED.,.F.,.F.,(4,2,2,2,2,2,1,4),(0.,0.00233324186650626,0.00492806572685197,
0.00905241385642049,0.0130581050133669,0.0189330953861274,0.0196729935413677,
0.020412891696608),.UNSPECIFIED.);
#1100=B_SPLINE_CURVE_WITH_KNOTS('',3,(#41733,#41734,#41735,#41736,#41737,
#41738,#41739,#41740,#41741,#41742,#41743,#41744,#41745,#41746),
 .UNSPECIFIED.,.F.,.F.,(4,2,2,2,2,2,4),(-0.0150495343999896,-0.0130939107218886,
-0.0110140328587893,-0.00716563542438969,-0.00331511579488975,-5.99773702798442E-7,
0.000659170132904621),.UNSPECIFIED.);
#1101=B_SPLINE_CURVE_WITH_KNOTS('',3,(#41747,#41748,#41749,#41750,#41751,
#41752,#41753,#41754,#41755,#41756,#41757,#41758,#41759,#41760,#41761),
 .UNSPECIFIED.,.F.,.F.,(4,2,2,2,2,2,1,4),(0.000106052581580669,0.00232820999548284,
0.00496681683786704,0.00922777203689892,0.0132846981695113,0.0188863847946317,
0.0192382229087076,0.0195900610227836),.UNSPECIFIED.);
#1102=B_SPLINE_CURVE_WITH_KNOTS('',3,(#41763,#41764,#41765,#41766,#41767,
#41768,#41769,#41770,#41771,#41772,#41773,#41774,#41775,#41776,#41777),
 .UNSPECIFIED.,.F.,.F.,(4,2,2,2,2,2,1,4),(-0.0115842429505587,-0.0100510264851629,
-0.00834917125888717,-0.00561121344317483,-0.00307176429142002,0.,0.000381702300701627,
0.000763404601403253),.UNSPECIFIED.);
#1103=B_SPLINE_CURVE_WITH_KNOTS('',3,(#41793,#41794,#41795,#41796,#41797,
#41798,#41799,#41800,#41801,#41802,#41803,#41804,#41805,#41806,#41807),
 .UNSPECIFIED.,.F.,.F.,(4,1,2,2,2,2,2,4),(-0.000880146681302628,-0.000439983912980285,
1.78855342058124E-7,0.00390653624110326,0.00730515376515244,0.0109221460955771,
0.0131581175541924,0.0150406638244627),.UNSPECIFIED.);
#1104=B_SPLINE_CURVE_WITH_KNOTS('',3,(#41823,#41824,#41825,#41826,#41827,
#41828,#41829,#41830,#41831,#41832,#41833,#41834,#41835,#41836,#41837),
 .UNSPECIFIED.,.F.,.F.,(4,2,2,2,2,2,1,4),(-0.0133513511352758,-0.011657592117576,
-0.00983788659285601,-0.00647112579959316,-0.00310254776237713,0.,0.000318746772545248,
0.000637493545090497),.UNSPECIFIED.);
#1105=B_SPLINE_CURVE_WITH_KNOTS('',3,(#41839,#41840,#41841,#41842,#41843,
#41844,#41845,#41846,#41847,#41848,#41849,#41850,#41851,#41852,#41853),
 .UNSPECIFIED.,.F.,.F.,(4,2,2,2,2,2,1,4),(0.,0.00233178099632009,0.00492433938161485,
0.0090459596421507,0.0128089241713556,0.0177017983313787,0.0182620427457793,
0.0188222871601798),.UNSPECIFIED.);
#1106=B_SPLINE_CURVE_WITH_KNOTS('',3,(#41887,#41888,#41889,#41890,#41891,
#41892,#41893,#41894,#41895,#41896,#41897,#41898,#41899),.UNSPECIFIED.,
 .F.,.F.,(4,2,2,2,2,1,4),(0.,0.00196326848972203,0.00405116207364883,0.00791555727476664,
0.0117816205713716,0.0181921635821883,0.0189428821816501),.UNSPECIFIED.);
#1107=B_SPLINE_CURVE_WITH_KNOTS('',3,(#41900,#41901,#41902,#41903,#41904,
#41905,#41906,#41907,#41908,#41909,#41910,#41911,#41912,#41913,#41914),
 .UNSPECIFIED.,.F.,.F.,(4,2,2,2,2,2,1,4),(0.000136572166951063,0.00247342851894918,
0.00532496585133604,0.00983368386008723,0.0137734612749379,0.0191740995937165,
0.0195771026144167,0.0199801056351169),.UNSPECIFIED.);
#1108=B_SPLINE_CURVE_WITH_KNOTS('',3,(#41916,#41917,#41918,#41919),
 .UNSPECIFIED.,.F.,.F.,(4,4),(8.3932008892544E-11,0.000180398243040848),
 .UNSPECIFIED.);
#1109=B_SPLINE_CURVE_WITH_KNOTS('',3,(#41938,#41939,#41940,#41941,#41942,
#41943,#41944,#41945,#41946,#41947,#41948,#41949,#41950,#41951,#41952,#41953,
#41954,#41955,#41956,#41957,#41958,#41959,#41960,#41961,#41962,#41963,#41964,
#41965),.UNSPECIFIED.,.F.,.F.,(4,2,2,2,2,2,2,2,2,2,2,2,2,4),(0.00894662764801732,
0.00909966464154512,0.00911121326348854,0.0091199542058202,0.00912623258445597,
0.00913058031359492,0.00929759041527048,0.0098850490504378,0.0106648416904178,
0.0139432102084079,0.0202273547328932,0.0255820468844395,0.0289792940110764,
0.0317584900748122),.UNSPECIFIED.);
#1110=B_SPLINE_CURVE_WITH_KNOTS('',3,(#41984,#41985,#41986,#41987,#41988,
#41989,#41990,#41991,#41992,#41993,#41994,#41995,#41996,#41997,#41998,#41999,
#42000),.UNSPECIFIED.,.F.,.F.,(4,2,2,2,2,2,2,1,4),(4.1951250921174E-5,0.00196435693919538,
0.00405344923205659,0.00791854639957213,0.0117851888818974,0.0158670573322602,
0.0160255880433537,0.0161000392070421,0.0162193043519429),.UNSPECIFIED.);
#1111=B_SPLINE_CURVE_WITH_KNOTS('',3,(#42002,#42003,#42004,#42005,#42006,
#42007,#42008,#42009,#42010,#42011,#42012,#42013,#42014,#42015,#42016),
 .UNSPECIFIED.,.F.,.F.,(4,2,2,2,2,2,1,4),(0.,0.00229420255473759,0.00482815180681898,
0.0090803315048094,0.013385498353122,0.0196056546104732,0.0205956034810639,
0.0215855523516545),.UNSPECIFIED.);
#1112=B_SPLINE_CURVE_WITH_KNOTS('',3,(#42050,#42051,#42052,#42053,#42054,
#42055,#42056,#42057,#42058,#42059,#42060,#42061,#42062,#42063),
 .UNSPECIFIED.,.F.,.F.,(4,2,2,2,2,2,4),(-0.015055943205555,-0.0130993943583035,
-0.0110185504070684,-0.0071683015355778,-0.00331602697752475,-6.31338995112432E-7,
0.000660068888145464),.UNSPECIFIED.);
#1113=B_SPLINE_CURVE_WITH_KNOTS('',3,(#42064,#42065,#42066,#42067,#42068,
#42069,#42070,#42071,#42072,#42073,#42074,#42075,#42076,#42077,#42078),
 .UNSPECIFIED.,.F.,.F.,(4,2,2,2,2,2,1,4),(0.000106892049855475,0.00233143420029682,
0.00497395335443926,0.00923768954676918,0.013398888189913,0.0195568925545534,
0.0206769167852616,0.0217969410159699),.UNSPECIFIED.);
#1114=B_SPLINE_CURVE_WITH_KNOTS('',3,(#42080,#42081,#42082,#42083,#42084,
#42085,#42086,#42087,#42088,#42089,#42090,#42091,#42092,#42093,#42094),
 .UNSPECIFIED.,.F.,.F.,(4,2,2,2,2,2,1,4),(-0.0111954009729321,-0.0097175856695965,
-0.00807710698695868,-0.00543830669534266,-0.00299142164096204,0.,0.000367280343763525,
0.000734560687527049),.UNSPECIFIED.);
#1115=B_SPLINE_CURVE_WITH_KNOTS('',3,(#42110,#42111,#42112,#42113,#42114,
#42115,#42116,#42117,#42118,#42119,#42120,#42121,#42122,#42123,#42124),
 .UNSPECIFIED.,.F.,.F.,(4,1,2,2,2,2,2,4),(-0.000861296926150031,-0.00043052882115021,
2.39283849611752E-7,0.0038927349112584,0.0072753761053844,0.0108691153816805,
0.0130893297188529,0.014958222467424),.UNSPECIFIED.);
#1116=B_SPLINE_CURVE_WITH_KNOTS('',3,(#42140,#42141,#42142,#42143,#42144,
#42145,#42146,#42147,#42148,#42149,#42150,#42151,#42152,#42153),
 .UNSPECIFIED.,.F.,.F.,(4,2,2,2,2,2,4),(-0.0111679208697887,-0.00977760366207731,
-0.0082830305279969,-0.00551771990195264,-0.0027509784102351,0.,0.000641921215264818),
 .UNSPECIFIED.);
#1117=B_SPLINE_CURVE_WITH_KNOTS('',3,(#42155,#42156,#42157,#42158,#42159,
#42160,#42161,#42162,#42163,#42164,#42165,#42166,#42167,#42168),
 .UNSPECIFIED.,.F.,.F.,(4,2,2,2,2,2,4),(0.,0.0023320376215534,0.00492498614474746,
0.00904702037128976,0.0128643072555835,0.0182355035241461,0.020352993324196),
 .UNSPECIFIED.);
#1118=B_SPLINE_CURVE_WITH_KNOTS('',3,(#42199,#42200,#42201,#42202,#42203,
#42204,#42205,#42206,#42207,#42208,#42209,#42210,#42211),.UNSPECIFIED.,
 .F.,.F.,(4,2,2,2,2,1,4),(-0.00785439775943529,-0.00694783516724324,-0.00598372616180969,
-0.00419962083761066,-0.00241481918361066,-4.02804812405996E-7,4.97241742472335E-5),
 .UNSPECIFIED.);
#1119=B_SPLINE_CURVE_WITH_KNOTS('',3,(#42212,#42213,#42214,#42215,#42216,
#42217,#42218,#42219,#42220,#42221,#42222,#42223,#42224,#42225,#42226),
 .UNSPECIFIED.,.F.,.F.,(4,2,2,2,2,2,1,4),(0.000111276481820315,0.00233269010494002,
0.00497708127010691,0.00924237493668451,0.0134510062558102,0.0196593549777347,
0.0205845154023894,0.0215096758270441),.UNSPECIFIED.);
#1120=B_SPLINE_CURVE_WITH_KNOTS('',3,(#42228,#42229,#42230,#42231,#42232,
#42233,#42234,#42235,#42236,#42237,#42238,#42239,#42240,#42241,#42242),
 .UNSPECIFIED.,.F.,.F.,(4,2,2,2,2,2,1,4),(-0.0105397741274358,-0.0091581563716996,
-0.00762462685010155,-0.00515737932018193,-0.00286969551484454,-8.51844338470298E-9,
0.000352910589692364,0.000705829697828113),.UNSPECIFIED.);
#1121=B_SPLINE_CURVE_WITH_KNOTS('',3,(#42258,#42259,#42260,#42261,#42262,
#42263,#42264,#42265,#42266,#42267,#42268,#42269,#42270,#42271,#42272),
 .UNSPECIFIED.,.F.,.F.,(4,1,2,2,2,2,2,4),(-0.000811689830736768,-0.000405547746171915,
5.94338392938157E-7,0.00333387706802661,0.00601768004150032,0.0088698255226293,
0.0106324256073501,0.0121139768793991),.UNSPECIFIED.);
#1122=B_SPLINE_CURVE_WITH_KNOTS('',3,(#42288,#42289,#42290,#42291,#42292,
#42293,#42294,#42295,#42296,#42297,#42298,#42299,#42300),.UNSPECIFIED.,
 .F.,.F.,(4,2,2,2,2,1,4),(-0.0105931122047967,-0.00934770902821425,-0.00800490542156122,
-0.0055199269461594,-0.00303397666856782,0.,6.34168513411634E-5),
 .UNSPECIFIED.);
#1123=B_SPLINE_CURVE_WITH_KNOTS('',3,(#42302,#42303,#42304,#42305,#42306,
#42307,#42308,#42309,#42310,#42311,#42312,#42313,#42314,#42315,#42316),
 .UNSPECIFIED.,.F.,.F.,(4,2,2,2,2,2,1,4),(0.,0.00232779176441591,0.00491551587469812,
0.00903475405431627,0.0129741800549623,0.0186882063450052,0.019607760317714,
0.0205273142904227),.UNSPECIFIED.);
#1124=B_SPLINE_CURVE_WITH_KNOTS('',3,(#42347,#42348,#42349,#42350,#42351,
#42352,#42353,#42354,#42355,#42356,#42357,#42358,#42359),.UNSPECIFIED.,
 .F.,.F.,(4,2,2,2,2,1,4),(-0.0085716535892449,-0.00757466960194273,-0.00651440028288434,
-0.0045523430563402,-0.00258952361985675,-4.44344898067189E-7,5.49800542840583E-5),
 .UNSPECIFIED.);
#1125=B_SPLINE_CURVE_WITH_KNOTS('',3,(#42360,#42361,#42362,#42363,#42364,
#42365,#42366,#42367,#42368,#42369,#42370,#42371,#42372,#42373,#42374),
 .UNSPECIFIED.,.F.,.F.,(4,2,2,2,2,2,1,4),(0.000112127479441767,0.00233289939706983,
0.00497738360754069,0.00924236727099269,0.0134674534094052,0.0197117179381725,
0.0205879706113953,0.0214642232846181),.UNSPECIFIED.);
#1126=B_SPLINE_CURVE_WITH_KNOTS('',3,(#42376,#42377,#42378,#42379,#42380,
#42381,#42382,#42383,#42384,#42385,#42386,#42387,#42388,#42389,#42390),
 .UNSPECIFIED.,.F.,.F.,(4,2,2,2,2,2,1,4),(-0.0104881836929382,-0.00911386915215036,
-0.00758836984497876,-0.00513419361121672,-0.00285886238502574,-1.287952204089E-8,
0.000350823059822679,0.0007016589991674),.UNSPECIFIED.);
#1127=B_SPLINE_CURVE_WITH_KNOTS('',3,(#42406,#42407,#42408,#42409,#42410,
#42411,#42412,#42413,#42414,#42415,#42416,#42417,#42418,#42419,#42420),
 .UNSPECIFIED.,.F.,.F.,(4,1,2,2,2,2,2,4),(-0.000792937822276422,-0.000396163246703989,
6.11328868443299E-7,0.00328748317884194,0.00591926510315487,0.00871205474317156,
0.0104370897693979,0.0118870329010417),.UNSPECIFIED.);
#1128=B_SPLINE_CURVE_WITH_KNOTS('',3,(#42436,#42437,#42438,#42439,#42440,
#42441,#42442,#42443,#42444,#42445,#42446,#42447,#42448),.UNSPECIFIED.,
 .F.,.F.,(4,2,2,2,2,1,4),(-0.00632636884576775,-0.00561706452187852,-0.00485183122085223,
-0.00343569349346982,-0.00201900471914639,0.,3.19199699655112E-5),
 .UNSPECIFIED.);
#1129=B_SPLINE_CURVE_WITH_KNOTS('',3,(#42450,#42451,#42452,#42453,#42454,
#42455,#42456,#42457,#42458,#42459,#42460,#42461,#42462,#42463,#42464),
 .UNSPECIFIED.,.F.,.F.,(4,2,2,2,2,2,1,4),(0.,0.00232848787311146,0.00491736409388601,
0.00903785504559387,0.013060779628687,0.0189785945344682,0.0196952694771613,
0.0204119444198545),.UNSPECIFIED.);
#1130=B_SPLINE_CURVE_WITH_KNOTS('',3,(#42495,#42496,#42497,#42498,#42499,
#42500,#42501,#42502,#42503,#42504,#42505,#42506,#42507),.UNSPECIFIED.,
 .F.,.F.,(4,2,2,2,2,1,4),(-0.0156746030251293,-0.0137108965814205,-0.0116225427742933,
-0.0077579753523329,-0.00389191820682102,-4.8072468667934E-7,6.54569592049717E-5),
 .UNSPECIFIED.);
#1131=B_SPLINE_CURVE_WITH_KNOTS('',3,(#42508,#42509,#42510,#42511,#42512,
#42513,#42514,#42515,#42516,#42517,#42518,#42519,#42520,#42521,#42522),
 .UNSPECIFIED.,.F.,.F.,(4,2,2,2,2,2,1,4),(0.00011297725140699,0.00233326265007159,
0.00497803831869269,0.00924288561238248,0.0134933353480553,0.0198043992888978,
0.0206163190377781,0.0214282387866584),.UNSPECIFIED.);
#1132=B_SPLINE_CURVE_WITH_KNOTS('',3,(#42524,#42525,#42526,#42527,#42528,
#42529,#42530,#42531,#42532,#42533,#42534,#42535,#42536,#42537,#42538),
 .UNSPECIFIED.,.F.,.F.,(4,2,2,2,2,2,1,4),(-0.0104230568527555,-0.00905794707620465,
-0.00754258263594496,-0.00510489078265507,-0.0028451140281092,-1.83565382009393E-8,
0.000348073673261863,0.000696165703061926),.UNSPECIFIED.);
#1133=B_SPLINE_CURVE_WITH_KNOTS('',3,(#42554,#42555,#42556,#42557,#42558,
#42559,#42560,#42561,#42562,#42563,#42564,#42565,#42566,#42567,#42568),
 .UNSPECIFIED.,.F.,.F.,(4,1,2,2,2,2,2,4),(-0.000796385399367999,-0.00039789197282334,
6.01453721317817E-7,0.00330857856143206,0.00595907914351395,0.00875202157016118,
0.0104725301786227,0.0119190167735485),.UNSPECIFIED.);
#1134=B_SPLINE_CURVE_WITH_KNOTS('',3,(#42584,#42585,#42586,#42587,#42588,
#42589,#42590,#42591,#42592,#42593,#42594,#42595,#42596),.UNSPECIFIED.,
 .F.,.F.,(4,2,2,2,2,1,4),(-0.00114042523245899,-0.00101957547515334,-0.000889119527853727,
-0.00064769685874317,-0.000406180953020858,0.,6.52267443316575E-5),
 .UNSPECIFIED.);
#1135=B_SPLINE_CURVE_WITH_KNOTS('',3,(#42598,#42599,#42600,#42601,#42602,
#42603,#42604,#42605,#42606,#42607,#42608,#42609,#42610,#42611,#42612),
 .UNSPECIFIED.,.F.,.F.,(4,2,2,2,2,2,1,4),(0.,0.00233245052595259,0.00492601376639143,
0.009049051688289,0.0130249488395919,0.0188184019519407,0.0196232789088459,
0.0204281558657512),.UNSPECIFIED.);
#1136=B_SPLINE_CURVE_WITH_KNOTS('',3,(#42643,#42644,#42645,#42646,#42647,
#42648,#42649,#42650,#42651,#42652,#42653,#42654,#42655),.UNSPECIFIED.,
 .F.,.F.,(4,2,2,2,2,1,4),(0.,0.00196351159177689,0.00405165736140035,0.00791583594583384,
0.0117814988291894,0.015672372049312,0.015737753906218),.UNSPECIFIED.);
#1137=B_SPLINE_CURVE_WITH_KNOTS('',3,(#42656,#42657,#42658,#42659,#42660,
#42661,#42662,#42663,#42664,#42665,#42666,#42667,#42668,#42669,#42670),
 .UNSPECIFIED.,.F.,.F.,(4,2,2,2,2,2,1,4),(0.000113883995237668,0.00233233712716634,
0.00497583829970885,0.00923940492023475,0.0134494508874806,0.0196608351532728,
0.0205767816286905,0.0214927281041083),.UNSPECIFIED.);
#1138=B_SPLINE_CURVE_WITH_KNOTS('',3,(#42672,#42673,#42674,#42675,#42676,
#42677,#42678,#42679,#42680,#42681,#42682,#42683,#42684,#42685,#42686),
 .UNSPECIFIED.,.F.,.F.,(4,2,2,2,2,2,1,4),(-0.0105033578550783,-0.0091269097672519,
-0.00759894321490606,-0.00514090077078628,-0.00286219709327909,-1.13168538602715E-8,
0.000351419063789825,0.000702849444433509),.UNSPECIFIED.);
#1139=B_SPLINE_CURVE_WITH_KNOTS('',3,(#42702,#42703,#42704,#42705,#42706,
#42707,#42708,#42709,#42710,#42711,#42712,#42713,#42714,#42715,#42716),
 .UNSPECIFIED.,.F.,.F.,(4,1,2,2,2,2,2,4),(-0.000760560840304545,-0.00037994807411008,
6.64692084385941E-7,0.00319739705683137,0.00571058681035043,0.00835475150748551,
0.00998261483882353,0.0113501898484002),.UNSPECIFIED.);
#1140=B_SPLINE_CURVE_WITH_KNOTS('',3,(#42732,#42733,#42734,#42735,#42736,
#42737,#42738,#42739,#42740,#42741,#42742,#42743,#42744),.UNSPECIFIED.,
 .F.,.F.,(4,2,2,2,2,1,4),(3.02719502833942E-5,0.00196345017130929,0.00405152224974051,
0.00791573660758486,0.0117814260340998,0.018211181166248,0.0190097167577563),
 .UNSPECIFIED.);
#1141=B_SPLINE_CURVE_WITH_KNOTS('',3,(#42746,#42747,#42748,#42749,#42750,
#42751,#42752,#42753,#42754,#42755),.UNSPECIFIED.,.F.,.F.,(4,3,3,4),(0.,
0.5,0.954472009937235,1.),.UNSPECIFIED.);
#1142=B_SPLINE_CURVE_WITH_KNOTS('',3,(#42789,#42790,#42791,#42792,#42793,
#42794,#42795,#42796,#42797,#42798,#42799,#42800,#42801),.UNSPECIFIED.,
 .F.,.F.,(4,2,2,2,2,1,4),(0.,0.00196327068521397,0.00405116683518219,0.00791556264156159,
0.0117816276323522,0.0182150743305803,0.0190236917019835),.UNSPECIFIED.);
#1143=B_SPLINE_CURVE_WITH_KNOTS('',3,(#42802,#42803,#42804,#42805,#42806,
#42807,#42808,#42809,#42810,#42811,#42812,#42813,#42814,#42815),
 .UNSPECIFIED.,.F.,.F.,(4,2,2,2,2,2,4),(0.000139162384345064,0.0024762649742147,
0.00533153906455379,0.00984378785210221,0.0137939163567501,0.0193287305983979,
0.0196872216305737),.UNSPECIFIED.);
#1144=B_SPLINE_CURVE_WITH_KNOTS('',3,(#42817,#42818,#42819,#42820),
 .UNSPECIFIED.,.F.,.F.,(4,4),(8.32473598532599E-11,0.000180393203869309),
 .UNSPECIFIED.);
#1145=B_SPLINE_CURVE_WITH_KNOTS('',3,(#42839,#42840,#42841,#42842,#42843,
#42844,#42845,#42846,#42847,#42848,#42849,#42850,#42851,#42852,#42853,#42854,
#42855,#42856),.UNSPECIFIED.,.F.,.F.,(4,2,2,2,2,2,2,2,4),(0.00769785679708774,
0.00802820462699518,0.00843145134922816,0.00899044509204644,0.0111243442863434,
0.0153131578831398,0.0188817433759505,0.0211457734297869,0.0229957599552858),
 .UNSPECIFIED.);
#1146=B_SPLINE_CURVE_WITH_KNOTS('',3,(#42875,#42876,#42877,#42878,#42879,
#42880,#42881,#42882,#42883,#42884,#42885,#42886,#42887,#42888,#42889,#42890,
#42891),.UNSPECIFIED.,.F.,.F.,(4,2,2,2,2,2,2,1,4),(-0.0060395950713934,
-0.00533643385535489,-0.00457161010811536,-0.00315658316525502,-0.00174099050172359,
-0.00017573884332551,-0.000110297877347887,-7.85738128386753E-5,-2.35863647916582E-5),
 .UNSPECIFIED.);
#1147=B_SPLINE_CURVE_WITH_KNOTS('',3,(#42893,#42894,#42895,#42896,#42897,
#42898,#42899,#42900,#42901,#42902,#42903,#42904,#42905,#42906,#42907),
 .UNSPECIFIED.,.F.,.F.,(4,2,2,2,2,2,1,4),(0.,0.00229368739167764,0.00482687780864931,
0.00907820400782217,0.0132315563727989,0.0189068992119232,0.0192249547905654,
0.0195430103692075),.UNSPECIFIED.);
#1148=B_SPLINE_CURVE_WITH_KNOTS('',3,(#42944,#42945,#42946,#42947,#42948,
#42949,#42950,#42951,#42952,#42953,#42954,#42955,#42956),.UNSPECIFIED.,
 .F.,.F.,(4,2,2,2,2,1,4),(0.,0.00196328295888409,0.00405119382129033,0.00791560040373507,
0.0117816828145636,0.0181787290681755,0.0189003258766864),.UNSPECIFIED.);
#1149=B_SPLINE_CURVE_WITH_KNOTS('',3,(#42957,#42958,#42959,#42960,#42961,
#42962,#42963,#42964,#42965,#42966,#42967,#42968,#42969,#42970,#42971,#42972,
#42973,#42974,#42975,#42976,#42977,#42978),.UNSPECIFIED.,.F.,.F.,(4,2,2,
2,2,2,2,2,2,2,4),(0.000140180528062204,0.00225584941024912,0.00477761261246817,
0.00890918499620693,0.013273463805397,0.015463798412026,0.0165317709770468,
0.0170651823497595,0.0173442289099364,0.0175722509086272,0.0178410054929824),
 .UNSPECIFIED.);
#1150=B_SPLINE_CURVE_WITH_KNOTS('',3,(#42997,#42998,#42999,#43000,#43001,
#43002,#43003,#43004,#43005,#43006,#43007,#43008,#43009,#43010),
 .UNSPECIFIED.,.F.,.F.,(4,2,2,2,2,2,4),(0.,0.00207941973197339,0.00431488716400025,
0.00832511413568298,0.0124961317069963,0.0167503250398471,0.0180491597892712),
 .UNSPECIFIED.);
#1151=B_SPLINE_CURVE_WITH_KNOTS('',3,(#43029,#43030,#43031,#43032,#43033,
#43034,#43035,#43036,#43037,#43038,#43039,#43040,#43041,#43042,#43043,#43044,
#43045,#43046,#43047,#43048,#43049,#43050),.UNSPECIFIED.,.F.,.F.,(4,2,2,
2,2,2,2,2,2,2,4),(-0.00520512896532105,-0.0047254121597404,-0.00384306945129063,
-0.0026259626535781,-0.00135029183013414,-0.000702398299474361,-0.000385625313690802,
-0.000227584692409082,-0.000144536400628624,-7.66530613735417E-5,0.),
 .UNSPECIFIED.);
#1152=B_SPLINE_CURVE_WITH_KNOTS('',3,(#43069,#43070,#43071,#43072,#43073,
#43074,#43075,#43076,#43077,#43078,#43079,#43080,#43081,#43082),
 .UNSPECIFIED.,.F.,.F.,(4,2,2,2,2,2,4),(-0.0149861184273252,-0.0130782901080037,
-0.0110008733235856,-0.00715736810866992,-0.0033122548327467,-5.78553775021709E-7,
0.000656745899211298),.UNSPECIFIED.);
#1153=B_SPLINE_CURVE_WITH_KNOTS('',3,(#43101,#43102,#43103,#43104,#43105,
#43106,#43107,#43108,#43109,#43110,#43111,#43112,#43113,#43114),
 .UNSPECIFIED.,.F.,.F.,(4,2,2,2,2,2,4),(-0.0155094238033158,-0.0134904514688655,
-0.0113307135610571,-0.00736843882793857,-0.00334201943138028,0.,0.000700784549264495),
 .UNSPECIFIED.);
#1154=B_SPLINE_CURVE_WITH_KNOTS('',3,(#43151,#43152,#43153,#43154,#43155,
#43156,#43157),.UNSPECIFIED.,.F.,.F.,(4,3,4),(4.63335483447215E-5,0.576904555942714,
1.),.UNSPECIFIED.);
#1155=B_SPLINE_CURVE_WITH_KNOTS('',3,(#43158,#43159,#43160,#43161,#43162,
#43163,#43164,#43165,#43166,#43167,#43168,#43169,#43170,#43171),
 .UNSPECIFIED.,.F.,.F.,(4,2,2,2,2,2,4),(0.00011713384202571,0.00225864572668593,
0.00478192661937105,0.00891724353890262,0.0128312590854899,0.0167147431913389,
0.017525068949556),.UNSPECIFIED.);
#1156=B_SPLINE_CURVE_WITH_KNOTS('',3,(#43190,#43191,#43192,#43193,#43194,
#43195,#43196,#43197,#43198,#43199,#43200,#43201,#43202,#43203),
 .UNSPECIFIED.,.F.,.F.,(4,2,2,2,2,2,4),(0.,0.00213082043024386,0.00443313724537573,
0.00848007384794817,0.012794220088842,0.0161393809355339,0.0168933269801154),
 .UNSPECIFIED.);
#1157=B_SPLINE_CURVE_WITH_KNOTS('',3,(#43205,#43206,#43207,#43208,#43209,
#43210,#43211,#43212,#43213,#43214,#43215,#43216,#43217,#43218,#43219,#43220,
#43221,#43222,#43223,#43224,#43225,#43226,#43227,#43228,#43229,#43230,#43231,
#43232),.UNSPECIFIED.,.F.,.F.,(4,2,2,2,2,2,2,2,2,2,2,2,2,4),(0.000174134990213334,
0.00187427244956009,0.00396421279048467,0.00796453993799608,0.0131627439566036,
0.0171335149626361,0.0189518130231438,0.0193835279188768,0.0196250377516676,
0.0196751501926279,0.0196996611938061,0.0197117721364523,0.0199235080293271,
0.0203275207337434),.UNSPECIFIED.);
#1158=B_SPLINE_CURVE_WITH_KNOTS('',3,(#43248,#43249,#43250,#43251,#43252,
#43253,#43254,#43255,#43256,#43257,#43258,#43259,#43260,#43261,#43262),
 .UNSPECIFIED.,.F.,.F.,(4,2,2,2,2,2,1,4),(-0.0088943782310824,-0.00781596641048315,
-0.0066515240749629,-0.00449643047488731,-0.00234060802490015,-7.76918320130951E-7,
0.000287494473515859,0.000575765865351848),.UNSPECIFIED.);
#1159=B_SPLINE_CURVE_WITH_KNOTS('',3,(#43278,#43279,#43280,#43281,#43282,
#43283,#43284,#43285,#43286,#43287,#43288,#43289,#43290,#43291),
 .UNSPECIFIED.,.F.,.F.,(4,2,2,2,2,2,4),(-0.0158043920350505,-0.0137354422361253,
-0.0115133073678156,-0.00749815840910723,-0.00334302701322283,-6.298460010698E-7,
0.000722872722575174),.UNSPECIFIED.);
#1160=B_SPLINE_CURVE_WITH_KNOTS('',3,(#43322,#43323,#43324,#43325,#43326,
#43327,#43328,#43329,#43330,#43331,#43332,#43333,#43334,#43335,#43336),
 .UNSPECIFIED.,.F.,.F.,(4,2,2,2,2,2,1,4),(0.,0.0019632699431003,0.00405114150044124,
0.00791493916943235,0.0117801488263792,0.0162003287979513,0.0168797194475004,
0.0175591100970496),.UNSPECIFIED.);
#1161=B_SPLINE_CURVE_WITH_KNOTS('',3,(#43337,#43338,#43339,#43340,#43341,
#43342,#43343,#43344,#43345,#43346,#43347,#43348,#43349),.UNSPECIFIED.,
 .F.,.F.,(4,3,3,3,4),(0.00643398620750897,0.459308200273434,0.500000335643866,
0.949872720004008,0.99999999998043),.UNSPECIFIED.);
#1162=B_SPLINE_CURVE_WITH_KNOTS('',3,(#43351,#43352,#43353,#43354,#43355,
#43356,#43357,#43358,#43359,#43360),.UNSPECIFIED.,.F.,.F.,(4,3,3,4),(0.,
0.451687166473715,0.5,1.),.UNSPECIFIED.);
#1163=B_SPLINE_CURVE_WITH_KNOTS('',3,(#43376,#43377,#43378,#43379,#43380,
#43381,#43382,#43383,#43384,#43385,#43386,#43387,#43388),.UNSPECIFIED.,
 .F.,.F.,(4,3,3,3,4),(6.243301773739E-9,0.452960189921173,0.5,0.953477189168755,
0.993525782404942),.UNSPECIFIED.);
#1164=B_SPLINE_CURVE_WITH_KNOTS('',3,(#43404,#43405,#43406,#43407,#43408,
#43409,#43410,#43411,#43412,#43413,#43414,#43415,#43416,#43417,#43418),
 .UNSPECIFIED.,.F.,.F.,(4,2,2,2,2,2,1,4),(2.13732516168125E-5,0.00196337715740596,
0.00405135866965422,0.00791551885237747,0.0117810712401529,0.0159267936047945,
0.0164430910383506,0.0169593884719067),.UNSPECIFIED.);
#1165=B_SPLINE_CURVE_WITH_KNOTS('',3,(#43420,#43421,#43422,#43423,#43424,
#43425,#43426,#43427,#43428,#43429),.UNSPECIFIED.,.F.,.F.,(4,3,3,4),(4.26803766547994E-9,
0.5,0.948505579092606,1.),.UNSPECIFIED.);
#1166=B_SPLINE_CURVE_WITH_KNOTS('',3,(#43460,#43461,#43462,#43463,#43464,
#43465,#43466,#43467,#43468,#43469,#43470,#43471,#43472,#43473,#43474,#43475),
 .UNSPECIFIED.,.F.,.F.,(4,2,2,2,2,2,2,4),(0.000728504471755486,0.000939141210919874,
0.00177033038102613,0.00320263890334485,0.00692959899102407,0.0107850896424002,
0.0140478837404244,0.0170344679497315),.UNSPECIFIED.);
#1167=B_SPLINE_CURVE_WITH_KNOTS('',3,(#43476,#43477,#43478,#43479,#43480,
#43481,#43482,#43483,#43484,#43485,#43486,#43487,#43488,#43489),
 .UNSPECIFIED.,.F.,.F.,(4,2,2,2,2,2,4),(0.00010160769219427,0.00122102113075305,
0.0025441425093596,0.00564882016696292,0.0110992314938815,0.018557172207377,
0.01940107775831),.UNSPECIFIED.);
#1168=B_SPLINE_CURVE_WITH_KNOTS('',3,(#43505,#43506,#43507,#43508,#43509,
#43510,#43511),.UNSPECIFIED.,.F.,.F.,(4,3,4),(0.,0.649593716766449,0.999996170084436),
 .UNSPECIFIED.);
#1169=B_SPLINE_CURVE_WITH_KNOTS('',3,(#43513,#43514,#43515,#43516,#43517,
#43518,#43519),.UNSPECIFIED.,.F.,.F.,(4,3,4),(0.00152959430806593,0.750813994531579,
0.999868145301564),.UNSPECIFIED.);
#1170=B_SPLINE_CURVE_WITH_KNOTS('',3,(#43521,#43522,#43523,#43524,#43525,
#43526,#43527,#43528,#43529,#43530,#43531,#43532,#43533,#43534,#43535,#43536,
#43537,#43538,#43539,#43540,#43541,#43542,#43543,#43544),.UNSPECIFIED.,
 .F.,.F.,(4,2,2,2,2,2,2,2,2,2,2,4),(0.00204715033410867,0.00214131685417548,
0.00214328334720006,0.00214525441504065,0.00218111916521674,0.00226943891369271,
0.00246440256884611,0.0064636073563424,0.010547188883976,0.0137087254753622,
0.0153157764781132,0.0166006569605146),.UNSPECIFIED.);
#1171=B_SPLINE_CURVE_WITH_KNOTS('',3,(#43546,#43547,#43548,#43549),
 .UNSPECIFIED.,.F.,.F.,(4,4),(6.83292023692837E-9,0.99943821988792),
 .UNSPECIFIED.);
#1172=B_SPLINE_CURVE_WITH_KNOTS('',3,(#43580,#43581,#43582,#43583,#43584,
#43585,#43586,#43587,#43588,#43589,#43590,#43591,#43592,#43593,#43594),
 .UNSPECIFIED.,.F.,.F.,(4,1,2,2,2,2,2,4),(-0.000721085007192466,-0.000360542503596233,
0.,0.00287183524996394,0.00517719429213056,0.00771610262833221,0.009312961775071,
0.0107491030887171),.UNSPECIFIED.);
#1173=B_SPLINE_CURVE_WITH_KNOTS('',3,(#43595,#43596,#43597,#43598,#43599,
#43600,#43601,#43602,#43603,#43604),.UNSPECIFIED.,.F.,.F.,(4,2,2,2,4),(-0.00965817669299273,
-0.0074786447771315,-0.00464773278744681,-0.00179228406875512,0.),
 .UNSPECIFIED.);
#1174=B_SPLINE_CURVE_WITH_KNOTS('',3,(#43606,#43607,#43608,#43609,#43610,
#43611,#43612,#43613,#43614,#43615,#43616,#43617,#43618,#43619,#43620,#43621),
 .UNSPECIFIED.,.F.,.F.,(4,2,2,2,2,2,2,4),(0.0109402855774774,0.0121575085049054,
0.0143534546456024,0.0170434917438361,0.0211697549569896,0.0237315274442865,
0.0248381170476492,0.0251943850241165),.UNSPECIFIED.);
#1175=B_SPLINE_CURVE_WITH_KNOTS('',3,(#43623,#43624,#43625,#43626,#43627,
#43628,#43629,#43630,#43631,#43632,#43633,#43634,#43635,#43636,#43637),
 .UNSPECIFIED.,.F.,.F.,(4,2,2,2,2,2,1,4),(0.000110756842378222,0.00245081867056697,
0.00524680256100879,0.00963989788679471,0.0136782996277394,0.0195995990701057,
0.0204950744567913,0.0213905498434769),.UNSPECIFIED.);
#1176=B_SPLINE_CURVE_WITH_KNOTS('',3,(#43639,#43640,#43641,#43642,#43643,
#43644,#43645,#43646,#43647,#43648,#43649,#43650,#43651,#43652,#43653),
 .UNSPECIFIED.,.F.,.F.,(4,2,2,2,2,2,1,4),(-0.012412672104359,-0.0108466451671881,
-0.00897946215730165,-0.00600237082743812,-0.00331077857606189,-4.09349858813621E-7,
0.000415773934254383,0.000831957218367579),.UNSPECIFIED.);
#1177=B_SPLINE_CURVE_WITH_KNOTS('',3,(#43669,#43670,#43671,#43672,#43673,
#43674,#43675,#43676,#43677,#43678,#43679,#43680,#43681,#43682),
 .UNSPECIFIED.,.F.,.F.,(4,2,2,2,2,2,4),(-0.015078381833914,-0.0131186091331513,
-0.0110344068594359,-0.00717766413762145,-0.00331927009469946,-7.58587308438002E-7,
0.000663174204454999),.UNSPECIFIED.);
#1178=B_SPLINE_CURVE_WITH_KNOTS('',3,(#43713,#43714,#43715,#43716,#43717,
#43718,#43719,#43720,#43721,#43722,#43723,#43724,#43725,#43726,#43727),
 .UNSPECIFIED.,.F.,.F.,(4,1,2,2,2,2,2,4),(-0.000734317183253655,-0.000367158591626828,
0.,0.00295316648201105,0.00537349468880681,0.00803885665043543,0.00971523565928993,
0.0112229190958255),.UNSPECIFIED.);
#1179=B_SPLINE_CURVE_WITH_KNOTS('',3,(#43728,#43729,#43730,#43731,#43732,
#43733,#43734,#43735,#43736,#43737,#43738,#43739,#43740,#43741),
 .UNSPECIFIED.,.F.,.F.,(4,2,2,2,2,2,4),(-0.0126319361261658,-0.0110411624711013,
-0.00932775041915123,-0.00615718988741039,-0.00298521368956833,0.,0.000652693410532094),
 .UNSPECIFIED.);
#1180=B_SPLINE_CURVE_WITH_KNOTS('',3,(#43757,#43758,#43759,#43760,#43761,
#43762,#43763,#43764,#43765,#43766,#43767,#43768,#43769,#43770),
 .UNSPECIFIED.,.F.,.F.,(4,2,2,2,2,2,4),(0.,0.0022508673695075,0.0047447068702816,
0.00880824860212537,0.012793275955846,0.0188290600607819,0.0220919733094374),
 .UNSPECIFIED.);
#1181=B_SPLINE_CURVE_WITH_KNOTS('',3,(#43772,#43773,#43774,#43775,#43776,
#43777,#43778,#43779,#43780,#43781,#43782,#43783,#43784,#43785,#43786),
 .UNSPECIFIED.,.F.,.F.,(4,2,2,2,2,2,1,4),(0.000109583238215975,0.00245093435459509,
0.00524713881000084,0.00964068384981554,0.0136193432454163,0.0194845949868915,
0.0206313249998054,0.0217780550127193),.UNSPECIFIED.);
#1182=B_SPLINE_CURVE_WITH_KNOTS('',3,(#43788,#43789,#43790,#43791,#43792,
#43793,#43794,#43795,#43796,#43797,#43798,#43799,#43800,#43801,#43802),
 .UNSPECIFIED.,.F.,.F.,(4,2,2,2,2,2,1,4),(-0.0125380391583743,-0.0109543469897537,
-0.00906695797544928,-0.00605748119240737,-0.00333652356516311,-3.59896165919374E-7,
0.000420640062250262,0.000841640020666443),.UNSPECIFIED.);
#1183=B_SPLINE_CURVE_WITH_KNOTS('',3,(#43818,#43819,#43820,#43821,#43822,
#43823,#43824,#43825,#43826,#43827,#43828,#43829,#43830,#43831),
 .UNSPECIFIED.,.F.,.F.,(4,2,2,2,2,2,4),(-0.0150733797038266,-0.0131143211030396,
-0.011030859344339,-0.00717556933822455,-0.00331852841954188,-7.25644891112764E-7,
0.000662487949083671),.UNSPECIFIED.);
#1184=B_SPLINE_CURVE_WITH_KNOTS('',3,(#43862,#43863,#43864,#43865,#43866,
#43867,#43868,#43869,#43870,#43871,#43872,#43873,#43874,#43875,#43876),
 .UNSPECIFIED.,.F.,.F.,(4,1,2,2,2,2,2,4),(-0.000741878016633449,-0.000370939008316724,
0.,0.00297259893383558,0.0054147943408359,0.00810416070365053,0.00979566612229234,
0.0113169507490356),.UNSPECIFIED.);
#1185=B_SPLINE_CURVE_WITH_KNOTS('',3,(#43877,#43878,#43879,#43880,#43881,
#43882,#43883,#43884,#43885,#43886,#43887,#43888,#43889,#43890),
 .UNSPECIFIED.,.F.,.F.,(4,2,2,2,2,2,4),(-0.0122871688845248,-0.0107438701097029,
-0.00908257557294534,-0.00600856433681326,-0.00293310884332506,0.,0.000649631234003708),
 .UNSPECIFIED.);
#1186=B_SPLINE_CURVE_WITH_KNOTS('',3,(#43906,#43907,#43908,#43909,#43910,
#43911,#43912,#43913,#43914,#43915,#43916,#43917,#43918,#43919),
 .UNSPECIFIED.,.F.,.F.,(4,2,2,2,2,2,4),(0.,0.00225039966924556,0.00474368416702002,
0.00880685738624697,0.0127791302606063,0.0166740141105481,0.0172515126691911),
 .UNSPECIFIED.);
#1187=B_SPLINE_CURVE_WITH_KNOTS('',3,(#43921,#43922,#43923,#43924,#43925,
#43926,#43927,#43928,#43929,#43930,#43931,#43932,#43933,#43934),
 .UNSPECIFIED.,.F.,.F.,(4,2,2,2,2,2,4),(0.000108721996107286,0.0024509596667275,
0.00524721540031518,0.00964094075402568,0.0135914837293887,0.017507436081882,
0.0180994566480111),.UNSPECIFIED.);
#1188=B_SPLINE_CURVE_WITH_KNOTS('',3,(#43936,#43937,#43938,#43939,#43940,
#43941,#43942,#43943,#43944,#43945,#43946,#43947,#43948,#43949,#43950),
 .UNSPECIFIED.,.F.,.F.,(4,2,2,2,2,2,1,4),(-0.0149129193286548,-0.0129965664222115,
-0.0107134808259071,-0.00707293891052898,-0.00378143624454696,-3.24086999198975E-7,
0.000422829226243187,0.000845982539485573),.UNSPECIFIED.);
#1189=B_SPLINE_CURVE_WITH_KNOTS('',3,(#43966,#43967,#43968,#43969,#43970,
#43971,#43972,#43973,#43974,#43975,#43976,#43977,#43978,#43979),
 .UNSPECIFIED.,.F.,.F.,(4,2,2,2,2,2,4),(-0.0150676149456439,-0.0131093839672474,
-0.0110267844150414,-0.00717316249718917,-0.003317694134226,-6.91760243556189E-7,
0.000661693396741128),.UNSPECIFIED.);
#1190=B_SPLINE_CURVE_WITH_KNOTS('',3,(#44010,#44011,#44012,#44013,#44014,
#44015,#44016,#44017,#44018,#44019,#44020,#44021,#44022,#44023,#44024),
 .UNSPECIFIED.,.F.,.F.,(4,1,2,2,2,2,2,4),(-0.000740226615683101,-0.00037011330784155,
0.,0.00296825453891254,0.00540526633452328,0.008088977356173,0.00977702223183042,
0.0112951461282497),.UNSPECIFIED.);
#1191=B_SPLINE_CURVE_WITH_KNOTS('',3,(#44025,#44026,#44027,#44028,#44029,
#44030,#44031,#44032,#44033,#44034,#44035,#44036,#44037,#44038),
 .UNSPECIFIED.,.F.,.F.,(4,2,2,2,2,2,4),(-0.011254734338536,-0.00985313094765622,
-0.00834524071717542,-0.00555519590875847,-0.0027637664637976,0.,0.000645994893972402),
 .UNSPECIFIED.);
#1192=B_SPLINE_CURVE_WITH_KNOTS('',3,(#44054,#44055,#44056,#44057,#44058,
#44059,#44060,#44061,#44062,#44063,#44064,#44065,#44066,#44067),
 .UNSPECIFIED.,.F.,.F.,(4,2,2,2,2,2,4),(0.,0.00224971467737683,0.00474217676161104,
0.008804821918669,0.0127594425323947,0.018558425141178,0.0211568201917662),
 .UNSPECIFIED.);
#1193=B_SPLINE_CURVE_WITH_KNOTS('',3,(#44069,#44070,#44071,#44072,#44073,
#44074,#44075,#44076,#44077,#44078,#44079,#44080,#44081,#44082),
 .UNSPECIFIED.,.F.,.F.,(4,2,2,2,2,2,4),(0.000107838954687328,0.00245083687006141,
0.00524686551857072,0.00964032925791452,0.0136011718567849,0.0196371711489655,
0.0229339743667445),.UNSPECIFIED.);
#1194=B_SPLINE_CURVE_WITH_KNOTS('',3,(#44084,#44085,#44086,#44087,#44088,
#44089,#44090,#44091,#44092,#44093,#44094,#44095,#44096,#44097,#44098),
 .UNSPECIFIED.,.F.,.F.,(4,2,2,2,2,2,1,4),(-0.014939291320971,-0.0130188828362878,
-0.0107316995046581,-0.00708448598111002,-0.00378695827246614,-2.83689470114909E-7,
0.000425980206607165,0.000852244102684445),.UNSPECIFIED.);
#1195=B_SPLINE_CURVE_WITH_KNOTS('',3,(#44114,#44115,#44116,#44117,#44118,
#44119,#44120,#44121,#44122,#44123,#44124,#44125,#44126,#44127),
 .UNSPECIFIED.,.F.,.F.,(4,2,2,2,2,2,4),(-0.0150614059516756,-0.0131040689956594,
-0.0110224033904192,-0.00717057369300718,-0.00331680728711196,-6.58184886700303E-7,
0.000660833663601821),.UNSPECIFIED.);
#1196=B_SPLINE_CURVE_WITH_KNOTS('',3,(#44158,#44159,#44160,#44161,#44162,
#44163,#44164,#44165,#44166,#44167,#44168,#44169,#44170,#44171,#44172),
 .UNSPECIFIED.,.F.,.F.,(4,1,2,2,2,2,2,4),(-0.000691739067306629,-0.000345856578478131,
2.59103503667726E-8,0.0027975315775318,0.00501871624556568,0.00746569969276276,
0.00900487309295416,0.0103889571762724),.UNSPECIFIED.);
#1197=B_SPLINE_CURVE_WITH_KNOTS('',3,(#44173,#44174,#44175,#44176,#44177,
#44178,#44179,#44180,#44181,#44182,#44183,#44184,#44185),.UNSPECIFIED.,
 .F.,.F.,(4,2,2,2,2,1,4),(3.16211434698517E-5,0.00196343737821928,0.00405149290676457,
0.00791568419994298,0.0117813340088185,0.0182067510991605,0.0189937367781405),
 .UNSPECIFIED.);
#1198=B_SPLINE_CURVE_WITH_KNOTS('',3,(#44201,#44202,#44203,#44204,#44205,
#44206,#44207,#44208,#44209,#44210,#44211,#44212,#44213,#44214,#44215),
 .UNSPECIFIED.,.F.,.F.,(4,2,2,2,2,2,1,4),(0.,0.00225539508390829,0.0047551224758348,
0.00882290010525813,0.012929760761633,0.0189658855667421,0.0197228197031485,
0.0204797538395548),.UNSPECIFIED.);
#1199=B_SPLINE_CURVE_WITH_KNOTS('',3,(#44217,#44218,#44219,#44220,#44221,
#44222,#44223,#44224,#44225,#44226,#44227,#44228,#44229,#44230,#44231),
 .UNSPECIFIED.,.F.,.F.,(4,2,2,2,2,2,1,4),(0.000114847568641728,0.00244997042572085,
0.00524435790927852,0.00963463871755652,0.0137272589487558,0.01978697300403,
0.0205522261776815,0.021317479351333),.UNSPECIFIED.);
#1200=B_SPLINE_CURVE_WITH_KNOTS('',3,(#44233,#44234,#44235,#44236,#44237,
#44238,#44239,#44240,#44241,#44242,#44243,#44244,#44245,#44246,#44247),
 .UNSPECIFIED.,.F.,.F.,(4,2,2,2,2,2,1,4),(-0.0118947324656203,-0.0104010198964424,
-0.00861751596243538,-0.00577422353032262,-0.00320311792038097,-6.29187275549489E-7,
0.000394523774615498,0.000789676736506546),.UNSPECIFIED.);
#1201=B_SPLINE_CURVE_WITH_KNOTS('',3,(#44263,#44264,#44265,#44266,#44267,
#44268,#44269,#44270,#44271,#44272,#44273,#44274,#44275),.UNSPECIFIED.,
 .F.,.F.,(4,2,2,2,2,1,4),(0.,0.0019634605910373,0.00405154255300626,0.00791565857793337,
0.0117812104822195,0.0156720023551305,0.0157373790506278),.UNSPECIFIED.);
#1202=B_SPLINE_CURVE_WITH_KNOTS('',3,(#44306,#44307,#44308,#44309,#44310,
#44311,#44312,#44313,#44314,#44315,#44316,#44317,#44318,#44319,#44320),
 .UNSPECIFIED.,.F.,.F.,(4,1,2,2,2,2,2,4),(-0.000763541080028175,-0.000381770540014087,
0.,0.0030327047674076,0.00554422819304898,0.00830974549903936,0.0100492407392823,
0.0116136695759151),.UNSPECIFIED.);
#1203=B_SPLINE_CURVE_WITH_KNOTS('',3,(#44321,#44322,#44323,#44324,#44325,
#44326,#44327,#44328,#44329,#44330,#44331,#44332,#44333,#44334,#44335),
 .UNSPECIFIED.,.F.,.F.,(4,2,2,2,2,2,1,4),(-0.0133315230507839,-0.011640861096409,
-0.009824081620331,-0.00646273446012228,-0.0030995729707021,0.,0.000318751292783897,
0.000637502585567794),.UNSPECIFIED.);
#1204=B_SPLINE_CURVE_WITH_KNOTS('',3,(#44351,#44352,#44353,#44354,#44355,
#44356,#44357,#44358,#44359,#44360,#44361,#44362,#44363,#44364,#44365),
 .UNSPECIFIED.,.F.,.F.,(4,2,2,2,2,2,1,4),(0.,0.0022461630475493,0.00473421914177116,
0.0087940687030795,0.0126718295068081,0.01772896307951,0.0182910875229529,
0.0188532119663958),.UNSPECIFIED.);
#1205=B_SPLINE_CURVE_WITH_KNOTS('',3,(#44367,#44368,#44369,#44370,#44371,
#44372,#44373,#44374,#44375,#44376,#44377,#44378,#44379,#44380,#44381),
 .UNSPECIFIED.,.F.,.F.,(4,2,2,2,2,2,1,4),(0.000106100181661028,0.00245103004290281,
0.00524743088659168,0.00964166827403447,0.0135194054565417,0.0188461184288979,
0.0191995608126034,0.019553003196309),.UNSPECIFIED.);
#1206=B_SPLINE_CURVE_WITH_KNOTS('',3,(#44383,#44384,#44385,#44386,#44387,
#44388,#44389,#44390,#44391,#44392,#44393,#44394,#44395,#44396,#44397),
 .UNSPECIFIED.,.F.,.F.,(4,2,2,2,2,2,1,4),(-0.0150589537599889,-0.0131215304824762,
-0.010815435264458,-0.00713770971273073,-0.00381261252897884,-1.7897945260581E-7,
0.000439962560525125,0.000880104100502855),.UNSPECIFIED.);
#1207=B_SPLINE_CURVE_WITH_KNOTS('',3,(#44413,#44414,#44415,#44416,#44417,
#44418,#44419,#44420,#44421,#44422,#44423,#44424,#44425,#44426),
 .UNSPECIFIED.,.F.,.F.,(4,2,2,2,2,2,4),(-0.0150490520073303,-0.0130934976202166,
-0.011013693455221,-0.00716543230475343,-0.0033150490758814,-5.96494445290544E-7,
0.000659105180738562),.UNSPECIFIED.);
#1208=B_SPLINE_CURVE_WITH_KNOTS('',3,(#44460,#44461,#44462,#44463,#44464,
#44465,#44466,#44467,#44468,#44469),.UNSPECIFIED.,.F.,.F.,(4,3,3,4),(4.76676660675416E-11,
0.458512147724096,0.5,0.99999948372105),.UNSPECIFIED.);
#1209=B_SPLINE_CURVE_WITH_KNOTS('',3,(#44470,#44471,#44472,#44473,#44474,
#44475,#44476,#44477,#44478,#44479,#44480,#44481,#44482,#44483,#44484,#44485,
#44486),.UNSPECIFIED.,.F.,.F.,(4,2,2,2,2,2,2,1,4),(4.25743825136903E-5,
0.00196427209076551,0.00405327225761388,0.00791819907389034,0.0117846711271358,
0.0158752614297264,0.0160346040583549,0.016109286249132,0.0162294355263165),
 .UNSPECIFIED.);
#1210=B_SPLINE_CURVE_WITH_KNOTS('',3,(#44505,#44506,#44507,#44508,#44509,
#44510,#44511,#44512,#44513,#44514,#44515,#44516,#44517,#44518,#44519),
 .UNSPECIFIED.,.F.,.F.,(4,2,2,2,2,2,1,4),(0.,0.00229420957926068,0.00482817002974407,
0.00908036440822177,0.0133874783015933,0.0196108582088963,0.0205947571667744,
0.0215786561246526),.UNSPECIFIED.);
#1211=B_SPLINE_CURVE_WITH_KNOTS('',3,(#44521,#44522,#44523,#44524,#44525,
#44526,#44527,#44528,#44529,#44530,#44531,#44532,#44533,#44534,#44535),
 .UNSPECIFIED.,.F.,.F.,(4,2,2,2,2,2,1,4),(0.000136707832181995,0.00249232514602642,
0.00536880437866845,0.00990130746918292,0.0138102490017995,0.0191471415464468,
0.0195724563892528,0.0199977712320588),.UNSPECIFIED.);
#1212=B_SPLINE_CURVE_WITH_KNOTS('',3,(#44537,#44538,#44539,#44540,#44541,
#44542,#44543,#44544,#44545,#44546,#44547,#44548,#44549,#44550,#44551,#44552,
#44553,#44554,#44555,#44556,#44557,#44558,#44559,#44560,#44561,#44562,#44563,
#44564),.UNSPECIFIED.,.F.,.F.,(4,2,2,2,2,2,2,2,2,2,2,2,2,4),(0.00898954517258166,
0.00914281246490069,0.00915480318218891,0.00916394223308905,0.009170539070818,
0.00917512298254225,0.00934376075639942,0.00993773086056826,0.0107255979885816,
0.0140390495835903,0.0203898888919342,0.0258014279076157,0.0292347438173574,
0.0320432823289119),.UNSPECIFIED.);
#1213=B_SPLINE_CURVE_WITH_KNOTS('',3,(#44583,#44584,#44585,#44586,#44587,
#44588,#44589,#44590,#44591,#44592,#44593,#44594,#44595),.UNSPECIFIED.,
 .F.,.F.,(4,2,2,2,2,1,4),(0.,0.00196326831438807,0.00405116172141169,0.00791555685180518,
0.0117816204128086,0.0182121807887324,0.0190127006546827),.UNSPECIFIED.);
#1214=B_SPLINE_CURVE_WITH_KNOTS('',3,(#44629,#44630,#44631,#44632,#44633,
#44634,#44635,#44636,#44637,#44638,#44639,#44640,#44641,#44642,#44643),
 .UNSPECIFIED.,.F.,.F.,(4,1,2,2,2,2,2,4),(-0.000734686664483305,-0.000367343332241652,
0.,0.00295428728510061,0.005375468594744,0.00804183895503185,0.00971909263264639,
0.0112274500128319),.UNSPECIFIED.);
#1215=B_SPLINE_CURVE_WITH_KNOTS('',3,(#44644,#44645,#44646,#44647,#44648,
#44649,#44650,#44651,#44652,#44653,#44654,#44655,#44656,#44657),
 .UNSPECIFIED.,.F.,.F.,(4,2,2,2,2,2,4),(-0.0111679813135756,-0.00977782326874345,
-0.00828321187638799,-0.0055178304310841,-0.00275101805988158,0.,0.000641924036864499),
 .UNSPECIFIED.);
#1216=B_SPLINE_CURVE_WITH_KNOTS('',3,(#44673,#44674,#44675,#44676,#44677,
#44678,#44679,#44680,#44681,#44682,#44683,#44684,#44685,#44686),
 .UNSPECIFIED.,.F.,.F.,(4,2,2,2,2,2,4),(0.,0.00224862323800864,0.00473974267430908,
0.00880152583573068,0.0127307468244572,0.0182732791623988,0.0204025687641099),
 .UNSPECIFIED.);
#1217=B_SPLINE_CURVE_WITH_KNOTS('',3,(#44688,#44689,#44690,#44691,#44692,
#44693,#44694,#44695,#44696,#44697,#44698,#44699,#44700,#44701,#44702),
 .UNSPECIFIED.,.F.,.F.,(4,2,2,2,2,2,1,4),(0.000107182900594769,0.0024506374855744,
0.00524629582418313,0.00963926824962338,0.0136265182058118,0.0194869643633496,
0.0205771760420138,0.021667387720678),.UNSPECIFIED.);
#1218=B_SPLINE_CURVE_WITH_KNOTS('',3,(#44704,#44705,#44706,#44707,#44708,
#44709,#44710,#44711,#44712,#44713,#44714,#44715,#44716,#44717,#44718),
 .UNSPECIFIED.,.F.,.F.,(4,2,2,2,2,2,1,4),(-0.0149775721862555,-0.0130517244210142,
-0.0107585030750918,-0.00710150465772868,-0.00379514746711448,-2.39497760071844E-7,
0.000430503915153775,0.000861247328067622),.UNSPECIFIED.);
#1219=B_SPLINE_CURVE_WITH_KNOTS('',3,(#44734,#44735,#44736,#44737,#44738,
#44739,#44740,#44741,#44742,#44743,#44744,#44745,#44746,#44747),
 .UNSPECIFIED.,.F.,.F.,(4,2,2,2,2,2,4),(-0.0150554445787514,-0.0130989671617,
-0.0110181991831687,-0.00716809080361883,-0.00331595685734504,-6.27284798819516E-7,
0.000660002856751512),.UNSPECIFIED.);
#1220=B_SPLINE_CURVE_WITH_KNOTS('',3,(#44778,#44779,#44780,#44781,#44782,
#44783,#44784,#44785,#44786,#44787,#44788,#44789,#44790,#44791,#44792),
 .UNSPECIFIED.,.F.,.F.,(4,1,2,2,2,2,2,4),(-0.000705657006003329,-0.000352824269207572,
8.46758818422687E-9,0.00283187350914316,0.00509218516814216,0.00758124097390481,
0.00914657677669795,0.0105544503558209),.UNSPECIFIED.);
#1221=B_SPLINE_CURVE_WITH_KNOTS('',3,(#44793,#44794,#44795,#44796),
 .UNSPECIFIED.,.F.,.F.,(4,4),(2.52662111139725E-7,0.000156519894285502),
 .UNSPECIFIED.);
#1222=B_SPLINE_CURVE_WITH_KNOTS('',3,(#44842,#44843,#44844,#44845,#44846,
#44847,#44848),.UNSPECIFIED.,.F.,.F.,(4,3,4),(0.,8.0731985910313E-5,0.000184468015134139),
 .UNSPECIFIED.);
#1223=B_SPLINE_CURVE_WITH_KNOTS('',3,(#44850,#44851,#44852,#44853,#44854,
#44855,#44856,#44857,#44858,#44859,#44860,#44861,#44862,#44863,#44864),
 .UNSPECIFIED.,.F.,.F.,(4,2,2,2,2,2,1,4),(0.000111698808826464,0.00245119018910623,
0.00524786599351128,0.00964187816046448,0.0136789300227376,0.0195975813525889,
0.0204982843709798,0.0213989873893708),.UNSPECIFIED.);
#1224=B_SPLINE_CURVE_WITH_KNOTS('',3,(#44866,#44867,#44868,#44869,#44870,
#44871,#44872,#44873,#44874,#44875,#44876,#44877,#44878,#44879,#44880),
 .UNSPECIFIED.,.F.,.F.,(4,2,2,2,2,2,1,4),(-0.0121689856441338,-0.0106303509242525,
-0.00879541739039853,-0.00587521095579035,-0.00324935971193159,-5.94103874715715E-7,
0.000405611248584354,0.000811816601043423),.UNSPECIFIED.);
#1225=B_SPLINE_CURVE_WITH_KNOTS('',3,(#44896,#44897,#44898,#44899,#44900,
#44901,#44902,#44903,#44904,#44905,#44906,#44907,#44908),.UNSPECIFIED.,
 .F.,.F.,(4,2,2,2,2,1,4),(-0.00734641636438769,-0.00650314695269393,-0.00560634882285633,
-0.00394680380774528,-0.00228661105698405,-4.0314916701506E-7,4.49899914394729E-5),
 .UNSPECIFIED.);
#1226=B_SPLINE_CURVE_WITH_KNOTS('',3,(#44939,#44940,#44941,#44942,#44943,
#44944,#44945,#44946,#44947,#44948,#44949,#44950,#44951,#44952,#44953),
 .UNSPECIFIED.,.F.,.F.,(4,1,2,2,2,2,2,4),(-0.000701295402296016,-0.000350641164626568,
1.30730428811931E-8,0.00282096645904851,0.00506882011954181,0.00754443484759998,
0.00910140169713002,0.0105016764816241),.UNSPECIFIED.);
#1227=B_SPLINE_CURVE_WITH_KNOTS('',3,(#44954,#44955,#44956,#44957),
 .UNSPECIFIED.,.F.,.F.,(4,4),(2.63661137154546E-7,0.000156519267932661),
 .UNSPECIFIED.);
#1228=B_SPLINE_CURVE_WITH_KNOTS('',3,(#45003,#45004,#45005,#45006,#45007,
#45008,#45009),.UNSPECIFIED.,.F.,.F.,(4,3,4),(0.,0.000143865342517527,0.000184570540086384),
 .UNSPECIFIED.);
#1229=B_SPLINE_CURVE_WITH_KNOTS('',3,(#45011,#45012,#45013,#45014,#45015,
#45016,#45017,#45018,#45019,#45020,#45021,#45022,#45023,#45024,#45025),
 .UNSPECIFIED.,.F.,.F.,(4,2,2,2,2,2,1,4),(0.000112557705947448,0.00245085244664319,
0.00524689426873268,0.0096398676966151,0.0136952476221313,0.0196544422019704,
0.0205060043367664,0.0213575664715625),.UNSPECIFIED.);
#1230=B_SPLINE_CURVE_WITH_KNOTS('',3,(#45027,#45028,#45029,#45030,#45031,
#45032,#45033,#45034,#45035,#45036,#45037,#45038,#45039,#45040,#45041),
 .UNSPECIFIED.,.F.,.F.,(4,2,2,2,2,2,1,4),(-0.011944752020003,-0.0104366177918527,
-0.00863786788440518,-0.00577558334657159,-0.00320190562003143,-6.11066602646329E-7,
0.000396248533472148,0.000793108133546943),.UNSPECIFIED.);
#1231=B_SPLINE_CURVE_WITH_KNOTS('',3,(#45057,#45058,#45059,#45060,#45061,
#45062,#45063,#45064,#45065,#45066,#45067,#45068,#45069),.UNSPECIFIED.,
 .F.,.F.,(4,2,2,2,2,1,4),(-0.00909175237345571,-0.00802830991517297,-0.00689736354987959,
-0.00480451655714594,-0.00271085651475671,-4.46707455368026E-7,5.80232275783389E-5),
 .UNSPECIFIED.);
#1232=B_SPLINE_CURVE_WITH_KNOTS('',3,(#45100,#45101,#45102,#45103,#45104,
#45105,#45106,#45107,#45108,#45109,#45110,#45111,#45112,#45113,#45114),
 .UNSPECIFIED.,.F.,.F.,(4,1,2,2,2,2,2,4),(-0.000694944197987434,-0.000347462280626568,
1.96367342977484E-8,0.00280536701289039,0.00503556246214006,0.00749203226490682,
0.00903705415467283,0.0104265061881677),.UNSPECIFIED.);
#1233=B_SPLINE_CURVE_WITH_KNOTS('',3,(#45115,#45116,#45117,#45118,#45119,
#45120,#45121,#45122,#45123,#45124,#45125,#45126,#45127),.UNSPECIFIED.,
 .F.,.F.,(4,2,2,2,2,1,4),(-0.00115302603191237,-0.00103082771804171,-0.000898911217383983,
-0.000654785644988868,-0.000410565788246101,0.,6.52261959239386E-5),
 .UNSPECIFIED.);
#1234=B_SPLINE_CURVE_WITH_KNOTS('',3,(#45143,#45144,#45145,#45146,#45147,
#45148,#45149,#45150,#45151,#45152,#45153,#45154,#45155,#45156,#45157),
 .UNSPECIFIED.,.F.,.F.,(4,2,2,2,2,2,1,4),(0.,0.00225413674326502,0.00475206800918924,
0.00881838664702737,0.0128986238151764,0.0188615545702435,0.0196792162708141,
0.0204968779713847),.UNSPECIFIED.);
#1235=B_SPLINE_CURVE_WITH_KNOTS('',3,(#45159,#45160,#45161,#45162,#45163,
#45164,#45165,#45166,#45167,#45168,#45169,#45170,#45171,#45172,#45173),
 .UNSPECIFIED.,.F.,.F.,(4,2,2,2,2,2,1,4),(0.000113387852022085,0.00245050920907356,
0.00524590629665468,0.00963782864983612,0.0137251491146221,0.0197690904467667,
0.0205469566713966,0.0213248228960264),.UNSPECIFIED.);
#1236=B_SPLINE_CURVE_WITH_KNOTS('',3,(#45175,#45176,#45177,#45178,#45179,
#45180,#45181,#45182,#45183,#45184,#45185,#45186,#45187,#45188,#45189),
 .UNSPECIFIED.,.F.,.F.,(4,2,2,2,2,2,1,4),(-0.0119786407496759,-0.0104721508238425,
-0.00867539394979939,-0.00581086664521615,-0.00322028623970441,-6.01136300057425E-7,
0.000398005967340617,0.000796613070981292),.UNSPECIFIED.);
#1237=B_SPLINE_CURVE_WITH_KNOTS('',3,(#45205,#45206,#45207,#45208,#45209,
#45210,#45211,#45212,#45213,#45214,#45215,#45216,#45217),.UNSPECIFIED.,
 .F.,.F.,(4,2,2,2,2,1,4),(-0.0156746082238113,-0.0137108816572334,-0.0116225064475064,
-0.00775789938403069,-0.00389180253681144,-3.19960164023303E-7,6.49564316540085E-5),
 .UNSPECIFIED.);
#1238=B_SPLINE_CURVE_WITH_KNOTS('',3,(#45248,#45249,#45250,#45251,#45252,
#45253,#45254,#45255,#45256,#45257,#45258,#45259,#45260,#45261,#45262),
 .UNSPECIFIED.,.F.,.F.,(4,1,2,2,2,2,2,4),(-0.000698046171675193,-0.000349014683457108,
1.68047609766433E-8,0.00281280649313789,0.00505118485493888,0.00751684215155518,
0.00906767756137545,0.0104623198843236),.UNSPECIFIED.);
#1239=B_SPLINE_CURVE_WITH_KNOTS('',3,(#45263,#45264,#45265,#45266,#45267,
#45268,#45269,#45270,#45271,#45272,#45273,#45274,#45275),.UNSPECIFIED.,
 .F.,.F.,(4,2,2,2,2,1,4),(3.0391652138187E-5,0.00196345031052539,0.00405152254689268,
0.00791573701057382,0.0117814265638152,0.0182103569252899,0.0190067212118065),
 .UNSPECIFIED.);
#1240=B_SPLINE_CURVE_WITH_KNOTS('',3,(#45291,#45292,#45293,#45294,#45295,
#45296,#45297,#45298,#45299,#45300),.UNSPECIFIED.,.F.,.F.,(4,3,3,4),(5.32625458252635E-7,
0.5,0.949950994221564,1.),.UNSPECIFIED.);
#1241=B_SPLINE_CURVE_WITH_KNOTS('',3,(#45302,#45303,#45304,#45305,#45306,
#45307,#45308,#45309,#45310,#45311,#45312,#45313,#45314,#45315,#45316),
 .UNSPECIFIED.,.F.,.F.,(4,2,2,2,2,2,1,4),(0.000114161305703342,0.00245028339395967,
0.00524525789255604,0.00963648905518044,0.0136996265586751,0.0196783118744954,
0.0205098152580543,0.0213413186416131),.UNSPECIFIED.);
#1242=B_SPLINE_CURVE_WITH_KNOTS('',3,(#45318,#45319,#45320,#45321,#45322,
#45323,#45324,#45325,#45326,#45327,#45328,#45329,#45330,#45331,#45332),
 .UNSPECIFIED.,.F.,.F.,(4,2,2,2,2,2,1,4),(-0.0112033757935951,-0.00984002274620014,
-0.00821566493097737,-0.00559369133845644,-0.00314184043085325,-6.63547733275108E-7,
0.000380127551360547,0.000760918650454369),.UNSPECIFIED.);
#1243=B_SPLINE_CURVE_WITH_KNOTS('',3,(#45348,#45349,#45350,#45351,#45352,
#45353,#45354,#45355,#45356,#45357,#45358,#45359,#45360,#45361),
 .UNSPECIFIED.,.F.,.F.,(4,2,2,2,2,2,4),(0.,0.00196294041915341,0.0040504787236346,
0.00791353350279755,0.0117780719871774,0.0183010045113864,0.0194590076073073),
 .UNSPECIFIED.);
#1244=B_SPLINE_CURVE_WITH_KNOTS('',3,(#45395,#45396,#45397,#45398,#45399,
#45400,#45401,#45402,#45403,#45404),.UNSPECIFIED.,.F.,.F.,(4,3,3,4),(6.40907306791326E-11,
0.458515632471353,0.5,0.999999486493091),.UNSPECIFIED.);
#1245=B_SPLINE_CURVE_WITH_KNOTS('',3,(#45405,#45406,#45407,#45408,#45409,
#45410,#45411,#45412,#45413,#45414,#45415,#45416,#45417,#45418,#45419,#45420,
#45421),.UNSPECIFIED.,.F.,.F.,(4,2,2,2,2,2,2,1,4),(-0.00582306471465524,
-0.00514676617698311,-0.00441095358738275,-0.00304960117926079,-0.00168770449944653,
-0.000171851700537288,-0.000107756089167128,-7.67827602927109E-5,-2.33062135913729E-5),
 .UNSPECIFIED.);
#1246=B_SPLINE_CURVE_WITH_KNOTS('',3,(#45440,#45441,#45442,#45443,#45444,
#45445,#45446,#45447,#45448,#45449,#45450,#45451,#45452,#45453,#45454),
 .UNSPECIFIED.,.F.,.F.,(4,2,2,2,2,2,1,4),(0.,0.00229369021876058,0.00482688557884032,
0.00907821922334884,0.0132316982713349,0.0189081068967721,0.0192243067083783,
0.0195405065199846),.UNSPECIFIED.);
#1247=B_SPLINE_CURVE_WITH_KNOTS('',3,(#45456,#45457,#45458,#45459,#45460,
#45461,#45462,#45463,#45464,#45465,#45466,#45467,#45468,#45469),
 .UNSPECIFIED.,.F.,.F.,(4,2,2,2,2,2,4),(0.000139385723503641,0.00249232539405233,
0.00536879945512003,0.00990126583114861,0.013826095010537,0.0193135105629825,
0.0197181924043684),.UNSPECIFIED.);
#1248=B_SPLINE_CURVE_WITH_KNOTS('',3,(#45471,#45472,#45473,#45474,#45475,
#45476,#45477),.UNSPECIFIED.,.F.,.F.,(4,3,4),(1.38512065397935E-6,0.0001113045099149,
0.000205256311026677),.UNSPECIFIED.);
#1249=B_SPLINE_CURVE_WITH_KNOTS('',3,(#45496,#45497,#45498,#45499,#45500,
#45501,#45502,#45503,#45504,#45505,#45506,#45507,#45508,#45509),
 .UNSPECIFIED.,.F.,.F.,(4,2,2,2,2,2,4),(0.,0.0019632705087533,0.00405116647296006,
0.00791556217502423,0.0117816273183626,0.0182744236276762,0.019285136254072),
 .UNSPECIFIED.);
#1250=B_SPLINE_CURVE_WITH_KNOTS('',3,(#45546,#45547,#45548,#45549,#45550,
#45551,#45552,#45553,#45554,#45555,#45556,#45557,#45558,#45559,#45560),
 .UNSPECIFIED.,.F.,.F.,(4,2,2,2,2,2,1,4),(0.,0.0020229803815632,0.00418692089039347,
0.00815726963453743,0.0121915813971656,0.0166403965411901,0.017358260390738,
0.0180761242402859),.UNSPECIFIED.);
#1251=B_SPLINE_CURVE_WITH_KNOTS('',3,(#45561,#45562,#45563,#45564,#45565,
#45566,#45567,#45568,#45569,#45570,#45571,#45572,#45573,#45574),
 .UNSPECIFIED.,.F.,.F.,(4,2,2,2,2,2,4),(4.62436974762622E-5,0.00196401966885003,
0.00405275852979369,0.00791719712913681,0.0117832769425412,0.0151123677737135,
0.0157730744381205),.UNSPECIFIED.);
#1252=B_SPLINE_CURVE_WITH_KNOTS('',3,(#45593,#45594,#45595,#45596,#45597,
#45598,#45599,#45600,#45601,#45602,#45603,#45604,#45605,#45606),
 .UNSPECIFIED.,.F.,.F.,(4,2,2,2,2,2,4),(-0.0158607099539636,-0.0137795764643132,
-0.0115422026804368,-0.00752912881153854,-0.0033549345003105,0.,0.000732369038597041),
 .UNSPECIFIED.);
#1253=B_SPLINE_CURVE_WITH_KNOTS('',3,(#45625,#45626,#45627,#45628,#45629,
#45630,#45631,#45632,#45633,#45634,#45635,#45636,#45637,#45638,#45639,#45640,
#45641,#45642,#45643,#45644,#45645,#45646),.UNSPECIFIED.,.F.,.F.,(4,2,2,
2,2,2,2,2,2,2,4),(0.000142338524652503,0.00184865257695027,0.00498757950643991,
0.00931561943583813,0.0138531791463855,0.0161575781939442,0.0172842269029924,
0.0178463672894087,0.018141812938064,0.0183816429813561,0.0186440263445286),
 .UNSPECIFIED.);
#1254=B_SPLINE_CURVE_WITH_KNOTS('',3,(#45665,#45666,#45667,#45668,#45669,
#45670,#45671,#45672,#45673,#45674,#45675,#45676,#45677,#45678,#45679,#45680,
#45681,#45682,#45683,#45684,#45685,#45686),.UNSPECIFIED.,.F.,.F.,(4,2,2,
2,2,2,2,2,2,2,4),(-0.0068296052231379,-0.00597794006538437,-0.00496179891473326,
-0.00329714673454892,-0.00111628877984325,-0.000579964236240451,-0.000316955826123173,
-0.00017927861012683,-0.000102681547137399,-5.83428845580563E-5,0.),
 .UNSPECIFIED.);
#1255=B_SPLINE_CURVE_WITH_KNOTS('',3,(#45705,#45706,#45707,#45708,#45709,
#45710,#45711,#45712,#45713,#45714,#45715,#45716,#45717),.UNSPECIFIED.,
 .F.,.F.,(4,2,2,2,2,1,4),(-0.0016025831250653,-0.0014296062846439,-0.00124564901181184,
-0.000905171694053628,-0.000564546716948114,0.,6.55513366705103E-5),
 .UNSPECIFIED.);
#1256=B_SPLINE_CURVE_WITH_KNOTS('',3,(#45751,#45752,#45753,#45754,#45755,
#45756,#45757,#45758,#45759,#45760,#45761,#45762,#45763,#45764),
 .UNSPECIFIED.,.F.,.F.,(4,2,2,2,2,2,4),(0.,0.00204631942275302,0.00424282204863565,
0.0082900825930658,0.0124353698077687,0.015775425206853,0.0164871129587233),
 .UNSPECIFIED.);
#1257=B_SPLINE_CURVE_WITH_KNOTS('',3,(#45765,#45766,#45767,#45768,#45769,
#45770,#45771,#45772,#45773,#45774,#45775,#45776,#45777,#45778,#45779),
 .UNSPECIFIED.,.F.,.F.,(4,2,2,2,2,2,1,4),(3.00484944896589E-5,0.00196306173968375,
0.00405067439867342,0.00791436594380513,0.011779298111804,0.0156048294251666,
0.0159903174909155,0.0163758055566643),.UNSPECIFIED.);
#1258=B_SPLINE_CURVE_WITH_KNOTS('',3,(#45795,#45796,#45797,#45798,#45799,
#45800,#45801,#45802,#45803,#45804,#45805,#45806,#45807,#45808),
 .UNSPECIFIED.,.F.,.F.,(4,2,2,2,2,2,4),(-0.00167205754200539,-0.0014878923674375,
-0.00128888885938142,-0.000939159922998387,-0.000566173695576969,0.,7.3929919955415E-5),
 .UNSPECIFIED.);
#1259=B_SPLINE_CURVE_WITH_KNOTS('',3,(#45824,#45825,#45826,#45827,#45828,
#45829,#45830,#45831,#45832,#45833,#45834,#45835,#45836,#45837),
 .UNSPECIFIED.,.F.,.F.,(4,2,2,2,2,2,4),(0.000118272099701553,0.00232295608069569,
0.00497082584063325,0.00927746644325167,0.0133382712947269,0.0174273312026365,
0.0182983902025005),.UNSPECIFIED.);
#1260=B_SPLINE_CURVE_WITH_KNOTS('',3,(#45853,#45854,#45855,#45856),
 .UNSPECIFIED.,.F.,.F.,(4,4),(0.00559373542229181,0.999482228601385),
 .UNSPECIFIED.);
#1261=B_SPLINE_CURVE_WITH_KNOTS('',3,(#45875,#45876,#45877,#45878,#45879,
#45880,#45881),.UNSPECIFIED.,.F.,.F.,(4,3,4),(4.6736355815065E-5,0.576883414132736,
1.),.UNSPECIFIED.);
#1262=B_SPLINE_CURVE_WITH_KNOTS('',3,(#45898,#45899,#45900,#45901,#45902,
#45903,#45904,#45905,#45906,#45907),.UNSPECIFIED.,.F.,.F.,(4,3,3,4),(0.,
0.451687035355523,0.5,0.999999498615503),.UNSPECIFIED.);
#1263=B_SPLINE_CURVE_WITH_KNOTS('',3,(#45908,#45909,#45910,#45911,#45912,
#45913,#45914,#45915,#45916,#45917,#45918,#45919,#45920,#45921,#45922),
 .UNSPECIFIED.,.F.,.F.,(4,2,2,2,2,2,1,4),(2.1727933380804E-5,0.0019633771796468,
0.00405135872367098,0.00791551897190362,0.0117810714665637,0.0159268438952171,
0.0164431479993082,0.0169594521033993),.UNSPECIFIED.);
#1264=B_SPLINE_CURVE_WITH_KNOTS('',3,(#45938,#45939,#45940,#45941,#45942,
#45943,#45944,#45945,#45946,#45947),.UNSPECIFIED.,.F.,.F.,(4,3,3,4),(5.51904757954955E-7,
0.5,0.948505736358945,1.),.UNSPECIFIED.);
#1265=B_SPLINE_CURVE_WITH_KNOTS('',3,(#45949,#45950,#45951,#45952,#45953,
#45954,#45955,#45956,#45957,#45958,#45959,#45960,#45961),.UNSPECIFIED.,
 .F.,.F.,(4,3,3,3,4),(0.00644697767278411,0.459320221896434,0.5,0.949871368012603,
0.999999999972781),.UNSPECIFIED.);
#1266=B_SPLINE_CURVE_WITH_KNOTS('',3,(#45963,#45964,#45965,#45966,#45967,
#45968,#45969,#45970,#45971,#45972,#45973,#45974,#45975),.UNSPECIFIED.,
 .F.,.F.,(4,3,3,3,4),(6.24353372205677E-9,0.452961086122329,0.5,0.953477723055937,
0.993513142879381),.UNSPECIFIED.);
#1267=B_SPLINE_CURVE_WITH_KNOTS('',3,(#45991,#45992,#45993,#45994,#45995,
#45996,#45997,#45998,#45999,#46000,#46001,#46002,#46003,#46004,#46005),
 .UNSPECIFIED.,.F.,.F.,(4,2,2,2,2,2,1,4),(0.,0.00196334098438198,0.00405128809761397,
0.00791522560527698,0.0117805752183942,0.0153693852933397,0.0157369807117346,
0.0161045761301295),.UNSPECIFIED.);
#1268=B_SPLINE_CURVE_WITH_KNOTS('',3,(#46036,#46037,#46038,#46039,#46040,
#46041,#46042,#46043,#46044,#46045,#46046,#46047,#46048,#46049,#46050,#46051),
 .UNSPECIFIED.,.F.,.F.,(4,2,2,2,2,2,2,4),(0.000722180881357717,0.000952514205597523,
0.00178841244962457,0.00322807978575928,0.0069807773394597,0.0108844917476973,
0.0141878961748357,0.0172120373492915),.UNSPECIFIED.);
#1269=B_SPLINE_CURVE_WITH_KNOTS('',3,(#46052,#46053,#46054,#46055,#46056,
#46057,#46058,#46059,#46060,#46061,#46062,#46063,#46064,#46065),
 .UNSPECIFIED.,.F.,.F.,(4,2,2,2,2,2,4),(0.000101808612729993,0.00122101813875672,
0.00254413922241313,0.00564882750579106,0.0110994395641791,0.0185573990395054,
0.0194013094863756),.UNSPECIFIED.);
#1270=B_SPLINE_CURVE_WITH_KNOTS('',3,(#46081,#46082,#46083,#46084,#46085,
#46086,#46087),.UNSPECIFIED.,.F.,.F.,(4,3,4),(0.,0.64959466758675,0.99999619133487),
 .UNSPECIFIED.);
#1271=B_SPLINE_CURVE_WITH_KNOTS('',3,(#46089,#46090,#46091,#46092),
 .UNSPECIFIED.,.F.,.F.,(4,4),(0.,0.999938556780183),.UNSPECIFIED.);
#1272=B_SPLINE_CURVE_WITH_KNOTS('',3,(#46094,#46095,#46096,#46097,#46098,
#46099,#46100,#46101,#46102,#46103,#46104,#46105,#46106,#46107,#46108,#46109,
#46110,#46111,#46112,#46113,#46114,#46115),.UNSPECIFIED.,.F.,.F.,(4,2,2,
2,2,2,2,2,2,2,4),(0.0020350607393473,0.00212844484945634,0.00213147934112845,
0.0021671948648844,0.00225515824413027,0.0024494424110281,0.00643252326101599,
0.0104961302197796,0.0136428306082811,0.0152424631856715,0.01652133042803),
 .UNSPECIFIED.);
#1273=B_SPLINE_CURVE_WITH_KNOTS('',3,(#46117,#46118,#46119,#46120,#46121,
#46122,#46123),.UNSPECIFIED.,.F.,.F.,(4,3,4),(0.000310842092326198,0.644205206716935,
1.),.UNSPECIFIED.);
#1274=B_SPLINE_CURVE_WITH_KNOTS('',3,(#46140,#46141,#46142,#46143,#46144,
#46145,#46146),.UNSPECIFIED.,.F.,.F.,(4,3,4),(0.00202397953287585,0.684966626555327,
0.999983023180911),.UNSPECIFIED.);
#1275=B_SPLINE_CURVE_WITH_KNOTS('',3,(#46147,#46148,#46149,#46150,#46151,
#46152,#46153),.UNSPECIFIED.,.F.,.F.,(4,3,4),(2.09197363928788E-6,0.658100868662447,
0.999283474902518),.UNSPECIFIED.);
#1276=B_SPLINE_CURVE_WITH_KNOTS('',3,(#46155,#46156,#46157,#46158,#46159,
#46160,#46161,#46162,#46163,#46164),.UNSPECIFIED.,.F.,.F.,(4,3,3,4),(5.72594025237121E-7,
0.5,0.959255595777748,0.99999999765769),.UNSPECIFIED.);
#1277=B_SPLINE_CURVE_WITH_KNOTS('',3,(#46166,#46167,#46168,#46169,#46170,
#46171,#46172),.UNSPECIFIED.,.F.,.F.,(4,3,4),(0.,0.666190232468981,0.999999997883627),
 .UNSPECIFIED.);
#1278=B_SPLINE_CURVE_WITH_KNOTS('',3,(#46174,#46175,#46176,#46177,#46178,
#46179,#46180,#46181,#46182,#46183,#46184,#46185,#46186),.UNSPECIFIED.,
 .F.,.F.,(4,3,3,3,4),(4.22191385656518E-7,0.451253718316959,0.5,0.949460142126203,
0.999999851640557),.UNSPECIFIED.);
#1279=B_SPLINE_CURVE_WITH_KNOTS('',3,(#46199,#46200,#46201,#46202,#46203,
#46204,#46205,#46206,#46207,#46208,#46209,#46210,#46211,#46212,#46213,#46214),
 .UNSPECIFIED.,.F.,.F.,(4,2,2,2,2,2,2,4),(0.,0.00196384398390232,0.00405236912385508,
0.00791685933181361,0.0117828564538374,0.017303424189852,0.0182095740570904,
0.0188188355030872),.UNSPECIFIED.);
#1280=B_SPLINE_CURVE_WITH_KNOTS('',3,(#46216,#46217,#46218,#46219,#46220,
#46221,#46222,#46223,#46224,#46225,#46226,#46227,#46228),.UNSPECIFIED.,
 .F.,.F.,(4,3,3,3,4),(9.26612717775814E-7,0.443369457603659,0.5,0.94042683514852,
1.),.UNSPECIFIED.);
#1281=B_SPLINE_CURVE_WITH_KNOTS('',3,(#46244,#46245,#46246,#46247,#46248,
#46249,#46250),.UNSPECIFIED.,.F.,.F.,(4,3,4),(2.84623535879637E-8,0.585567534871793,
1.),.UNSPECIFIED.);
#1282=B_SPLINE_CURVE_WITH_KNOTS('',3,(#46252,#46253,#46254,#46255,#46256,
#46257,#46258,#46259,#46260,#46261),.UNSPECIFIED.,.F.,.F.,(4,3,3,4),(1.61060839561296E-7,
0.432923028701991,0.5,1.),.UNSPECIFIED.);
#1283=B_SPLINE_CURVE_WITH_KNOTS('',3,(#46263,#46264,#46265,#46266,#46267,
#46268,#46269),.UNSPECIFIED.,.F.,.F.,(4,3,4),(9.06643405643E-7,0.651743429231903,
0.999981902721839),.UNSPECIFIED.);
#1284=B_SPLINE_CURVE_WITH_KNOTS('',3,(#46288,#46289,#46290,#46291),
 .UNSPECIFIED.,.F.,.F.,(4,4),(2.36129832897646E-7,0.000200843834661843),
 .UNSPECIFIED.);
#1285=B_SPLINE_CURVE_WITH_KNOTS('',3,(#46293,#46294,#46295,#46296),
 .UNSPECIFIED.,.F.,.F.,(4,4),(7.44913368333112E-6,0.999999690593774),
 .UNSPECIFIED.);
#1286=B_SPLINE_CURVE_WITH_KNOTS('',3,(#46357,#46358,#46359,#46360,#46361,
#46362,#46363,#46364,#46365,#46366,#46367,#46368,#46369,#46370,#46371),
 .UNSPECIFIED.,.F.,.F.,(4,2,2,2,2,2,1,4),(-0.00778271397382138,-0.00683466317105913,
-0.00582123844929078,-0.00396333406938175,-0.00207855114507763,0.,0.000250637049053843,
0.000501274098107686),.UNSPECIFIED.);
#1287=B_SPLINE_CURVE_WITH_KNOTS('',3,(#46373,#46374,#46375,#46376,#46377,
#46378,#46379,#46380,#46381,#46382,#46383,#46384,#46385,#46386,#46387,#46388,
#46389,#46390,#46391,#46392,#46393,#46394),.UNSPECIFIED.,.F.,.F.,(4,2,2,
2,2,2,2,2,2,2,4),(-0.00014392415925499,0.,0.000143447984501406,0.000221109744414235,
0.00037269299334882,0.00066348171332673,0.00123679142420446,0.00338009045823901,
0.00507124205404184,0.00641905230452008,0.00701747059813978),
 .UNSPECIFIED.);
#1288=B_SPLINE_CURVE_WITH_KNOTS('',3,(#46452,#46453,#46454,#46455),
 .UNSPECIFIED.,.F.,.F.,(4,4),(2.37150890517029E-7,0.000201167851821411),
 .UNSPECIFIED.);
#1289=B_SPLINE_CURVE_WITH_KNOTS('',3,(#46457,#46458,#46459,#46460,#46461,
#46462,#46463,#46464,#46465,#46466,#46467,#46468,#46469,#46470),
 .UNSPECIFIED.,.F.,.F.,(4,2,2,2,2,2,4),(0.0135158126676436,0.014973489136333,
0.0171160883848495,0.0201226995874232,0.0244078688421797,0.0257108161548246,
0.026156838373642),.UNSPECIFIED.);
#1290=B_SPLINE_CURVE_WITH_KNOTS('',3,(#46489,#46490,#46491,#46492,#46493,
#46494,#46495,#46496,#46497,#46498),.UNSPECIFIED.,.F.,.F.,(4,3,3,4),(3.54217342568251E-7,
0.5,0.932995637830957,1.),.UNSPECIFIED.);
#1291=B_SPLINE_CURVE_WITH_KNOTS('',3,(#46500,#46501,#46502,#46503,#46504,
#46505,#46506,#46507,#46508,#46509,#46510,#46511,#46512,#46513,#46514),
 .UNSPECIFIED.,.F.,.F.,(4,2,2,2,2,2,1,4),(0.0113718137346511,0.0125803262387957,
0.0142088530539494,0.0166548137430588,0.0214923420820296,0.02224678217811,
0.0224951901254519,0.0226872803324734),.UNSPECIFIED.);
#1292=B_SPLINE_CURVE_WITH_KNOTS('',3,(#46516,#46517,#46518,#46519,#46520,
#46521,#46522,#46523,#46524,#46525,#46526,#46527,#46528,#46529,#46530,#46531),
 .UNSPECIFIED.,.F.,.F.,(4,2,2,2,2,2,2,4),(0.0340922557365839,0.0343333033692608,
0.0346628514377239,0.0356154235520354,0.038017654942319,0.0396060348908877,
0.0406978337520487,0.0414157425803844),.UNSPECIFIED.);
#1293=B_SPLINE_CURVE_WITH_KNOTS('',3,(#46533,#46534,#46535,#46536,#46537,
#46538,#46539,#46540,#46541,#46542,#46543,#46544,#46545,#46546,#46547),
 .UNSPECIFIED.,.F.,.F.,(4,2,2,2,2,2,1,4),(0.,0.00222424191990565,0.00465511287046728,
0.00879447482255024,0.0133938157884664,0.0178039143331782,0.0182880999169529,
0.0187722855007277),.UNSPECIFIED.);
#1294=B_SPLINE_CURVE_WITH_KNOTS('',3,(#46549,#46550,#46551,#46552,#46553,
#46554,#46555,#46556,#46557,#46558,#46559,#46560,#46561,#46562),
 .UNSPECIFIED.,.F.,.F.,(4,2,2,2,2,2,4),(0.0156003477411163,0.0172855752039469,
0.0197606565720376,0.023234278347158,0.0281861916552709,0.029684187273598,
0.0301983776561063),.UNSPECIFIED.);
#1295=B_SPLINE_CURVE_WITH_KNOTS('',3,(#46584,#46585,#46586,#46587,#46588,
#46589,#46590,#46591,#46592,#46593,#46594,#46595,#46596,#46597),
 .UNSPECIFIED.,.F.,.F.,(4,2,2,2,2,2,4),(-0.0205682128831986,-0.017816287435113,
-0.0146537481341808,-0.00960273674078747,-0.00481443689872726,0.,0.00102941491059151),
 .UNSPECIFIED.);
#1296=B_SPLINE_CURVE_WITH_KNOTS('',3,(#46599,#46600,#46601,#46602,#46603,
#46604,#46605,#46606,#46607,#46608,#46609,#46610,#46611,#46612,#46613,#46614,
#46615,#46616,#46617,#46618,#46619,#46620),.UNSPECIFIED.,.F.,.F.,(4,2,2,
2,2,2,2,2,2,2,4),(-0.000143830183900261,0.,0.000143597679787919,0.000221235739118977,
0.000372775263706832,0.000663460743001667,0.0012365400442185,0.00337954254859572,
0.00507043814008076,0.00641801410969039,0.00701649344940931),
 .UNSPECIFIED.);
#1297=B_SPLINE_CURVE_WITH_KNOTS('',3,(#46684,#46685,#46686,#46687,#46688,
#46689,#46690,#46691,#46692,#46693,#46694,#46695,#46696,#46697),
 .UNSPECIFIED.,.F.,.F.,(4,2,2,2,2,2,4),(2.99246733186488E-6,0.00201249960757762,
0.0041632863175498,0.00810591663337533,0.0121030557146972,0.0158488156731948,
0.016732647820978),.UNSPECIFIED.);
#1298=B_SPLINE_CURVE_WITH_KNOTS('',3,(#46699,#46700,#46701,#46702,#46703,
#46704,#46705),.UNSPECIFIED.,.F.,.F.,(4,3,4),(5.48439606298742E-7,0.5,0.999997140301748),
 .UNSPECIFIED.);
#1299=B_SPLINE_CURVE_WITH_KNOTS('',3,(#46763,#46764,#46765,#46766),
 .UNSPECIFIED.,.F.,.F.,(4,4),(2.30992785970066E-7,0.000202736252405272),
 .UNSPECIFIED.);
#1300=B_SPLINE_CURVE_WITH_KNOTS('',3,(#46768,#46769,#46770,#46771,#46772,
#46773,#46774),.UNSPECIFIED.,.F.,.F.,(4,3,4),(0.,0.546479382302658,1.),
 .UNSPECIFIED.);
#1301=B_SPLINE_CURVE_WITH_KNOTS('',3,(#46793,#46794,#46795,#46796,#46797,
#46798,#46799,#46800,#46801,#46802,#46803,#46804,#46805,#46806,#46807,#46808,
#46809,#46810,#46811,#46812,#46813,#46814,#46815,#46816,#46817,#46818,#46819,
#46820,#46821,#46822,#46823,#46824,#46825,#46826,#46827,#46828,#46829),
 .UNSPECIFIED.,.F.,.F.,(4,1,2,2,2,2,2,2,2,2,2,2,2,2,2,2,2,2,4),(0.0059034039032535,
0.00649662725925484,0.00656341819149157,0.00658448987750684,0.00660487226112149,
0.00663152428214414,0.00665679213150518,0.00670867157264048,0.00728399544932138,
0.00780646930469712,0.00856811246381833,0.00980419850919031,0.0121806465476813,
0.0191679676383439,0.041410165517959,0.0802961750511084,0.115456796415773,
0.136085623600931,0.154936455995216),.UNSPECIFIED.);
#1302=B_SPLINE_CURVE_WITH_KNOTS('',3,(#46831,#46832,#46833,#46834,#46835,
#46836,#46837),.UNSPECIFIED.,.F.,.F.,(4,3,4),(2.86657951474293E-8,0.591763262396974,
1.),.UNSPECIFIED.);
#1303=B_SPLINE_CURVE_WITH_KNOTS('',3,(#46839,#46840,#46841,#46842,#46843,
#46844,#46845,#46846,#46847,#46848),.UNSPECIFIED.,.F.,.F.,(4,3,3,4),(5.87574713772567E-7,
0.500000293787357,0.930259890397214,0.999999731521238),.UNSPECIFIED.);
#1304=B_SPLINE_CURVE_WITH_KNOTS('',3,(#46864,#46865,#46866,#46867,#46868,
#46869,#46870,#46871,#46872,#46873,#46874,#46875,#46876,#46877,#46878,#46879),
 .UNSPECIFIED.,.F.,.F.,(4,2,2,2,2,2,2,4),(-0.00390306697050034,-0.00352231899423164,
-0.00311739545282296,-0.00236817122813141,-0.00161861983209088,-0.000555049807796949,
-0.000416527677959817,-0.000252358784354016),.UNSPECIFIED.);
#1305=B_SPLINE_CURVE_WITH_KNOTS('',3,(#46881,#46882,#46883,#46884,#46885,
#46886,#46887,#46888,#46889,#46890,#46891,#46892,#46893),.UNSPECIFIED.,
 .F.,.F.,(4,3,3,3,4),(0.,0.451351771143798,0.499999612007475,0.952090754403713,
0.999999223904282),.UNSPECIFIED.);
#1306=B_SPLINE_CURVE_WITH_KNOTS('',3,(#46906,#46907,#46908,#46909,#46910,
#46911,#46912),.UNSPECIFIED.,.F.,.F.,(4,3,4),(0.,0.663177241834219,0.999999999703733),
 .UNSPECIFIED.);
#1307=B_SPLINE_CURVE_WITH_KNOTS('',3,(#46914,#46915,#46916,#46917,#46918,
#46919,#46920,#46921,#46922,#46923),.UNSPECIFIED.,.F.,.F.,(4,3,3,4),(4.05016758157343E-7,
0.5,0.95857558711876,0.999999999242644),.UNSPECIFIED.);
#1308=B_SPLINE_CURVE_WITH_KNOTS('',3,(#46925,#46926,#46927,#46928,#46929,
#46930,#46931),.UNSPECIFIED.,.F.,.F.,(4,3,4),(1.19975828902745E-5,0.575510273364395,
0.99815504015047),.UNSPECIFIED.);
#1309=B_SPLINE_CURVE_WITH_KNOTS('',3,(#46933,#46934,#46935,#46936,#46937,
#46938,#46939),.UNSPECIFIED.,.F.,.F.,(4,3,4),(0.000609342180978295,0.5,
0.99999969898345),.UNSPECIFIED.);
#1310=B_SPLINE_CURVE_WITH_KNOTS('',3,(#46992,#46993,#46994,#46995,#46996,
#46997,#46998),.UNSPECIFIED.,.F.,.F.,(4,3,4),(1.62696442369048E-8,0.000133938713825017,
0.000161353569749288),.UNSPECIFIED.);
#1311=B_SPLINE_CURVE_WITH_KNOTS('',3,(#46999,#47000,#47001,#47002,#47003,
#47004,#47005,#47006,#47007,#47008,#47009,#47010,#47011,#47012,#47013,#47014,
#47015,#47016,#47017,#47018,#47019,#47020),.UNSPECIFIED.,.F.,.F.,(4,2,2,
2,2,2,2,2,2,2,4),(-0.0121117789361161,-0.0105531999363958,-0.00882659923363592,
-0.00598279969381208,-0.00275319141802341,-0.00142567726470279,-0.000757158957527394,
-0.000425414570489878,-0.000260434122667489,-0.000159073980362508,-2.05838487038443E-5),
 .UNSPECIFIED.);
#1312=B_SPLINE_CURVE_WITH_KNOTS('',3,(#47069,#47070,#47071,#47072,#47073,
#47074,#47075),.UNSPECIFIED.,.F.,.F.,(4,3,4),(1.65353367717499E-8,0.000133977101550613,
0.000161445935848968),.UNSPECIFIED.);
#1313=B_SPLINE_CURVE_WITH_KNOTS('',3,(#47127,#47128,#47129,#47130,#47131,
#47132,#47133,#47134,#47135,#47136,#47137,#47138,#47139,#47140,#47141,#47142,
#47143,#47144,#47145,#47146,#47147),.UNSPECIFIED.,.F.,.F.,(4,2,2,2,2,2,
2,2,2,1,4),(0.,0.00222984288937753,0.00469946423214668,0.00876653081177419,
0.0133799493316473,0.0153650476469126,0.0163343894682131,0.0168305855295093,
0.0171007793566801,0.0172993328283054,0.01748691231476),.UNSPECIFIED.);
#1532=(
BOUNDED_SURFACE()
B_SPLINE_SURFACE(2,2,((#35087,#35088,#35089),(#35090,#35091,#35092),(#35093,
#35094,#35095)),.UNSPECIFIED.,.F.,.F.,.F.)
B_SPLINE_SURFACE_WITH_KNOTS((3,3),(3,3),(-2.00840310324026,-1.7944713619242),
(-0.411288011040583,0.054890026555908),.UNSPECIFIED.)
GEOMETRIC_REPRESENTATION_ITEM()
RATIONAL_B_SPLINE_SURFACE(((1.,0.972957523892801,1.),(0.994284603862378,
0.967396686218674,0.994284603862378),(1.,0.972957523892801,1.)))
REPRESENTATION_ITEM('')
SURFACE()
);
#1533=(
BOUNDED_SURFACE()
B_SPLINE_SURFACE(3,2,((#36527,#36528,#36529),(#36530,#36531,#36532),(#36533,
#36534,#36535),(#36536,#36537,#36538),(#36539,#36540,#36541),(#36542,#36543,
#36544),(#36545,#36546,#36547),(#36548,#36549,#36550),(#36551,#36552,#36553),
(#36554,#36555,#36556),(#36557,#36558,#36559),(#36560,#36561,#36562),(#36563,
#36564,#36565)),.UNSPECIFIED.,.F.,.F.,.F.)
B_SPLINE_SURFACE_WITH_KNOTS((4,1,1,1,1,1,1,1,1,1,4),(3,3),(-9.12136692509678E-5,
0.00220796830307519,0.0044159366061504,0.005519920757688,0.00662390490922561,
0.00883187321230082,0.011039841515376,0.0121438256669136,0.0132478098184512,
0.0154557781215264,0.0177549600938526),(0.,1.00009121366925),
 .UNSPECIFIED.)
GEOMETRIC_REPRESENTATION_ITEM()
RATIONAL_B_SPLINE_SURFACE(((1.,0.856598302581804,1.00002616039),(1.,0.85648245509437,
1.00002618152375),(1.,0.837039368671017,1.00002972847425),(1.,0.783240704790969,
1.00003954282132),(1.,0.741022900299178,1.00004724450303),(1.,0.710759323434978,
1.00005276540681),(1.,0.713774372303659,1.00005221537947),(1.,0.710758784450604,
1.00005276550514),(1.,0.741025562278053,1.00004724401741),(1.,0.783315033613179,
1.00003952926171),(1.,0.836980639913045,1.00002973918798),(1.,0.85648437213857,
1.00002618117402),(1.,0.856596624849924,1.00002616069606)))
REPRESENTATION_ITEM('')
SURFACE()
);
#1534=(
BOUNDED_SURFACE()
B_SPLINE_SURFACE(3,2,((#36578,#36579,#36580),(#36581,#36582,#36583),(#36584,
#36585,#36586),(#36587,#36588,#36589),(#36590,#36591,#36592),(#36593,#36594,
#36595),(#36596,#36597,#36598)),.UNSPECIFIED.,.F.,.F.,.F.)
B_SPLINE_SURFACE_WITH_KNOTS((4,1,1,1,4),(3,3),(0.0220837783457775,0.0258964944248447,
0.0286667756071232,0.0314370567894017,0.0352497216550509),(-0.00765169206451642,
1.00921035252307),.UNSPECIFIED.)
GEOMETRIC_REPRESENTATION_ITEM()
RATIONAL_B_SPLINE_SURFACE(((1.01141897281319,0.246902245950543,1.01376629482688),
(1.01094701638963,0.278028453921076,1.01319732147188),(1.00923044814925,
0.391238609305028,1.01112788975729),(1.00696653098374,0.54054721705706,
1.00839859425289),(1.00514075800961,0.660959582399751,1.00619750931644),
(1.00458410278544,0.697671798635305,1.00552642619379),(1.0046514192879,
0.693232178045747,1.00560758050029)))
REPRESENTATION_ITEM('')
SURFACE()
);
#1535=(
BOUNDED_SURFACE()
B_SPLINE_SURFACE(3,2,((#36612,#36613,#36614),(#36615,#36616,#36617),(#36618,
#36619,#36620),(#36621,#36622,#36623),(#36624,#36625,#36626),(#36627,#36628,
#36629),(#36630,#36631,#36632)),.UNSPECIFIED.,.F.,.F.,.F.)
B_SPLINE_SURFACE_WITH_KNOTS((4,1,1,1,4),(3,3),(0.0225273553584918,0.0261980037033457,
0.0288843286844024,0.0315706536654592,0.0353315086389343),(0.,1.00171344488683),
 .UNSPECIFIED.)
GEOMETRIC_REPRESENTATION_ITEM()
RATIONAL_B_SPLINE_SURFACE(((1.,0.698070739631419,1.00103467829473),(1.,
0.701445296152567,1.00102311406149),(1.,0.667087022821676,1.00114085607701),
(1.,0.554485456741017,1.00152672923231),(1.,0.412396180757329,1.00201365351913),
(1.,0.303473902619339,1.0023869181602),(1.,0.264839160729741,1.00251931516209)))
REPRESENTATION_ITEM('')
SURFACE()
);
#1536=(
BOUNDED_SURFACE()
B_SPLINE_SURFACE(3,2,((#36657,#36658,#36659),(#36660,#36661,#36662),(#36663,
#36664,#36665),(#36666,#36667,#36668),(#36669,#36670,#36671),(#36672,#36673,
#36674),(#36675,#36676,#36677)),.UNSPECIFIED.,.F.,.F.,.F.)
B_SPLINE_SURFACE_WITH_KNOTS((4,1,1,1,4),(3,3),(0.0225273401345282,0.026197989064192,
0.028884314475386,0.03157063988658,0.0353314954622503),(0.,1.00171342949153),
 .UNSPECIFIED.)
GEOMETRIC_REPRESENTATION_ITEM()
RATIONAL_B_SPLINE_SURFACE(((1.,0.698070764188803,1.00103466891399),(1.,
0.701445290615732,1.00102310488779),(1.,0.667086987296867,1.00114084594816),
(1.,0.554485918057329,1.00152671393378),(1.,0.412395167858293,1.00201363889751),
(1.,0.303472815512153,1.00238690043911),(1.,0.264838377974932,1.00251929520844)))
REPRESENTATION_ITEM('')
SURFACE()
);
#1537=(
BOUNDED_SURFACE()
B_SPLINE_SURFACE(3,2,((#36679,#36680,#36681),(#36682,#36683,#36684),(#36685,
#36686,#36687),(#36688,#36689,#36690),(#36691,#36692,#36693),(#36694,#36695,
#36696),(#36697,#36698,#36699)),.UNSPECIFIED.,.F.,.F.,.F.)
B_SPLINE_SURFACE_WITH_KNOTS((4,1,1,1,4),(3,3),(0.0223953062325209,0.0261531475701134,
0.0288373199541088,0.0315214923381043,0.0352152692137),(-0.00583702121317319,
1.00094993511605),.UNSPECIFIED.)
GEOMETRIC_REPRESENTATION_ITEM()
RATIONAL_B_SPLINE_SURFACE(((1.008611578014,0.261626297741005,1.00139466579746),
(1.00816947060695,0.299533459750967,1.00132306543822),(1.00688616459349,
0.409566651199769,1.00111523093893),(1.0052192786986,0.552488739050661,
1.00084527475412),(1.003898428583,0.665741035947371,1.00063135989707),(1.00349620161079,
0.700228770730926,1.00056621827029),(1.00354053058602,0.696427916868363,
1.00057339745458)))
REPRESENTATION_ITEM('')
SURFACE()
);
#1538=(
BOUNDED_SURFACE()
B_SPLINE_SURFACE(3,2,((#36707,#36708,#36709),(#36710,#36711,#36712),(#36713,
#36714,#36715),(#36716,#36717,#36718),(#36719,#36720,#36721),(#36722,#36723,
#36724),(#36725,#36726,#36727),(#36728,#36729,#36730),(#36731,#36732,#36733),
(#36734,#36735,#36736),(#36737,#36738,#36739),(#36740,#36741,#36742),(#36743,
#36744,#36745)),.UNSPECIFIED.,.F.,.F.,.F.)
B_SPLINE_SURFACE_WITH_KNOTS((4,1,1,1,1,1,1,1,1,1,4),(3,3),(-9.11921919217132E-5,
0.00220796838434516,0.00441593676869044,0.00551992096086308,0.00662390515303572,
0.008831873537381,0.0110398419217263,0.0121438261138989,0.0132478103060716,
0.0154557786904168,0.0177549392666837),(0.,1.00009119219192),
 .UNSPECIFIED.)
GEOMETRIC_REPRESENTATION_ITEM()
RATIONAL_B_SPLINE_SURFACE(((1.,0.856596899436669,1.00002615448614),(1.,
0.85648081496737,1.00002617565813),(1.,0.837038206403486,1.00002972168632),
(1.,0.783241039910642,1.00003953344938),(1.,0.741023293792506,1.00004723330699),
(1.,0.710759112115924,1.00005275302112),(1.,0.71377437769044,1.00005220308377),
(1.,0.710759010469376,1.00005275303966),(1.,0.741025173682679,1.00004723296413),
(1.,0.783314706872162,1.00003952001367),(1.,0.836981393995776,1.00002973204801),
(1.,0.856485647362579,1.00002617477678),(1.,0.85659802774457,1.00002615428035)))
REPRESENTATION_ITEM('')
SURFACE()
);
#1539=(
BOUNDED_SURFACE()
B_SPLINE_SURFACE(3,2,((#36746,#36747,#36748),(#36749,#36750,#36751),(#36752,
#36753,#36754),(#36755,#36756,#36757),(#36758,#36759,#36760),(#36761,#36762,
#36763),(#36764,#36765,#36766),(#36767,#36768,#36769),(#36770,#36771,#36772),
(#36773,#36774,#36775),(#36776,#36777,#36778)),.UNSPECIFIED.,.F.,.F.,.F.)
B_SPLINE_SURFACE_WITH_KNOTS((4,1,1,1,1,1,1,1,4),(3,3),(0.,0.00377228174191368,
0.00754456348382736,0.011316845225741,0.0150891269676547,0.0188614087095684,
0.0226336904514821,0.0264059721933958,0.0301782539353095),(0.,1.),
 .UNSPECIFIED.)
GEOMETRIC_REPRESENTATION_ITEM()
RATIONAL_B_SPLINE_SURFACE(((1.,0.720825457499061,1.),(1.,0.746053483029738,
1.),(1.,0.792459011243824,1.),(1.,0.852569440734204,1.),(1.,0.897509773183224,
1.),(1.,0.916020285468781,1.),(1.,0.897590557115624,1.),(1.,0.852747215867504,
1.),(1.,0.792807767335747,1.),(1.,0.746067376211881,1.),(1.,0.72082545750045,
1.)))
REPRESENTATION_ITEM('')
SURFACE()
);
#1540=(
BOUNDED_SURFACE()
B_SPLINE_SURFACE(3,2,((#36809,#36810,#36811),(#36812,#36813,#36814),(#36815,
#36816,#36817),(#36818,#36819,#36820),(#36821,#36822,#36823),(#36824,#36825,
#36826),(#36827,#36828,#36829),(#36830,#36831,#36832),(#36833,#36834,#36835),
(#36836,#36837,#36838),(#36839,#36840,#36841)),.UNSPECIFIED.,.F.,.F.,.F.)
B_SPLINE_SURFACE_WITH_KNOTS((4,1,1,1,1,1,1,1,4),(3,3),(-1.73472347597681E-18,
0.00377227680972667,0.00754455361945335,0.01131683042918,0.0150891072389067,
0.0188613840486334,0.02263366085836,0.0264059376680867,0.0301782144778134),
(0.,1.),.UNSPECIFIED.)
GEOMETRIC_REPRESENTATION_ITEM()
RATIONAL_B_SPLINE_SURFACE(((1.,0.720825215852201,1.),(1.,0.746052603520604,
1.),(1.,0.792461511277909,1.),(1.,0.852568820521414,1.),(1.,0.897509277356171,
1.),(1.,0.91602054372931,1.),(1.,0.897590043072446,1.),(1.,0.852746545403375,
1.),(1.,0.7928103156905,1.),(1.,0.746066497116235,1.),(1.,0.72082521585216,
1.)))
REPRESENTATION_ITEM('')
SURFACE()
);
#1541=(
BOUNDED_SURFACE()
B_SPLINE_SURFACE(3,2,((#36849,#36850,#36851),(#36852,#36853,#36854),(#36855,
#36856,#36857),(#36858,#36859,#36860),(#36861,#36862,#36863),(#36864,#36865,
#36866),(#36867,#36868,#36869),(#36870,#36871,#36872),(#36873,#36874,#36875),
(#36876,#36877,#36878),(#36879,#36880,#36881),(#36882,#36883,#36884),(#36885,
#36886,#36887)),.UNSPECIFIED.,.F.,.F.,.F.)
B_SPLINE_SURFACE_WITH_KNOTS((4,1,1,1,1,1,1,1,1,1,4),(3,3),(-0.00176595467568201,
0.0022074433446026,0.00441488668920515,0.00551860836150642,0.0066223300338077,
0.00882977337841024,0.0110372167230128,0.0121409383953141,0.0132446600676153,
0.0154521034122179,0.0194255014325015),(0.,1.00864869369591),
 .UNSPECIFIED.)
GEOMETRIC_REPRESENTATION_ITEM()
RATIONAL_B_SPLINE_SURFACE(((1.,0.544825883657364,1.00787332302111),(1.,
0.493235442718456,1.00876570286374),(1.,0.525872619257827,1.00820116497777),
(1.,0.621115631978769,1.00655370969037),(1.,0.669445109196877,1.00571773600048),
(1.,0.70093114970011,1.00517310976046),(1.,0.697705140131851,1.0052289112977),
(1.,0.700929440745956,1.00517313932091),(1.,0.669452202490575,1.00571761330503),
(1.,0.621028362011165,1.00655521923281),(1.,0.526002484867079,1.00819891864201),
(1.,0.493141690839259,1.00876732452632),(1.,0.544954936890859,1.00787109073733)))
REPRESENTATION_ITEM('')
SURFACE()
);
#1542=(
BOUNDED_SURFACE()
B_SPLINE_SURFACE(3,2,((#36891,#36892,#36893),(#36894,#36895,#36896),(#36897,
#36898,#36899),(#36900,#36901,#36902),(#36903,#36904,#36905),(#36906,#36907,
#36908),(#36909,#36910,#36911)),.UNSPECIFIED.,.F.,.F.,.F.)
B_SPLINE_SURFACE_WITH_KNOTS((4,1,1,1,4),(3,3),(0.0261906037883101,0.0302303928825723,
0.033115956521331,0.0360015201600897,0.0400413092543519),(-0.0507184440799791,
1.00026154811442),.UNSPECIFIED.)
GEOMETRIC_REPRESENTATION_ITEM()
RATIONAL_B_SPLINE_SURFACE(((1.03014167181211,0.702771482890882,1.00014797223261),
(1.03110563607959,0.693265783553587,1.00015270454957),(1.02714115683959,
0.732359709496436,1.00013324203111),(1.01704078885099,0.831959937984839,
1.00008365705749),(1.00803324096205,0.920783813399147,1.00003943698305),
(1.00421260453237,0.958459298272233,1.00002068062122),(1.00382474942852,
0.962283956641881,1.00001877655346)))
REPRESENTATION_ITEM('')
SURFACE()
);
#1543=(
BOUNDED_SURFACE()
B_SPLINE_SURFACE(3,2,((#36929,#36930,#36931),(#36932,#36933,#36934),(#36935,
#36936,#36937),(#36938,#36939,#36940),(#36941,#36942,#36943),(#36944,#36945,
#36946),(#36947,#36948,#36949)),.UNSPECIFIED.,.F.,.F.,.F.)
B_SPLINE_SURFACE_WITH_KNOTS((4,1,1,1,4),(3,3),(-0.00115047521367835,0.00287618803419606,
0.00575237606839212,0.00862856410258818,0.0126552273504408),(-0.000568079850883721,
1.04798315002903),.UNSPECIFIED.)
GEOMETRIC_REPRESENTATION_ITEM()
RATIONAL_B_SPLINE_SURFACE(((1.0003214960984,0.703447277837381,1.02844217030743),
(1.00033176605283,0.69397412105832,1.02935073434453),(1.00028951139962,
0.732950433664678,1.02561254265631),(1.00018183730347,0.832270601096544,
1.01608681280814),(1.00008575580974,0.920897581817965,1.00758665923973),
(1.00004504507645,0.958449760014905,1.00398505531614),(1.00004061088175,
0.962539926325762,1.00359277024133)))
REPRESENTATION_ITEM('')
SURFACE()
);
#1544=(
BOUNDED_SURFACE()
B_SPLINE_SURFACE(3,2,((#36960,#36961,#36962),(#36963,#36964,#36965),(#36966,
#36967,#36968),(#36969,#36970,#36971),(#36972,#36973,#36974),(#36975,#36976,
#36977),(#36978,#36979,#36980)),.UNSPECIFIED.,.F.,.F.,.F.)
B_SPLINE_SURFACE_WITH_KNOTS((4,1,1,1,4),(3,3),(-0.00115111019723794,0.00287777549291802,
0.0057555509858653,0.00863332647881258,0.0126622121689389),(-0.000643035815390294,
1.07541381943444),.UNSPECIFIED.)
GEOMETRIC_REPRESENTATION_ITEM()
RATIONAL_B_SPLINE_SURFACE(((1.00004576857842,0.961726564359363,1.00576872230422),
(1.00005117817168,0.957202855590032,1.00645055342909),(1.00009690251692,
0.918966409424796,1.01221370053452),(1.00020563830265,0.828037386912416,
1.02591887937431),(1.0003277752714,0.725901782649337,1.04131315816077),
(1.00037553613851,0.685962319009775,1.0473329907381),(1.00036398122763,
0.695624977392983,1.04587659697569)))
REPRESENTATION_ITEM('')
SURFACE()
);
#1545=(
BOUNDED_SURFACE()
B_SPLINE_SURFACE(3,2,((#36995,#36996,#36997),(#36998,#36999,#37000),(#37001,
#37002,#37003),(#37004,#37005,#37006),(#37007,#37008,#37009),(#37010,#37011,
#37012),(#37013,#37014,#37015)),.UNSPECIFIED.,.F.,.F.,.F.)
B_SPLINE_SURFACE_WITH_KNOTS((4,1,1,1,4),(3,3),(0.0261827954531206,0.0302498424885473,
0.0331548760852807,0.036059909682014,0.0400490479324759),(-0.000287608915424847,
1.05864682838005),.UNSPECIFIED.)
GEOMETRIC_REPRESENTATION_ITEM()
RATIONAL_B_SPLINE_SURFACE(((1.00016268700008,0.700581569757827,1.03510922546522),
(1.00016800320713,0.690797319202815,1.03625650774329),(1.00014630959746,
0.730723475269262,1.03157484397877),(1.00009133985094,0.831892930759882,
1.01971190948892),(1.00004296133221,0.920931514840218,1.00927141749565),
(1.00002264108182,0.95833006218513,1.00488613623644),(1.00002066329306,
0.961970097374021,1.00445931275719)))
REPRESENTATION_ITEM('')
SURFACE()
);
#1546=(
BOUNDED_SURFACE()
B_SPLINE_SURFACE(3,2,((#37022,#37023,#37024),(#37025,#37026,#37027),(#37028,
#37029,#37030),(#37031,#37032,#37033),(#37034,#37035,#37036),(#37037,#37038,
#37039),(#37040,#37041,#37042),(#37043,#37044,#37045),(#37046,#37047,#37048),
(#37049,#37050,#37051),(#37052,#37053,#37054),(#37055,#37056,#37057),(#37058,
#37059,#37060)),.UNSPECIFIED.,.F.,.F.,.F.)
B_SPLINE_SURFACE_WITH_KNOTS((4,1,1,1,1,1,1,1,1,1,4),(3,3),(-0.00176595473644677,
0.0022074434205581,0.00441488684111636,0.00551860855139549,0.00662233026167463,
0.00882977368223289,0.0110372171027912,0.0121409388130703,0.0132446605233494,
0.0154521039439077,0.0194255021009125),(0.,1.01020005259311),
 .UNSPECIFIED.)
GEOMETRIC_REPRESENTATION_ITEM()
RATIONAL_B_SPLINE_SURFACE(((1.,0.544126551146727,1.00929986630821),(1.,
0.492459105087841,1.01035388764251),(1.,0.5251450880049,1.00968709015289),
(1.,0.620532420331288,1.00774117854),(1.,0.668936288031776,1.00675373454749),
(1.,0.700471393560587,1.00611041507764),(1.,0.697240194317183,1.00617633188209),
(1.,0.700469222078685,1.0061104593761),(1.,0.668944216768396,1.00675357280043),
(1.,0.620445949537654,1.00774294255329),(1.,0.525271753063256,1.00968450617238),
(1.,0.492359013196966,1.01035592952762),(1.,0.544254308534535,1.00929726004406)))
REPRESENTATION_ITEM('')
SURFACE()
);
#1547=(
BOUNDED_SURFACE()
B_SPLINE_SURFACE(3,2,((#37072,#37073,#37074),(#37075,#37076,#37077),(#37078,
#37079,#37080),(#37081,#37082,#37083),(#37084,#37085,#37086),(#37087,#37088,
#37089),(#37090,#37091,#37092),(#37093,#37094,#37095),(#37096,#37097,#37098),
(#37099,#37100,#37101),(#37102,#37103,#37104),(#37105,#37106,#37107)),
 .UNSPECIFIED.,.F.,.F.,.F.)
B_SPLINE_SURFACE_WITH_KNOTS((4,1,1,1,1,1,1,1,1,4),(3,3),(-0.0030542815954037,
0.00381785199425464,0.00763570398850928,0.0114535559827639,0.0152714079770186,
0.0171803339741459,0.0190892599712732,0.0229071119655278,0.0267249639597825,
0.0335970975494408),(-0.0368451854302645,1.01725950520625),
 .UNSPECIFIED.)
GEOMETRIC_REPRESENTATION_ITEM()
RATIONAL_B_SPLINE_SURFACE(((1.01871196188825,0.741534782597279,1.00859972889014),
(1.02219172652787,0.693469372382115,1.01019897501307),(1.02778619975629,
0.616193844146687,1.01277010856576),(1.03620063164043,0.499966696013097,
1.01663725159439),(1.0425598341734,0.412128089083168,1.01955984293289),
(1.04521778205111,0.375414297116216,1.02078139475567),(1.0442088809608,
0.389350080077,1.02031771938558),(1.0414873683936,0.426941880527789,1.01906695421255),
(1.03623393472764,0.4995066860085,1.01665255717928),(1.02781586355586,0.615784103016817,
1.01278374159022),(1.02216498736205,0.693838716032383,1.01018668610514),
(1.01874578590278,0.741067577110249,1.00861527388518)))
REPRESENTATION_ITEM('')
SURFACE()
);
#1548=(
BOUNDED_SURFACE()
B_SPLINE_SURFACE(3,2,((#37109,#37110,#37111),(#37112,#37113,#37114),(#37115,
#37116,#37117),(#37118,#37119,#37120),(#37121,#37122,#37123),(#37124,#37125,
#37126),(#37127,#37128,#37129),(#37130,#37131,#37132),(#37133,#37134,#37135),
(#37136,#37137,#37138),(#37139,#37140,#37141),(#37142,#37143,#37144)),
 .UNSPECIFIED.,.F.,.F.,.F.)
B_SPLINE_SURFACE_WITH_KNOTS((4,1,1,1,1,1,1,1,1,4),(3,3),(-0.00305427764783682,
0.00381784705979506,0.00763569411959017,0.0114535411793853,0.0152713882391804,
0.0171803117690779,0.0190892352989755,0.0229070823587706,0.0267249294185657,
0.0335970541261962),(-0.0368459337971598,1.01726409934155),
 .UNSPECIFIED.)
GEOMETRIC_REPRESENTATION_ITEM()
RATIONAL_B_SPLINE_SURFACE(((1.01871302304651,0.741524163778113,1.00860236370568),
(1.02219179877096,0.693473164098863,1.01020155449158),(1.0277870960048,
0.616187461632156,1.01277370874625),(1.03620133847609,0.49996474585093,
1.01664173016993),(1.04256065696545,0.4121259097498,1.01956510446546),(1.04521871380193,
0.375411186435116,1.02078701134822),(1.04420986197529,0.389346071187173,
1.02032324286376),(1.04148811400065,0.426940535853924,1.019072057209),(1.03623465494052,
0.499504558259523,1.01665704572551),(1.02781675696288,0.615777766153,1.01278734386809),
(1.02216506046242,0.693842490136804,1.0101892629097),(1.0187468466081,0.741056971847484,
1.00861791237346)))
REPRESENTATION_ITEM('')
SURFACE()
);
#1549=(
BOUNDED_SURFACE()
B_SPLINE_SURFACE(3,2,((#40991,#40992,#40993),(#40994,#40995,#40996),(#40997,
#40998,#40999),(#41000,#41001,#41002),(#41003,#41004,#41005)),
 .UNSPECIFIED.,.F.,.F.,.F.)
B_SPLINE_SURFACE_WITH_KNOTS((4,1,4),(3,3),(0.00211353105058633,0.00519232055190078,
0.00827110090347046),(-0.00516083805459814,1.00866525867518),
 .UNSPECIFIED.)
GEOMETRIC_REPRESENTATION_ITEM()
RATIONAL_B_SPLINE_SURFACE(((1.00303922812236,0.702984379259216,1.00512077981927),
(1.00303934171677,0.702973277982015,1.0051209712139),(1.00303825215374,
0.703079758057304,1.00511913541476),(1.00303914737112,0.702992270862198,
1.00512064376191),(1.00303903424133,0.703003326733027,1.00512045315011)))
REPRESENTATION_ITEM('')
SURFACE()
);
#1550=(
BOUNDED_SURFACE()
B_SPLINE_SURFACE(3,2,((#41051,#41052,#41053),(#41054,#41055,#41056),(#41057,
#41058,#41059),(#41060,#41061,#41062),(#41063,#41064,#41065)),
 .UNSPECIFIED.,.F.,.F.,.F.)
B_SPLINE_SURFACE_WITH_KNOTS((4,1,4),(3,3),(0.00221234569844904,0.00528825921434574,
0.00836416458159152),(-0.00575439008396576,1.00913990416131),
 .UNSPECIFIED.)
GEOMETRIC_REPRESENTATION_ITEM()
RATIONAL_B_SPLINE_SURFACE(((1.00339056153718,0.702685410650244,1.00540347836286),
(1.00339068855421,0.70267427266794,1.00540368078766),(1.00338968434316,
0.702762330823273,1.00540208039415),(1.00339089447563,0.70265621564664,
1.005404008961),(1.0033907691906,0.702667201751574,1.00540380929647)))
REPRESENTATION_ITEM('')
SURFACE()
);
#1551=(
BOUNDED_SURFACE()
B_SPLINE_SURFACE(3,2,((#41081,#41082,#41083),(#41084,#41085,#41086),(#41087,
#41088,#41089),(#41090,#41091,#41092),(#41093,#41094,#41095)),
 .UNSPECIFIED.,.F.,.F.,.F.)
B_SPLINE_SURFACE_WITH_KNOTS((4,1,4),(3,3),(0.00222416842683505,0.00530805677349043,
0.0083919356037823),(-0.00409731518056885,1.0410723457723),
 .UNSPECIFIED.)
GEOMETRIC_REPRESENTATION_ITEM()
RATIONAL_B_SPLINE_SURFACE(((1.0024101526089,0.693757123833212,1.02504954154737),
(1.00241039130659,0.693726794025117,1.02505202241418),(1.00240948251975,
0.693842267831515,1.02504257708129),(1.00241057855278,0.693703001832813,
1.02505396852805),(1.00241027824273,0.693741160335315,1.02505084730281)))
REPRESENTATION_ITEM('')
SURFACE()
);
#1552=(
BOUNDED_SURFACE()
B_SPLINE_SURFACE(3,2,((#41125,#41126,#41127),(#41128,#41129,#41130),(#41131,
#41132,#41133),(#41134,#41135,#41136),(#41137,#41138,#41139)),
 .UNSPECIFIED.,.F.,.F.,.F.)
B_SPLINE_SURFACE_WITH_KNOTS((4,1,4),(3,3),(0.00210886666210934,0.00518760413944781,
0.00826633150911516),(-0.00505999595092042,1.00745187552521),
 .UNSPECIFIED.)
GEOMETRIC_REPRESENTATION_ITEM()
RATIONAL_B_SPLINE_SURFACE(((1.00297954446705,0.703373335363558,1.00439842930772),
(1.00297965807745,0.70336202495157,1.00439859702038),(1.0029785791549,0.70346943640386,
1.00439700430558),(1.00297947505286,0.703380245849253,1.00439832683789),
(1.00297936120932,0.703391579470171,1.00439815878108)))
REPRESENTATION_ITEM('')
SURFACE()
);
#1553=(
BOUNDED_SURFACE()
B_SPLINE_SURFACE(3,2,((#41185,#41186,#41187),(#41188,#41189,#41190),(#41191,
#41192,#41193),(#41194,#41195,#41196),(#41197,#41198,#41199)),
 .UNSPECIFIED.,.F.,.F.,.F.)
B_SPLINE_SURFACE_WITH_KNOTS((4,1,4),(3,3),(0.00220767749077139,0.00528378315884176,
0.00835988069763376),(-0.00560693921170706,1.00691897286156),
 .UNSPECIFIED.)
GEOMETRIC_REPRESENTATION_ITEM()
RATIONAL_B_SPLINE_SURFACE(((1.00330320591931,0.703386463026645,1.00408148016421),
(1.00330333288896,0.70337506170423,1.0040816370494),(1.00330233511646,0.703464657338961,
1.00408040418994),(1.00330352567297,0.70335775053797,1.00408187525559),
(1.00330340109961,0.703368936684566,1.00408172133128)))
REPRESENTATION_ITEM('')
SURFACE()
);
#1554=(
BOUNDED_SURFACE()
B_SPLINE_SURFACE(3,2,((#41215,#41216,#41217),(#41218,#41219,#41220),(#41221,
#41222,#41223),(#41224,#41225,#41226),(#41227,#41228,#41229)),
 .UNSPECIFIED.,.F.,.F.,.F.)
B_SPLINE_SURFACE_WITH_KNOTS((4,1,4),(3,3),(0.00222837931943227,0.00530337439357363,
0.008387101212674),(-0.00371892845766894,1.04348929973661),
 .UNSPECIFIED.)
GEOMETRIC_REPRESENTATION_ITEM()
RATIONAL_B_SPLINE_SURFACE(((1.00218675766921,0.693162880560133,1.02658527365176),
(1.00218697373197,0.693132563495335,1.02658790041173),(1.00218613883333,
0.693249713144516,1.02657775022036),(1.00218713984747,0.693109254830448,
1.02658991994325),(1.00218686662003,0.693147593015035,1.02658659820979)))
REPRESENTATION_ITEM('')
SURFACE()
);
#1555=(
BOUNDED_SURFACE()
B_SPLINE_SURFACE(3,2,((#41259,#41260,#41261),(#41262,#41263,#41264),(#41265,
#41266,#41267),(#41268,#41269,#41270),(#41271,#41272,#41273)),
 .UNSPECIFIED.,.F.,.F.,.F.)
B_SPLINE_SURFACE_WITH_KNOTS((4,1,4),(3,3),(0.00213710998071491,0.00521859354582936,
0.00830006498572616),(-0.0047763098346721,1.04045393253535),
 .UNSPECIFIED.)
GEOMETRIC_REPRESENTATION_ITEM()
RATIONAL_B_SPLINE_SURFACE(((1.00281160073715,0.69370896974105,1.02465899497813),
(1.00281195203053,0.693670700434191,1.02466207597807),(1.00281066656601,
0.693810736765885,1.02465080187972),(1.00281175009521,0.693692698926688,
1.02466030491506),(1.00281146517294,0.693723737877578,1.02465780601937)))
REPRESENTATION_ITEM('')
SURFACE()
);
#1556=(
BOUNDED_SURFACE()
B_SPLINE_SURFACE(3,2,((#41274,#41275,#41276),(#41277,#41278,#41279),(#41280,
#41281,#41282),(#41283,#41284,#41285),(#41286,#41287,#41288)),
 .UNSPECIFIED.,.F.,.F.,.F.)
B_SPLINE_SURFACE_WITH_KNOTS((4,1,4),(3,3),(0.00218918062982001,0.00518293797295347,
0.00817668510764242),(-8.59234239166145E-5,1.00619494117646),
 .UNSPECIFIED.)
GEOMETRIC_REPRESENTATION_ITEM()
RATIONAL_B_SPLINE_SURFACE(((1.00005034519059,0.705219481653293,1.00365198021966),
(1.00005034650813,0.705211767201325,1.00365207579255),(1.00005032906604,
0.705313893907877,1.00365081056405),(1.00005034362165,0.705228668089402,
1.00365186641064),(1.00005034221189,0.705236922522977,1.00365176414802)))
REPRESENTATION_ITEM('')
SURFACE()
);
#1557=(
BOUNDED_SURFACE()
B_SPLINE_SURFACE(3,2,((#41333,#41334,#41335),(#41336,#41337,#41338),(#41339,
#41340,#41341),(#41342,#41343,#41344),(#41345,#41346,#41347)),
 .UNSPECIFIED.,.F.,.F.,.F.)
B_SPLINE_SURFACE_WITH_KNOTS((4,1,4),(3,3),(0.0022120171615497,0.00527933863147846,
0.00824260155135531),(-0.00590011768353364,1.00557329179908),
 .UNSPECIFIED.)
GEOMETRIC_REPRESENTATION_ITEM()
RATIONAL_B_SPLINE_SURFACE(((1.00347694896963,0.703697377703806,1.00328328282864),
(1.00347708155473,0.703686078915469,1.00328340802874),(1.0034760363704,
0.703775148631286,1.00328242106121),(1.00347723423213,0.703673067877452,
1.00328355220201),(1.00347715795409,0.703679568226981,1.00328348017266)))
REPRESENTATION_ITEM('')
SURFACE()
);
#1558=(
BOUNDED_SURFACE()
B_SPLINE_SURFACE(3,2,((#41363,#41364,#41365),(#41366,#41367,#41368),(#41369,
#41370,#41371),(#41372,#41373,#41374),(#41375,#41376,#41377)),
 .UNSPECIFIED.,.F.,.F.,.F.)
B_SPLINE_SURFACE_WITH_KNOTS((4,1,4),(3,3),(0.00222404092240201,0.00529888594152649,
0.00838256483619836),(0.,1.04068548646261),.UNSPECIFIED.)
GEOMETRIC_REPRESENTATION_ITEM()
RATIONAL_B_SPLINE_SURFACE(((1.,0.695167490611038,1.02480451786822),(1.,
0.69513692670821,1.02480700488273),(1.,0.695255211522984,1.02479737993227),
(1.,0.695114648184839,1.02480881770785),(0.999999999999999,0.695152833845352,
1.0248057105035)))
REPRESENTATION_ITEM('')
SURFACE()
);
#1559=(
BOUNDED_SURFACE()
B_SPLINE_SURFACE(3,2,((#41407,#41408,#41409),(#41410,#41411,#41412),(#41413,
#41414,#41415),(#41416,#41417,#41418),(#41419,#41420,#41421)),
 .UNSPECIFIED.,.F.,.F.,.F.)
B_SPLINE_SURFACE_WITH_KNOTS((4,1,4),(3,3),(0.00213247470912648,0.00521406655521492,
0.00829564634926749),(-0.00540439094631414,1.03776288419203),
 .UNSPECIFIED.)
GEOMETRIC_REPRESENTATION_ITEM()
RATIONAL_B_SPLINE_SURFACE(((1.00318331520391,0.694306668775563,1.0229591285056),
(1.00318371379977,0.694268391668199,1.02296200331162),(1.00318224820494,
0.694409132543476,1.02295143295397),(1.00318349318509,0.69428957726687,
1.02296041216509),(1.00318316652491,0.694320946399417,1.02295805618322)))
REPRESENTATION_ITEM('')
SURFACE()
);
#1560=(
BOUNDED_SURFACE()
B_SPLINE_SURFACE(3,2,((#41422,#41423,#41424),(#41425,#41426,#41427),(#41428,
#41429,#41430),(#41431,#41432,#41433),(#41434,#41435,#41436)),
 .UNSPECIFIED.,.F.,.F.,.F.)
B_SPLINE_SURFACE_WITH_KNOTS((4,1,4),(3,3),(0.00233261591753651,0.00517832061855419,
0.00802401515924038),(-7.72572681589754E-5,1.00514489144249),
 .UNSPECIFIED.)
GEOMETRIC_REPRESENTATION_ITEM()
RATIONAL_B_SPLINE_SURFACE(((1.00004526716879,0.705528796585439,1.00302980947609),
(1.00004526749927,0.705526646764979,1.00302983159556),(1.00004525314264,
0.70562003930361,1.00302887068123),(1.00004526513196,0.705542046570605,
1.0030296731472),(1.00004526460806,0.705545454637005,1.00302963808166)))
REPRESENTATION_ITEM('')
SURFACE()
);
#1561=(
BOUNDED_SURFACE()
B_SPLINE_SURFACE(3,2,((#41481,#41482,#41483),(#41484,#41485,#41486),(#41487,
#41488,#41489),(#41490,#41491,#41492),(#41493,#41494,#41495)),
 .UNSPECIFIED.,.F.,.F.,.F.)
B_SPLINE_SURFACE_WITH_KNOTS((4,1,4),(3,3),(0.00243689541702302,0.00527505369168907,
0.00811320384373953),(0.,1.00460943847749),.UNSPECIFIED.)
GEOMETRIC_REPRESENTATION_ITEM()
RATIONAL_B_SPLINE_SURFACE(((1.,0.705724883744445,1.00271288608767),(1.,
0.705721625583332,1.00271291612426),(1.,0.705799460846715,1.00271219857054),
(1.,0.705706915990024,1.00271305173019),(1.,0.705708813997457,1.00271303423269)))
REPRESENTATION_ITEM('')
SURFACE()
);
#1562=(
BOUNDED_SURFACE()
B_SPLINE_SURFACE(3,2,((#41511,#41512,#41513),(#41514,#41515,#41516),(#41517,
#41518,#41519),(#41520,#41521,#41522),(#41523,#41524,#41525)),
 .UNSPECIFIED.,.F.,.F.,.F.)
B_SPLINE_SURFACE_WITH_KNOTS((4,1,4),(3,3),(0.00221982944241213,0.00529456505217135,
0.008378248795424),(0.,1.0382896554605),.UNSPECIFIED.)
GEOMETRIC_REPRESENTATION_ITEM()
RATIONAL_B_SPLINE_SURFACE(((1.,0.69586844611684,1.02329018482571),(1.,0.695837517046898,
1.02329255335257),(1.,0.695957500887875,1.02328336507271),(1.,0.6958162707029,
1.02329418038295),(1.,0.6958544674275,1.0232912553041)))
REPRESENTATION_ITEM('')
SURFACE()
);
#1563=(
BOUNDED_SURFACE()
B_SPLINE_SURFACE(3,2,((#41555,#41556,#41557),(#41558,#41559,#41560),(#41561,
#41562,#41563),(#41564,#41565,#41566),(#41567,#41568,#41569)),
 .UNSPECIFIED.,.F.,.F.,.F.)
B_SPLINE_SURFACE_WITH_KNOTS((4,1,4),(3,3),(0.00212792315612553,0.00520972108197668,
0.00829150685946455),(-0.00526004879476004,1.03627119860815),
 .UNSPECIFIED.)
GEOMETRIC_REPRESENTATION_ITEM()
RATIONAL_B_SPLINE_SURFACE(((1.00309785139817,0.694793504025019,1.02202052760681),
(1.00309824020449,0.694755198050842,1.02202329136765),(1.00309680397593,
0.694896698151953,1.02201308219149),(1.00309803532104,0.694775383576623,
1.02202183498998),(1.00309771298394,0.694807140870483,1.02201954371382)))
REPRESENTATION_ITEM('')
SURFACE()
);
#1564=(
BOUNDED_SURFACE()
B_SPLINE_SURFACE(3,2,((#41570,#41571,#41572),(#41573,#41574,#41575),(#41576,
#41577,#41578),(#41579,#41580,#41581),(#41582,#41583,#41584)),
 .UNSPECIFIED.,.F.,.F.,.F.)
B_SPLINE_SURFACE_WITH_KNOTS((4,1,4),(3,3),(0.00213818526553338,0.0052157458800678,
0.00829330762307971),(-0.00554775121829963,1.01491778474661),
 .UNSPECIFIED.)
GEOMETRIC_REPRESENTATION_ITEM()
RATIONAL_B_SPLINE_SURFACE(((1.00326831063643,0.701019795764348,1.00887031106351),
(1.00326841298166,0.701010433374775,1.0088705888321),(1.00326732556116,
0.701109908987846,1.00886763753426),(1.003268229636,0.701027205563585,1.00887009122547),
(1.00326811057159,0.701038097399366,1.00886976808042)))
REPRESENTATION_ITEM('')
SURFACE()
);
#1565=(
BOUNDED_SURFACE()
B_SPLINE_SURFACE(3,2,((#41629,#41630,#41631),(#41632,#41633,#41634),(#41635,
#41636,#41637),(#41638,#41639,#41640),(#41641,#41642,#41643)),
 .UNSPECIFIED.,.F.,.F.,.F.)
B_SPLINE_SURFACE_WITH_KNOTS((4,1,4),(3,3),(0.002137775280116,0.00521728249168771,
0.00829679082832463),(-0.015531588982551,1.00678065132455),
 .UNSPECIFIED.)
GEOMETRIC_REPRESENTATION_ITEM()
RATIONAL_B_SPLINE_SURFACE(((1.00924086261519,0.70046593417571,1.00399953462119),
(1.00924114133672,0.700456899673426,1.00399965525456),(1.00923811504382,
0.700554994175509,1.00399834544575),(1.0092406084373,0.700474173118263,
1.00399942461054),(1.00924030377847,0.700484048354195,1.00399929275125)))
REPRESENTATION_ITEM('')
SURFACE()
);
#1566=(
BOUNDED_SURFACE()
B_SPLINE_SURFACE(3,2,((#41659,#41660,#41661),(#41662,#41663,#41664),(#41665,
#41666,#41667),(#41668,#41669,#41670),(#41671,#41672,#41673)),
 .UNSPECIFIED.,.F.,.F.,.F.)
B_SPLINE_SURFACE_WITH_KNOTS((4,1,4),(3,3),(0.00216604370290396,0.00524889691178157,
0.00833175256952228),(-0.044566622087351,1.00513202347875),
 .UNSPECIFIED.)
GEOMETRIC_REPRESENTATION_ITEM()
RATIONAL_B_SPLINE_SURFACE(((1.02727300006651,0.69238259352349,1.00302203016815),
(1.02727633149881,0.692345017658627,1.00302239931305),(1.02726460789245,
0.69247725046666,1.00302110025933),(1.02727436205614,0.692367231380822,
1.00302218108567),(1.02727180366488,0.692396087967221,1.00302189759887)))
REPRESENTATION_ITEM('')
SURFACE()
);
#1567=(
BOUNDED_SURFACE()
B_SPLINE_SURFACE(3,2,((#41703,#41704,#41705),(#41706,#41707,#41708),(#41709,
#41710,#41711),(#41712,#41713,#41714),(#41715,#41716,#41717)),
 .UNSPECIFIED.,.F.,.F.,.F.)
B_SPLINE_SURFACE_WITH_KNOTS((4,1,4),(3,3),(0.00216543696354447,0.00524970208791062,
0.00833396653031472),(-0.00587539799910988,1.04292218799995),
 .UNSPECIFIED.)
GEOMETRIC_REPRESENTATION_ITEM()
RATIONAL_B_SPLINE_SURFACE(((1.00346232181416,0.692633563902817,1.02622525467492),
(1.00346274197103,0.692596264619502,1.02622843714083),(1.00346127232254,
0.692726732162592,1.02621730533155),(1.00346250014727,0.692617732441765,
1.02622660545382),(1.00346217135636,0.692646920741768,1.02622411503681)))
REPRESENTATION_ITEM('')
SURFACE()
);
#1568=(
BOUNDED_SURFACE()
B_SPLINE_SURFACE(3,2,((#41718,#41719,#41720),(#41721,#41722,#41723),(#41724,
#41725,#41726),(#41727,#41728,#41729),(#41730,#41731,#41732)),
 .UNSPECIFIED.,.F.,.F.,.F.)
B_SPLINE_SURFACE_WITH_KNOTS((4,1,4),(3,3),(0.00247947538704121,0.0051691692688655,
0.00785885309266148),(0.,1.00371535323371),.UNSPECIFIED.)
GEOMETRIC_REPRESENTATION_ITEM()
RATIONAL_B_SPLINE_SURFACE(((1.,0.705970164087497,1.00218484940333),(1.,
0.705972859468082,1.00218482937474),(1.,0.70605787745789,1.00218419763102),
(1.,0.705986056430116,1.00218473131199),(1.,0.705985239891227,1.00218473737945)))
REPRESENTATION_ITEM('')
SURFACE()
);
#1569=(
BOUNDED_SURFACE()
B_SPLINE_SURFACE(3,2,((#41778,#41779,#41780),(#41781,#41782,#41783),(#41784,
#41785,#41786),(#41787,#41788,#41789),(#41790,#41791,#41792)),
 .UNSPECIFIED.,.F.,.F.,.F.)
B_SPLINE_SURFACE_WITH_KNOTS((4,1,4),(3,3),(0.00267719565163109,0.00526763354664624,
0.00785807144166138),(0.,1.00296412736609),.UNSPECIFIED.)
GEOMETRIC_REPRESENTATION_ITEM()
RATIONAL_B_SPLINE_SURFACE(((1.,0.706205282353514,1.00174168992518),(1.,
0.706208521892236,1.00174167072037),(1.,0.706274936988307,1.00174127699476),
(1.,0.706196203322784,1.00174174374799),(1.,0.706190892079292,1.00174177523439)))
REPRESENTATION_ITEM('')
SURFACE()
);
#1570=(
BOUNDED_SURFACE()
B_SPLINE_SURFACE(3,2,((#41808,#41809,#41810),(#41811,#41812,#41813),(#41814,
#41815,#41816),(#41817,#41818,#41819),(#41820,#41821,#41822)),
 .UNSPECIFIED.,.F.,.F.,.F.)
B_SPLINE_SURFACE_WITH_KNOTS((4,1,4),(3,3),(0.00221168766977545,0.00528551896642512,
0.00836848652357398),(-0.00323543465076996,1.0329973662126),
 .UNSPECIFIED.)
GEOMETRIC_REPRESENTATION_ITEM()
RATIONAL_B_SPLINE_SURFACE(((1.00190156217512,0.696406930093278,1.01996887164199),
(1.00190175990839,0.696375361075404,1.01997094809804),(1.00190098872769,
0.696498483590981,1.01996284969938),(1.00190188263966,0.696355766470008,
1.01997223693562),(1.00190164269477,0.696394074764875,1.0199697172028)))
REPRESENTATION_ITEM('')
SURFACE()
);
#1571=(
BOUNDED_SURFACE()
B_SPLINE_SURFACE(3,2,((#41854,#41855,#41856),(#41857,#41858,#41859),(#41860,
#41861,#41862),(#41863,#41864,#41865),(#41866,#41867,#41868)),
 .UNSPECIFIED.,.F.,.F.,.F.)
B_SPLINE_SURFACE_WITH_KNOTS((4,1,4),(3,3),(0.00211918404214125,0.00520185796130005,
0.00828451973195975),(-0.00495630116524082,1.03080453538952),
 .UNSPECIFIED.)
GEOMETRIC_REPRESENTATION_ITEM()
RATIONAL_B_SPLINE_SURFACE(((1.00291808547175,0.6965056233853,1.01860304884576),
(1.0029184535517,0.696467341369736,1.01860539538744),(1.00291708203809,
0.696609985124191,1.01859665186883),(1.00291827395877,0.696486019864228,
1.01860425046691),(1.00291796306127,0.696518354641951,1.01860226846824)))
REPRESENTATION_ITEM('')
SURFACE()
);
#1572=(
BOUNDED_SURFACE()
B_SPLINE_SURFACE(3,2,((#41869,#41870,#41871),(#41872,#41873,#41874),(#41875,
#41876,#41877),(#41878,#41879,#41880),(#41881,#41882,#41883),(#41884,#41885,
#41886)),.UNSPECIFIED.,.F.,.F.,.F.)
B_SPLINE_SURFACE_WITH_KNOTS((4,1,1,4),(3,3),(0.00206501500476494,0.00583597574226651,
0.00742288849389084,0.00960693139660508),(-0.0135007365230585,1.00552142297207),
 .UNSPECIFIED.)
GEOMETRIC_REPRESENTATION_ITEM()
RATIONAL_B_SPLINE_SURFACE(((1.00801609181928,0.701462893341436,1.00325254638159),
(1.00801649298684,0.701447952968216,1.00325270915619),(1.00801421110542,
0.701532935312785,1.00325178327793),(1.0080170203036,0.701428314518215,
1.00325292311609),(1.00802044103978,0.701300918686746,1.0032543110871),
(1.00801836836181,0.701378109829282,1.00325347009359)))
REPRESENTATION_ITEM('')
SURFACE()
);
#1573=(
BOUNDED_SURFACE()
B_SPLINE_SURFACE(3,2,((#41920,#41921,#41922),(#41923,#41924,#41925),(#41926,
#41927,#41928),(#41929,#41930,#41931),(#41932,#41933,#41934),(#41935,#41936,
#41937)),.UNSPECIFIED.,.F.,.F.,.F.)
B_SPLINE_SURFACE_WITH_KNOTS((4,1,1,4),(3,3),(0.00206609914260828,0.00583090828463318,
0.00741523232466728,0.00959571243431081),(-0.00622355113870663,1.01477263265198),
 .UNSPECIFIED.)
GEOMETRIC_REPRESENTATION_ITEM()
RATIONAL_B_SPLINE_SURFACE(((1.00366871744853,0.700874212332019,1.00878229800042),
(1.00366887894059,0.700861045213046,1.00878268458549),(1.00366786004834,
0.700944119734037,1.00878024552731),(1.00366914086107,0.700839689747176,
1.00878331157946),(1.00367078368537,0.700705743451035,1.00878724422698),
(1.00366979976439,0.700785966619564,1.00878488888418)))
REPRESENTATION_ITEM('')
SURFACE()
);
#1574=(
BOUNDED_SURFACE()
B_SPLINE_SURFACE(3,2,((#41966,#41967,#41968),(#41969,#41970,#41971),(#41972,
#41973,#41974),(#41975,#41976,#41977),(#41978,#41979,#41980),(#41981,#41982,
#41983)),.UNSPECIFIED.,.F.,.F.,.F.)
B_SPLINE_SURFACE_WITH_KNOTS((4,1,1,4),(3,3),(0.00207738560236064,0.00585322491241914,
0.00744219183711539,0.0096290583604494),(-0.00990380407034745,1.06114958053671),
 .UNSPECIFIED.)
GEOMETRIC_REPRESENTATION_ITEM()
RATIONAL_B_SPLINE_SURFACE(((1.00585937207028,0.685919476704603,1.03801361024168),
(1.00586010065921,0.685880422077222,1.03801833707851),(1.00585811055901,
0.685987097622889,1.03800542598624),(1.00586022036471,0.685874005491064,
1.03801911368701),(1.00586244311324,0.685754859273445,1.03803353412235),
(1.00586161631504,0.685799178222131,1.03802817013727)))
REPRESENTATION_ITEM('')
SURFACE()
);
#1575=(
BOUNDED_SURFACE()
B_SPLINE_SURFACE(3,2,((#42017,#42018,#42019),(#42020,#42021,#42022),(#42023,
#42024,#42025),(#42026,#42027,#42028),(#42029,#42030,#42031),(#42032,#42033,
#42034)),.UNSPECIFIED.,.F.,.F.,.F.)
B_SPLINE_SURFACE_WITH_KNOTS((4,1,1,4),(3,3),(0.00207838220750666,0.00584814811204442,
0.00743455922903145,0.00961791173284076),(-0.0645177248056397,1.00996895944737),
 .UNSPECIFIED.)
GEOMETRIC_REPRESENTATION_ITEM()
RATIONAL_B_SPLINE_SURFACE(((1.0402346106114,0.684892659950512,1.0058982845107),
(1.04023973342761,0.684852539343795,1.00589903550163),(1.04022614361739,
0.684958971315759,1.0058970432724),(1.040240467454,0.684846790633866,1.0058991431079),
(1.04025671917778,0.684719511225116,1.00590152556641),(1.04025057634624,
0.684767620335115,1.00590062504401)))
REPRESENTATION_ITEM('')
SURFACE()
);
#1576=(
BOUNDED_SURFACE()
B_SPLINE_SURFACE(3,2,((#42035,#42036,#42037),(#42038,#42039,#42040),(#42041,
#42042,#42043),(#42044,#42045,#42046),(#42047,#42048,#42049)),
 .UNSPECIFIED.,.F.,.F.,.F.)
B_SPLINE_SURFACE_WITH_KNOTS((4,1,4),(3,3),(0.00242285948437873,0.0051736196439449,
0.00792436969222164),(0.,1.00437695596552),.UNSPECIFIED.)
GEOMETRIC_REPRESENTATION_ITEM()
RATIONAL_B_SPLINE_SURFACE(((1.,0.705776383171405,1.00257560762975),(1.,
0.705777293944189,1.00257559965693),(1.,0.705865449509473,1.00257482795087),
(1.,0.705791558721078,1.00257547478433),(0.999999999999999,0.705792282982492,
1.0025754684442)))
REPRESENTATION_ITEM('')
SURFACE()
);
#1577=(
BOUNDED_SURFACE()
B_SPLINE_SURFACE(3,2,((#42095,#42096,#42097),(#42098,#42099,#42100),(#42101,
#42102,#42103),(#42104,#42105,#42106),(#42107,#42108,#42109)),
 .UNSPECIFIED.,.F.,.F.,.F.)
B_SPLINE_SURFACE_WITH_KNOTS((4,1,4),(3,3),(0.00243078313184364,0.00527111731602525,
0.00811144338637717),(0.,1.00382472942682),.UNSPECIFIED.)
GEOMETRIC_REPRESENTATION_ITEM()
RATIONAL_B_SPLINE_SURFACE(((1.,0.705953974699161,1.00224929297161),(1.,
0.705950577782826,1.00224931895619),(1.,0.706029820377507,1.00224871279322),
(1.,0.705936375867464,1.00224942759315),(1.,0.705938430322632,1.00224941187768)))
REPRESENTATION_ITEM('')
SURFACE()
);
#1578=(
BOUNDED_SURFACE()
B_SPLINE_SURFACE(3,2,((#42125,#42126,#42127),(#42128,#42129,#42130),(#42131,
#42132,#42133),(#42134,#42135,#42136),(#42137,#42138,#42139)),
 .UNSPECIFIED.,.F.,.F.,.F.)
B_SPLINE_SURFACE_WITH_KNOTS((4,1,4),(3,3),(0.00221566111994076,0.00529019030192516,
0.00837375924116679),(-0.00339130215178826,1.03561277968481),
 .UNSPECIFIED.)
GEOMETRIC_REPRESENTATION_ITEM()
RATIONAL_B_SPLINE_SURFACE(((1.00199347489228,0.695587723001425,1.02160614203281),
(1.00199368000553,0.695556401317895,1.02160836513876),(1.00199288246575,
0.695678189106253,1.02159972105817),(1.00199381434552,0.695535887017177,
1.02160982117364),(1.00199356332364,0.695574219148555,1.02160710049009)))
REPRESENTATION_ITEM('')
SURFACE()
);
#1579=(
BOUNDED_SURFACE()
B_SPLINE_SURFACE(3,2,((#42169,#42170,#42171),(#42172,#42173,#42174),(#42175,
#42176,#42177),(#42178,#42179,#42180),(#42181,#42182,#42183)),
 .UNSPECIFIED.,.F.,.F.,.F.)
B_SPLINE_SURFACE_WITH_KNOTS((4,1,4),(3,3),(0.00212349273369012,0.00520565186730131,
0.00828779885095397),(-0.00480844917136824,1.03341610948654),
 .UNSPECIFIED.)
GEOMETRIC_REPRESENTATION_ITEM()
RATIONAL_B_SPLINE_SURFACE(((1.00283061667055,0.69577951134894,1.02023130347533),
(1.00283097276619,0.695741239975037,1.02023384860233),(1.00282965163483,
0.695883228549338,1.02022440606297),(1.00283079197036,0.6957606710036,1.02023255639799),
(1.00283049396244,0.695792699401415,1.02023042644205)))
REPRESENTATION_ITEM('')
SURFACE()
);
#1580=(
BOUNDED_SURFACE()
B_SPLINE_SURFACE(3,2,((#42184,#42185,#42186),(#42187,#42188,#42189),(#42190,
#42191,#42192),(#42193,#42194,#42195),(#42196,#42197,#42198)),
 .UNSPECIFIED.,.F.,.F.,.F.)
B_SPLINE_SURFACE_WITH_KNOTS((4,1,4),(3,3),(0.00211837924580892,0.00519732079082784,
0.00827625862043334),(-0.00532010498308729,1.01360000328723),
 .UNSPECIFIED.)
GEOMETRIC_REPRESENTATION_ITEM()
RATIONAL_B_SPLINE_SURFACE(((1.00313352122389,0.701475567287313,1.00807632313618),
(1.00313363791523,0.70146445033165,1.00807662389591),(1.00313251661584,
0.701571274329799,1.00807373386403),(1.00313341826975,0.701485375526323,
1.00807605778267),(1.00313330429228,0.701496233936907,1.00807576401766)))
REPRESENTATION_ITEM('')
SURFACE()
);
#1581=(
BOUNDED_SURFACE()
B_SPLINE_SURFACE(3,2,((#42243,#42244,#42245),(#42246,#42247,#42248),(#42249,
#42250,#42251),(#42252,#42253,#42254),(#42255,#42256,#42257)),
 .UNSPECIFIED.,.F.,.F.,.F.)
B_SPLINE_SURFACE_WITH_KNOTS((4,1,4),(3,3),(0.00211872601142628,0.00519507594284825,
0.00827142282117545),(-0.0125752621045938,1.00753736038806),
 .UNSPECIFIED.)
GEOMETRIC_REPRESENTATION_ITEM()
RATIONAL_B_SPLINE_SURFACE(((1.00746022322175,0.701113508392646,1.00444926121364),
(1.00746049609062,0.701102576170414,1.00444942395205),(1.00745784401348,
0.701208829027323,1.00444784225891),(1.00745999974221,0.701122461880137,
1.00444912793092),(1.00745972953064,0.701133287640395,1.00444896677732)))
REPRESENTATION_ITEM('')
SURFACE()
);
#1582=(
BOUNDED_SURFACE()
B_SPLINE_SURFACE(3,2,((#42273,#42274,#42275),(#42276,#42277,#42278),(#42279,
#42280,#42281),(#42282,#42283,#42284),(#42285,#42286,#42287)),
 .UNSPECIFIED.,.F.,.F.,.F.)
B_SPLINE_SURFACE_WITH_KNOTS((4,1,4),(3,3),(0.00214652638394637,0.00523052097319175,
0.00831451160094196),(-0.0445550628231248,1.00430563736809),
 .UNSPECIFIED.)
GEOMETRIC_REPRESENTATION_ITEM()
RATIONAL_B_SPLINE_SURFACE(((1.02726594007204,0.692646097681134,1.00253335135591),
(1.02726933899953,0.69260778344634,1.00253366715935),(1.02725699574049,
0.692746922196893,1.00253252031417),(1.02726708176979,0.692633227952121,
1.0025334574341),(1.02726443043493,0.692663114987534,1.0025332110915)))
REPRESENTATION_ITEM('')
SURFACE()
);
#1583=(
BOUNDED_SURFACE()
B_SPLINE_SURFACE(3,2,((#42317,#42318,#42319),(#42320,#42321,#42322),(#42323,
#42324,#42325),(#42326,#42327,#42328),(#42329,#42330,#42331)),
 .UNSPECIFIED.,.F.,.F.,.F.)
B_SPLINE_SURFACE_WITH_KNOTS((4,1,4),(3,3),(0.00214672101519236,0.00522830221175709,
0.00830987665062646),(-0.00501736956493107,1.04391786530058),
 .UNSPECIFIED.)
GEOMETRIC_REPRESENTATION_ITEM()
RATIONAL_B_SPLINE_SURFACE(((1.00295420698496,0.692608136042445,1.02685955507165),
(1.00295457482959,0.692569860983192,1.02686289950325),(1.00295324247231,
0.692708495747623,1.02685078575358),(1.00295434419837,0.692593858679657,
1.02686080261154),(1.0029540534599,0.692624110668846,1.02685815922678)))
REPRESENTATION_ITEM('')
SURFACE()
);
#1584=(
BOUNDED_SURFACE()
B_SPLINE_SURFACE(3,2,((#42332,#42333,#42334),(#42335,#42336,#42337),(#42338,
#42339,#42340),(#42341,#42342,#42343),(#42344,#42345,#42346)),
 .UNSPECIFIED.,.F.,.F.,.F.)
B_SPLINE_SURFACE_WITH_KNOTS((4,1,4),(3,3),(0.00212309359701631,0.00520196736840092,
0.00828083965993362),(-0.00538667073334126,1.01435395411296),
 .UNSPECIFIED.)
GEOMETRIC_REPRESENTATION_ITEM()
RATIONAL_B_SPLINE_SURFACE(((1.00317292968628,0.701233103961014,1.00853037209161),
(1.00317304291575,0.701222442137482,1.00853067650727),(1.00317192956387,
0.70132727669669,1.00852768327806),(1.00317283024653,0.701242467328061,
1.00853010474939),(1.00317271575512,0.701253247978216,1.008529796941)))
REPRESENTATION_ITEM('')
SURFACE()
);
#1585=(
BOUNDED_SURFACE()
B_SPLINE_SURFACE(3,2,((#42391,#42392,#42393),(#42394,#42395,#42396),(#42397,
#42398,#42399),(#42400,#42401,#42402),(#42403,#42404,#42405)),
 .UNSPECIFIED.,.F.,.F.,.F.)
B_SPLINE_SURFACE_WITH_KNOTS((4,1,4),(3,3),(0.00212328649712472,0.00520006178542504,
0.0082768361456668),(-0.0121981081337134,1.00757620462087),
 .UNSPECIFIED.)
GEOMETRIC_REPRESENTATION_ITEM()
RATIONAL_B_SPLINE_SURFACE(((1.00723375242928,0.701215254384846,1.00447234439468),
(1.00723400107668,0.701204984189714,1.00447249812358),(1.00723150164427,
0.701308221379959,1.0044709528229),(1.00723356035961,0.701223187679178,
1.00447222564556),(1.00723330348688,0.701233797615521,1.00447206683127)))
REPRESENTATION_ITEM('')
SURFACE()
);
#1586=(
BOUNDED_SURFACE()
B_SPLINE_SURFACE(3,2,((#42421,#42422,#42423),(#42424,#42425,#42426),(#42427,
#42428,#42429),(#42430,#42431,#42432),(#42433,#42434,#42435)),
 .UNSPECIFIED.,.F.,.F.,.F.)
B_SPLINE_SURFACE_WITH_KNOTS((4,1,4),(3,3),(0.00215121360431741,0.00523488372589789,
0.00831855159752948),(-0.0446503843220741,1.00450356492348),
 .UNSPECIFIED.)
GEOMETRIC_REPRESENTATION_ITEM()
RATIONAL_B_SPLINE_SURFACE(((1.02732668542833,0.692555691390288,1.00265032234403),
(1.02733007044875,0.692517607544939,1.00265065064566),(1.02731787184475,
0.692654850364981,1.00264946754452),(1.0273278731463,0.692542328733031,
1.00265043753676),(1.0273252504547,0.692571835846397,1.00265018317082)))
REPRESENTATION_ITEM('')
SURFACE()
);
#1587=(
BOUNDED_SURFACE()
B_SPLINE_SURFACE(3,2,((#42465,#42466,#42467),(#42468,#42469,#42470),(#42471,
#42472,#42473),(#42474,#42475,#42476),(#42477,#42478,#42479)),
 .UNSPECIFIED.,.F.,.F.,.F.)
B_SPLINE_SURFACE_WITH_KNOTS((4,1,4),(3,3),(0.0021508461774662,0.0052332832138809,
0.00831571518714347),(-0.00531073766834972,1.04411327492098),
 .UNSPECIFIED.)
GEOMETRIC_REPRESENTATION_ITEM()
RATIONAL_B_SPLINE_SURFACE(((1.00312783777046,0.692458369995794,1.02698397756318),
(1.00312822235194,0.692420556392284,1.02698729536256),(1.00312684516247,
0.692555967217898,1.02697541429566),(1.00312799463627,0.692442946316364,
1.02698533085061),(1.0031276897709,0.692472921909204,1.02698270076529)))
REPRESENTATION_ITEM('')
SURFACE()
);
#1588=(
BOUNDED_SURFACE()
B_SPLINE_SURFACE(3,2,((#42480,#42481,#42482),(#42483,#42484,#42485),(#42486,
#42487,#42488),(#42489,#42490,#42491),(#42492,#42493,#42494)),
 .UNSPECIFIED.,.F.,.F.,.F.)
B_SPLINE_SURFACE_WITH_KNOTS((4,1,4),(3,3),(0.0021280017507586,0.00520643335911326,
0.00828486609849074),(-0.00545222989642442,1.01483574006136),
 .UNSPECIFIED.)
GEOMETRIC_REPRESENTATION_ITEM()
RATIONAL_B_SPLINE_SURFACE(((1.00321174730507,0.701071451701929,1.00882085607408),
(1.00321185722931,0.701061220668788,1.00882115797388),(1.00321075044288,
0.701164233150451,1.0088181182566),(1.00321165357415,0.701080175566389,
1.00882059864817),(1.00321153695881,0.701091029363851,1.00882027837168)))
REPRESENTATION_ITEM('')
SURFACE()
);
#1589=(
BOUNDED_SURFACE()
B_SPLINE_SURFACE(3,2,((#42539,#42540,#42541),(#42542,#42543,#42544),(#42545,
#42546,#42547),(#42548,#42549,#42550),(#42551,#42552,#42553)),
 .UNSPECIFIED.,.F.,.F.,.F.)
B_SPLINE_SURFACE_WITH_KNOTS((4,1,4),(3,3),(0.00212778800052849,0.0052053406359233,
0.00828289438645528),(-0.0123411007820522,1.00604991564916),
 .UNSPECIFIED.)
GEOMETRIC_REPRESENTATION_ITEM()
RATIONAL_B_SPLINE_SURFACE(((1.00731954899057,0.701632309420459,1.00356592662071),
(1.00731978090901,0.701622855700233,1.00356603960637),(1.00731734036416,
0.701722339935083,1.00356485062549),(1.00731937739681,0.701639304118356,
1.00356584302392),(1.00731912529299,0.701649580657985,1.00356572020437)))
REPRESENTATION_ITEM('')
SURFACE()
);
#1590=(
BOUNDED_SURFACE()
B_SPLINE_SURFACE(3,2,((#42569,#42570,#42571),(#42572,#42573,#42574),(#42575,
#42576,#42577),(#42578,#42579,#42580),(#42581,#42582,#42583)),
 .UNSPECIFIED.,.F.,.F.,.F.)
B_SPLINE_SURFACE_WITH_KNOTS((4,1,4),(3,3),(0.0021560260114394,0.00523931072137745,
0.00832259563410914),(-0.0447835452829565,1.00470829840081),
 .UNSPECIFIED.)
GEOMETRIC_REPRESENTATION_ITEM()
RATIONAL_B_SPLINE_SURFACE(((1.02741159374151,0.692451908000683,1.00277136329061),
(1.02741496864924,0.692414042765858,1.00277170450009),(1.02740290435876,
0.692549399708443,1.0027704847778),(1.02741282944973,0.692438043804821,
1.00277148822302),(1.02741023266766,0.692467178753231,1.00277122568351)))
REPRESENTATION_ITEM('')
SURFACE()
);
#1591=(
BOUNDED_SURFACE()
B_SPLINE_SURFACE(3,2,((#42613,#42614,#42615),(#42616,#42617,#42618),(#42619,
#42620,#42621),(#42622,#42623,#42624),(#42625,#42626,#42627)),
 .UNSPECIFIED.,.F.,.F.,.F.)
B_SPLINE_SURFACE_WITH_KNOTS((4,1,4),(3,3),(0.00215602788258475,0.00523917993081111,
0.00832232919221315),(-0.00552106013962827,1.04545478644752),
 .UNSPECIFIED.)
GEOMETRIC_REPRESENTATION_ITEM()
RATIONAL_B_SPLINE_SURFACE(((1.00325239185633,0.691993903191183,1.02784031168291),
(1.00325279353845,0.691955863327452,1.0278437500618),(1.00325135869187,
0.692091745322464,1.02783146784683),(1.00325255025752,0.691978902374865,
1.02784166758919),(1.00325223397536,0.692008854742086,1.02783896022967)))
REPRESENTATION_ITEM('')
SURFACE()
);
#1592=(
BOUNDED_SURFACE()
B_SPLINE_SURFACE(3,2,((#42628,#42629,#42630),(#42631,#42632,#42633),(#42634,
#42635,#42636),(#42637,#42638,#42639),(#42640,#42641,#42642)),
 .UNSPECIFIED.,.F.,.F.,.F.)
B_SPLINE_SURFACE_WITH_KNOTS((4,1,4),(3,3),(0.00213299782738826,0.00521097577115018,
0.00828895484434125),(-0.00550087397147942,1.01477086238353),
 .UNSPECIFIED.)
GEOMETRIC_REPRESENTATION_ITEM()
RATIONAL_B_SPLINE_SURFACE(((1.003240550509,0.701076763936148,1.0087816978033),
(1.00324065665487,0.701066972554508,1.00878198545225),(1.00323955961029,
0.701168168976641,1.00877901252713),(1.00324046420802,0.701084724734234,
1.00878146393281),(1.00324034568342,0.701095657987022,1.00878114273824)))
REPRESENTATION_ITEM('')
SURFACE()
);
#1593=(
BOUNDED_SURFACE()
B_SPLINE_SURFACE(3,2,((#42687,#42688,#42689),(#42690,#42691,#42692),(#42693,
#42694,#42695),(#42696,#42697,#42698),(#42699,#42700,#42701)),
 .UNSPECIFIED.,.F.,.F.,.F.)
B_SPLINE_SURFACE_WITH_KNOTS((4,1,4),(3,3),(0.00213310765920635,0.00521163324568507,
0.00829015996762764),(-0.0156377890551712,1.00702192656802),
 .UNSPECIFIED.)
GEOMETRIC_REPRESENTATION_ITEM()
RATIONAL_B_SPLINE_SURFACE(((1.00930506145392,0.700360232778602,1.00414285996969),
(1.00930536821373,0.700350354559057,1.00414299654729),(1.00930220263952,
0.700452291760049,1.00414158714976),(1.00930480530383,0.700368481273429,
1.00414274592489),(1.00930448227842,0.700378883274418,1.00414260210542)))
REPRESENTATION_ITEM('')
SURFACE()
);
#1594=(
BOUNDED_SURFACE()
B_SPLINE_SURFACE(3,2,((#42717,#42718,#42719),(#42720,#42721,#42722),(#42723,
#42724,#42725),(#42726,#42727,#42728),(#42729,#42730,#42731)),
 .UNSPECIFIED.,.F.,.F.,.F.)
B_SPLINE_SURFACE_WITH_KNOTS((4,1,4),(3,3),(0.00216106225273672,0.00524376924181206,
0.00832647862208329),(-0.0446517915472245,1.00491634737552),
 .UNSPECIFIED.)
GEOMETRIC_REPRESENTATION_ITEM()
RATIONAL_B_SPLINE_SURFACE(((1.02732742650838,0.692425328535973,1.00289441476859),
(1.02733077687705,0.692387619586655,1.00289476962662),(1.02731889160327,
0.6925213902941,1.00289351078463),(1.02732871811155,0.69241079133026,1.00289455157018),
(1.02732615236371,0.692439669243409,1.00289427981614)))
REPRESENTATION_ITEM('')
SURFACE()
);
#1595=(
BOUNDED_SURFACE()
B_SPLINE_SURFACE(3,2,((#42756,#42757,#42758),(#42759,#42760,#42761),(#42762,
#42763,#42764),(#42765,#42766,#42767),(#42768,#42769,#42770)),
 .UNSPECIFIED.,.F.,.F.,.F.)
B_SPLINE_SURFACE_WITH_KNOTS((4,1,4),(3,3),(0.00216083159531938,0.00524514060142026,
0.00832944899172471),(-0.00570770278406545,1.04561266300805),
 .UNSPECIFIED.)
GEOMETRIC_REPRESENTATION_ITEM()
RATIONAL_B_SPLINE_SURFACE(((1.00336295925547,0.691888008928606,1.02794117990572),
(1.00336337356489,0.691850050187208,1.0279446221996),(1.00336190347963,
0.69198473837774,1.02793240798181),(1.00336312152517,0.69187314189091,1.02794252812516),
(1.00336279729876,0.691902847289583,1.02793983428684)))
REPRESENTATION_ITEM('')
SURFACE()
);
#1596=(
BOUNDED_SURFACE()
B_SPLINE_SURFACE(3,2,((#42771,#42772,#42773),(#42774,#42775,#42776),(#42777,
#42778,#42779),(#42780,#42781,#42782),(#42783,#42784,#42785),(#42786,#42787,
#42788)),.UNSPECIFIED.,.F.,.F.,.F.)
B_SPLINE_SURFACE_WITH_KNOTS((4,1,1,4),(3,3),(0.00206897381009835,0.00584008937427813,
0.00742706726542499,0.00961119981566884),(-0.0133262372495361,1.00554811092291),
 .UNSPECIFIED.)
GEOMETRIC_REPRESENTATION_ITEM()
RATIONAL_B_SPLINE_SURFACE(((1.00791112140402,0.701506499763767,1.00326835491122),
(1.00791150703105,0.701491949720231,1.00326851422694),(1.00790926322385,
0.701576610520087,1.00326758723341),(1.00791204091466,0.701471805826733,
1.00326873479252),(1.0079153810578,0.701345779317039,1.00327011471993),
(1.00791335564888,0.70142219975936,1.00326927795421)))
REPRESENTATION_ITEM('')
SURFACE()
);
#1597=(
BOUNDED_SURFACE()
B_SPLINE_SURFACE(3,2,((#42821,#42822,#42823),(#42824,#42825,#42826),(#42827,
#42828,#42829),(#42830,#42831,#42832),(#42833,#42834,#42835),(#42836,#42837,
#42838)),.UNSPECIFIED.,.F.,.F.,.F.)
B_SPLINE_SURFACE_WITH_KNOTS((4,1,1,4),(3,3),(0.00206996661703809,0.0058353060121813,
0.00741985318197331,0.00960064037745484),(-0.00834800729421259,1.01461865695033),
 .UNSPECIFIED.)
GEOMETRIC_REPRESENTATION_ITEM()
RATIONAL_B_SPLINE_SURFACE(((1.00493145052503,0.700279457869589,1.00868943892189),
(1.0049316670474,0.700266298211422,1.00868982044411),(1.00493030045999,
0.700349355786042,1.00868741245526),(1.004932019035,0.700244905334656,1.00869044066218),
(1.00493419864013,0.700112434689801,1.00869428122502),(1.00493289102759,
0.700191907927257,1.00869197715257)))
REPRESENTATION_ITEM('')
SURFACE()
);
#1598=(
BOUNDED_SURFACE()
B_SPLINE_SURFACE(3,2,((#42857,#42858,#42859),(#42860,#42861,#42862),(#42863,
#42864,#42865),(#42866,#42867,#42868),(#42869,#42870,#42871),(#42872,#42873,
#42874)),.UNSPECIFIED.,.F.,.F.,.F.)
B_SPLINE_SURFACE_WITH_KNOTS((4,1,1,4),(3,3),(0.00208137534035049,0.00585739874086686,
0.00744644313070167,0.00963341629415647),(-0.0100342287213997,1.06112763756809),
 .UNSPECIFIED.)
GEOMETRIC_REPRESENTATION_ITEM()
RATIONAL_B_SPLINE_SURFACE(((1.0059372961562,0.685883449975777,1.03799914827316),
(1.00593804189723,0.685843996057386,1.03800392107261),(1.00593602425211,
0.685950740896645,1.03799100798995),(1.00593815920701,0.685837789706304,
1.03800467186417),(1.00594039944253,0.685719268576007,1.03801900954234),
(1.00593956271628,0.685763536127451,1.03801365443052)))
REPRESENTATION_ITEM('')
SURFACE()
);
#1599=(
BOUNDED_SURFACE()
B_SPLINE_SURFACE(3,2,((#42908,#42909,#42910),(#42911,#42912,#42913),(#42914,
#42915,#42916),(#42917,#42918,#42919),(#42920,#42921,#42922),(#42923,#42924,
#42925)),.UNSPECIFIED.,.F.,.F.,.F.)
B_SPLINE_SURFACE_WITH_KNOTS((4,1,1,4),(3,3),(0.00208245624318126,0.00585171550471199,
0.00743791339961705,0.0096209724434026),(-0.0634162322184188,1.00964045485374),
 .UNSPECIFIED.)
GEOMETRIC_REPRESENTATION_ITEM()
RATIONAL_B_SPLINE_SURFACE(((1.0395067583518,0.685330296084069,1.0057020621191),
(1.03951179919293,0.685290145992003,1.00570278967029),(1.03949841639537,
0.685396739423676,1.00570085811361),(1.03951261007788,0.685283687326768,
1.00570290670638),(1.03952817116967,0.685159743871252,1.00570515265912),
(1.0395222844102,0.685206631668106,1.00570430301542)))
REPRESENTATION_ITEM('')
SURFACE()
);
#1600=(
BOUNDED_SURFACE()
B_SPLINE_SURFACE(3,2,((#42926,#42927,#42928),(#42929,#42930,#42931),(#42932,
#42933,#42934),(#42935,#42936,#42937),(#42938,#42939,#42940),(#42941,#42942,
#42943)),.UNSPECIFIED.,.F.,.F.,.F.)
B_SPLINE_SURFACE_WITH_KNOTS((4,1,1,4),(3,3),(0.00207550115510636,0.00583206770309977,
0.00741292302561788,0.00958862921574725),(-0.0139548191437294,1.00546415117684),
 .UNSPECIFIED.)
GEOMETRIC_REPRESENTATION_ITEM()
RATIONAL_B_SPLINE_SURFACE(((1.00828942257687,0.701345444582124,1.00321862782116),
(1.00828980522591,0.701331658352956,1.00321877639663),(1.00828751542455,
0.701414156211213,1.00321788730956),(1.00829030395828,0.701313689828347,
1.00321897004508),(1.0082938627312,0.701185472967017,1.00322035185008),
(1.00829178378737,0.701260373967849,1.00321954463505)))
REPRESENTATION_ITEM('')
SURFACE()
);
#1601=(
BOUNDED_SURFACE()
B_SPLINE_SURFACE(3,2,((#42979,#42980,#42981),(#42982,#42983,#42984),(#42985,
#42986,#42987),(#42988,#42989,#42990),(#42991,#42992,#42993),(#42994,#42995,
#42996)),.UNSPECIFIED.,.F.,.F.,.F.)
B_SPLINE_SURFACE_WITH_KNOTS((4,1,1,4),(3,3),(0.00562012573083522,0.00630029289699113,
0.00664037648006909,0.00698046006314705),(0.,1.00004938595224),
 .UNSPECIFIED.)
GEOMETRIC_REPRESENTATION_ITEM()
RATIONAL_B_SPLINE_SURFACE(((1.,0.704092907135692,1.00002922730711),(1.,
0.704090406431475,1.00002922755411),(1.,0.703664702577133,1.00002926960169),
(1.,0.702970262149341,1.0000293381929),(1.,0.703271663610187,1.0000293084229),
(1.,0.703272425211359,1.00002930834768)))
REPRESENTATION_ITEM('')
SURFACE()
);
#1602=(
BOUNDED_SURFACE()
B_SPLINE_SURFACE(3,2,((#43011,#43012,#43013),(#43014,#43015,#43016),(#43017,
#43018,#43019),(#43020,#43021,#43022),(#43023,#43024,#43025),(#43026,#43027,
#43028)),.UNSPECIFIED.,.F.,.F.,.F.)
B_SPLINE_SURFACE_WITH_KNOTS((4,1,1,4),(3,3),(0.00207453111129043,0.00583682887046017,
0.00742009603050453,0.00959912157199512),(-0.00709208229884144,1.01455199349045),
 .UNSPECIFIED.)
GEOMETRIC_REPRESENTATION_ITEM()
RATIONAL_B_SPLINE_SURFACE(((1.00418431442723,0.700677941873041,1.00864924429771),
(1.00418449834326,0.700664785565795,1.00864962446387),(1.00418333960424,
0.700747675165923,1.00864722927654),(1.00418479483858,0.700643575977048,
1.00865023733856),(1.00418663690651,0.700511804913243,1.00865404501023),
(1.00418553484717,0.700590639970702,1.00865176698343)))
REPRESENTATION_ITEM('')
SURFACE()
);
#1603=(
BOUNDED_SURFACE()
B_SPLINE_SURFACE(3,2,((#43051,#43052,#43053),(#43054,#43055,#43056),(#43057,
#43058,#43059),(#43060,#43061,#43062),(#43063,#43064,#43065),(#43066,#43067,
#43068)),.UNSPECIFIED.,.F.,.F.,.F.)
B_SPLINE_SURFACE_WITH_KNOTS((4,1,1,4),(3,3),(0.00211751772537189,0.00570450909625921,
0.00721400412766881,0.00929149854507189),(-0.00844675675792914,1.05533037709487),
 .UNSPECIFIED.)
GEOMETRIC_REPRESENTATION_ITEM()
RATIONAL_B_SPLINE_SURFACE(((1.00499014862227,0.688130707990867,1.03420759866455),
(1.00499072016438,0.688094988326579,1.0342115166006),(1.00498920859429,
0.688189456914593,1.03420115474828),(1.00499054744122,0.688105783004858,
1.03421033257886),(1.00499226460991,0.687998465122432,1.0342221038149),
(1.0049914820894,0.688047370302582,1.03421673961645)))
REPRESENTATION_ITEM('')
SURFACE()
);
#1604=(
BOUNDED_SURFACE()
B_SPLINE_SURFACE(3,2,((#43083,#43084,#43085),(#43086,#43087,#43088),(#43089,
#43090,#43091),(#43092,#43093,#43094),(#43095,#43096,#43097),(#43098,#43099,
#43100)),.UNSPECIFIED.,.F.,.F.,.F.)
B_SPLINE_SURFACE_WITH_KNOTS((4,1,1,4),(3,3),(0.00606474645459548,0.00687768219289253,
0.00721978592523264,0.00769061870795424),(-0.00208860429383766,1.00954344417007),
 .UNSPECIFIED.)
GEOMETRIC_REPRESENTATION_ITEM()
RATIONAL_B_SPLINE_SURFACE(((1.00124267640761,0.699665335788881,1.00572039361805),
(1.00124236841496,0.699739772599195,1.00571897584013),(1.00124365335567,
0.699429223342106,1.00572489078835),(1.00123971608937,0.700380796529177,
1.00570676642965),(1.00123395160836,0.701773977778471,1.00568023088088),
(1.00123674694762,0.701098389771248,1.00569309862406)))
REPRESENTATION_ITEM('')
SURFACE()
);
#1605=(
BOUNDED_SURFACE()
B_SPLINE_SURFACE(3,2,((#43115,#43116,#43117),(#43118,#43119,#43120),(#43121,
#43122,#43123),(#43124,#43125,#43126),(#43127,#43128,#43129),(#43130,#43131,
#43132)),.UNSPECIFIED.,.F.,.F.,.F.)
B_SPLINE_SURFACE_WITH_KNOTS((4,1,1,4),(3,3),(0.00211111585136037,0.00418032934692781,
0.00568380331161446,0.00925648951110398),(-0.00558429959324884,1.05817709439886),
 .UNSPECIFIED.)
GEOMETRIC_REPRESENTATION_ITEM()
RATIONAL_B_SPLINE_SURFACE(((1.00329060357544,0.688134171423838,1.03607436996445),
(1.00329116786007,0.688080691540763,1.03608055612821),(1.00328994720374,
0.688196378826951,1.03606717426467),(1.00328910968704,0.688275754186287,
1.03605799270062),(1.00329008190375,0.688183612679626,1.03606865095971),
(1.00328970654605,0.688219187077167,1.03606453597223)))
REPRESENTATION_ITEM('')
SURFACE()
);
#1606=(
BOUNDED_SURFACE()
B_SPLINE_SURFACE(3,2,((#43133,#43134,#43135),(#43136,#43137,#43138),(#43139,
#43140,#43141),(#43142,#43143,#43144),(#43145,#43146,#43147),(#43148,#43149,
#43150)),.UNSPECIFIED.,.F.,.F.,.F.)
B_SPLINE_SURFACE_WITH_KNOTS((4,1,1,4),(3,3),(0.00206989346412758,0.00402645380207103,
0.00544807632115799,0.00882626159430671),(-0.00595850905898064,1.01180195773527),
 .UNSPECIFIED.)
GEOMETRIC_REPRESENTATION_ITEM()
RATIONAL_B_SPLINE_SURFACE(((1.0035120861051,0.701789401008881,1.0069967612183),
(1.00351252080015,0.701752491130503,1.00699762721571),(1.00351163037285,
0.701828097151536,1.0069958533107),(1.00351087607069,0.701892144812239,
1.00699435059353),(1.00351171129339,0.70182122620348,1.0069960145202),(1.00351156571752,
0.701833587024572,1.00699572450464)))
REPRESENTATION_ITEM('')
SURFACE()
);
#1607=(
BOUNDED_SURFACE()
B_SPLINE_SURFACE(3,2,((#43172,#43173,#43174),(#43175,#43176,#43177),(#43178,
#43179,#43180),(#43181,#43182,#43183),(#43184,#43185,#43186),(#43187,#43188,
#43189)),.UNSPECIFIED.,.F.,.F.,.F.)
B_SPLINE_SURFACE_WITH_KNOTS((4,1,1,4),(3,3),(0.00579676790523706,0.00657748490359677,
0.0069060300593971,0.00735820154402503),(0.,1.01353017141622),
 .UNSPECIFIED.)
GEOMETRIC_REPRESENTATION_ITEM()
RATIONAL_B_SPLINE_SURFACE(((1.,0.699822260672061,1.00812291253688),(1.,
0.699895928175691,1.00812091906898),(1.,0.699649690014438,1.00812758235804),
(1.,0.69899042483752,1.00814542229975),(1.,0.699390436250587,1.00813459785377),
(1.,0.699218266641026,1.00813925682243)))
REPRESENTATION_ITEM('')
SURFACE()
);
#1608=(
BOUNDED_SURFACE()
B_SPLINE_SURFACE(3,2,((#43233,#43234,#43235),(#43236,#43237,#43238),(#43239,
#43240,#43241),(#43242,#43243,#43244),(#43245,#43246,#43247)),
 .UNSPECIFIED.,.F.,.F.,.F.)
B_SPLINE_SURFACE_WITH_KNOTS((4,1,4),(3,3),(0.00217494176891105,0.00539842225200163,
0.00863013951237006),(-0.00371571512923231,1.05640803844583),
 .UNSPECIFIED.)
GEOMETRIC_REPRESENTATION_ITEM()
RATIONAL_B_SPLINE_SURFACE(((1.00218484151612,0.689354498488246,1.03490916812134),
(1.00218506494712,0.689322730584858,1.03491273807833),(1.00218418879701,
0.689447303506582,1.03489873904391),(1.00218536490516,0.689280081900558,
1.03491753077638),(1.00218509616368,0.689318292146319,1.03491323685329)))
REPRESENTATION_ITEM('')
SURFACE()
);
#1609=(
BOUNDED_SURFACE()
B_SPLINE_SURFACE(3,2,((#43263,#43264,#43265),(#43266,#43267,#43268),(#43269,
#43270,#43271),(#43272,#43273,#43274),(#43275,#43276,#43277)),
 .UNSPECIFIED.,.F.,.F.,.F.)
B_SPLINE_SURFACE_WITH_KNOTS((4,1,4),(3,3),(0.00576650017740751,0.00655247885962792,
0.00733845477348281),(0.,1.05287365404843),.UNSPECIFIED.)
GEOMETRIC_REPRESENTATION_ITEM()
RATIONAL_B_SPLINE_SURFACE(((1.,0.68746170886739,1.03305008296447),(1.,0.687609668253521,
1.03303443665767),(1.,0.686759401653278,1.03312435006181),(1.,0.689240361632676,
1.0328619952225),(1.,0.688759740156979,1.03291281964977)))
REPRESENTATION_ITEM('')
SURFACE()
);
#1610=(
BOUNDED_SURFACE()
B_SPLINE_SURFACE(3,2,((#43292,#43293,#43294),(#43295,#43296,#43297),(#43298,
#43299,#43300),(#43301,#43302,#43303),(#43304,#43305,#43306)),
 .UNSPECIFIED.,.F.,.F.,.F.)
B_SPLINE_SURFACE_WITH_KNOTS((4,1,4),(3,3),(0.00213679191355045,0.00535178046044285,
0.00855851013636219),(-0.00508088630754948,1.05456301268146),
 .UNSPECIFIED.)
GEOMETRIC_REPRESENTATION_ITEM()
RATIONAL_B_SPLINE_SURFACE(((1.00299197946971,0.689418739054714,1.03371234749458),
(1.00299234361822,0.689380938761304,1.03371645056449),(1.00299073389702,
0.689548035241304,1.03369831291323),(1.00299192835185,0.689424045324576,
1.03371177152031),(1.00299162252656,0.689455791399116,1.03370832561152)))
REPRESENTATION_ITEM('')
SURFACE()
);
#1611=(
BOUNDED_SURFACE()
B_SPLINE_SURFACE(3,2,((#43307,#43308,#43309),(#43310,#43311,#43312),(#43313,
#43314,#43315),(#43316,#43317,#43318),(#43319,#43320,#43321)),
 .UNSPECIFIED.,.F.,.F.,.F.)
B_SPLINE_SURFACE_WITH_KNOTS((4,1,4),(3,3),(0.00206760785143967,0.00523238397297043,
0.00839715035804973),(-0.00490441686180068,1.01404629551803),
 .UNSPECIFIED.)
GEOMETRIC_REPRESENTATION_ITEM()
RATIONAL_B_SPLINE_SURFACE(((1.00288754135804,0.701463125129675,1.00834517917058),
(1.00288769200597,0.701447549954039,1.00834561455275),(1.00288651080142,
0.701569672227322,1.00834220079607),(1.00288740164171,0.70147757010922,
1.00834477538146),(1.00288728891469,0.701489224720478,1.00834444959317)))
REPRESENTATION_ITEM('')
SURFACE()
);
#1612=(
BOUNDED_SURFACE()
B_SPLINE_SURFACE(3,2,((#43361,#43362,#43363),(#43364,#43365,#43366),(#43367,
#43368,#43369),(#43370,#43371,#43372),(#43373,#43374,#43375)),
 .UNSPECIFIED.,.F.,.F.,.F.)
B_SPLINE_SURFACE_WITH_KNOTS((4,1,4),(3,3),(0.002170029345752,0.00533298360778802,
0.00849593060227173),(-0.00937893121976585,1.01422351742609),
 .UNSPECIFIED.)
GEOMETRIC_REPRESENTATION_ITEM()
RATIONAL_B_SPLINE_SURFACE(((1.00554607201155,0.700088980780457,1.00845120436019),
(1.00554628250909,0.700077597854026,1.00845152512012),(1.00554458089537,
0.700169614817188,1.00844893217051),(1.00554685665382,0.700046550234841,
1.0084524000122),(1.00554656556966,0.700062290987494,1.00845195645291)))
REPRESENTATION_ITEM('')
SURFACE()
);
#1613=(
BOUNDED_SURFACE()
B_SPLINE_SURFACE(3,2,((#43389,#43390,#43391),(#43392,#43393,#43394),(#43395,
#43396,#43397),(#43398,#43399,#43400),(#43401,#43402,#43403)),
 .UNSPECIFIED.,.F.,.F.,.F.)
B_SPLINE_SURFACE_WITH_KNOTS((4,1,4),(3,3),(0.00219592593545592,0.00532324237200424,
0.00845896001036928),(-0.00320737611465728,1.04761084667385),
 .UNSPECIFIED.)
GEOMETRIC_REPRESENTATION_ITEM()
RATIONAL_B_SPLINE_SURFACE(((1.00188499121938,0.692112164947285,1.02921962346904),
(1.00188517626665,0.692081939977089,1.02922249192355),(1.00188445707106,
0.692199410855367,1.02921134352975),(1.00188535828696,0.692052209419153,
1.02922531345662),(1.00188512579573,0.69209018372002,1.02922170956375)))
REPRESENTATION_ITEM('')
SURFACE()
);
#1614=(
BOUNDED_SURFACE()
B_SPLINE_SURFACE(3,2,((#43430,#43431,#43432),(#43433,#43434,#43435),(#43436,
#43437,#43438),(#43439,#43440,#43441),(#43442,#43443,#43444)),
 .UNSPECIFIED.,.F.,.F.,.F.)
B_SPLINE_SURFACE_WITH_KNOTS((4,1,4),(3,3),(0.00211122737223723,0.00524610948281742,
0.00837256921945858),(-0.00425993730565382,1.04600237267559),
 .UNSPECIFIED.)
GEOMETRIC_REPRESENTATION_ITEM()
RATIONAL_B_SPLINE_SURFACE(((1.00250639350022,0.692227555543412,1.02819115126479),
(1.00250670366833,0.692189468469,1.02819463994123),(1.00250550329272,0.692336868521937,
1.02818113848175),(1.00250645781776,0.692219657675385,1.02819187468885),
(1.00250621151727,0.692249902129454,1.02818910437593)))
REPRESENTATION_ITEM('')
SURFACE()
);
#1615=(
BOUNDED_SURFACE()
B_SPLINE_SURFACE(3,2,((#43445,#43446,#43447),(#43448,#43449,#43450),(#43451,
#43452,#43453),(#43454,#43455,#43456),(#43457,#43458,#43459)),
 .UNSPECIFIED.,.F.,.F.,.F.)
B_SPLINE_SURFACE_WITH_KNOTS((4,1,4),(3,3),(0.006583329098368,0.00749456862587076,
0.00840580588587755),(-0.00374155041453272,1.03290826060198),
 .UNSPECIFIED.)
GEOMETRIC_REPRESENTATION_ITEM()
RATIONAL_B_SPLINE_SURFACE(((1.00222383231565,0.693003259388743,1.0201277491697),
(1.00222310392596,0.693103812501358,1.02012115656607),(1.00222748707377,
0.692498725470239,1.02016082812728),(1.00220858018415,0.695108793436242,
1.01998970320514),(1.00221230047744,0.694595212485627,1.02002337531687)))
REPRESENTATION_ITEM('')
SURFACE()
);
#1616=(
BOUNDED_SURFACE()
B_SPLINE_SURFACE(3,2,((#43490,#43491,#43492),(#43493,#43494,#43495),(#43496,
#43497,#43498),(#43499,#43500,#43501),(#43502,#43503,#43504)),
 .UNSPECIFIED.,.F.,.F.,.F.)
B_SPLINE_SURFACE_WITH_KNOTS((4,1,4),(3,3),(0.00227074891388854,0.00518182924437649,
0.00809291038442371),(-0.0057448981998482,1.00828145765618),
 .UNSPECIFIED.)
GEOMETRIC_REPRESENTATION_ITEM()
RATIONAL_B_SPLINE_SURFACE(((1.00338492186034,0.702943903419068,1.00489178136424),
(1.00338501455575,0.702935768597727,1.00489191532468),(1.00338425005556,
0.703002860084568,1.00489081049335),(1.00338494782254,0.702941625012127,
1.00489181888398),(1.00338502158477,0.702935151740146,1.00489192548281)))
REPRESENTATION_ITEM('')
SURFACE()
);
#1617=(
BOUNDED_SURFACE()
B_SPLINE_SURFACE(3,2,((#43550,#43551,#43552),(#43553,#43554,#43555),(#43556,
#43557,#43558),(#43559,#43560,#43561),(#43562,#43563,#43564)),
 .UNSPECIFIED.,.F.,.F.,.F.)
B_SPLINE_SURFACE_WITH_KNOTS((4,1,4),(3,3),(0.00345689067726456,0.00436603992331825,
0.00527519124507475),(-0.0036794560107073,1.03264354334434),
 .UNSPECIFIED.)
GEOMETRIC_REPRESENTATION_ITEM()
RATIONAL_B_SPLINE_SURFACE(((1.00217552367056,0.694683016928517,1.01985788040247),
(1.00217188868089,0.695193158047507,1.01982470071745),(1.00219036149319,
0.692600649680304,1.01999331800359),(1.00218608865275,0.693200307946796,
1.01995431610459),(1.00218679920266,0.693100588068842,1.0199608019063)))
REPRESENTATION_ITEM('')
SURFACE()
);
#1618=(
BOUNDED_SURFACE()
B_SPLINE_SURFACE(3,2,((#43565,#43566,#43567),(#43568,#43569,#43570),(#43571,
#43572,#43573),(#43574,#43575,#43576),(#43577,#43578,#43579)),
 .UNSPECIFIED.,.F.,.F.,.F.)
B_SPLINE_SURFACE_WITH_KNOTS((4,1,4),(3,3),(0.00222417800671133,0.00530805645561326,
0.00839192864935772),(-0.00406685372208074,1.04107360049962),
 .UNSPECIFIED.)
GEOMETRIC_REPRESENTATION_ITEM()
RATIONAL_B_SPLINE_SURFACE(((1.00239216177419,0.693766408819533,1.02505033698307),
(1.00239239865957,0.693736083838975,1.02505281760898),(1.00239149665043,
0.693851554916822,1.02504337191296),(1.00239258464149,0.693712275286194,
1.02505476518197),(1.00239228636051,0.693750459849733,1.02505164163115)))
REPRESENTATION_ITEM('')
SURFACE()
);
#1619=(
BOUNDED_SURFACE()
B_SPLINE_SURFACE(3,2,((#43654,#43655,#43656),(#43657,#43658,#43659),(#43660,
#43661,#43662),(#43663,#43664,#43665),(#43666,#43667,#43668)),
 .UNSPECIFIED.,.F.,.F.,.F.)
B_SPLINE_SURFACE_WITH_KNOTS((4,1,4),(3,3),(0.00211355742364673,0.00519233852776365,
0.00827111050613143),(-0.0051509153970441,1.00869647758464),
 .UNSPECIFIED.)
GEOMETRIC_REPRESENTATION_ITEM()
RATIONAL_B_SPLINE_SURFACE(((1.00303335472695,0.702978094692853,1.00513938789791),
(1.00303346790981,0.702967011983877,1.00513957966269),(1.00303238072114,
0.703073467997359,1.00513773764789),(1.00303327408742,0.702985990804776,
1.00513925127101),(1.00303316117799,0.702997046740221,1.0051390599695)))
REPRESENTATION_ITEM('')
SURFACE()
);
#1620=(
BOUNDED_SURFACE()
B_SPLINE_SURFACE(3,2,((#43683,#43684,#43685),(#43686,#43687,#43688),(#43689,
#43690,#43691),(#43692,#43693,#43694),(#43695,#43696,#43697)),
 .UNSPECIFIED.,.F.,.F.,.F.)
B_SPLINE_SURFACE_WITH_KNOTS((4,1,4),(3,3),(0.0022123564208203,0.00528826645871868,
0.00836416483792585),(-0.00574674248185728,1.00871944995166),
 .UNSPECIFIED.)
GEOMETRIC_REPRESENTATION_ITEM()
RATIONAL_B_SPLINE_SURFACE(((1.00338602967336,0.702812271509221,1.00515275950288),
(1.00338615667078,0.702801125099646,1.00515295276378),(1.00338515382689,
0.702889143494477,1.00515142666571),(1.00338636185634,0.702783116211503,
1.00515326500907),(1.00338623721726,0.702794055632565,1.00515307533702)))
REPRESENTATION_ITEM('')
SURFACE()
);
#1621=(
BOUNDED_SURFACE()
B_SPLINE_SURFACE(3,2,((#43698,#43699,#43700),(#43701,#43702,#43703),(#43704,
#43705,#43706),(#43707,#43708,#43709),(#43710,#43711,#43712)),
 .UNSPECIFIED.,.F.,.F.,.F.)
B_SPLINE_SURFACE_WITH_KNOTS((4,1,4),(3,3),(0.00221964849955536,0.00530337508156829,
0.00838709540025036),(-0.00386775963484442,1.04349299216076),
 .UNSPECIFIED.)
GEOMETRIC_REPRESENTATION_ITEM()
RATIONAL_B_SPLINE_SURFACE(((1.00227460680574,0.693114664954495,1.02658760232749),
(1.00227483592651,0.693083752445582,1.02659028049226),(1.00227396352775,
0.693201454716058,1.02658008312926),(1.00227500636979,0.693060756584338,
1.02659227278301),(1.00227472193803,0.693099131539325,1.02658894809484)))
REPRESENTATION_ITEM('')
SURFACE()
);
#1622=(
BOUNDED_SURFACE()
B_SPLINE_SURFACE(3,2,((#43742,#43743,#43744),(#43745,#43746,#43747),(#43748,
#43749,#43750),(#43751,#43752,#43753),(#43754,#43755,#43756)),
 .UNSPECIFIED.,.F.,.F.,.F.)
B_SPLINE_SURFACE_WITH_KNOTS((4,1,4),(3,3),(0.00213713482294571,0.00521861296289499,
0.00830007897582003),(-0.004774040707985,1.04045105083211),
 .UNSPECIFIED.)
GEOMETRIC_REPRESENTATION_ITEM()
RATIONAL_B_SPLINE_SURFACE(((1.00281025847898,0.693710559793116,1.02465716856158),
(1.00281060986467,0.693672262345152,1.02466025161475),(1.0028093248937,
0.693812311042481,1.02464897729744),(1.00281040793758,0.693694270333668,
1.02465847990926),(1.00281012318337,0.69372530563075,1.02465598147983)))
REPRESENTATION_ITEM('')
SURFACE()
);
#1623=(
BOUNDED_SURFACE()
B_SPLINE_SURFACE(3,2,((#43803,#43804,#43805),(#43806,#43807,#43808),(#43809,
#43810,#43811),(#43812,#43813,#43814),(#43815,#43816,#43817)),
 .UNSPECIFIED.,.F.,.F.,.F.)
B_SPLINE_SURFACE_WITH_KNOTS((4,1,4),(3,3),(0.0021088933074858,0.00518762498109073,
0.00826634651087212),(-0.00504323689701123,1.00761456883791),
 .UNSPECIFIED.)
GEOMETRIC_REPRESENTATION_ITEM()
RATIONAL_B_SPLINE_SURFACE(((1.00296962652022,0.703330175196368,1.00449518400848),
(1.00296973954876,0.703318883488138,1.00449535510207),(1.00296866453602,
0.703426278757948,1.00449372783344),(1.00296955720505,0.703337099878823,
1.00449507908469),(1.00296944388406,0.703348420802902,1.00449490754841)))
REPRESENTATION_ITEM('')
SURFACE()
);
#1624=(
BOUNDED_SURFACE()
B_SPLINE_SURFACE(3,2,((#43832,#43833,#43834),(#43835,#43836,#43837),(#43838,
#43839,#43840),(#43841,#43842,#43843),(#43844,#43845,#43846)),
 .UNSPECIFIED.,.F.,.F.,.F.)
B_SPLINE_SURFACE_WITH_KNOTS((4,1,4),(3,3),(0.00220768902546015,0.00528378993761675,
0.00835987926008497),(-0.00604801792390039,1.00690079957375),
 .UNSPECIFIED.)
GEOMETRIC_REPRESENTATION_ITEM()
RATIONAL_B_SPLINE_SURFACE(((1.0035646205897,0.703260866096649,1.00407068626359),
(1.00356475777255,0.703249446222167,1.00407084292215),(1.00356368106794,
0.703339077189256,1.00406961335886),(1.00356496531083,0.703232169564474,
1.00407107992444),(1.00356483141439,0.70324331585921,1.00407092701886)))
REPRESENTATION_ITEM('')
SURFACE()
);
#1625=(
BOUNDED_SURFACE()
B_SPLINE_SURFACE(3,2,((#43847,#43848,#43849),(#43850,#43851,#43852),(#43853,
#43854,#43855),(#43856,#43857,#43858),(#43859,#43860,#43861)),
 .UNSPECIFIED.,.F.,.F.,.F.)
B_SPLINE_SURFACE_WITH_KNOTS((4,1,4),(3,3),(0.00222405182330376,0.00529888890448264,
0.00838256300938198),(0.,1.04068598403832),.UNSPECIFIED.)
GEOMETRIC_REPRESENTATION_ITEM()
RATIONAL_B_SPLINE_SURFACE(((1.,0.695167345048307,1.02480483306745),(1.,
0.695136783885436,1.02480731988941),(1.,0.695255069647583,1.02479769474415),
(1.,0.695114492118214,1.02480913381439),(1.,0.695152707362112,1.02480602416478)))
REPRESENTATION_ITEM('')
SURFACE()
);
#1626=(
BOUNDED_SURFACE()
B_SPLINE_SURFACE(3,2,((#43891,#43892,#43893),(#43894,#43895,#43896),(#43897,
#43898,#43899),(#43900,#43901,#43902),(#43903,#43904,#43905)),
 .UNSPECIFIED.,.F.,.F.,.F.)
B_SPLINE_SURFACE_WITH_KNOTS((4,1,4),(3,3),(0.00213250098277698,0.00521408838432189,
0.00829566364757425),(-0.00540301929015671,1.03776088171629),
 .UNSPECIFIED.)
GEOMETRIC_REPRESENTATION_ITEM()
RATIONAL_B_SPLINE_SURFACE(((1.00318250272087,0.694307713339714,1.02295786527358),
(1.00318290152577,0.694269406511714,1.02296074216329),(1.00318143614362,
0.694410162408009,1.02295017122302),(1.00318268085919,0.694290602431972,
1.02295915032371),(1.00318235429806,0.694321969951759,1.02295679458454)))
REPRESENTATION_ITEM('')
SURFACE()
);
#1627=(
BOUNDED_SURFACE()
B_SPLINE_SURFACE(3,2,((#43951,#43952,#43953),(#43954,#43955,#43956),(#43957,
#43958,#43959),(#43960,#43961,#43962),(#43963,#43964,#43965)),
 .UNSPECIFIED.,.F.,.F.,.F.)
B_SPLINE_SURFACE_WITH_KNOTS((4,1,4),(3,3),(0.00218672559995519,0.00518296150941844,
0.00817918722256176),(-0.00482832253702671,1.00621350692926),
 .UNSPECIFIED.)
GEOMETRIC_REPRESENTATION_ITEM()
RATIONAL_B_SPLINE_SURFACE(((1.00284247866485,0.703807557313486,1.00366299226778),
(1.00284255386132,0.7037997216781,1.00366308917056),(1.00284156785576,0.703902465596022,
1.00366181854335),(1.00284239085209,0.703816707593733,1.00366287910687),
(1.00284231050323,0.703825080118213,1.00366277556442)))
REPRESENTATION_ITEM('')
SURFACE()
);
#1628=(
BOUNDED_SURFACE()
B_SPLINE_SURFACE(3,2,((#43980,#43981,#43982),(#43983,#43984,#43985),(#43986,
#43987,#43988),(#43989,#43990,#43991),(#43992,#43993,#43994)),
 .UNSPECIFIED.,.F.,.F.,.F.)
B_SPLINE_SURFACE_WITH_KNOTS((4,1,4),(3,3),(0.00236713033829012,0.00527934748302146,
0.00819155303031432),(0.,1.00557059275432),.UNSPECIFIED.)
GEOMETRIC_REPRESENTATION_ITEM()
RATIONAL_B_SPLINE_SURFACE(((1.,0.705444427620648,1.00328169827448),(1.,
0.705438897999593,1.00328175988101),(1.,0.705519693531559,1.003280859723),
(1.,0.705423279098818,1.00328193389409),(1.,0.70542771532932,1.00328188446922)))
REPRESENTATION_ITEM('')
SURFACE()
);
#1629=(
BOUNDED_SURFACE()
B_SPLINE_SURFACE(3,2,((#43995,#43996,#43997),(#43998,#43999,#44000),(#44001,
#44002,#44003),(#44004,#44005,#44006),(#44007,#44008,#44009)),
 .UNSPECIFIED.,.F.,.F.,.F.)
B_SPLINE_SURFACE_WITH_KNOTS((4,1,4),(3,3),(0.00221984090545246,0.0052945704827959,
0.00837825146220991),(0.,1.03829076028441),.UNSPECIFIED.)
GEOMETRIC_REPRESENTATION_ITEM()
RATIONAL_B_SPLINE_SURFACE(((1.,0.695868122289244,1.02329088164854),(1.,
0.69583719577093,1.02329325004834),(1.,0.695957181965263,1.02328406132313),
(1.,0.695815936027,1.02329487815185),(1.,0.69585416407111,1.02329195059011)))
REPRESENTATION_ITEM('')
SURFACE()
);
#1630=(
BOUNDED_SURFACE()
B_SPLINE_SURFACE(3,2,((#44039,#44040,#44041),(#44042,#44043,#44044),(#44045,
#44046,#44047),(#44048,#44049,#44050),(#44051,#44052,#44053)),
 .UNSPECIFIED.,.F.,.F.,.F.)
B_SPLINE_SURFACE_WITH_KNOTS((4,1,4),(3,3),(0.00212794996907239,0.00520974641510763,
0.00829153071066992),(-0.00525793491290963,1.0362694004451),
 .UNSPECIFIED.)
GEOMETRIC_REPRESENTATION_ITEM()
RATIONAL_B_SPLINE_SURFACE(((1.00309659972907,0.69479472099637,1.02201939623592),
(1.00309698870907,0.694756382573413,1.02202216220684),(1.00309555288293,
0.694897899641948,1.02201195229036),(1.00309678377646,0.694776581022652,
1.0220207049658),(1.00309646159645,0.694808335543697,1.02201841399828)))
REPRESENTATION_ITEM('')
SURFACE()
);
#1631=(
BOUNDED_SURFACE()
B_SPLINE_SURFACE(3,2,((#44099,#44100,#44101),(#44102,#44103,#44104),(#44105,
#44106,#44107),(#44108,#44109,#44110),(#44111,#44112,#44113)),
 .UNSPECIFIED.,.F.,.F.,.F.)
B_SPLINE_SURFACE_WITH_KNOTS((4,1,4),(3,3),(0.00233053591587337,0.00517834652518091,
0.00802614698836607),(-7.3643504785873E-5,1.00515727646814),
 .UNSPECIFIED.)
GEOMETRIC_REPRESENTATION_ITEM()
RATIONAL_B_SPLINE_SURFACE(((1.00004314960779,0.705526245967311,1.00303714031107),
(1.00004314993106,0.705524039760155,1.00303716306543),(1.00004313623197,
0.705617528983217,1.00303619883726),(1.00004314767456,0.705539439208663,
1.00303700423876),(1.00004314716727,0.705542901193404,1.00303696853258)))
REPRESENTATION_ITEM('')
SURFACE()
);
#1632=(
BOUNDED_SURFACE()
B_SPLINE_SURFACE(3,2,((#44128,#44129,#44130),(#44131,#44132,#44133),(#44134,
#44135,#44136),(#44137,#44138,#44139),(#44140,#44141,#44142)),
 .UNSPECIFIED.,.F.,.F.,.F.)
B_SPLINE_SURFACE_WITH_KNOTS((4,1,4),(3,3),(0.0024368838680126,0.00527506449450404,
0.00811323354646179),(0.,1.0046118093486),.UNSPECIFIED.)
GEOMETRIC_REPRESENTATION_ITEM()
RATIONAL_B_SPLINE_SURFACE(((1.,0.705724192469964,1.00271428784047),(1.,
0.705720922940111,1.00271431799736),(1.,0.705798756048654,1.00271360009445),
(1.,0.705706251659519,1.00271445331966),(1.,0.705708115890236,1.00271443612471)))
REPRESENTATION_ITEM('')
SURFACE()
);
#1633=(
BOUNDED_SURFACE()
B_SPLINE_SURFACE(3,2,((#44143,#44144,#44145),(#44146,#44147,#44148),(#44149,
#44150,#44151),(#44152,#44153,#44154),(#44155,#44156,#44157)),
 .UNSPECIFIED.,.F.,.F.,.F.)
B_SPLINE_SURFACE_WITH_KNOTS((4,1,4),(3,3),(0.00216602181407597,0.0052489536371796,
0.0083318848142593),(-0.0444466707917243,1.0051340701333),.UNSPECIFIED.)
GEOMETRIC_REPRESENTATION_ITEM()
RATIONAL_B_SPLINE_SURFACE(((1.02719646592756,0.69241749798202,1.00302324092364),
(1.027199787454,0.69237993268158,1.00302361015451),(1.02718810626605,0.692512042825083,
1.00302231163853),(1.02719782769207,0.692402096902532,1.00302339230148),
(1.02719527830541,0.692430929572478,1.00302310890399)))
REPRESENTATION_ITEM('')
SURFACE()
);
#1634=(
BOUNDED_SURFACE()
B_SPLINE_SURFACE(3,2,((#44186,#44187,#44188),(#44189,#44190,#44191),(#44192,
#44193,#44194),(#44195,#44196,#44197),(#44198,#44199,#44200)),
 .UNSPECIFIED.,.F.,.F.,.F.)
B_SPLINE_SURFACE_WITH_KNOTS((4,1,4),(3,3),(0.00216545784130295,0.00524970120976066,
0.00833394389446095),(-0.0058777833286939,1.04293073295283),
 .UNSPECIFIED.)
GEOMETRIC_REPRESENTATION_ITEM()
RATIONAL_B_SPLINE_SURFACE(((1.00346373556471,0.692630283187857,1.02623068962352),
(1.00346415610398,0.692592964796872,1.02623387434562),(1.00346268565001,
0.692723451957841,1.02622273867404),(1.00346391422394,0.6926144290796,1.02623204260063),
(1.003463585266,0.692643620600768,1.0262295514192)))
REPRESENTATION_ITEM('')
SURFACE()
);
#1635=(
BOUNDED_SURFACE()
B_SPLINE_SURFACE(3,2,((#44248,#44249,#44250),(#44251,#44252,#44253),(#44254,
#44255,#44256),(#44257,#44258,#44259),(#44260,#44261,#44262)),
 .UNSPECIFIED.,.F.,.F.,.F.)
B_SPLINE_SURFACE_WITH_KNOTS((4,1,4),(3,3),(0.00213816488674072,0.00521583965643689,
0.00829351555392586),(-0.00552986428889216,1.01473434870462),
 .UNSPECIFIED.)
GEOMETRIC_REPRESENTATION_ITEM()
RATIONAL_B_SPLINE_SURFACE(((1.00325771456763,0.701079567892973,1.00875965270882),
(1.00325781626736,0.701070236158245,1.00875992616873),(1.00325673379108,
0.701169561703866,1.00875701550358),(1.00325763395525,0.701086964700353,
1.00875943595059),(1.0032575157888,0.701097807383465,1.00875911821339)))
REPRESENTATION_ITEM('')
SURFACE()
);
#1636=(
BOUNDED_SURFACE()
B_SPLINE_SURFACE(3,2,((#44276,#44277,#44278),(#44279,#44280,#44281),(#44282,
#44283,#44284),(#44285,#44286,#44287),(#44288,#44289,#44290)),
 .UNSPECIFIED.,.F.,.F.,.F.)
B_SPLINE_SURFACE_WITH_KNOTS((4,1,4),(3,3),(0.00213779274189611,0.00521727844313784,
0.00829676872894075),(-0.0154960333971323,1.00577171680884),
 .UNSPECIFIED.)
GEOMETRIC_REPRESENTATION_ITEM()
RATIONAL_B_SPLINE_SURFACE(((1.00921938543943,0.700781197642686,1.00340100781529),
(1.00921966265681,0.700772200443111,1.00340111008007),(1.00921664376362,
0.70087017981592,1.00339999641806),(1.00921913287023,0.700789394876286,
1.00340091464315),(1.00921882744111,0.700799307699139,1.00340080197112)))
REPRESENTATION_ITEM('')
SURFACE()
);
#1637=(
BOUNDED_SURFACE()
B_SPLINE_SURFACE(3,2,((#44291,#44292,#44293),(#44294,#44295,#44296),(#44297,
#44298,#44299),(#44300,#44301,#44302),(#44303,#44304,#44305)),
 .UNSPECIFIED.,.F.,.F.,.F.)
B_SPLINE_SURFACE_WITH_KNOTS((4,1,4),(3,3),(0.00221169983238519,0.0052855296342299,
0.0083684987093601),(-0.00324346846181243,1.03300158810162),
 .UNSPECIFIED.)
GEOMETRIC_REPRESENTATION_ITEM()
RATIONAL_B_SPLINE_SURFACE(((1.00190629916672,0.696403174620331,1.01997150835538),
(1.00190649735207,0.696371611661272,1.01997358466135),(1.00190572425457,
0.696494735014529,1.01996548523845),(1.00190662047827,0.696352002607635,
1.01997487460362),(1.00190637972075,0.69639034560195,1.01997235228663)))
REPRESENTATION_ITEM('')
SURFACE()
);
#1638=(
BOUNDED_SURFACE()
B_SPLINE_SURFACE(3,2,((#44336,#44337,#44338),(#44339,#44340,#44341),(#44342,
#44343,#44344),(#44345,#44346,#44347),(#44348,#44349,#44350)),
 .UNSPECIFIED.,.F.,.F.,.F.)
B_SPLINE_SURFACE_WITH_KNOTS((4,1,4),(3,3),(0.00211921303525452,0.00520188789026804,
0.00828455059289162),(-0.00497615288010077,1.03080289128597),
 .UNSPECIFIED.)
GEOMETRIC_REPRESENTATION_ITEM()
RATIONAL_B_SPLINE_SURFACE(((1.00292983108751,0.696499957967487,1.01860202496771),
(1.00293020100174,0.696461638698849,1.01860437361975),(1.00292882376335,
0.696604306277997,1.01859562928531),(1.00293002052061,0.696480334667596,
1.01860322771257),(1.00292970839583,0.696512667549343,1.01860124597619)))
REPRESENTATION_ITEM('')
SURFACE()
);
#1639=(
BOUNDED_SURFACE()
B_SPLINE_SURFACE(3,2,((#44398,#44399,#44400),(#44401,#44402,#44403),(#44404,
#44405,#44406),(#44407,#44408,#44409),(#44410,#44411,#44412)),
 .UNSPECIFIED.,.F.,.F.,.F.)
B_SPLINE_SURFACE_WITH_KNOTS((4,1,4),(3,3),(0.00247806168022139,0.00516920088530873,
0.00786033004716436),(0.,1.00372616184728),.UNSPECIFIED.)
GEOMETRIC_REPRESENTATION_ITEM()
RATIONAL_B_SPLINE_SURFACE(((1.,0.705967000528768,1.00219122908894),(1.,
0.70596966991393,1.00219120919582),(1.,0.706054739691718,1.0021905752283),
(1.,0.705982858434738,1.0021911109107),(0.999999999999999,0.705982071723989,
1.00219111677352)))
REPRESENTATION_ITEM('')
SURFACE()
);
#1640=(
BOUNDED_SURFACE()
B_SPLINE_SURFACE(3,2,((#44427,#44428,#44429),(#44430,#44431,#44432),(#44433,
#44434,#44435),(#44436,#44437,#44438),(#44439,#44440,#44441)),
 .UNSPECIFIED.,.F.,.F.,.F.)
B_SPLINE_SURFACE_WITH_KNOTS((4,1,4),(3,3),(0.00267720881073118,0.00526764836792767,
0.00785808792512416),(0.,1.00296333742759),.UNSPECIFIED.)
GEOMETRIC_REPRESENTATION_ITEM()
RATIONAL_B_SPLINE_SURFACE(((1.,0.706205515038292,1.00174122438661),(1.,
0.706208745150634,1.00174120524278),(1.,0.706275159085219,1.00174081162899),
(1.,0.706196462696256,1.0017412780369),(1.,0.706191126887914,1.0017413096605)))
REPRESENTATION_ITEM('')
SURFACE()
);
#1641=(
BOUNDED_SURFACE()
B_SPLINE_SURFACE(3,2,((#44442,#44443,#44444),(#44445,#44446,#44447),(#44448,
#44449,#44450),(#44451,#44452,#44453),(#44454,#44455,#44456),(#44457,#44458,
#44459)),.UNSPECIFIED.,.F.,.F.,.F.)
B_SPLINE_SURFACE_WITH_KNOTS((4,1,1,4),(3,3),(0.00207740162366139,0.00585323454960992,
0.00744219878966224,0.00962906509384405),(-0.00992421051928284,1.06115213291247),
 .UNSPECIFIED.)
GEOMETRIC_REPRESENTATION_ITEM()
RATIONAL_B_SPLINE_SURFACE(((1.00587156388292,0.685911998576704,1.03801528924904),
(1.00587229355607,0.685872966116927,1.03802001349906),(1.00587030000394,
0.685979607348392,1.03800710629713),(1.00587241313185,0.685866569640664,
1.0380207876894),(1.00587464193811,0.685747343942645,1.03803521803814),
(1.00587381122293,0.685791781451287,1.03802983959408)))
REPRESENTATION_ITEM('')
SURFACE()
);
#1642=(
BOUNDED_SURFACE()
B_SPLINE_SURFACE(3,2,((#44487,#44488,#44489),(#44490,#44491,#44492),(#44493,
#44494,#44495),(#44496,#44497,#44498),(#44499,#44500,#44501),(#44502,#44503,
#44504)),.UNSPECIFIED.,.F.,.F.,.F.)
B_SPLINE_SURFACE_WITH_KNOTS((4,1,1,4),(3,3),(0.00207839781632833,0.00584816658647622,
0.00743457891160079,0.00961793307792553),(-0.0645166657950686,1.00997111844977),
 .UNSPECIFIED.)
GEOMETRIC_REPRESENTATION_ITEM()
RATIONAL_B_SPLINE_SURFACE(((1.04023391045298,0.684892260072604,1.00589957457065),
(1.0402390319118,0.684852149347703,1.00590032553987),(1.04022544444458,
0.684958564956782,1.00589833318379),(1.04023976549679,0.684846403987535,
1.00590043310683),(1.04025602169469,0.684719087161401,1.00590281678395),
(1.04024986609632,0.684767297158138,1.00590191417689)))
REPRESENTATION_ITEM('')
SURFACE()
);
#1643=(
BOUNDED_SURFACE()
B_SPLINE_SURFACE(3,2,((#44565,#44566,#44567),(#44568,#44569,#44570),(#44571,
#44572,#44573),(#44574,#44575,#44576),(#44577,#44578,#44579),(#44580,#44581,
#44582)),.UNSPECIFIED.,.F.,.F.,.F.)
B_SPLINE_SURFACE_WITH_KNOTS((4,1,1,4),(3,3),(0.00206507808144807,0.00583603875252445,
0.00742295148565546,0.00960699434655795),(-0.0135229107749584,1.00542045039503),
 .UNSPECIFIED.)
GEOMETRIC_REPRESENTATION_ITEM()
RATIONAL_B_SPLINE_SURFACE(((1.00802943361181,0.701486699145671,1.00319274510453),
(1.00802983521136,0.701471768726875,1.00319290479263),(1.00802754903546,
0.701556762755815,1.00319199574011),(1.0080303645787,0.701452088236144,
1.00319311528506),(1.00803378849418,0.701324796030788,1.00319447673718),
(1.00803171445255,0.701401903463793,1.00319365203564)))
REPRESENTATION_ITEM('')
SURFACE()
);
#1644=(
BOUNDED_SURFACE()
B_SPLINE_SURFACE(3,2,((#44596,#44597,#44598),(#44599,#44600,#44601),(#44602,
#44603,#44604),(#44605,#44606,#44607),(#44608,#44609,#44610),(#44611,#44612,
#44613)),.UNSPECIFIED.,.F.,.F.,.F.)
B_SPLINE_SURFACE_WITH_KNOTS((4,1,1,4),(3,3),(0.00206606642132582,0.0058308811139682,
0.00741520747929493,0.00959569080576064),(-0.00535992176287023,1.01476618027226),
 .UNSPECIFIED.)
GEOMETRIC_REPRESENTATION_ITEM()
RATIONAL_B_SPLINE_SURFACE(((1.00315690508187,0.70113658592927,1.00877840586715),
(1.00315704437056,0.701123399504209,1.0087787931872),(1.00315616753589,
0.701206409222792,1.00877635497306),(1.00315726922125,0.701102112945542,
1.00877941842951),(1.00315868258643,0.700968310017838,1.00878334857402),
(1.00315783740284,0.701048323336468,1.00878099837204)))
REPRESENTATION_ITEM('')
SURFACE()
);
#1645=(
BOUNDED_SURFACE()
B_SPLINE_SURFACE(3,2,((#44614,#44615,#44616),(#44617,#44618,#44619),(#44620,
#44621,#44622),(#44623,#44624,#44625),(#44626,#44627,#44628)),
 .UNSPECIFIED.,.F.,.F.,.F.)
B_SPLINE_SURFACE_WITH_KNOTS((4,1,4),(3,3),(0.00221567299324823,0.00529019818489015,
0.00837376654817291),(-0.00338061827446617,1.03561415616917),
 .UNSPECIFIED.)
GEOMETRIC_REPRESENTATION_ITEM()
RATIONAL_B_SPLINE_SURFACE(((1.00198717354311,0.695590668589538,1.02160700592179),
(1.00198737798433,0.695559350832966,1.0216092288594),(1.00198658295342,
0.695681139303956,1.0216005843011),(1.00198751198972,0.695538822937044,
1.02161068593159),(1.00198726154498,0.695577187837766,1.02160796278695)))
REPRESENTATION_ITEM('')
SURFACE()
);
#1646=(
BOUNDED_SURFACE()
B_SPLINE_SURFACE(3,2,((#44658,#44659,#44660),(#44661,#44662,#44663),(#44664,
#44665,#44666),(#44667,#44668,#44669),(#44670,#44671,#44672)),
 .UNSPECIFIED.,.F.,.F.,.F.)
B_SPLINE_SURFACE_WITH_KNOTS((4,1,4),(3,3),(0.00212352061007265,0.00520567904197513,
0.00828782532148532),(-0.00509675325938166,1.03341354675208),
 .UNSPECIFIED.)
GEOMETRIC_REPRESENTATION_ITEM()
RATIONAL_B_SPLINE_SURFACE(((1.00300119491187,0.695690193929004,1.02022970033526),
(1.00300157279743,0.69565187776315,1.02023224749128),(1.00300017187814,
0.695793925677851,1.02022280452661),(1.0030013809653,0.695671328815938,
1.02023095443742),(1.00300106502948,0.695703363512021,1.02022882485668)))
REPRESENTATION_ITEM('')
SURFACE()
);
#1647=(
BOUNDED_SURFACE()
B_SPLINE_SURFACE(3,2,((#44719,#44720,#44721),(#44722,#44723,#44724),(#44725,
#44726,#44727),(#44728,#44729,#44730),(#44731,#44732,#44733)),
 .UNSPECIFIED.,.F.,.F.,.F.)
B_SPLINE_SURFACE_WITH_KNOTS((4,1,4),(3,3),(0.00242089776087212,0.00517364817267956,
0.00792638848906705),(0.,1.00438630646283),.UNSPECIFIED.)
GEOMETRIC_REPRESENTATION_ITEM()
RATIONAL_B_SPLINE_SURFACE(((0.999999999999999,0.705773647857135,1.00258113389988),
(1.,0.705774512519574,1.00258112631453),(1.,0.705862755339751,1.00258035219442),
(1.,0.705788773568408,1.00258100120787),(1.,0.705789544485571,1.00258099444491)))
REPRESENTATION_ITEM('')
SURFACE()
);
#1648=(
BOUNDED_SURFACE()
B_SPLINE_SURFACE(3,2,((#44748,#44749,#44750),(#44751,#44752,#44753),(#44754,
#44755,#44756),(#44757,#44758,#44759),(#44760,#44761,#44762)),
 .UNSPECIFIED.,.F.,.F.,.F.)
B_SPLINE_SURFACE_WITH_KNOTS((4,1,4),(3,3),(0.00243077395143883,0.00527113010473627,
0.00811147475653914),(0.,1.0038266298341),.UNSPECIFIED.)
GEOMETRIC_REPRESENTATION_ITEM()
RATIONAL_B_SPLINE_SURFACE(((0.999999999999999,0.705953422236314,1.00225041481417),
(1.,0.705950011646756,1.0022504409163),(1.,0.706029253698611,1.0022498344563),
(1.,0.705935850122719,1.00225054929812),(1.,0.705937868958441,1.00225053384744)))
REPRESENTATION_ITEM('')
SURFACE()
);
#1649=(
BOUNDED_SURFACE()
B_SPLINE_SURFACE(3,2,((#44763,#44764,#44765),(#44766,#44767,#44768),(#44769,
#44770,#44771),(#44772,#44773,#44774),(#44775,#44776,#44777)),
 .UNSPECIFIED.,.F.,.F.,.F.)
B_SPLINE_SURFACE_WITH_KNOTS((4,1,4),(3,3),(0.00214655059911542,0.00523053798972514,
0.00831451824855835),(-0.0445562277105792,1.00427533437828),
 .UNSPECIFIED.)
GEOMETRIC_REPRESENTATION_ITEM()
RATIONAL_B_SPLINE_SURFACE(((1.02726668218841,0.692655434185802,1.00251544567194),
(1.0272700833989,0.692617096424234,1.00251575944537),(1.02725773849294,
0.692756245725015,1.00251462058513),(1.02726782460646,0.692642557079007,
1.00251555106396),(1.02726517368982,0.692672437679016,1.00251530650774)))
REPRESENTATION_ITEM('')
SURFACE()
);
#1650=(
BOUNDED_SURFACE()
B_SPLINE_SURFACE(3,2,((#44881,#44882,#44883),(#44884,#44885,#44886),(#44887,
#44888,#44889),(#44890,#44891,#44892),(#44893,#44894,#44895)),
 .UNSPECIFIED.,.F.,.F.,.F.)
B_SPLINE_SURFACE_WITH_KNOTS((4,1,4),(3,3),(0.00211840448974134,0.00519733850462133,
0.00827626876039074),(-0.00531044220281859,1.01360741147715),
 .UNSPECIFIED.)
GEOMETRIC_REPRESENTATION_ITEM()
RATIONAL_B_SPLINE_SURFACE(((1.00312779985738,0.701476278137035,1.0080807816251),
(1.00312791614054,0.701465179830938,1.00808108204675),(1.00312679729283,
0.701571964982313,1.00807819146411),(1.00312769672486,0.701486121319756,
1.00808051517857),(1.00312758346358,0.701496931211594,1.00808022256405)))
REPRESENTATION_ITEM('')
SURFACE()
);
#1651=(
BOUNDED_SURFACE()
B_SPLINE_SURFACE(3,2,((#44909,#44910,#44911),(#44912,#44913,#44914),(#44915,
#44916,#44917),(#44918,#44919,#44920),(#44921,#44922,#44923)),
 .UNSPECIFIED.,.F.,.F.,.F.)
B_SPLINE_SURFACE_WITH_KNOTS((4,1,4),(3,3),(0.00211874843791123,0.00519509076672421,
0.00827143358138237),(-0.0125740566466983,1.00548824263856),
 .UNSPECIFIED.)
GEOMETRIC_REPRESENTATION_ITEM()
RATIONAL_B_SPLINE_SURFACE(((1.00745949944159,0.701729219975106,1.0032330898743),
(1.00745977129585,0.701718349784357,1.00323320770114),(1.00745712020765,
0.701824354503976,1.00323205866876),(1.00745927654141,0.701738132719556,
1.0032329932651),(1.00745900509947,0.701748986423287,1.00323287561697)))
REPRESENTATION_ITEM('')
SURFACE()
);
#1652=(
BOUNDED_SURFACE()
B_SPLINE_SURFACE(3,2,((#44924,#44925,#44926),(#44927,#44928,#44929),(#44930,
#44931,#44932),(#44933,#44934,#44935),(#44936,#44937,#44938)),
 .UNSPECIFIED.,.F.,.F.,.F.)
B_SPLINE_SURFACE_WITH_KNOTS((4,1,4),(3,3),(0.00215123432211629,0.00523490276681949,
0.00831856581076139),(-0.0446521768288519,1.00447160747577),
 .UNSPECIFIED.)
GEOMETRIC_REPRESENTATION_ITEM()
RATIONAL_B_SPLINE_SURFACE(((1.02732782824787,0.692565371325594,1.00263143174123),
(1.02733121531728,0.692527267220997,1.0026317578865),(1.02731901536931,
0.692664515100408,1.00263058313781),(1.02732901642887,0.692552004438952,
1.0026315461527),(1.02732639440196,0.692581501911628,1.00263129367436)))
REPRESENTATION_ITEM('')
SURFACE()
);
#1653=(
BOUNDED_SURFACE()
B_SPLINE_SURFACE(3,2,((#45042,#45043,#45044),(#45045,#45046,#45047),(#45048,
#45049,#45050),(#45051,#45052,#45053),(#45054,#45055,#45056)),
 .UNSPECIFIED.,.F.,.F.,.F.)
B_SPLINE_SURFACE_WITH_KNOTS((4,1,4),(3,3),(0.00212311714528586,0.00520198579321628,
0.00828085288284644),(-0.00537925943683262,1.01436188121935),
 .UNSPECIFIED.)
GEOMETRIC_REPRESENTATION_ITEM()
RATIONAL_B_SPLINE_SURFACE(((1.00316854084855,0.701232988150657,1.0085351498297),
(1.00316865374682,0.701222342783812,1.00853545394561),(1.00316754232714,
0.701327140403275,1.00853246009639),(1.00316844120367,0.701242383832614,
1.00853488141468),(1.00316832736094,0.701253118254473,1.00853457475466)))
REPRESENTATION_ITEM('')
SURFACE()
);
#1654=(
BOUNDED_SURFACE()
B_SPLINE_SURFACE(3,2,((#45070,#45071,#45072),(#45073,#45074,#45075),(#45076,
#45077,#45078),(#45079,#45080,#45081),(#45082,#45083,#45084)),
 .UNSPECIFIED.,.F.,.F.,.F.)
B_SPLINE_SURFACE_WITH_KNOTS((4,1,4),(3,3),(0.00212330681955807,0.00520007589671178,
0.00827684772276528),(-0.0121951366433616,1.00556207700585),
 .UNSPECIFIED.)
GEOMETRIC_REPRESENTATION_ITEM()
RATIONAL_B_SPLINE_SURFACE(((1.00723196921242,0.701820535877395,1.00327681207336),
(1.0072322169053,0.701810323315722,1.00327692430324),(1.00722971878562,
0.701913322646367,1.00327579240285),(1.00723177777283,0.701828429073946,
1.0032767253319),(1.00723151977724,0.701839066423805,1.00327660843385)))
REPRESENTATION_ITEM('')
SURFACE()
);
#1655=(
BOUNDED_SURFACE()
B_SPLINE_SURFACE(3,2,((#45085,#45086,#45087),(#45088,#45089,#45090),(#45091,
#45092,#45093),(#45094,#45095,#45096),(#45097,#45098,#45099)),
 .UNSPECIFIED.,.F.,.F.,.F.)
B_SPLINE_SURFACE_WITH_KNOTS((4,1,4),(3,3),(0.00215603338555798,0.00523933845636758,
0.0083226405745289),(-0.0447685632758762,1.00467765051002),
 .UNSPECIFIED.)
GEOMETRIC_REPRESENTATION_ITEM()
RATIONAL_B_SPLINE_SURFACE(((1.02740202841322,0.692466142220858,1.00275323936646),
(1.02740540355604,0.692428262883068,1.00275357848647),(1.02739334485071,
0.692563598125863,1.002752366879),(1.02740326485242,0.692452265623459,1.00275336359862),
(1.02740066994345,0.692481388371397,1.00275310287319)))
REPRESENTATION_ITEM('')
SURFACE()
);
#1656=(
BOUNDED_SURFACE()
B_SPLINE_SURFACE(3,2,((#45128,#45129,#45130),(#45131,#45132,#45133),(#45134,
#45135,#45136),(#45137,#45138,#45139),(#45140,#45141,#45142)),
 .UNSPECIFIED.,.F.,.F.,.F.)
B_SPLINE_SURFACE_WITH_KNOTS((4,1,4),(3,3),(0.002156044127766,0.00523919183544554,
0.00832233675413979),(-0.00548162111442793,1.0454477898263),
 .UNSPECIFIED.)
GEOMETRIC_REPRESENTATION_ITEM()
RATIONAL_B_SPLINE_SURFACE(((1.00322903191596,0.692008598862286,1.02783583820613),
(1.00322943091132,0.691970541901698,1.02783927774176),(1.00322800638677,
0.692106415848783,1.02782699764175),(1.00322918942026,0.691993575792936,
1.02783719597043),(1.00322887542929,0.69202352486771,1.02783448921434)))
REPRESENTATION_ITEM('')
SURFACE()
);
#1657=(
BOUNDED_SURFACE()
B_SPLINE_SURFACE(3,2,((#45190,#45191,#45192),(#45193,#45194,#45195),(#45196,
#45197,#45198),(#45199,#45200,#45201),(#45202,#45203,#45204)),
 .UNSPECIFIED.,.F.,.F.,.F.)
B_SPLINE_SURFACE_WITH_KNOTS((4,1,4),(3,3),(0.00212802408085649,0.00520645763078059,
0.00828489231196136),(-0.00544652756431799,1.01484739119941),
 .UNSPECIFIED.)
GEOMETRIC_REPRESENTATION_ITEM()
RATIONAL_B_SPLINE_SURFACE(((1.00320837001835,0.701069722901491,1.00882788477518),
(1.00320847966809,0.701059506614525,1.00882818647832),(1.00320737445807,
0.701162481251729,1.00882514547411),(1.0032082761041,0.701078473080572,
1.00882762636853),(1.00320816004395,0.701089286637446,1.00882730702706)))
REPRESENTATION_ITEM('')
SURFACE()
);
#1658=(
BOUNDED_SURFACE()
B_SPLINE_SURFACE(3,2,((#45218,#45219,#45220),(#45221,#45222,#45223),(#45224,
#45225,#45226),(#45227,#45228,#45229),(#45230,#45231,#45232)),
 .UNSPECIFIED.,.F.,.F.,.F.)
B_SPLINE_SURFACE_WITH_KNOTS((4,1,4),(3,3),(0.00212780620908921,0.00520535309141684,
0.00828290460668537),(-0.0123335526006055,1.00564508813243),
 .UNSPECIFIED.)
GEOMETRIC_REPRESENTATION_ITEM()
RATIONAL_B_SPLINE_SURFACE(((1.00731501770778,0.701756056773149,1.00332597532949),
(1.00731524864014,0.701746641323926,1.00332608032928),(1.00731281032856,
0.701846054844198,1.00332497168341),(1.00731484685567,0.701763022662945,
1.00332589764685),(1.00731459376117,0.701773341694953,1.00332578257042)))
REPRESENTATION_ITEM('')
SURFACE()
);
#1659=(
BOUNDED_SURFACE()
B_SPLINE_SURFACE(3,2,((#45233,#45234,#45235),(#45236,#45237,#45238),(#45239,
#45240,#45241),(#45242,#45243,#45244),(#45245,#45246,#45247)),
 .UNSPECIFIED.,.F.,.F.,.F.)
B_SPLINE_SURFACE_WITH_KNOTS((4,1,4),(3,3),(0.00216103530262931,0.00524384440588618,
0.00832665287687961),(-0.0446064778924999,1.0048995043461),
 .UNSPECIFIED.)
GEOMETRIC_REPRESENTATION_ITEM()
RATIONAL_B_SPLINE_SURFACE(((1.02729850625157,0.692444146963455,1.00288445000016),
(1.02730185345113,0.692406436078964,1.00288480367628),(1.02728998621801,
0.692540137057693,1.00288354974538),(1.02729979876591,0.692429584981676,
1.00288458657148),(1.02729723696384,0.692458447264937,1.00288431588304)))
REPRESENTATION_ITEM('')
SURFACE()
);
#1660=(
BOUNDED_SURFACE()
B_SPLINE_SURFACE(3,2,((#45276,#45277,#45278),(#45279,#45280,#45281),(#45282,
#45283,#45284),(#45285,#45286,#45287),(#45288,#45289,#45290)),
 .UNSPECIFIED.,.F.,.F.,.F.)
B_SPLINE_SURFACE_WITH_KNOTS((4,1,4),(3,3),(0.00216084865593138,0.0052451443109893,
0.00832943934876088),(-0.00568511307436906,1.04556686179785),
 .UNSPECIFIED.)
GEOMETRIC_REPRESENTATION_ITEM()
RATIONAL_B_SPLINE_SURFACE(((1.00334957403885,0.691908816802213,1.02791189889522),
(1.00334998689027,0.691870843054131,1.02791533917354),(1.00334852263475,
0.692005524123632,1.02790313757674),(1.00334973592382,0.691893926750258,
1.02791324787776),(1.00334941299497,0.691923629491969,1.02791055692142)))
REPRESENTATION_ITEM('')
SURFACE()
);
#1661=(
BOUNDED_SURFACE()
B_SPLINE_SURFACE(3,2,((#45333,#45334,#45335),(#45336,#45337,#45338),(#45339,
#45340,#45341),(#45342,#45343,#45344),(#45345,#45346,#45347)),
 .UNSPECIFIED.,.F.,.F.,.F.)
B_SPLINE_SURFACE_WITH_KNOTS((4,1,4),(3,3),(0.00213302336063595,0.00521101927613581,
0.00828901632118316),(-0.00549073681840203,1.0147633501061),
 .UNSPECIFIED.)
GEOMETRIC_REPRESENTATION_ITEM()
RATIONAL_B_SPLINE_SURFACE(((1.00323454601582,0.701082056419879,1.00877716625763),
(1.00323465179662,0.701072280773333,1.00877745330121),(1.0032335573809,
0.7011734203137,1.0087744835278),(1.00323445964151,0.701090038631704,1.00877693187492),
(1.0032343417967,0.701100929163706,1.00877661209481)))
REPRESENTATION_ITEM('')
SURFACE()
);
#1662=(
BOUNDED_SURFACE()
B_SPLINE_SURFACE(3,2,((#45362,#45363,#45364),(#45365,#45366,#45367),(#45368,
#45369,#45370),(#45371,#45372,#45373),(#45374,#45375,#45376)),
 .UNSPECIFIED.,.F.,.F.,.F.)
B_SPLINE_SURFACE_WITH_KNOTS((4,1,4),(3,3),(0.00213312433381201,0.00521163967845316,
0.00829016000657247),(-0.0156178445535448,1.00571793255727),
 .UNSPECIFIED.)
GEOMETRIC_REPRESENTATION_ITEM()
RATIONAL_B_SPLINE_SURFACE(((1.00929301133279,0.700760075002523,1.00336914940697),
(1.00929331665074,0.70075024360155,1.00336926009895),(1.00929015613772,
0.700852013807781,1.00336811426578),(1.00929275637582,0.70076828475314,
1.0033690569732),(1.00929243233675,0.700778718984092,1.00336893949394)))
REPRESENTATION_ITEM('')
SURFACE()
);
#1663=(
BOUNDED_SURFACE()
B_SPLINE_SURFACE(3,2,((#45377,#45378,#45379),(#45380,#45381,#45382),(#45383,
#45384,#45385),(#45386,#45387,#45388),(#45389,#45390,#45391),(#45392,#45393,
#45394)),.UNSPECIFIED.,.F.,.F.,.F.)
B_SPLINE_SURFACE_WITH_KNOTS((4,1,1,4),(3,3),(0.00208139341848436,0.00585739462970524,
0.00744642968342663,0.0096333934474643),(-0.0100479807687911,1.06113579455401),
 .UNSPECIFIED.)
GEOMETRIC_REPRESENTATION_ITEM()
RATIONAL_B_SPLINE_SURFACE(((1.00594551440041,0.685876484175346,1.0380045120459),
(1.00594626072007,0.685837053347266,1.03800928261959),(1.00594424103948,
0.685943760542502,1.03799637255497),(1.00594637770504,0.685830872598689,
1.03801003040293),(1.00594862274388,0.68571225889319,1.03802438098725),
(1.0059477826065,0.685756646458221,1.03801901071834)))
REPRESENTATION_ITEM('')
SURFACE()
);
#1664=(
BOUNDED_SURFACE()
B_SPLINE_SURFACE(3,2,((#45422,#45423,#45424),(#45425,#45426,#45427),(#45428,
#45429,#45430),(#45431,#45432,#45433),(#45434,#45435,#45436),(#45437,#45438,
#45439)),.UNSPECIFIED.,.F.,.F.,.F.)
B_SPLINE_SURFACE_WITH_KNOTS((4,1,1,4),(3,3),(0.00208246989021945,0.00585173909416552,
0.00743794117493988,0.00962100597940954),(-0.0634120194467482,1.01004449590126),
 .UNSPECIFIED.)
GEOMETRIC_REPRESENTATION_ITEM()
RATIONAL_B_SPLINE_SURFACE(((1.03950397758292,0.685198194337763,1.00594341874322),
(1.03950901710132,0.68515803510341,1.00594417694454),(1.03949563649155,
0.685264663356425,1.00594216381645),(1.03950982841265,0.685151569874148,
1.00594429900726),(1.0395253903989,0.685027558529697,1.00594664032594),
(1.03951949311786,0.68507455315746,1.00594575307324)))
REPRESENTATION_ITEM('')
SURFACE()
);
#1665=(
BOUNDED_SURFACE()
B_SPLINE_SURFACE(3,2,((#45478,#45479,#45480),(#45481,#45482,#45483),(#45484,
#45485,#45486),(#45487,#45488,#45489),(#45490,#45491,#45492),(#45493,#45494,
#45495)),.UNSPECIFIED.,.F.,.F.,.F.)
B_SPLINE_SURFACE_WITH_KNOTS((4,1,1,4),(3,3),(0.00206902137639543,0.0058401154462197,
0.00742708429774716,0.00961120439636198),(-0.0133376601097449,1.00544905730155),
 .UNSPECIFIED.)
GEOMETRIC_REPRESENTATION_ITEM()
RATIONAL_B_SPLINE_SURFACE(((1.00791799171496,0.701532910309794,1.00320968682838),
(1.00791837853318,0.701518329275477,1.00320984363144),(1.0079161281519,
0.701603156941006,1.00320893140275),(1.00791891490684,0.701498110779302,
1.00321006105923),(1.00792225352701,0.701372262169953,1.00321141442326),
(1.00792022918322,0.70144856939801,1.00321059382256)))
REPRESENTATION_ITEM('')
SURFACE()
);
#1666=(
BOUNDED_SURFACE()
B_SPLINE_SURFACE(3,2,((#45510,#45511,#45512),(#45513,#45514,#45515),(#45516,
#45517,#45518),(#45519,#45520,#45521),(#45522,#45523,#45524),(#45525,#45526,
#45527)),.UNSPECIFIED.,.F.,.F.,.F.)
B_SPLINE_SURFACE_WITH_KNOTS((4,1,1,4),(3,3),(0.00206993025455239,0.00583529331732963,
0.00741985043665655,0.00960064723499827),(-0.00538361942335849,1.01460879274893),
 .UNSPECIFIED.)
GEOMETRIC_REPRESENTATION_ITEM()
RATIONAL_B_SPLINE_SURFACE(((1.00317093655876,0.701176112786129,1.00868349075652),
(1.00317107609581,0.701162963042384,1.00868387287349),(1.00317019729362,
0.70124577992633,1.00868146630669),(1.0031713020113,0.701141673135268,1.00868449153458),
(1.00317270302626,0.701009643771633,1.00868832816146),(1.00317186374986,
0.701088735810024,1.00868602983454)))
REPRESENTATION_ITEM('')
SURFACE()
);
#1667=(
BOUNDED_SURFACE()
B_SPLINE_SURFACE(3,2,((#45528,#45529,#45530),(#45531,#45532,#45533),(#45534,
#45535,#45536),(#45537,#45538,#45539),(#45540,#45541,#45542),(#45543,#45544,
#45545)),.UNSPECIFIED.,.F.,.F.,.F.)
B_SPLINE_SURFACE_WITH_KNOTS((4,1,1,4),(3,3),(0.00211869188141098,0.00569878884162654,
0.00720538255197427,0.00927888394959123),(-0.00871872596836085,1.05558447453005),
 .UNSPECIFIED.)
GEOMETRIC_REPRESENTATION_ITEM()
RATIONAL_B_SPLINE_SURFACE(((1.00515221228299,0.687966416849009,1.03437297609083),
(1.00515279666831,0.6879310247041,1.03437687481654),(1.00515125599611,0.68802433247961,
1.03436659622439),(1.00515259663208,0.687943139504264,1.03437554027513),
(1.00515441105761,0.687833252397824,1.03438764521218),(1.00515357264877,
0.687884028976962,1.03438205176893)))
REPRESENTATION_ITEM('')
SURFACE()
);
#1668=(
BOUNDED_SURFACE()
B_SPLINE_SURFACE(3,2,((#45575,#45576,#45577),(#45578,#45579,#45580),(#45581,
#45582,#45583),(#45584,#45585,#45586),(#45587,#45588,#45589),(#45590,#45591,
#45592)),.UNSPECIFIED.,.F.,.F.,.F.)
B_SPLINE_SURFACE_WITH_KNOTS((4,1,1,4),(3,3),(0.00209859031566758,0.00417178913822665,
0.00567815886986545,0.00925772626818232),(-0.00545725414786132,1.05802705461411),
 .UNSPECIFIED.)
GEOMETRIC_REPRESENTATION_ITEM()
RATIONAL_B_SPLINE_SURFACE(((1.00321534304372,0.688219339890755,1.03597632707853),
(1.00321587624839,0.688167636883823,1.03598229308132),(1.00321470970128,
0.688280752909962,1.03596924063877),(1.00321386482928,0.68836267721651,
1.03595978740442),(1.00321482739532,0.688269340527273,1.03597055751203),
(1.00321445716244,0.688305240725027,1.03596641499319)))
REPRESENTATION_ITEM('')
SURFACE()
);
#1669=(
BOUNDED_SURFACE()
B_SPLINE_SURFACE(3,2,((#45607,#45608,#45609),(#45610,#45611,#45612),(#45613,
#45614,#45615),(#45616,#45617,#45618),(#45619,#45620,#45621),(#45622,#45623,
#45624)),.UNSPECIFIED.,.F.,.F.,.F.)
B_SPLINE_SURFACE_WITH_KNOTS((4,1,1,4),(3,3),(0.00606711198524399,0.00688009229885085,
0.00722221478938814,0.00769307340420083),(-0.00991670930616596,1.00217563956271),
 .UNSPECIFIED.)
GEOMETRIC_REPRESENTATION_ITEM()
RATIONAL_B_SPLINE_SURFACE(((1.00594634748185,0.699526756281591,1.00129457713788),
(1.00594486311264,0.699601762532408,1.00129425397641),(1.00595105902295,
0.699288678698464,1.00129560288578),(1.00593196169786,0.700253680362731,
1.00129144521411),(1.00590427588377,0.701652664594436,1.00128541774564),
(1.00591770573521,0.700974044477186,1.00128834155369)))
REPRESENTATION_ITEM('')
SURFACE()
);
#1670=(
BOUNDED_SURFACE()
B_SPLINE_SURFACE(3,2,((#45647,#45648,#45649),(#45650,#45651,#45652),(#45653,
#45654,#45655),(#45656,#45657,#45658),(#45659,#45660,#45661),(#45662,#45663,
#45664)),.UNSPECIFIED.,.F.,.F.,.F.)
B_SPLINE_SURFACE_WITH_KNOTS((4,1,1,4),(3,3),(0.00586170810752336,0.00620302448742682,
0.00654434086733029,0.00722697362713722),(0.,1.),.UNSPECIFIED.)
GEOMETRIC_REPRESENTATION_ITEM()
RATIONAL_B_SPLINE_SURFACE(((1.,0.703291914743876,1.),(1.,0.703291156633914,
1.),(1.,0.702986672263162,1.),(1.,0.7036715161092,1.),(1.,0.704097894613167,
1.),(1.,0.704100348801905,1.)))
REPRESENTATION_ITEM('')
SURFACE()
);
#1671=(
BOUNDED_SURFACE()
B_SPLINE_SURFACE(3,2,((#45687,#45688,#45689),(#45690,#45691,#45692),(#45693,
#45694,#45695),(#45696,#45697,#45698),(#45699,#45700,#45701),(#45702,#45703,
#45704)),.UNSPECIFIED.,.F.,.F.,.F.)
B_SPLINE_SURFACE_WITH_KNOTS((4,1,1,4),(3,3),(0.00207336170120452,0.0058428956621075,
0.00742920796878192,0.00961242447694922),(-0.0132972947360473,1.00601408397336),
 .UNSPECIFIED.)
GEOMETRIC_REPRESENTATION_ITEM()
RATIONAL_B_SPLINE_SURFACE(((1.00789371657458,0.701374858896592,1.00354449933517),
(1.00789409196049,0.70136065776996,1.00354466789394),(1.00789185890845,
0.701445135781318,1.00354366519117),(1.00789463032497,0.701340291043177,
1.00354490963463),(1.00789794199947,0.701215007945169,1.00354639666903),
(1.00789593869161,0.701290794564665,1.00354549712782)))
REPRESENTATION_ITEM('')
SURFACE()
);
#1672=(
BOUNDED_SURFACE()
B_SPLINE_SURFACE(3,2,((#45718,#45719,#45720),(#45721,#45722,#45723),(#45724,
#45725,#45726),(#45727,#45728,#45729),(#45730,#45731,#45732),(#45733,#45734,
#45735)),.UNSPECIFIED.,.F.,.F.,.F.)
B_SPLINE_SURFACE_WITH_KNOTS((4,1,1,4),(3,3),(0.00207669134204795,0.00582595496795364,
0.00740373706151585,0.00957521363909962),(-0.00543600822727895,1.01524353115776),
 .UNSPECIFIED.)
GEOMETRIC_REPRESENTATION_ITEM()
RATIONAL_B_SPLINE_SURFACE(((1.00320196063785,0.70097233288763,1.00906644982378),
(1.00320209762572,0.700959539736781,1.00906683770916),(1.00320123008922,
0.701040558039555,1.00906438125293),(1.00320229942714,0.700940693718888,
1.00906740911607),(1.00320373776939,0.700806368480488,1.00907148182629),
(1.00320290663572,0.700883987161842,1.00906912844579)))
REPRESENTATION_ITEM('')
SURFACE()
);
#1673=(
BOUNDED_SURFACE()
B_SPLINE_SURFACE(3,2,((#45736,#45737,#45738),(#45739,#45740,#45741),(#45742,
#45743,#45744),(#45745,#45746,#45747),(#45748,#45749,#45750)),
 .UNSPECIFIED.,.F.,.F.,.F.)
B_SPLINE_SURFACE_WITH_KNOTS((4,1,4),(3,3),(0.00217622474172813,0.00539216358099794,
0.00861633928504423),(-0.00372387570917386,1.05641859002687),
 .UNSPECIFIED.)
GEOMETRIC_REPRESENTATION_ITEM()
RATIONAL_B_SPLINE_SURFACE(((1.00218965794407,0.689348696115286,1.03491605013112),
(1.00218988124539,0.689317015895015,1.03491961086995),(1.00218900484019,
0.689441353313379,1.03490563580698),(1.00219017995013,0.689274638034762,
1.03492437398368),(1.00218991474363,0.689312263429291,1.0349201450294)))
REPRESENTATION_ITEM('')
SURFACE()
);
#1674=(
BOUNDED_SURFACE()
B_SPLINE_SURFACE(3,2,((#45780,#45781,#45782),(#45783,#45784,#45785),(#45786,
#45787,#45788),(#45789,#45790,#45791),(#45792,#45793,#45794)),
 .UNSPECIFIED.,.F.,.F.,.F.)
B_SPLINE_SURFACE_WITH_KNOTS((4,1,4),(3,3),(0.00212311658518805,0.0053456007449197,
0.00856807426106279),(-0.00599908652418573,1.05456025857004),
 .UNSPECIFIED.)
GEOMETRIC_REPRESENTATION_ITEM()
RATIONAL_B_SPLINE_SURFACE(((1.00353590342769,0.689121530506963,1.03371052402231),
(1.00353634139136,0.689083024513225,1.03371469947142),(1.0035344304439,
0.689251036007775,1.03369648091954),(1.0035358507774,0.689126159547288,
1.03371002206611),(1.00353548205318,0.689158577972859,1.03370650673063)))
REPRESENTATION_ITEM('')
SURFACE()
);
#1675=(
BOUNDED_SURFACE()
B_SPLINE_SURFACE(3,2,((#45809,#45810,#45811),(#45812,#45813,#45814),(#45815,
#45816,#45817),(#45818,#45819,#45820),(#45821,#45822,#45823)),
 .UNSPECIFIED.,.F.,.F.,.F.)
B_SPLINE_SURFACE_WITH_KNOTS((4,1,4),(3,3),(0.00576991625672856,0.00655606720393187,
0.00734221533127076),(-0.057191197943434,1.),.UNSPECIFIED.)
GEOMETRIC_REPRESENTATION_ITEM()
RATIONAL_B_SPLINE_SURFACE(((1.03589548298643,0.686180004290742,1.),(1.03587833722817,
0.686329902866713,1.),(1.03597689454535,0.685468255264237,1.),(1.03568868718054,
0.687987938145351,1.),(1.03574452383035,0.687499780423329,1.)))
REPRESENTATION_ITEM('')
SURFACE()
);
#1676=(
BOUNDED_SURFACE()
B_SPLINE_SURFACE(3,2,((#45838,#45839,#45840),(#45841,#45842,#45843),(#45844,
#45845,#45846),(#45847,#45848,#45849),(#45850,#45851,#45852)),
 .UNSPECIFIED.,.F.,.F.,.F.)
B_SPLINE_SURFACE_WITH_KNOTS((4,1,4),(3,3),(0.00466657533706555,0.00544764278228739,
0.00622871275121123),(0.,1.07164194621731),.UNSPECIFIED.)
GEOMETRIC_REPRESENTATION_ITEM()
RATIONAL_B_SPLINE_SURFACE(((1.,0.682037840892741,1.0455588558038),(1.,0.682033056803698,
1.0455595412867),(1.,0.682024198389298,1.0455608105548),(1.,0.682718710372074,
1.04546129817456),(1.,0.682583619049144,1.04548065458515)))
REPRESENTATION_ITEM('')
SURFACE()
);
#1677=(
BOUNDED_SURFACE()
B_SPLINE_SURFACE(3,2,((#45857,#45858,#45859),(#45860,#45861,#45862),(#45863,
#45864,#45865),(#45866,#45867,#45868),(#45869,#45870,#45871),(#45872,#45873,
#45874)),.UNSPECIFIED.,.F.,.F.,.F.)
B_SPLINE_SURFACE_WITH_KNOTS((4,1,1,4),(3,3),(0.00204566630298345,0.00400993138179308,
0.00543715219179253,0.00882864065979569),(-0.00571744098087493,1.01125109042059),
 .UNSPECIFIED.)
GEOMETRIC_REPRESENTATION_ITEM()
RATIONAL_B_SPLINE_SURFACE(((1.00336919435212,0.702024299561637,1.00666656334336),
(1.00336959338059,0.701989008992314,1.0066673528937),(1.0033687757138,0.702061324451092,
1.00666573499135),(1.00336801089579,0.702128965897631,1.00666422165993),
(1.00336883090118,0.70205644361065,1.00666584418962),(1.0033686873612,0.702069138463297,
1.00666556016969)))
REPRESENTATION_ITEM('')
SURFACE()
);
#1678=(
BOUNDED_SURFACE()
B_SPLINE_SURFACE(3,2,((#45883,#45884,#45885),(#45886,#45887,#45888),(#45889,
#45890,#45891),(#45892,#45893,#45894),(#45895,#45896,#45897)),
 .UNSPECIFIED.,.F.,.F.,.F.)
B_SPLINE_SURFACE_WITH_KNOTS((4,1,4),(3,3),(0.0021959381419612,0.00532325757153969,
0.00845897824613069),(-0.00319606621206401,1.04760710946989),
 .UNSPECIFIED.)
GEOMETRIC_REPRESENTATION_ITEM()
RATIONAL_B_SPLINE_SURFACE(((1.00187832317392,0.692116891994823,1.0292172259266),
(1.00187850752375,0.692086674512343,1.02922009347922),(1.00187779088182,
0.692204142021837,1.02920894614871),(1.00187868898111,0.692056931145811,
1.02922291603959),(1.00187845708403,0.692094942278776,1.02921930889184)))
REPRESENTATION_ITEM('')
SURFACE()
);
#1679=(
BOUNDED_SURFACE()
B_SPLINE_SURFACE(3,2,((#45923,#45924,#45925),(#45926,#45927,#45928),(#45929,
#45930,#45931),(#45932,#45933,#45934),(#45935,#45936,#45937)),
 .UNSPECIFIED.,.F.,.F.,.F.)
B_SPLINE_SURFACE_WITH_KNOTS((4,1,4),(3,3),(0.00211126073213577,0.005246147458561,
0.00837261176721595),(-0.00426982890845349,1.04600228977135),
 .UNSPECIFIED.)
GEOMETRIC_REPRESENTATION_ITEM()
RATIONAL_B_SPLINE_SURFACE(((1.00251223791948,0.692224438834479,1.02819109612041),
(1.00251254913415,0.692186311764292,1.02819458841816),(1.0025113457616,
0.692333737555445,1.02818108476429),(1.00251230256491,0.692216519088568,
1.02819182153966),(1.00251205570066,0.692246762556132,1.02818905135057)))
REPRESENTATION_ITEM('')
SURFACE()
);
#1680=(
BOUNDED_SURFACE()
B_SPLINE_SURFACE(3,2,((#45976,#45977,#45978),(#45979,#45980,#45981),(#45982,
#45983,#45984),(#45985,#45986,#45987),(#45988,#45989,#45990)),
 .UNSPECIFIED.,.F.,.F.,.F.)
B_SPLINE_SURFACE_WITH_KNOTS((4,1,4),(3,3),(0.0020676411228087,0.00523242399231858,
0.00839719713565984),(-0.00487431079868958,1.01404338604498),
 .UNSPECIFIED.)
GEOMETRIC_REPRESENTATION_ITEM()
RATIONAL_B_SPLINE_SURFACE(((1.0028697300377,0.701473052287329,1.00834342667499),
(1.00286987939032,0.701457515709757,1.00834386090144),(1.00286870618288,
0.701579559954994,1.00834044992893),(1.00286959084033,0.701487532452169,
1.00834302197386),(1.00286947935389,0.70149912995714,1.0083426978392)))
REPRESENTATION_ITEM('')
SURFACE()
);
#1681=(
BOUNDED_SURFACE()
B_SPLINE_SURFACE(3,2,((#46006,#46007,#46008),(#46009,#46010,#46011),(#46012,
#46013,#46014),(#46015,#46016,#46017),(#46018,#46019,#46020)),
 .UNSPECIFIED.,.F.,.F.,.F.)
B_SPLINE_SURFACE_WITH_KNOTS((4,1,4),(3,3),(0.00217004352235611,0.00533300005217428,
0.00849594930601141),(-0.00629182520020718,1.01422385876462),
 .UNSPECIFIED.)
GEOMETRIC_REPRESENTATION_ITEM()
RATIONAL_B_SPLINE_SURFACE(((1.00370918483522,0.701018900626283,1.00845140932802),
(1.00370932633503,0.701007494948168,1.00845173173654),(1.0037081879283,
0.701099256915289,1.00844913786707),(1.00370970938845,0.700976618694825,
1.00845260452702),(1.00370951547823,0.700992248945929,1.00845216270093)))
REPRESENTATION_ITEM('')
SURFACE()
);
#1682=(
BOUNDED_SURFACE()
B_SPLINE_SURFACE(3,2,((#46021,#46022,#46023),(#46024,#46025,#46026),(#46027,
#46028,#46029),(#46030,#46031,#46032),(#46033,#46034,#46035)),
 .UNSPECIFIED.,.F.,.F.,.F.)
B_SPLINE_SURFACE_WITH_KNOTS((4,1,4),(3,3),(0.00658134838002377,0.00749225635020362,
0.00840316205258835),(-0.00373012175731709,1.03258272302577),
 .UNSPECIFIED.)
GEOMETRIC_REPRESENTATION_ITEM()
RATIONAL_B_SPLINE_SURFACE(((1.00221701425539,0.693103976914044,1.01992235850238),
(1.00221628705211,0.693204641938182,1.0199158237657),(1.00222066280505,
0.692598916841125,1.01995514481136),(1.00220180759727,0.69520899851706,
1.0197857096315),(1.00220551783436,0.694695399200248,1.01981905027116)))
REPRESENTATION_ITEM('')
SURFACE()
);
#1683=(
BOUNDED_SURFACE()
B_SPLINE_SURFACE(3,2,((#46066,#46067,#46068),(#46069,#46070,#46071),(#46072,
#46073,#46074),(#46075,#46076,#46077),(#46078,#46079,#46080)),
 .UNSPECIFIED.,.F.,.F.,.F.)
B_SPLINE_SURFACE_WITH_KNOTS((4,1,4),(3,3),(0.00227075980744937,0.00518182494025859,
0.00809289088251492),(-0.00521186425511147,1.0082792049588),
 .UNSPECIFIED.)
GEOMETRIC_REPRESENTATION_ITEM()
RATIONAL_B_SPLINE_SURFACE(((1.00306922824857,0.703103283428404,1.0048904399369),
(1.00306931230498,0.703095152370975,1.00489057387051),(1.0030686191024,
0.703162208175352,1.00488946933696),(1.0030692514443,0.703101039627365,
1.00489047689647),(1.00306931856182,0.703094547125393,1.00489058384003)))
REPRESENTATION_ITEM('')
SURFACE()
);
#1684=(
BOUNDED_SURFACE()
B_SPLINE_SURFACE(3,2,((#46124,#46125,#46126),(#46127,#46128,#46129),(#46130,
#46131,#46132),(#46133,#46134,#46135),(#46136,#46137,#46138)),
 .UNSPECIFIED.,.F.,.F.,.F.)
B_SPLINE_SURFACE_WITH_KNOTS((4,1,4),(3,3),(0.0034568776936703,0.00436551562806062,
0.00527415564536653),(-0.0036707976681412,1.03238825219618),
 .UNSPECIFIED.)
GEOMETRIC_REPRESENTATION_ITEM()
RATIONAL_B_SPLINE_SURFACE(((1.00217038145229,0.694762063835327,1.01969767194357),
(1.00216674940448,0.695272867490565,1.01966470866596),(1.00218520712167,
0.692677012510241,1.0198322248681),(1.00218093167134,0.693278302957743,
1.01979342227977),(1.00218164267322,0.693178309130949,1.01979987510022)))
REPRESENTATION_ITEM('')
SURFACE()
);
#1685=(
BOUNDED_SURFACE()
B_SPLINE_SURFACE(3,2,((#46187,#46188,#46189),(#46190,#46191,#46192),(#46193,
#46194,#46195),(#46196,#46197,#46198)),.UNSPECIFIED.,.F.,.F.,.F.)
B_SPLINE_SURFACE_WITH_KNOTS((4,4),(3,3),(0.00370520097294563,0.00941954636052541),
(-0.0101428155788133,1.05214450432649),.UNSPECIFIED.)
GEOMETRIC_REPRESENTATION_ITEM()
RATIONAL_B_SPLINE_SURFACE(((1.00600421848268,0.688427284912467,1.03215134260149),
(1.00599942234611,0.688676167476638,1.03212566028657),(1.00600312517364,
0.688484019234624,1.03214548815872),(1.00600227584133,0.688528093042654,
1.03214094016067)))
REPRESENTATION_ITEM('')
SURFACE()
);
#1686=(
BOUNDED_SURFACE()
B_SPLINE_SURFACE(3,2,((#46229,#46230,#46231),(#46232,#46233,#46234),(#46235,
#46236,#46237),(#46238,#46239,#46240),(#46241,#46242,#46243)),
 .UNSPECIFIED.,.F.,.F.,.F.)
B_SPLINE_SURFACE_WITH_KNOTS((4,1,4),(3,3),(0.00223723210298208,0.00504001293429967,
0.00784280154769125),(-0.0115719706077613,1.02620831455806),
 .UNSPECIFIED.)
GEOMETRIC_REPRESENTATION_ITEM()
RATIONAL_B_SPLINE_SURFACE(((1.00685773465935,0.695837442077627,1.01575618930365),
(1.00685815020969,0.695819011085351,1.01575714406352),(1.00685675136247,
0.695881054452243,1.01575393010109),(1.00685696168086,0.695871726156367,
1.01575441332426),(1.00685966802559,0.695751691075158,1.01576063136594)))
REPRESENTATION_ITEM('')
SURFACE()
);
#1687=(
BOUNDED_SURFACE()
B_SPLINE_SURFACE(3,2,((#46270,#46271,#46272),(#46273,#46274,#46275),(#46276,
#46277,#46278),(#46279,#46280,#46281),(#46282,#46283,#46284),(#46285,#46286,
#46287)),.UNSPECIFIED.,.F.,.F.,.F.)
B_SPLINE_SURFACE_WITH_KNOTS((4,1,1,4),(3,3),(0.0022677946226757,0.00391401491016076,
0.00511014847692749,0.00795245641742074),(-0.023127469090911,1.01566061070927),
 .UNSPECIFIED.)
GEOMETRIC_REPRESENTATION_ITEM()
RATIONAL_B_SPLINE_SURFACE(((1.01388126111192,0.695090628112123,1.0093310039554),
(1.01386984071289,0.695341483323618,1.00932332714653),(1.01389028228548,
0.694892473179237,1.00933706800142),(1.01393022057232,0.694015207212054,
1.00936391457605),(1.0139354303761,0.693900771067822,1.00936741661375),
(1.01394154050068,0.693766558892522,1.0093715238484)))
REPRESENTATION_ITEM('')
SURFACE()
);
#1688=(
BOUNDED_SURFACE()
B_SPLINE_SURFACE(3,2,((#46297,#46298,#46299),(#46300,#46301,#46302),(#46303,
#46304,#46305),(#46306,#46307,#46308),(#46309,#46310,#46311),(#46312,#46313,
#46314),(#46315,#46316,#46317),(#46318,#46319,#46320),(#46321,#46322,#46323),
(#46324,#46325,#46326),(#46327,#46328,#46329),(#46330,#46331,#46332),(#46333,
#46334,#46335),(#46336,#46337,#46338),(#46339,#46340,#46341),(#46342,#46343,
#46344),(#46345,#46346,#46347),(#46348,#46349,#46350),(#46351,#46352,#46353),
(#46354,#46355,#46356)),.UNSPECIFIED.,.F.,.F.,.F.)
B_SPLINE_SURFACE_WITH_KNOTS((4,1,1,1,1,1,1,1,1,1,1,1,1,1,1,1,1,4),(3,3),
(0.00261725296323532,0.00654848262222231,0.00767005292085768,0.00879162321949305,
0.0110347638167638,0.0121563341153991,0.0132779044140345,0.0143994747126699,
0.0155210450113053,0.0160818301606229,0.0166426153099406,0.0172034004592583,
0.017764185608576,0.0183249707578937,0.0188857559072114,0.0200073262058467,
0.0211288965044821,0.0239385696629217),(-0.0168546607502698,1.01516107000004),
 .UNSPECIFIED.)
GEOMETRIC_REPRESENTATION_ITEM()
RATIONAL_B_SPLINE_SURFACE(((1.01001782862897,0.698236966842449,1.00899620838692),
(1.01007197783254,0.69660585210528,1.00904483544348),(1.0100059927647,0.698593493833998,
1.00898557954655),(1.01008063671936,0.696345023931289,1.00905261129522),
(1.0100833239308,0.696264078138843,1.00905502446428),(1.01010437659876,
0.695629917067113,1.0090739301768),(1.01011267293465,0.695380009869258,
1.00908138045063),(1.0101193585501,0.695178621757002,1.00908738426563),
(1.01012286714301,0.695072933820154,1.00909053505151),(1.01011222145419,
0.695393609633978,1.00908097501224),(1.01009640880339,0.695869927770989,
1.00906677493884),(1.01005939440848,0.696984897540488,1.00903353527961),
(1.01003148595116,0.697825572804787,1.00900847293256),(1.0100535225878,
0.697161772039365,1.00902826226842),(1.01007027801628,0.696657054988678,
1.00904330897483),(1.01008761546103,0.696134806095195,1.00905887834337),
(1.01009729394663,0.695843264956113,1.009067569815),(1.01010211520435,0.695698036143758,
1.00907189939986),(1.01010122883875,0.695724735779169,1.009071103426),(1.01010042823197,
0.695748852135982,1.00907038446527)))
REPRESENTATION_ITEM('')
SURFACE()
);
#1689=(
BOUNDED_SURFACE()
B_SPLINE_SURFACE(3,2,((#46395,#46396,#46397),(#46398,#46399,#46400),(#46401,
#46402,#46403),(#46404,#46405,#46406),(#46407,#46408,#46409),(#46410,#46411,
#46412),(#46413,#46414,#46415),(#46416,#46417,#46418),(#46419,#46420,#46421),
(#46422,#46423,#46424),(#46425,#46426,#46427),(#46428,#46429,#46430),(#46431,
#46432,#46433),(#46434,#46435,#46436),(#46437,#46438,#46439),(#46440,#46441,
#46442),(#46443,#46444,#46445),(#46446,#46447,#46448),(#46449,#46450,#46451)),
 .UNSPECIFIED.,.F.,.F.,.F.)
B_SPLINE_SURFACE_WITH_KNOTS((4,1,1,1,1,1,1,1,1,1,1,1,1,1,1,1,4),(3,3),(0.00189550760743663,
0.00466304228864453,0.00576778402465584,0.00687252576066714,0.0074248966286728,
0.00797726749667845,0.0085296383646841,0.00908200923268976,0.00963438010069541,
0.0101867509687011,0.0112914927047124,0.0123962344407237,0.0146057179127463,
0.0168152013847689,0.0179199431207802,0.0190246848567915,0.0228969445771743),
(-0.018513716758316,1.01985338840949),.UNSPECIFIED.)
GEOMETRIC_REPRESENTATION_ITEM()
RATIONAL_B_SPLINE_SURFACE(((1.01111188940034,0.693834894151823,1.01193163048407),
(1.01111283607111,0.693808810598902,1.01193264699219),(1.01111479004412,
0.693754972918195,1.01193474511278),(1.0111066333323,0.69397971422442,1.01192598666784),
(1.01109405899069,0.694326174172893,1.01191248469782),(1.01107262942219,
0.694916621564155,1.01188947423726),(1.01104907236643,0.695565687462041,
1.01186417934145),(1.01104294959085,0.695734387866366,1.01185760487934),
(1.01107741820809,0.694784676483697,1.01189461629922),(1.01110652212194,
0.693982778395654,1.01192586725333),(1.01112142406403,0.693572186235118,
1.01194186853448),(1.01113071500695,0.693316193539388,1.01195184488448),
(1.01112525611268,0.693466602068436,1.01194598327923),(1.01111305723012,
0.693802717020363,1.01193288446644),(1.011091079394,0.694408270790531,1.01190928529172),
(1.01108796371199,0.694494116957465,1.01190593976108),(1.01101183808791,
0.696591600914965,1.01182419823323),(1.01107887545404,0.694744525088673,
1.01189618104843),(1.01102439606068,0.696245591975988,1.01183768262686)))
REPRESENTATION_ITEM('')
SURFACE()
);
#1690=(
BOUNDED_SURFACE()
B_SPLINE_SURFACE(3,2,((#46471,#46472,#46473),(#46474,#46475,#46476),(#46477,
#46478,#46479),(#46480,#46481,#46482),(#46483,#46484,#46485),(#46486,#46487,
#46488)),.UNSPECIFIED.,.F.,.F.,.F.)
B_SPLINE_SURFACE_WITH_KNOTS((4,1,1,4),(3,3),(0.00224117495089493,0.00389489708768512,
0.00509648123116401,0.00783693620606977),(0.,1.02101478396072),
 .UNSPECIFIED.)
GEOMETRIC_REPRESENTATION_ITEM()
RATIONAL_B_SPLINE_SURFACE(((1.,0.700585568194159,1.01258425919824),(1.,
0.700796860676309,1.01257537866651),(1.,0.70043057939319,1.01259077331058),
(1.,0.699548374367667,1.01262785200662),(1.,0.699365641730608,1.0126355321804),
(1.,0.69922285003429,1.0126415336537)))
REPRESENTATION_ITEM('')
SURFACE()
);
#1691=(
BOUNDED_SURFACE()
B_SPLINE_SURFACE(3,2,((#46563,#46564,#46565),(#46566,#46567,#46568),(#46569,
#46570,#46571),(#46572,#46573,#46574),(#46575,#46576,#46577),(#46578,#46579,
#46580),(#46581,#46582,#46583)),.UNSPECIFIED.,.F.,.F.,.F.)
B_SPLINE_SURFACE_WITH_KNOTS((4,1,1,1,4),(3,3),(0.0022673108647627,0.00394001125857995,
0.00515538157865687,0.00637075189873378,0.00792618538211219),(0.,1.00491872988737),
 .UNSPECIFIED.)
GEOMETRIC_REPRESENTATION_ITEM()
RATIONAL_B_SPLINE_SURFACE(((0.999999999999999,0.705232353097564,1.0028997648693),
(1.,0.705372001636867,1.00289839108241),(1.,0.705175813388567,1.00290032107641),
(1.,0.704343570165377,1.00290850823564),(1.,0.704147620189805,1.00291043588564),
(1.,0.704070859823098,1.00291119101266),(1.,0.704099757322705,1.00291090673467)))
REPRESENTATION_ITEM('')
SURFACE()
);
#1692=(
BOUNDED_SURFACE()
B_SPLINE_SURFACE(3,2,((#46621,#46622,#46623),(#46624,#46625,#46626),(#46627,
#46628,#46629),(#46630,#46631,#46632),(#46633,#46634,#46635),(#46636,#46637,
#46638),(#46639,#46640,#46641),(#46642,#46643,#46644),(#46645,#46646,#46647),
(#46648,#46649,#46650),(#46651,#46652,#46653),(#46654,#46655,#46656),(#46657,
#46658,#46659),(#46660,#46661,#46662),(#46663,#46664,#46665),(#46666,#46667,
#46668),(#46669,#46670,#46671),(#46672,#46673,#46674),(#46675,#46676,#46677),
(#46678,#46679,#46680),(#46681,#46682,#46683)),.UNSPECIFIED.,.F.,.F.,.F.)
B_SPLINE_SURFACE_WITH_KNOTS((4,1,1,1,1,1,1,1,1,1,1,1,1,1,1,1,1,1,4),(3,
3),(0.0026099542776046,0.00653870538517126,0.00765956913959363,0.00878043289401599,
0.00990129664843836,0.0110221604028607,0.0121430241572831,0.0132638879117055,
0.0143847516661278,0.0155056154205502,0.0160660472977614,0.0166264791749726,
0.0171869110521838,0.0177473429293949,0.0183077748066061,0.0188682066838173,
0.0199890704382397,0.021109934192662,0.023799829665576),(-0.00915496827453823,
1.00911975686673),.UNSPECIFIED.)
GEOMETRIC_REPRESENTATION_ITEM()
RATIONAL_B_SPLINE_SURFACE(((1.00540015433993,0.702355647466065,1.0053791968233),
(1.00542931479058,0.70074838906034,1.00540824410485),(1.00539359424759,
0.702717224990173,1.00537266219009),(1.00543444598592,0.700465569122908,
1.00541335538647),(1.00543429432824,0.700473928152822,1.00541320431736),
(1.0054419791353,0.700050358884654,1.00542085930037),(1.00544783298105,
0.699727708082337,1.00542669042788),(1.00545126427263,0.699538583014119,
1.00543010840291),(1.00545513095102,0.699325460403949,1.00543396007508),
(1.00545611971578,0.699270961915871,1.00543494500253),(1.00545189388041,
0.699503880450216,1.00543073556724),(1.00544147140227,0.700078343986232,
1.00542035353781),(1.00542302697162,0.701094959489083,1.00540198068835),
(1.00540736527206,0.701958197117509,1.00538637977044),(1.00541940619836,
0.701294528361412,1.00539837396699),(1.00542915527787,0.700757181042318,
1.00540808521119),(1.00543773400721,0.700284340789683,1.00541663064725),
(1.00544231061344,0.700032088555579,1.00542118949208),(1.0054454782231,
0.699857497040831,1.00542434480853),(1.00544494080388,0.699887118378614,
1.00542380947498),(1.0054436718169,0.699957062084557,1.00542254541283)))
REPRESENTATION_ITEM('')
SURFACE()
);
#1693=(
BOUNDED_SURFACE()
B_SPLINE_SURFACE(3,2,((#46706,#46707,#46708),(#46709,#46710,#46711),(#46712,
#46713,#46714),(#46715,#46716,#46717),(#46718,#46719,#46720),(#46721,#46722,
#46723),(#46724,#46725,#46726),(#46727,#46728,#46729),(#46730,#46731,#46732),
(#46733,#46734,#46735),(#46736,#46737,#46738),(#46739,#46740,#46741),(#46742,
#46743,#46744),(#46745,#46746,#46747),(#46748,#46749,#46750),(#46751,#46752,
#46753),(#46754,#46755,#46756),(#46757,#46758,#46759),(#46760,#46761,#46762)),
 .UNSPECIFIED.,.F.,.F.,.F.)
B_SPLINE_SURFACE_WITH_KNOTS((4,1,1,1,1,1,1,1,1,1,1,1,1,1,1,1,4),(3,3),(0.00261602648474055,
0.0065189601614092,0.00763244721963373,0.00874593427785826,0.0109729083943073,
0.0131998825107564,0.0143133695689809,0.0154268566272054,0.0159836001563177,
0.01654034368543,0.0170970872145422,0.0176538307436545,0.0182105742727668,
0.018767317801879,0.0198808048601036,0.0209942919183281,0.0236648513076151),
(-0.00774064349916484,1.01712637670702),.UNSPECIFIED.)
GEOMETRIC_REPRESENTATION_ITEM()
RATIONAL_B_SPLINE_SURFACE(((1.00456041043005,0.700340568355079,1.01018400253521),
(1.00458323931118,0.698840508294276,1.01023498246058),(1.00455494103971,
0.700699955832171,1.01017178865975),(1.00458745716147,0.698563358103575,
1.01024440148079),(1.00458727396229,0.698575395915544,1.01024399237267),
(1.00459859336925,0.69783161043644,1.01026927011268),(1.00460271760422,
0.697560611602978,1.01027848007745),(1.00460401826295,0.697475146783281,
1.01028138462123),(1.00460123571268,0.697657985026857,1.0102751708167),
(1.00459370847254,0.698152591496079,1.01025836148916),(1.00458255918927,
0.698885198338898,1.01023346365796),(1.00456722749737,0.699892626541195,
1.01019922595248),(1.00457157945601,0.699606664242021,1.01020894445446),
(1.00458110377577,0.698980831920699,1.01023021352619),(1.00458980036183,
0.698409389047836,1.01024963415859),(1.00459454344474,0.698097726413681,
1.01026022609304),(1.00459691632312,0.697941807248642,1.01026552504579),
(1.00459766104331,0.697892872523841,1.01026718810495),(1.00459534538961,
0.698045031519126,1.01026201694252)))
REPRESENTATION_ITEM('')
SURFACE()
);
#1694=(
BOUNDED_SURFACE()
B_SPLINE_SURFACE(3,2,((#46775,#46776,#46777),(#46778,#46779,#46780),(#46781,
#46782,#46783),(#46784,#46785,#46786),(#46787,#46788,#46789),(#46790,#46791,
#46792)),.UNSPECIFIED.,.F.,.F.,.F.)
B_SPLINE_SURFACE_WITH_KNOTS((4,1,1,4),(3,3),(0.00298650820277577,0.00587270729901942,
0.00708730098828811,0.00875892826895514),(-0.00731480018610578,1.04923751574683),
 .UNSPECIFIED.)
GEOMETRIC_REPRESENTATION_ITEM()
RATIONAL_B_SPLINE_SURFACE(((1.00433922363568,0.688684065923349,1.0304238586339),
(1.00433990537915,0.68863515449948,1.03042863858276),(1.00433814205992,
0.688761663161044,1.03041627531698),(1.00432100539233,0.689991126798849,
1.0302961239729),(1.00432211189368,0.689911741284742,1.03030388205205),
(1.004322288045,0.68989910337546,1.0303051171124)))
REPRESENTATION_ITEM('')
SURFACE()
);
#1695=(
BOUNDED_SURFACE()
B_SPLINE_SURFACE(3,2,((#46849,#46850,#46851),(#46852,#46853,#46854),(#46855,
#46856,#46857),(#46858,#46859,#46860),(#46861,#46862,#46863)),
 .UNSPECIFIED.,.F.,.F.,.F.)
B_SPLINE_SURFACE_WITH_KNOTS((4,1,4),(3,3),(0.00223740564663838,0.0050827929085138,
0.00792754419391784),(0.,1.02944699552801),.UNSPECIFIED.)
GEOMETRIC_REPRESENTATION_ITEM()
RATIONAL_B_SPLINE_SURFACE(((1.,0.698456271057167,1.01775911367536),(1.,
0.698436923194511,1.01776025314821),(1.,0.698505261200251,1.01775622845031),
(1.,0.698479809865279,1.017757727381),(1.,0.698365201647692,1.01776447711635)))
REPRESENTATION_ITEM('')
SURFACE()
);
#1696=(
BOUNDED_SURFACE()
B_SPLINE_SURFACE(3,2,((#46894,#46895,#46896),(#46897,#46898,#46899),(#46900,
#46901,#46902),(#46903,#46904,#46905)),.UNSPECIFIED.,.F.,.F.,.F.)
B_SPLINE_SURFACE_WITH_KNOTS((4,4),(3,3),(0.00378061934590702,0.00940525617675301),
(-0.0098380819768058,1.05450423974215),.UNSPECIFIED.)
GEOMETRIC_REPRESENTATION_ITEM()
RATIONAL_B_SPLINE_SURFACE(((1.00582192970445,0.687828329926041,1.03368087708045),
(1.00581735048427,0.688073867554131,1.03365438549437),(1.00582100747812,
0.68787777967012,1.03367554184055),(1.00582018844164,0.687921696378225,
1.03367080357187)))
REPRESENTATION_ITEM('')
SURFACE()
);
#1697=(
BOUNDED_SURFACE()
B_SPLINE_SURFACE(3,2,((#46941,#46942,#46943),(#46944,#46945,#46946),(#46947,
#46948,#46949),(#46950,#46951,#46952),(#46953,#46954,#46955),(#46956,#46957,
#46958),(#46959,#46960,#46961),(#46962,#46963,#46964),(#46965,#46966,#46967),
(#46968,#46969,#46970),(#46971,#46972,#46973),(#46974,#46975,#46976),(#46977,
#46978,#46979),(#46980,#46981,#46982),(#46983,#46984,#46985),(#46986,#46987,
#46988),(#46989,#46990,#46991)),.UNSPECIFIED.,.F.,.F.,.F.)
B_SPLINE_SURFACE_WITH_KNOTS((4,1,1,1,1,1,1,1,1,1,1,1,1,1,4),(3,3),(0.00180746184059761,
0.00487438597791521,0.00609862095279201,0.0073228559276688,0.0085470909025456,
0.0109955608522992,0.012219795827176,0.0134440308020528,0.0146682657769296,
0.0158925007518064,0.0171167357266832,0.01834097070156,0.0195652056764368,
0.0207894406513136,0.0250804959149023),(-0.0297036389200334,1.02228150212663),
 .UNSPECIFIED.)
GEOMETRIC_REPRESENTATION_ITEM()
RATIONAL_B_SPLINE_SURFACE(((1.01792057067006,0.691428609233124,1.01334580881894),
(1.01790539739825,0.691689875331743,1.01333450897875),(1.01794456212783,
0.691015504225207,1.01336367573928),(1.01790852581577,0.691636007619508,
1.01333683877409),(1.01801477009808,0.689806604607884,1.01341596102449),
(1.01801439627506,0.689813041405708,1.01341568263098),(1.01805278429309,
0.68915204436873,1.01344427095883),(1.01805069082588,0.689188091440009,
1.01344271191176),(1.01802936526785,0.68955529275428,1.01342683034048),
(1.0179780084348,0.690439597706898,1.01338858387568),(1.01791815953341,
0.691470126202861,1.01334401319706),(1.01791203091527,0.691575653881418,
1.01333944909207),(1.01795792283585,0.69078544836753,1.01337362572682),
(1.01799733489626,0.690106818511361,1.0134029766796),(1.018029784441,0.689548075080012,
1.01342714250714),(1.01804311488889,0.689318540266558,1.01343706995936),
(1.01799270295897,0.690186575085961,1.01339952718289)))
REPRESENTATION_ITEM('')
SURFACE()
);
#1698=(
BOUNDED_SURFACE()
B_SPLINE_SURFACE(3,2,((#47021,#47022,#47023),(#47024,#47025,#47026),(#47027,
#47028,#47029),(#47030,#47031,#47032),(#47033,#47034,#47035),(#47036,#47037,
#47038),(#47039,#47040,#47041),(#47042,#47043,#47044),(#47045,#47046,#47047),
(#47048,#47049,#47050),(#47051,#47052,#47053),(#47054,#47055,#47056),(#47057,
#47058,#47059),(#47060,#47061,#47062),(#47063,#47064,#47065),(#47066,#47067,
#47068)),.UNSPECIFIED.,.F.,.F.,.F.)
B_SPLINE_SURFACE_WITH_KNOTS((4,1,1,1,1,1,1,1,1,1,1,1,1,4),(3,3),(0.00174152498507269,
0.00601094925968871,0.00722900264372801,0.00844705602776732,0.00966510941180663,
0.0108831627958459,0.0121012161798852,0.0133192695639245,0.0145373229479639,
0.0157553763320032,0.0181914831000818,0.0194095364841211,0.0206275898681604,
0.0248970811962703),(-0.0178990764671792,1.06365987093854),
 .UNSPECIFIED.)
GEOMETRIC_REPRESENTATION_ITEM()
RATIONAL_B_SPLINE_SURFACE(((1.01072723796849,0.68092932560185,1.03986769249072),
(1.01074407302893,0.680428584022208,1.03993025985562),(1.01074291317966,
0.680463082547352,1.03992594928526),(1.01072004020438,0.681143415701839,
1.03984094205905),(1.01069798203529,0.681799513283581,1.03975896305336),
(1.01066933012785,0.682651734839026,1.03965247847288),(1.01067408104556,
0.682510423671846,1.03967013521984),(1.01070834185496,0.681491371089037,
1.03979746523874),(1.01073952588273,0.680563834214891,1.03991336042385),
(1.01075250782449,0.680177699692236,1.03996160770461),(1.01075350499417,
0.680148039904642,1.03996531367757),(1.01073183542055,0.680792579112819,
1.03988477888383),(1.01073000021761,0.680847165339321,1.03987795836704),
(1.01062128833396,0.684080688650128,1.03947393153737),(1.01073288101176,
0.680761479076527,1.03988866481501),(1.01059952149607,0.68472812088421,
1.03939303526176)))
REPRESENTATION_ITEM('')
SURFACE()
);
#1699=(
BOUNDED_SURFACE()
B_SPLINE_SURFACE(3,2,((#47076,#47077,#47078),(#47079,#47080,#47081),(#47082,
#47083,#47084),(#47085,#47086,#47087),(#47088,#47089,#47090),(#47091,#47092,
#47093),(#47094,#47095,#47096),(#47097,#47098,#47099),(#47100,#47101,#47102),
(#47103,#47104,#47105),(#47106,#47107,#47108),(#47109,#47110,#47111),(#47112,
#47113,#47114),(#47115,#47116,#47117),(#47118,#47119,#47120),(#47121,#47122,
#47123),(#47124,#47125,#47126)),.UNSPECIFIED.,.F.,.F.,.F.)
B_SPLINE_SURFACE_WITH_KNOTS((4,1,1,1,1,1,1,1,1,1,1,1,1,1,4),(3,3),(0.00226621447219306,
0.00524773882639187,0.00649265357668405,0.00773756832697622,0.0089824830772684,
0.0114723125778527,0.0127172273281449,0.0139621420784371,0.0152070568287293,
0.0164519715790214,0.0176968863293136,0.0189418010796058,0.020186715829898,
0.0214316305801901,0.0256040630347784),(0.,1.0152345218586),
 .UNSPECIFIED.)
GEOMETRIC_REPRESENTATION_ITEM()
RATIONAL_B_SPLINE_SURFACE(((1.,0.702313782623218,1.00907021437126),(1.,
0.702936907568063,1.00905122835008),(1.,0.702063225272511,1.00907784861414),
(1.,0.702911891024781,1.00905199058023),(1.,0.700831363730455,1.00911538225731),
(1.,0.70083848523692,1.00911516527182),(1.,0.70013918089471,1.0091364724064),
(1.,0.700266820798498,1.00913258334059),(1.,0.700674435878907,1.00912016369888),
(1.,0.701686628187104,1.00908932316719),(1.,0.702697815661407,1.00905851325183),
(1.,0.702654729965943,1.00905982603177),(1.,0.70185121745699,1.00908430828954),
(1.,0.701240439049059,1.00910291812355),(1.,0.700774764154181,1.00911710679228),
(1.,0.700672231940488,1.00912023085078),(1.,0.701062661849745,1.00910833482481)))
REPRESENTATION_ITEM('')
SURFACE()
);
#1700=(
BOUNDED_SURFACE()
B_SPLINE_SURFACE(3,2,((#47148,#47149,#47150),(#47151,#47152,#47153),(#47154,
#47155,#47156),(#47157,#47158,#47159),(#47160,#47161,#47162),(#47163,#47164,
#47165),(#47166,#47167,#47168),(#47169,#47170,#47171),(#47172,#47173,#47174),
(#47175,#47176,#47177),(#47178,#47179,#47180),(#47181,#47182,#47183),(#47184,
#47185,#47186),(#47187,#47188,#47189),(#47190,#47191,#47192),(#47193,#47194,
#47195),(#47196,#47197,#47198)),.UNSPECIFIED.,.F.,.F.,.F.)
B_SPLINE_SURFACE_WITH_KNOTS((4,1,1,1,1,1,1,1,1,1,1,1,1,1,4),(3,3),(-0.000294877643038348,
0.00281429782281611,0.00405540675591689,0.00529651568901767,0.00653762462211845,
0.00901984248832001,0.0102609514214208,0.0115020603545216,0.0127431692876223,
0.0139842782207231,0.0152253871538239,0.0164664960869247,0.0177076050200255,
0.0189487139531262,0.0232989706253928),(-0.0100183419747615,1.01952514777027),
 .UNSPECIFIED.)
GEOMETRIC_REPRESENTATION_ITEM()
RATIONAL_B_SPLINE_SURFACE(((1.00594367839033,0.697510790065643,1.0116929060728),
(1.00591694996598,0.698871068908738,1.01164032365921),(1.0059425385726,
0.69756879834631,1.01169066372711),(1.00591857689445,0.698788270298672,
1.0116435242903),(1.00596467551473,0.696442191942373,1.01173421338914),
(1.00596269074434,0.696543202055686,1.01173030878122),(1.00597755291228,
0.695786827780223,1.01175954689308),(1.00597476616083,0.695928652789648,
1.0117540645603),(1.00596594731885,0.696377466532329,1.0117367153896),(1.00594533763073,
0.697426347017788,1.01169617027065),(1.00592631693439,0.698394359590233,
1.01165875115051),(1.00592742439226,0.698337998186643,1.01166092983516),
(1.00594396371463,0.69749626917183,1.01169346738687),(1.00595489070713,
0.696940166181218,1.01171496388929),(1.00596573666354,0.696388187327233,
1.01173630097069),(1.00596720726343,0.696313344684252,1.01173919405899),
(1.00595737839104,0.696813561494266,1.01171985787118)))
REPRESENTATION_ITEM('')
SURFACE()
);
#1746=SHAPE_REPRESENTATION_RELATIONSHIP('SRR','None',#54633,#1760);
#1760=ADVANCED_BREP_SHAPE_REPRESENTATION('',(#1804),#54569);
#1786=STYLED_ITEM('',(#54714),#1804);
#1804=MANIFOLD_SOLID_BREP('Body1',#17669);
#2017=LINE('',#27007,#2610);
#2018=LINE('',#27155,#2611);
#2019=LINE('',#27232,#2612);
#2020=LINE('',#27654,#2613);
#2021=LINE('',#27771,#2614);
#2022=LINE('',#27891,#2615);
#2023=LINE('',#27999,#2616);
#2024=LINE('',#28107,#2617);
#2025=LINE('',#28178,#2618);
#2026=LINE('',#28255,#2619);
#2027=LINE('',#28350,#2620);
#2028=LINE('',#28491,#2621);
#2029=LINE('',#28632,#2622);
#2030=LINE('',#28740,#2623);
#2031=LINE('',#28848,#2624);
#2032=LINE('',#30659,#2625);
#2033=LINE('',#30713,#2626);
#2034=LINE('',#30767,#2627);
#2035=LINE('',#30821,#2628);
#2036=LINE('',#30875,#2629);
#2037=LINE('',#30929,#2630);
#2038=LINE('',#30981,#2631);
#2039=LINE('',#31014,#2632);
#2040=LINE('',#31047,#2633);
#2041=LINE('',#31080,#2634);
#2042=LINE('',#31138,#2635);
#2043=LINE('',#31195,#2636);
#2044=LINE('',#31395,#2637);
#2045=LINE('',#31435,#2638);
#2046=LINE('',#31536,#2639);
#2047=LINE('',#31910,#2640);
#2048=LINE('',#32077,#2641);
#2049=LINE('',#32285,#2642);
#2050=LINE('',#32314,#2643);
#2051=LINE('',#32385,#2644);
#2052=LINE('',#32431,#2645);
#2053=LINE('',#32477,#2646);
#2054=LINE('',#32523,#2647);
#2055=LINE('',#32606,#2648);
#2056=LINE('',#32652,#2649);
#2057=LINE('',#32735,#2650);
#2058=LINE('',#32777,#2651);
#2059=LINE('',#32885,#2652);
#2060=LINE('',#32931,#2653);
#2061=LINE('',#33051,#2654);
#2062=LINE('',#33104,#2655);
#2063=LINE('',#33156,#2656);
#2064=LINE('',#33202,#2657);
#2065=LINE('',#33322,#2658);
#2066=LINE('',#33364,#2659);
#2067=LINE('',#33472,#2660);
#2068=LINE('',#33514,#2661);
#2069=LINE('',#33622,#2662);
#2070=LINE('',#33664,#2663);
#2071=LINE('',#33772,#2664);
#2072=LINE('',#33814,#2665);
#2073=LINE('',#33922,#2666);
#2074=LINE('',#33975,#2667);
#2075=LINE('',#34484,#2668);
#2076=LINE('',#34526,#2669);
#2077=LINE('',#35085,#2670);
#2078=LINE('',#35086,#2671);
#2079=LINE('',#35143,#2672);
#2080=LINE('',#35147,#2673);
#2081=LINE('',#35167,#2674);
#2082=LINE('',#35214,#2675);
#2083=LINE('',#35926,#2676);
#2084=LINE('',#35952,#2677);
#2085=LINE('',#36068,#2678);
#2086=LINE('',#36165,#2679);
#2610=VECTOR('',#21179,0.01);
#2611=VECTOR('',#21180,0.01);
#2612=VECTOR('',#21181,0.01);
#2613=VECTOR('',#21182,0.01);
#2614=VECTOR('',#21183,0.01);
#2615=VECTOR('',#21184,0.01);
#2616=VECTOR('',#21185,0.01);
#2617=VECTOR('',#21186,0.01);
#2618=VECTOR('',#21187,0.01);
#2619=VECTOR('',#21188,0.01);
#2620=VECTOR('',#21189,0.01);
#2621=VECTOR('',#21190,0.01);
#2622=VECTOR('',#21191,0.01);
#2623=VECTOR('',#21192,0.01);
#2624=VECTOR('',#21193,0.01);
#2625=VECTOR('',#21200,0.01);
#2626=VECTOR('',#21201,0.01);
#2627=VECTOR('',#21202,0.01);
#2628=VECTOR('',#21203,0.01);
#2629=VECTOR('',#21204,0.01);
#2630=VECTOR('',#21205,0.01);
#2631=VECTOR('',#21206,0.01);
#2632=VECTOR('',#21207,0.01);
#2633=VECTOR('',#21208,0.01);
#2634=VECTOR('',#21209,0.01);
#2635=VECTOR('',#21210,0.01);
#2636=VECTOR('',#21211,0.01);
#2637=VECTOR('',#21212,0.01);
#2638=VECTOR('',#21213,0.01);
#2639=VECTOR('',#21214,0.01);
#2640=VECTOR('',#21219,0.01);
#2641=VECTOR('',#21222,0.01);
#2642=VECTOR('',#21225,0.01);
#2643=VECTOR('',#21226,0.01);
#2644=VECTOR('',#21227,0.01);
#2645=VECTOR('',#21228,0.01);
#2646=VECTOR('',#21229,0.01);
#2647=VECTOR('',#21230,0.01);
#2648=VECTOR('',#21231,0.01);
#2649=VECTOR('',#21232,0.01);
#2650=VECTOR('',#21233,0.01);
#2651=VECTOR('',#21234,0.01);
#2652=VECTOR('',#21235,0.01);
#2653=VECTOR('',#21236,0.01);
#2654=VECTOR('',#21237,0.01);
#2655=VECTOR('',#21238,0.01);
#2656=VECTOR('',#21239,0.01);
#2657=VECTOR('',#21240,0.01);
#2658=VECTOR('',#21241,0.01);
#2659=VECTOR('',#21242,0.01);
#2660=VECTOR('',#21243,0.01);
#2661=VECTOR('',#21244,0.01);
#2662=VECTOR('',#21245,0.01);
#2663=VECTOR('',#21246,0.01);
#2664=VECTOR('',#21247,0.01);
#2665=VECTOR('',#21248,0.01);
#2666=VECTOR('',#21249,0.01);
#2667=VECTOR('',#21250,0.01);
#2668=VECTOR('',#21251,0.01);
#2669=VECTOR('',#21252,0.01);
#2670=VECTOR('',#21253,0.01);
#2671=VECTOR('',#21254,0.01);
#2672=VECTOR('',#21261,1.);
#2673=VECTOR('',#21264,1.);
#2674=VECTOR('',#21269,1.);
#2675=VECTOR('',#21274,1.);
#2676=VECTOR('',#21297,1.);
#2677=VECTOR('',#21298,1.);
#2678=VECTOR('',#21301,1.);
#2679=VECTOR('',#21304,1.);
#3205=CYLINDRICAL_SURFACE('',#18525,0.00899250965190647);
#3206=CYLINDRICAL_SURFACE('',#18538,0.00899245661942092);
#3207=CYLINDRICAL_SURFACE('',#18543,0.0208790072664728);
#3208=CYLINDRICAL_SURFACE('',#18544,0.0055);
#3209=CYLINDRICAL_SURFACE('',#18545,0.0055);
#3210=CYLINDRICAL_SURFACE('',#18546,0.0208790057965016);
#3211=CYLINDRICAL_SURFACE('',#18549,0.004);
#3212=CYLINDRICAL_SURFACE('',#18550,0.004);
#3213=CYLINDRICAL_SURFACE('',#18552,0.00816904972011834);
#3214=CYLINDRICAL_SURFACE('',#18554,0.00816904972011834);
#3215=CYLINDRICAL_SURFACE('',#18555,0.00816904972011834);
#3216=CYLINDRICAL_SURFACE('',#18557,0.00816904972011834);
#3217=CYLINDRICAL_SURFACE('',#18581,9.9978220630668E-5);
#3218=CYLINDRICAL_SURFACE('',#18585,9.99782191435892E-5);
#3219=CYLINDRICAL_SURFACE('',#18600,9.9975692043519E-5);
#3220=CYLINDRICAL_SURFACE('',#18603,9.99782206312813E-5);
#3221=CYLINDRICAL_SURFACE('',#18619,0.00922904672092924);
#3222=CYLINDRICAL_SURFACE('',#18620,0.00919655447393812);
#3223=CYLINDRICAL_SURFACE('',#18621,0.00916484752937528);
#3224=CYLINDRICAL_SURFACE('',#18622,0.00913387652341414);
#3225=CYLINDRICAL_SURFACE('',#18623,0.00940354056819424);
#3226=CYLINDRICAL_SURFACE('',#18624,0.0090741001070128);
#3227=CYLINDRICAL_SURFACE('',#18625,0.00893498310288807);
#3228=CYLINDRICAL_SURFACE('',#18626,0.00910365113802367);
#3229=CYLINDRICAL_SURFACE('',#18627,0.00926228971845552);
#3230=CYLINDRICAL_SURFACE('',#18628,0.00929634095813992);
#3231=CYLINDRICAL_SURFACE('',#18629,0.00933121777652104);
#3232=CYLINDRICAL_SURFACE('',#18630,0.00936694531422377);
#3233=CYLINDRICAL_SURFACE('',#18631,0.00896125355933549);
#3234=CYLINDRICAL_SURFACE('',#18632,0.00898813022568495);
#3235=CYLINDRICAL_SURFACE('',#18633,0.0090162483098341);
#3236=CYLINDRICAL_SURFACE('',#18634,0.00904504186665572);
#3237=CYLINDRICAL_SURFACE('',#18635,0.00944176434989097);
#3238=CYLINDRICAL_SURFACE('',#18638,0.00922903063599022);
#3239=CYLINDRICAL_SURFACE('',#18639,0.0091965290470675);
#3240=CYLINDRICAL_SURFACE('',#18640,0.00916482066045435);
#3241=CYLINDRICAL_SURFACE('',#18641,0.00913384823750702);
#3242=CYLINDRICAL_SURFACE('',#18642,0.00940351008025872);
#3243=CYLINDRICAL_SURFACE('',#18643,0.00907404122166741);
#3244=CYLINDRICAL_SURFACE('',#18644,0.00893489737206019);
#3245=CYLINDRICAL_SURFACE('',#18645,0.00910361854634517);
#3246=CYLINDRICAL_SURFACE('',#18646,0.00926227916230088);
#3247=CYLINDRICAL_SURFACE('',#18647,0.0092963345462741);
#3248=CYLINDRICAL_SURFACE('',#18648,0.0093312128177526);
#3249=CYLINDRICAL_SURFACE('',#18649,0.00936693006801195);
#3250=CYLINDRICAL_SURFACE('',#18650,0.00896117725022564);
#3251=CYLINDRICAL_SURFACE('',#18651,0.00898806494315033);
#3252=CYLINDRICAL_SURFACE('',#18652,0.00901619755067071);
#3253=CYLINDRICAL_SURFACE('',#18653,0.00904499652239313);
#3254=CYLINDRICAL_SURFACE('',#18654,0.00944177138396684);
#3255=CYLINDRICAL_SURFACE('',#18657,9.99999926721475E-5);
#3256=CYLINDRICAL_SURFACE('',#18658,9.9999993193412E-5);
#3257=CYLINDRICAL_SURFACE('',#18660,9.99999931392734E-5);
#3258=CYLINDRICAL_SURFACE('',#18661,9.99999934745441E-5);
#3259=CYLINDRICAL_SURFACE('',#18662,9.9999993342419E-5);
#3260=CYLINDRICAL_SURFACE('',#18663,9.99999935401327E-5);
#3261=CYLINDRICAL_SURFACE('',#18664,9.99999931014713E-5);
#3262=CYLINDRICAL_SURFACE('',#18665,9.99999936857353E-5);
#3263=CYLINDRICAL_SURFACE('',#18666,9.99999927304824E-5);
#3264=CYLINDRICAL_SURFACE('',#18667,9.99999928406026E-5);
#3265=CYLINDRICAL_SURFACE('',#18668,9.99999939684521E-5);
#3266=CYLINDRICAL_SURFACE('',#18669,9.99999946770892E-5);
#3267=CYLINDRICAL_SURFACE('',#18670,9.99999905417014E-5);
#3268=CYLINDRICAL_SURFACE('',#18671,9.99999885290244E-5);
#3269=CYLINDRICAL_SURFACE('',#18672,9.99999926628113E-5);
#3270=CYLINDRICAL_SURFACE('',#18673,9.99999939595615E-5);
#3271=CYLINDRICAL_SURFACE('',#18674,9.99999928350082E-5);
#3272=CYLINDRICAL_SURFACE('',#18675,9.99999930681036E-5);
#3273=CYLINDRICAL_SURFACE('',#18676,9.99999927905074E-5);
#3274=CYLINDRICAL_SURFACE('',#18677,9.99999924750999E-5);
#3275=CYLINDRICAL_SURFACE('',#18678,9.99999926945566E-5);
#3276=CYLINDRICAL_SURFACE('',#18679,9.9999992897476E-5);
#3277=CYLINDRICAL_SURFACE('',#18680,9.99999930879845E-5);
#3278=CYLINDRICAL_SURFACE('',#18681,9.99999916320171E-5);
#3279=CYLINDRICAL_SURFACE('',#18682,9.9999990509756E-5);
#3280=CYLINDRICAL_SURFACE('',#18683,9.99999909505769E-5);
#3281=CYLINDRICAL_SURFACE('',#18685,9.99996240727958E-5);
#3282=CYLINDRICAL_SURFACE('',#18686,9.99996321868604E-5);
#3283=CYLINDRICAL_SURFACE('',#18691,9.9999992669382E-5);
#3284=CYLINDRICAL_SURFACE('',#18692,9.99999931979935E-5);
#3285=CYLINDRICAL_SURFACE('',#18693,9.99999931392223E-5);
#3286=CYLINDRICAL_SURFACE('',#18694,9.99999934779342E-5);
#3287=CYLINDRICAL_SURFACE('',#18695,9.9999993345512E-5);
#3288=CYLINDRICAL_SURFACE('',#18696,9.99999935437013E-5);
#3289=CYLINDRICAL_SURFACE('',#18697,9.99999931072116E-5);
#3290=CYLINDRICAL_SURFACE('',#18698,9.99999936854522E-5);
#3291=CYLINDRICAL_SURFACE('',#18699,9.99999927924378E-5);
#3292=CYLINDRICAL_SURFACE('',#18700,9.99999928656628E-5);
#3293=CYLINDRICAL_SURFACE('',#18701,9.99999939755481E-5);
#3294=CYLINDRICAL_SURFACE('',#18702,9.9999994677093E-5);
#3295=CYLINDRICAL_SURFACE('',#18703,9.99999905763174E-5);
#3296=CYLINDRICAL_SURFACE('',#18704,9.9999988507358E-5);
#3297=CYLINDRICAL_SURFACE('',#18705,9.99999926697609E-5);
#3298=CYLINDRICAL_SURFACE('',#18706,9.99999939599216E-5);
#3299=CYLINDRICAL_SURFACE('',#18707,9.99999928286534E-5);
#3300=CYLINDRICAL_SURFACE('',#18708,9.99999930733179E-5);
#3301=CYLINDRICAL_SURFACE('',#18709,9.99999927766249E-5);
#3302=CYLINDRICAL_SURFACE('',#18710,9.99999924822146E-5);
#3303=CYLINDRICAL_SURFACE('',#18711,9.9999992646252E-5);
#3304=CYLINDRICAL_SURFACE('',#18712,9.99999929064612E-5);
#3305=CYLINDRICAL_SURFACE('',#18713,9.99999929016321E-5);
#3306=CYLINDRICAL_SURFACE('',#18714,9.99999916467037E-5);
#3307=CYLINDRICAL_SURFACE('',#18715,9.99999905246489E-5);
#3308=CYLINDRICAL_SURFACE('',#18716,9.99999909501884E-5);
#3309=CYLINDRICAL_SURFACE('',#18718,9.99996239781536E-5);
#3310=CYLINDRICAL_SURFACE('',#18719,9.99996322518559E-5);
#3311=CYLINDRICAL_SURFACE('',#18726,9.99999890432553E-5);
#3312=CYLINDRICAL_SURFACE('',#18732,9.99999916933113E-5);
#3313=CYLINDRICAL_SURFACE('',#18737,9.99999916975992E-5);
#3314=CYLINDRICAL_SURFACE('',#18743,9.99999890830763E-5);
#3482=FACE_BOUND('',#4796,.T.);
#3483=FACE_BOUND('',#4797,.T.);
#3484=FACE_BOUND('',#4801,.T.);
#3485=FACE_BOUND('',#4802,.T.);
#3486=FACE_BOUND('',#4803,.T.);
#3487=FACE_BOUND('',#4804,.T.);
#3488=FACE_BOUND('',#4805,.T.);
#3489=FACE_BOUND('',#4806,.T.);
#3490=FACE_BOUND('',#4807,.T.);
#3491=FACE_BOUND('',#4808,.T.);
#3492=FACE_BOUND('',#4809,.T.);
#3493=FACE_BOUND('',#4810,.T.);
#3494=FACE_BOUND('',#4811,.T.);
#3495=FACE_BOUND('',#4812,.T.);
#3496=FACE_BOUND('',#4813,.T.);
#3497=FACE_BOUND('',#4814,.T.);
#3498=FACE_BOUND('',#4815,.T.);
#3499=FACE_BOUND('',#4816,.T.);
#3500=FACE_BOUND('',#4817,.T.);
#3781=FACE_OUTER_BOUND('',#4792,.T.);
#3782=FACE_OUTER_BOUND('',#4793,.T.);
#3783=FACE_OUTER_BOUND('',#4794,.T.);
#3784=FACE_OUTER_BOUND('',#4795,.T.);
#3785=FACE_OUTER_BOUND('',#4798,.T.);
#3786=FACE_OUTER_BOUND('',#4799,.T.);
#3787=FACE_OUTER_BOUND('',#4800,.T.);
#3788=FACE_OUTER_BOUND('',#4818,.T.);
#3789=FACE_OUTER_BOUND('',#4819,.T.);
#3790=FACE_OUTER_BOUND('',#4820,.T.);
#3791=FACE_OUTER_BOUND('',#4821,.T.);
#3792=FACE_OUTER_BOUND('',#4822,.T.);
#3793=FACE_OUTER_BOUND('',#4823,.T.);
#3794=FACE_OUTER_BOUND('',#4824,.T.);
#3795=FACE_OUTER_BOUND('',#4825,.T.);
#3796=FACE_OUTER_BOUND('',#4826,.T.);
#3797=FACE_OUTER_BOUND('',#4827,.T.);
#3798=FACE_OUTER_BOUND('',#4828,.T.);
#3799=FACE_OUTER_BOUND('',#4829,.T.);
#3800=FACE_OUTER_BOUND('',#4830,.T.);
#3801=FACE_OUTER_BOUND('',#4831,.T.);
#3802=FACE_OUTER_BOUND('',#4832,.T.);
#3803=FACE_OUTER_BOUND('',#4833,.T.);
#3804=FACE_OUTER_BOUND('',#4834,.T.);
#3805=FACE_OUTER_BOUND('',#4835,.T.);
#3806=FACE_OUTER_BOUND('',#4836,.T.);
#3807=FACE_OUTER_BOUND('',#4837,.T.);
#3808=FACE_OUTER_BOUND('',#4838,.T.);
#3809=FACE_OUTER_BOUND('',#4839,.T.);
#3810=FACE_OUTER_BOUND('',#4840,.T.);
#3811=FACE_OUTER_BOUND('',#4841,.T.);
#3812=FACE_OUTER_BOUND('',#4842,.T.);
#3813=FACE_OUTER_BOUND('',#4843,.T.);
#3814=FACE_OUTER_BOUND('',#4844,.T.);
#3815=FACE_OUTER_BOUND('',#4845,.T.);
#3816=FACE_OUTER_BOUND('',#4846,.T.);
#3817=FACE_OUTER_BOUND('',#4847,.T.);
#3818=FACE_OUTER_BOUND('',#4848,.T.);
#3819=FACE_OUTER_BOUND('',#4849,.T.);
#3820=FACE_OUTER_BOUND('',#4850,.T.);
#3821=FACE_OUTER_BOUND('',#4851,.T.);
#3822=FACE_OUTER_BOUND('',#4852,.T.);
#3823=FACE_OUTER_BOUND('',#4853,.T.);
#3824=FACE_OUTER_BOUND('',#4854,.T.);
#3825=FACE_OUTER_BOUND('',#4855,.T.);
#3826=FACE_OUTER_BOUND('',#4856,.T.);
#3827=FACE_OUTER_BOUND('',#4857,.T.);
#3828=FACE_OUTER_BOUND('',#4858,.T.);
#3829=FACE_OUTER_BOUND('',#4859,.T.);
#3830=FACE_OUTER_BOUND('',#4860,.T.);
#3831=FACE_OUTER_BOUND('',#4861,.T.);
#3832=FACE_OUTER_BOUND('',#4862,.T.);
#3833=FACE_OUTER_BOUND('',#4863,.T.);
#3834=FACE_OUTER_BOUND('',#4864,.T.);
#3835=FACE_OUTER_BOUND('',#4865,.T.);
#3836=FACE_OUTER_BOUND('',#4866,.T.);
#3837=FACE_OUTER_BOUND('',#4867,.T.);
#3838=FACE_OUTER_BOUND('',#4868,.T.);
#3839=FACE_OUTER_BOUND('',#4869,.T.);
#3840=FACE_OUTER_BOUND('',#4870,.T.);
#3841=FACE_OUTER_BOUND('',#4871,.T.);
#3842=FACE_OUTER_BOUND('',#4872,.T.);
#3843=FACE_OUTER_BOUND('',#4873,.T.);
#3844=FACE_OUTER_BOUND('',#4874,.T.);
#3845=FACE_OUTER_BOUND('',#4875,.T.);
#3846=FACE_OUTER_BOUND('',#4876,.T.);
#3847=FACE_OUTER_BOUND('',#4877,.T.);
#3848=FACE_OUTER_BOUND('',#4878,.T.);
#3849=FACE_OUTER_BOUND('',#4879,.T.);
#3850=FACE_OUTER_BOUND('',#4880,.T.);
#3851=FACE_OUTER_BOUND('',#4881,.T.);
#3852=FACE_OUTER_BOUND('',#4882,.T.);
#3853=FACE_OUTER_BOUND('',#4883,.T.);
#3854=FACE_OUTER_BOUND('',#4884,.T.);
#3855=FACE_OUTER_BOUND('',#4885,.T.);
#3856=FACE_OUTER_BOUND('',#4886,.T.);
#3857=FACE_OUTER_BOUND('',#4887,.T.);
#3858=FACE_OUTER_BOUND('',#4888,.T.);
#3859=FACE_OUTER_BOUND('',#4889,.T.);
#3860=FACE_OUTER_BOUND('',#4890,.T.);
#3861=FACE_OUTER_BOUND('',#4891,.T.);
#3862=FACE_OUTER_BOUND('',#4892,.T.);
#3863=FACE_OUTER_BOUND('',#4893,.T.);
#3864=FACE_OUTER_BOUND('',#4894,.T.);
#3865=FACE_OUTER_BOUND('',#4895,.T.);
#3866=FACE_OUTER_BOUND('',#4896,.T.);
#3867=FACE_OUTER_BOUND('',#4897,.T.);
#3868=FACE_OUTER_BOUND('',#4898,.T.);
#3869=FACE_OUTER_BOUND('',#4899,.T.);
#3870=FACE_OUTER_BOUND('',#4900,.T.);
#3871=FACE_OUTER_BOUND('',#4901,.T.);
#3872=FACE_OUTER_BOUND('',#4902,.T.);
#3873=FACE_OUTER_BOUND('',#4903,.T.);
#3874=FACE_OUTER_BOUND('',#4904,.T.);
#3875=FACE_OUTER_BOUND('',#4905,.T.);
#3876=FACE_OUTER_BOUND('',#4906,.T.);
#3877=FACE_OUTER_BOUND('',#4907,.T.);
#3878=FACE_OUTER_BOUND('',#4908,.T.);
#3879=FACE_OUTER_BOUND('',#4909,.T.);
#3880=FACE_OUTER_BOUND('',#4910,.T.);
#3881=FACE_OUTER_BOUND('',#4911,.T.);
#3882=FACE_OUTER_BOUND('',#4912,.T.);
#3883=FACE_OUTER_BOUND('',#4913,.T.);
#3884=FACE_OUTER_BOUND('',#4914,.T.);
#3885=FACE_OUTER_BOUND('',#4915,.T.);
#3886=FACE_OUTER_BOUND('',#4916,.T.);
#3887=FACE_OUTER_BOUND('',#4917,.T.);
#3888=FACE_OUTER_BOUND('',#4918,.T.);
#3889=FACE_OUTER_BOUND('',#4919,.T.);
#3890=FACE_OUTER_BOUND('',#4920,.T.);
#3891=FACE_OUTER_BOUND('',#4921,.T.);
#3892=FACE_OUTER_BOUND('',#4922,.T.);
#3893=FACE_OUTER_BOUND('',#4923,.T.);
#3894=FACE_OUTER_BOUND('',#4924,.T.);
#3895=FACE_OUTER_BOUND('',#4925,.T.);
#3896=FACE_OUTER_BOUND('',#4926,.T.);
#3897=FACE_OUTER_BOUND('',#4927,.T.);
#3898=FACE_OUTER_BOUND('',#4928,.T.);
#3899=FACE_OUTER_BOUND('',#4929,.T.);
#3900=FACE_OUTER_BOUND('',#4930,.T.);
#3901=FACE_OUTER_BOUND('',#4931,.T.);
#3902=FACE_OUTER_BOUND('',#4932,.T.);
#3903=FACE_OUTER_BOUND('',#4933,.T.);
#3904=FACE_OUTER_BOUND('',#4934,.T.);
#3905=FACE_OUTER_BOUND('',#4935,.T.);
#3906=FACE_OUTER_BOUND('',#4936,.T.);
#3907=FACE_OUTER_BOUND('',#4937,.T.);
#3908=FACE_OUTER_BOUND('',#4938,.T.);
#3909=FACE_OUTER_BOUND('',#4939,.T.);
#3910=FACE_OUTER_BOUND('',#4940,.T.);
#3911=FACE_OUTER_BOUND('',#4941,.T.);
#3912=FACE_OUTER_BOUND('',#4942,.T.);
#3913=FACE_OUTER_BOUND('',#4943,.T.);
#3914=FACE_OUTER_BOUND('',#4944,.T.);
#3915=FACE_OUTER_BOUND('',#4945,.T.);
#3916=FACE_OUTER_BOUND('',#4946,.T.);
#3917=FACE_OUTER_BOUND('',#4947,.T.);
#3918=FACE_OUTER_BOUND('',#4948,.T.);
#3919=FACE_OUTER_BOUND('',#4949,.T.);
#3920=FACE_OUTER_BOUND('',#4950,.T.);
#3921=FACE_OUTER_BOUND('',#4951,.T.);
#3922=FACE_OUTER_BOUND('',#4952,.T.);
#3923=FACE_OUTER_BOUND('',#4953,.T.);
#3924=FACE_OUTER_BOUND('',#4954,.T.);
#3925=FACE_OUTER_BOUND('',#4955,.T.);
#3926=FACE_OUTER_BOUND('',#4956,.T.);
#3927=FACE_OUTER_BOUND('',#4957,.T.);
#3928=FACE_OUTER_BOUND('',#4958,.T.);
#3929=FACE_OUTER_BOUND('',#4959,.T.);
#3930=FACE_OUTER_BOUND('',#4960,.T.);
#3931=FACE_OUTER_BOUND('',#4961,.T.);
#3932=FACE_OUTER_BOUND('',#4962,.T.);
#3933=FACE_OUTER_BOUND('',#4963,.T.);
#3934=FACE_OUTER_BOUND('',#4964,.T.);
#3935=FACE_OUTER_BOUND('',#4965,.T.);
#3936=FACE_OUTER_BOUND('',#4966,.T.);
#3937=FACE_OUTER_BOUND('',#4967,.T.);
#3938=FACE_OUTER_BOUND('',#4968,.T.);
#3939=FACE_OUTER_BOUND('',#4969,.T.);
#3940=FACE_OUTER_BOUND('',#4970,.T.);
#3941=FACE_OUTER_BOUND('',#4971,.T.);
#3942=FACE_OUTER_BOUND('',#4972,.T.);
#3943=FACE_OUTER_BOUND('',#4973,.T.);
#3944=FACE_OUTER_BOUND('',#4974,.T.);
#3945=FACE_OUTER_BOUND('',#4975,.T.);
#3946=FACE_OUTER_BOUND('',#4976,.T.);
#3947=FACE_OUTER_BOUND('',#4977,.T.);
#3948=FACE_OUTER_BOUND('',#4978,.T.);
#3949=FACE_OUTER_BOUND('',#4979,.T.);
#3950=FACE_OUTER_BOUND('',#4980,.T.);
#3951=FACE_OUTER_BOUND('',#4981,.T.);
#3952=FACE_OUTER_BOUND('',#4982,.T.);
#3953=FACE_OUTER_BOUND('',#4983,.T.);
#3954=FACE_OUTER_BOUND('',#4984,.T.);
#3955=FACE_OUTER_BOUND('',#4985,.T.);
#3956=FACE_OUTER_BOUND('',#4986,.T.);
#3957=FACE_OUTER_BOUND('',#4987,.T.);
#3958=FACE_OUTER_BOUND('',#4988,.T.);
#3959=FACE_OUTER_BOUND('',#4989,.T.);
#3960=FACE_OUTER_BOUND('',#4990,.T.);
#3961=FACE_OUTER_BOUND('',#4991,.T.);
#3962=FACE_OUTER_BOUND('',#4992,.T.);
#3963=FACE_OUTER_BOUND('',#4993,.T.);
#3964=FACE_OUTER_BOUND('',#4994,.T.);
#3965=FACE_OUTER_BOUND('',#4995,.T.);
#3966=FACE_OUTER_BOUND('',#4996,.T.);
#3967=FACE_OUTER_BOUND('',#4997,.T.);
#3968=FACE_OUTER_BOUND('',#4998,.T.);
#3969=FACE_OUTER_BOUND('',#4999,.T.);
#3970=FACE_OUTER_BOUND('',#5000,.T.);
#3971=FACE_OUTER_BOUND('',#5001,.T.);
#3972=FACE_OUTER_BOUND('',#5002,.T.);
#3973=FACE_OUTER_BOUND('',#5003,.T.);
#3974=FACE_OUTER_BOUND('',#5004,.T.);
#3975=FACE_OUTER_BOUND('',#5005,.T.);
#3976=FACE_OUTER_BOUND('',#5006,.T.);
#3977=FACE_OUTER_BOUND('',#5007,.T.);
#3978=FACE_OUTER_BOUND('',#5008,.T.);
#3979=FACE_OUTER_BOUND('',#5009,.T.);
#3980=FACE_OUTER_BOUND('',#5010,.T.);
#3981=FACE_OUTER_BOUND('',#5011,.T.);
#3982=FACE_OUTER_BOUND('',#5012,.T.);
#3983=FACE_OUTER_BOUND('',#5013,.T.);
#3984=FACE_OUTER_BOUND('',#5014,.T.);
#3985=FACE_OUTER_BOUND('',#5015,.T.);
#3986=FACE_OUTER_BOUND('',#5016,.T.);
#3987=FACE_OUTER_BOUND('',#5017,.T.);
#3988=FACE_OUTER_BOUND('',#5018,.T.);
#3989=FACE_OUTER_BOUND('',#5019,.T.);
#3990=FACE_OUTER_BOUND('',#5020,.T.);
#3991=FACE_OUTER_BOUND('',#5021,.T.);
#3992=FACE_OUTER_BOUND('',#5022,.T.);
#3993=FACE_OUTER_BOUND('',#5023,.T.);
#3994=FACE_OUTER_BOUND('',#5024,.T.);
#3995=FACE_OUTER_BOUND('',#5025,.T.);
#3996=FACE_OUTER_BOUND('',#5026,.T.);
#3997=FACE_OUTER_BOUND('',#5027,.T.);
#3998=FACE_OUTER_BOUND('',#5028,.T.);
#3999=FACE_OUTER_BOUND('',#5029,.T.);
#4000=FACE_OUTER_BOUND('',#5030,.T.);
#4001=FACE_OUTER_BOUND('',#5031,.T.);
#4002=FACE_OUTER_BOUND('',#5032,.T.);
#4003=FACE_OUTER_BOUND('',#5033,.T.);
#4004=FACE_OUTER_BOUND('',#5034,.T.);
#4005=FACE_OUTER_BOUND('',#5035,.T.);
#4006=FACE_OUTER_BOUND('',#5036,.T.);
#4007=FACE_OUTER_BOUND('',#5037,.T.);
#4008=FACE_OUTER_BOUND('',#5038,.T.);
#4009=FACE_OUTER_BOUND('',#5039,.T.);
#4010=FACE_OUTER_BOUND('',#5040,.T.);
#4011=FACE_OUTER_BOUND('',#5041,.T.);
#4012=FACE_OUTER_BOUND('',#5042,.T.);
#4013=FACE_OUTER_BOUND('',#5043,.T.);
#4014=FACE_OUTER_BOUND('',#5044,.T.);
#4015=FACE_OUTER_BOUND('',#5045,.T.);
#4016=FACE_OUTER_BOUND('',#5046,.T.);
#4017=FACE_OUTER_BOUND('',#5047,.T.);
#4018=FACE_OUTER_BOUND('',#5048,.T.);
#4019=FACE_OUTER_BOUND('',#5049,.T.);
#4020=FACE_OUTER_BOUND('',#5050,.T.);
#4021=FACE_OUTER_BOUND('',#5051,.T.);
#4022=FACE_OUTER_BOUND('',#5052,.T.);
#4023=FACE_OUTER_BOUND('',#5053,.T.);
#4024=FACE_OUTER_BOUND('',#5054,.T.);
#4025=FACE_OUTER_BOUND('',#5055,.T.);
#4026=FACE_OUTER_BOUND('',#5056,.T.);
#4027=FACE_OUTER_BOUND('',#5057,.T.);
#4028=FACE_OUTER_BOUND('',#5058,.T.);
#4029=FACE_OUTER_BOUND('',#5059,.T.);
#4030=FACE_OUTER_BOUND('',#5060,.T.);
#4031=FACE_OUTER_BOUND('',#5061,.T.);
#4032=FACE_OUTER_BOUND('',#5062,.T.);
#4033=FACE_OUTER_BOUND('',#5063,.T.);
#4034=FACE_OUTER_BOUND('',#5064,.T.);
#4035=FACE_OUTER_BOUND('',#5065,.T.);
#4036=FACE_OUTER_BOUND('',#5066,.T.);
#4037=FACE_OUTER_BOUND('',#5067,.T.);
#4038=FACE_OUTER_BOUND('',#5068,.T.);
#4039=FACE_OUTER_BOUND('',#5069,.T.);
#4040=FACE_OUTER_BOUND('',#5070,.T.);
#4041=FACE_OUTER_BOUND('',#5071,.T.);
#4042=FACE_OUTER_BOUND('',#5072,.T.);
#4043=FACE_OUTER_BOUND('',#5073,.T.);
#4044=FACE_OUTER_BOUND('',#5074,.T.);
#4045=FACE_OUTER_BOUND('',#5075,.T.);
#4046=FACE_OUTER_BOUND('',#5076,.T.);
#4047=FACE_OUTER_BOUND('',#5077,.T.);
#4048=FACE_OUTER_BOUND('',#5078,.T.);
#4049=FACE_OUTER_BOUND('',#5079,.T.);
#4050=FACE_OUTER_BOUND('',#5080,.T.);
#4051=FACE_OUTER_BOUND('',#5081,.T.);
#4052=FACE_OUTER_BOUND('',#5082,.T.);
#4053=FACE_OUTER_BOUND('',#5083,.T.);
#4054=FACE_OUTER_BOUND('',#5084,.T.);
#4055=FACE_OUTER_BOUND('',#5085,.T.);
#4056=FACE_OUTER_BOUND('',#5086,.T.);
#4057=FACE_OUTER_BOUND('',#5087,.T.);
#4058=FACE_OUTER_BOUND('',#5088,.T.);
#4059=FACE_OUTER_BOUND('',#5089,.T.);
#4060=FACE_OUTER_BOUND('',#5090,.T.);
#4061=FACE_OUTER_BOUND('',#5091,.T.);
#4062=FACE_OUTER_BOUND('',#5092,.T.);
#4063=FACE_OUTER_BOUND('',#5093,.T.);
#4064=FACE_OUTER_BOUND('',#5094,.T.);
#4065=FACE_OUTER_BOUND('',#5095,.T.);
#4066=FACE_OUTER_BOUND('',#5096,.T.);
#4067=FACE_OUTER_BOUND('',#5097,.T.);
#4068=FACE_OUTER_BOUND('',#5098,.T.);
#4069=FACE_OUTER_BOUND('',#5099,.T.);
#4070=FACE_OUTER_BOUND('',#5100,.T.);
#4071=FACE_OUTER_BOUND('',#5101,.T.);
#4072=FACE_OUTER_BOUND('',#5102,.T.);
#4073=FACE_OUTER_BOUND('',#5103,.T.);
#4074=FACE_OUTER_BOUND('',#5104,.T.);
#4075=FACE_OUTER_BOUND('',#5105,.T.);
#4076=FACE_OUTER_BOUND('',#5106,.T.);
#4077=FACE_OUTER_BOUND('',#5107,.T.);
#4078=FACE_OUTER_BOUND('',#5108,.T.);
#4079=FACE_OUTER_BOUND('',#5109,.T.);
#4080=FACE_OUTER_BOUND('',#5110,.T.);
#4081=FACE_OUTER_BOUND('',#5111,.T.);
#4082=FACE_OUTER_BOUND('',#5112,.T.);
#4083=FACE_OUTER_BOUND('',#5113,.T.);
#4084=FACE_OUTER_BOUND('',#5114,.T.);
#4085=FACE_OUTER_BOUND('',#5115,.T.);
#4086=FACE_OUTER_BOUND('',#5116,.T.);
#4087=FACE_OUTER_BOUND('',#5117,.T.);
#4088=FACE_OUTER_BOUND('',#5118,.T.);
#4089=FACE_OUTER_BOUND('',#5119,.T.);
#4090=FACE_OUTER_BOUND('',#5120,.T.);
#4091=FACE_OUTER_BOUND('',#5121,.T.);
#4092=FACE_OUTER_BOUND('',#5122,.T.);
#4093=FACE_OUTER_BOUND('',#5123,.T.);
#4094=FACE_OUTER_BOUND('',#5124,.T.);
#4095=FACE_OUTER_BOUND('',#5125,.T.);
#4096=FACE_OUTER_BOUND('',#5126,.T.);
#4097=FACE_OUTER_BOUND('',#5127,.T.);
#4098=FACE_OUTER_BOUND('',#5128,.T.);
#4099=FACE_OUTER_BOUND('',#5129,.T.);
#4100=FACE_OUTER_BOUND('',#5130,.T.);
#4101=FACE_OUTER_BOUND('',#5131,.T.);
#4102=FACE_OUTER_BOUND('',#5132,.T.);
#4103=FACE_OUTER_BOUND('',#5133,.T.);
#4104=FACE_OUTER_BOUND('',#5134,.T.);
#4105=FACE_OUTER_BOUND('',#5135,.T.);
#4106=FACE_OUTER_BOUND('',#5136,.T.);
#4107=FACE_OUTER_BOUND('',#5137,.T.);
#4108=FACE_OUTER_BOUND('',#5138,.T.);
#4109=FACE_OUTER_BOUND('',#5139,.T.);
#4110=FACE_OUTER_BOUND('',#5140,.T.);
#4111=FACE_OUTER_BOUND('',#5141,.T.);
#4112=FACE_OUTER_BOUND('',#5142,.T.);
#4113=FACE_OUTER_BOUND('',#5143,.T.);
#4114=FACE_OUTER_BOUND('',#5144,.T.);
#4115=FACE_OUTER_BOUND('',#5145,.T.);
#4116=FACE_OUTER_BOUND('',#5146,.T.);
#4117=FACE_OUTER_BOUND('',#5147,.T.);
#4118=FACE_OUTER_BOUND('',#5148,.T.);
#4119=FACE_OUTER_BOUND('',#5149,.T.);
#4120=FACE_OUTER_BOUND('',#5150,.T.);
#4121=FACE_OUTER_BOUND('',#5151,.T.);
#4122=FACE_OUTER_BOUND('',#5152,.T.);
#4123=FACE_OUTER_BOUND('',#5153,.T.);
#4124=FACE_OUTER_BOUND('',#5154,.T.);
#4125=FACE_OUTER_BOUND('',#5155,.T.);
#4126=FACE_OUTER_BOUND('',#5156,.T.);
#4127=FACE_OUTER_BOUND('',#5157,.T.);
#4128=FACE_OUTER_BOUND('',#5158,.T.);
#4129=FACE_OUTER_BOUND('',#5159,.T.);
#4130=FACE_OUTER_BOUND('',#5160,.T.);
#4131=FACE_OUTER_BOUND('',#5161,.T.);
#4132=FACE_OUTER_BOUND('',#5162,.T.);
#4133=FACE_OUTER_BOUND('',#5163,.T.);
#4134=FACE_OUTER_BOUND('',#5164,.T.);
#4135=FACE_OUTER_BOUND('',#5165,.T.);
#4136=FACE_OUTER_BOUND('',#5166,.T.);
#4792=EDGE_LOOP('',(#12417,#12418,#12419,#12420,#12421,#12422,#12423));
#4793=EDGE_LOOP('',(#12424,#12425,#12426,#12427,#12428,#12429,#12430,#12431,
#12432,#12433,#12434,#12435,#12436,#12437));
#4794=EDGE_LOOP('',(#12438,#12439,#12440,#12441,#12442,#12443,#12444,#12445,
#12446,#12447,#12448,#12449,#12450,#12451,#12452,#12453,#12454,#12455,#12456,
#12457,#12458,#12459,#12460,#12461,#12462,#12463,#12464,#12465,#12466,#12467,
#12468,#12469,#12470,#12471,#12472,#12473,#12474,#12475,#12476,#12477,#12478,
#12479,#12480,#12481,#12482,#12483,#12484,#12485,#12486,#12487,#12488,#12489,
#12490,#12491,#12492,#12493,#12494,#12495,#12496,#12497,#12498,#12499,#12500,
#12501,#12502,#12503,#12504,#12505,#12506,#12507,#12508,#12509,#12510,#12511,
#12512,#12513,#12514,#12515,#12516,#12517,#12518,#12519,#12520,#12521,#12522,
#12523,#12524,#12525,#12526,#12527,#12528,#12529,#12530,#12531,#12532,#12533,
#12534,#12535,#12536,#12537,#12538,#12539,#12540,#12541,#12542,#12543,#12544,
#12545,#12546,#12547,#12548,#12549,#12550,#12551,#12552,#12553,#12554,#12555,
#12556,#12557,#12558,#12559,#12560,#12561,#12562,#12563,#12564,#12565,#12566,
#12567,#12568,#12569,#12570,#12571,#12572,#12573,#12574,#12575,#12576));
#4795=EDGE_LOOP('',(#12577,#12578,#12579,#12580,#12581,#12582,#12583,#12584,
#12585,#12586,#12587,#12588,#12589,#12590,#12591,#12592,#12593,#12594,#12595,
#12596,#12597,#12598,#12599,#12600,#12601,#12602,#12603,#12604,#12605,#12606,
#12607,#12608,#12609,#12610,#12611,#12612,#12613));
#4796=EDGE_LOOP('',(#12614,#12615,#12616,#12617));
#4797=EDGE_LOOP('',(#12618,#12619,#12620,#12621));
#4798=EDGE_LOOP('',(#12622,#12623,#12624,#12625,#12626,#12627));
#4799=EDGE_LOOP('',(#12628,#12629,#12630,#12631));
#4800=EDGE_LOOP('',(#12632,#12633,#12634,#12635,#12636,#12637,#12638,#12639,
#12640,#12641,#12642,#12643,#12644,#12645,#12646,#12647,#12648,#12649,#12650,
#12651,#12652,#12653,#12654,#12655,#12656,#12657,#12658,#12659,#12660,#12661,
#12662,#12663,#12664,#12665,#12666,#12667,#12668,#12669,#12670,#12671,#12672,
#12673,#12674,#12675,#12676,#12677,#12678,#12679,#12680,#12681,#12682,#12683,
#12684,#12685,#12686,#12687,#12688,#12689,#12690,#12691,#12692,#12693,#12694,
#12695,#12696,#12697,#12698,#12699,#12700,#12701,#12702,#12703,#12704,#12705,
#12706,#12707,#12708,#12709,#12710,#12711,#12712,#12713,#12714,#12715,#12716,
#12717,#12718,#12719,#12720,#12721,#12722,#12723,#12724,#12725,#12726,#12727,
#12728,#12729,#12730,#12731,#12732,#12733,#12734,#12735,#12736,#12737,#12738,
#12739,#12740,#12741,#12742,#12743,#12744,#12745,#12746,#12747,#12748,#12749,
#12750,#12751,#12752,#12753,#12754,#12755,#12756,#12757,#12758,#12759,#12760,
#12761,#12762,#12763));
#4801=EDGE_LOOP('',(#12764,#12765,#12766,#12767,#12768,#12769));
#4802=EDGE_LOOP('',(#12770,#12771,#12772,#12773,#12774,#12775));
#4803=EDGE_LOOP('',(#12776,#12777,#12778,#12779,#12780,#12781));
#4804=EDGE_LOOP('',(#12782,#12783,#12784,#12785,#12786,#12787));
#4805=EDGE_LOOP('',(#12788,#12789,#12790,#12791,#12792,#12793));
#4806=EDGE_LOOP('',(#12794,#12795,#12796,#12797,#12798,#12799));
#4807=EDGE_LOOP('',(#12800,#12801,#12802,#12803,#12804,#12805,#12806,#12807,
#12808,#12809));
#4808=EDGE_LOOP('',(#12810,#12811,#12812,#12813,#12814,#12815));
#4809=EDGE_LOOP('',(#12816,#12817,#12818,#12819,#12820,#12821));
#4810=EDGE_LOOP('',(#12822,#12823,#12824,#12825,#12826,#12827));
#4811=EDGE_LOOP('',(#12828,#12829,#12830,#12831,#12832,#12833));
#4812=EDGE_LOOP('',(#12834,#12835,#12836,#12837,#12838,#12839));
#4813=EDGE_LOOP('',(#12840,#12841,#12842,#12843,#12844,#12845,#12846,#12847,
#12848,#12849));
#4814=EDGE_LOOP('',(#12850,#12851,#12852,#12853,#12854,#12855,#12856,#12857,
#12858,#12859));
#4815=EDGE_LOOP('',(#12860,#12861,#12862,#12863,#12864,#12865,#12866,#12867,
#12868,#12869,#12870,#12871));
#4816=EDGE_LOOP('',(#12872,#12873,#12874,#12875,#12876,#12877,#12878,#12879));
#4817=EDGE_LOOP('',(#12880,#12881,#12882,#12883,#12884,#12885,#12886,#12887,
#12888,#12889,#12890));
#4818=EDGE_LOOP('',(#12891,#12892,#12893,#12894));
#4819=EDGE_LOOP('',(#12895,#12896,#12897,#12898));
#4820=EDGE_LOOP('',(#12899,#12900,#12901,#12902));
#4821=EDGE_LOOP('',(#12903,#12904,#12905,#12906));
#4822=EDGE_LOOP('',(#12907,#12908,#12909,#12910,#12911));
#4823=EDGE_LOOP('',(#12912,#12913,#12914,#12915,#12916));
#4824=EDGE_LOOP('',(#12917,#12918,#12919,#12920,#12921));
#4825=EDGE_LOOP('',(#12922,#12923,#12924,#12925,#12926));
#4826=EDGE_LOOP('',(#12927,#12928,#12929,#12930));
#4827=EDGE_LOOP('',(#12931,#12932,#12933,#12934,#12935,#12936,#12937,#12938,
#12939,#12940,#12941,#12942,#12943,#12944,#12945,#12946,#12947));
#4828=EDGE_LOOP('',(#12948,#12949,#12950,#12951,#12952,#12953,#12954));
#4829=EDGE_LOOP('',(#12955,#12956,#12957,#12958,#12959,#12960));
#4830=EDGE_LOOP('',(#12961,#12962,#12963,#12964,#12965,#12966));
#4831=EDGE_LOOP('',(#12967,#12968,#12969,#12970,#12971,#12972,#12973));
#4832=EDGE_LOOP('',(#12974,#12975,#12976,#12977,#12978,#12979,#12980));
#4833=EDGE_LOOP('',(#12981,#12982,#12983,#12984,#12985,#12986,#12987,#12988,
#12989,#12990,#12991,#12992));
#4834=EDGE_LOOP('',(#12993,#12994,#12995,#12996,#12997,#12998,#12999,#13000,
#13001,#13002,#13003,#13004));
#4835=EDGE_LOOP('',(#13005,#13006,#13007,#13008,#13009,#13010,#13011));
#4836=EDGE_LOOP('',(#13012,#13013,#13014,#13015));
#4837=EDGE_LOOP('',(#13016,#13017,#13018,#13019));
#4838=EDGE_LOOP('',(#13020,#13021,#13022,#13023));
#4839=EDGE_LOOP('',(#13024,#13025,#13026,#13027));
#4840=EDGE_LOOP('',(#13028,#13029,#13030,#13031,#13032));
#4841=EDGE_LOOP('',(#13033,#13034,#13035,#13036));
#4842=EDGE_LOOP('',(#13037,#13038,#13039,#13040));
#4843=EDGE_LOOP('',(#13041,#13042,#13043,#13044,#13045,#13046,#13047));
#4844=EDGE_LOOP('',(#13048,#13049,#13050,#13051,#13052));
#4845=EDGE_LOOP('',(#13053,#13054,#13055,#13056));
#4846=EDGE_LOOP('',(#13057,#13058,#13059,#13060));
#4847=EDGE_LOOP('',(#13061,#13062,#13063,#13064,#13065));
#4848=EDGE_LOOP('',(#13066,#13067,#13068,#13069,#13070));
#4849=EDGE_LOOP('',(#13071,#13072,#13073,#13074));
#4850=EDGE_LOOP('',(#13075,#13076,#13077,#13078));
#4851=EDGE_LOOP('',(#13079,#13080,#13081,#13082,#13083,#13084));
#4852=EDGE_LOOP('',(#13085,#13086,#13087,#13088,#13089));
#4853=EDGE_LOOP('',(#13090,#13091,#13092,#13093,#13094,#13095,#13096,#13097));
#4854=EDGE_LOOP('',(#13098,#13099,#13100,#13101,#13102,#13103,#13104,#13105,
#13106));
#4855=EDGE_LOOP('',(#13107,#13108,#13109,#13110,#13111));
#4856=EDGE_LOOP('',(#13112,#13113,#13114));
#4857=EDGE_LOOP('',(#13115,#13116,#13117,#13118));
#4858=EDGE_LOOP('',(#13119,#13120,#13121,#13122,#13123));
#4859=EDGE_LOOP('',(#13124,#13125,#13126,#13127,#13128,#13129));
#4860=EDGE_LOOP('',(#13130,#13131,#13132,#13133,#13134));
#4861=EDGE_LOOP('',(#13135,#13136,#13137,#13138,#13139));
#4862=EDGE_LOOP('',(#13140,#13141,#13142,#13143));
#4863=EDGE_LOOP('',(#13144,#13145,#13146,#13147));
#4864=EDGE_LOOP('',(#13148,#13149,#13150,#13151));
#4865=EDGE_LOOP('',(#13152,#13153,#13154));
#4866=EDGE_LOOP('',(#13155,#13156,#13157,#13158));
#4867=EDGE_LOOP('',(#13159,#13160,#13161,#13162));
#4868=EDGE_LOOP('',(#13163,#13164,#13165));
#4869=EDGE_LOOP('',(#13166,#13167,#13168,#13169));
#4870=EDGE_LOOP('',(#13170,#13171,#13172));
#4871=EDGE_LOOP('',(#13173,#13174,#13175,#13176));
#4872=EDGE_LOOP('',(#13177,#13178,#13179,#13180));
#4873=EDGE_LOOP('',(#13181,#13182,#13183,#13184,#13185,#13186,#13187));
#4874=EDGE_LOOP('',(#13188,#13189,#13190,#13191,#13192));
#4875=EDGE_LOOP('',(#13193,#13194,#13195,#13196,#13197));
#4876=EDGE_LOOP('',(#13198,#13199,#13200));
#4877=EDGE_LOOP('',(#13201,#13202,#13203,#13204));
#4878=EDGE_LOOP('',(#13205,#13206,#13207));
#4879=EDGE_LOOP('',(#13208,#13209,#13210,#13211,#13212,#13213,#13214,#13215,
#13216,#13217));
#4880=EDGE_LOOP('',(#13218,#13219,#13220,#13221,#13222,#13223,#13224));
#4881=EDGE_LOOP('',(#13225,#13226,#13227,#13228,#13229,#13230,#13231));
#4882=EDGE_LOOP('',(#13232,#13233,#13234,#13235,#13236,#13237,#13238,#13239));
#4883=EDGE_LOOP('',(#13240,#13241,#13242,#13243));
#4884=EDGE_LOOP('',(#13244,#13245,#13246,#13247,#13248,#13249,#13250,#13251));
#4885=EDGE_LOOP('',(#13252,#13253,#13254,#13255,#13256,#13257));
#4886=EDGE_LOOP('',(#13258,#13259,#13260,#13261,#13262,#13263));
#4887=EDGE_LOOP('',(#13264,#13265,#13266,#13267,#13268,#13269));
#4888=EDGE_LOOP('',(#13270,#13271,#13272,#13273,#13274,#13275));
#4889=EDGE_LOOP('',(#13276,#13277,#13278,#13279,#13280,#13281));
#4890=EDGE_LOOP('',(#13282,#13283,#13284,#13285,#13286,#13287));
#4891=EDGE_LOOP('',(#13288,#13289,#13290,#13291,#13292,#13293));
#4892=EDGE_LOOP('',(#13294,#13295,#13296,#13297,#13298,#13299));
#4893=EDGE_LOOP('',(#13300,#13301,#13302,#13303,#13304,#13305));
#4894=EDGE_LOOP('',(#13306,#13307,#13308,#13309,#13310,#13311));
#4895=EDGE_LOOP('',(#13312,#13313,#13314,#13315,#13316,#13317));
#4896=EDGE_LOOP('',(#13318,#13319,#13320,#13321,#13322,#13323));
#4897=EDGE_LOOP('',(#13324,#13325,#13326,#13327,#13328,#13329));
#4898=EDGE_LOOP('',(#13330,#13331,#13332,#13333,#13334,#13335));
#4899=EDGE_LOOP('',(#13336,#13337,#13338,#13339,#13340,#13341));
#4900=EDGE_LOOP('',(#13342,#13343,#13344,#13345,#13346,#13347));
#4901=EDGE_LOOP('',(#13348,#13349,#13350,#13351,#13352,#13353));
#4902=EDGE_LOOP('',(#13354,#13355,#13356,#13357));
#4903=EDGE_LOOP('',(#13358,#13359,#13360,#13361));
#4904=EDGE_LOOP('',(#13362,#13363,#13364,#13365,#13366,#13367));
#4905=EDGE_LOOP('',(#13368,#13369,#13370,#13371,#13372,#13373));
#4906=EDGE_LOOP('',(#13374,#13375,#13376,#13377,#13378,#13379));
#4907=EDGE_LOOP('',(#13380,#13381,#13382,#13383,#13384,#13385));
#4908=EDGE_LOOP('',(#13386,#13387,#13388,#13389,#13390,#13391));
#4909=EDGE_LOOP('',(#13392,#13393,#13394,#13395,#13396,#13397));
#4910=EDGE_LOOP('',(#13398,#13399,#13400,#13401,#13402,#13403));
#4911=EDGE_LOOP('',(#13404,#13405,#13406,#13407,#13408,#13409));
#4912=EDGE_LOOP('',(#13410,#13411,#13412,#13413,#13414,#13415));
#4913=EDGE_LOOP('',(#13416,#13417,#13418,#13419,#13420,#13421));
#4914=EDGE_LOOP('',(#13422,#13423,#13424,#13425,#13426,#13427));
#4915=EDGE_LOOP('',(#13428,#13429,#13430,#13431,#13432,#13433));
#4916=EDGE_LOOP('',(#13434,#13435,#13436,#13437,#13438,#13439));
#4917=EDGE_LOOP('',(#13440,#13441,#13442,#13443,#13444,#13445));
#4918=EDGE_LOOP('',(#13446,#13447,#13448,#13449,#13450,#13451));
#4919=EDGE_LOOP('',(#13452,#13453,#13454,#13455,#13456,#13457));
#4920=EDGE_LOOP('',(#13458,#13459,#13460,#13461,#13462,#13463));
#4921=EDGE_LOOP('',(#13464,#13465,#13466,#13467));
#4922=EDGE_LOOP('',(#13468,#13469,#13470,#13471));
#4923=EDGE_LOOP('',(#13472,#13473,#13474,#13475));
#4924=EDGE_LOOP('',(#13476,#13477,#13478,#13479));
#4925=EDGE_LOOP('',(#13480,#13481,#13482,#13483));
#4926=EDGE_LOOP('',(#13484,#13485,#13486,#13487));
#4927=EDGE_LOOP('',(#13488,#13489,#13490,#13491));
#4928=EDGE_LOOP('',(#13492,#13493,#13494,#13495));
#4929=EDGE_LOOP('',(#13496,#13497,#13498,#13499));
#4930=EDGE_LOOP('',(#13500,#13501,#13502,#13503));
#4931=EDGE_LOOP('',(#13504,#13505,#13506,#13507));
#4932=EDGE_LOOP('',(#13508,#13509,#13510,#13511));
#4933=EDGE_LOOP('',(#13512,#13513,#13514,#13515));
#4934=EDGE_LOOP('',(#13516,#13517,#13518,#13519));
#4935=EDGE_LOOP('',(#13520,#13521,#13522,#13523));
#4936=EDGE_LOOP('',(#13524,#13525,#13526,#13527));
#4937=EDGE_LOOP('',(#13528,#13529,#13530,#13531));
#4938=EDGE_LOOP('',(#13532,#13533,#13534,#13535));
#4939=EDGE_LOOP('',(#13536,#13537,#13538,#13539));
#4940=EDGE_LOOP('',(#13540,#13541,#13542,#13543));
#4941=EDGE_LOOP('',(#13544,#13545,#13546,#13547));
#4942=EDGE_LOOP('',(#13548,#13549,#13550,#13551));
#4943=EDGE_LOOP('',(#13552,#13553,#13554,#13555));
#4944=EDGE_LOOP('',(#13556,#13557,#13558,#13559));
#4945=EDGE_LOOP('',(#13560,#13561,#13562,#13563));
#4946=EDGE_LOOP('',(#13564,#13565,#13566,#13567));
#4947=EDGE_LOOP('',(#13568,#13569,#13570,#13571));
#4948=EDGE_LOOP('',(#13572,#13573,#13574,#13575));
#4949=EDGE_LOOP('',(#13576,#13577,#13578,#13579));
#4950=EDGE_LOOP('',(#13580,#13581,#13582,#13583));
#4951=EDGE_LOOP('',(#13584,#13585,#13586,#13587));
#4952=EDGE_LOOP('',(#13588,#13589,#13590,#13591));
#4953=EDGE_LOOP('',(#13592,#13593,#13594,#13595));
#4954=EDGE_LOOP('',(#13596,#13597,#13598,#13599));
#4955=EDGE_LOOP('',(#13600,#13601,#13602,#13603));
#4956=EDGE_LOOP('',(#13604,#13605,#13606,#13607));
#4957=EDGE_LOOP('',(#13608,#13609,#13610,#13611));
#4958=EDGE_LOOP('',(#13612,#13613,#13614,#13615));
#4959=EDGE_LOOP('',(#13616,#13617,#13618,#13619,#13620));
#4960=EDGE_LOOP('',(#13621,#13622,#13623,#13624));
#4961=EDGE_LOOP('',(#13625,#13626,#13627,#13628,#13629));
#4962=EDGE_LOOP('',(#13630,#13631,#13632,#13633,#13634));
#4963=EDGE_LOOP('',(#13635,#13636,#13637,#13638));
#4964=EDGE_LOOP('',(#13639,#13640,#13641,#13642,#13643));
#4965=EDGE_LOOP('',(#13644,#13645,#13646,#13647));
#4966=EDGE_LOOP('',(#13648,#13649,#13650,#13651));
#4967=EDGE_LOOP('',(#13652,#13653,#13654,#13655));
#4968=EDGE_LOOP('',(#13656,#13657,#13658,#13659));
#4969=EDGE_LOOP('',(#13660,#13661,#13662,#13663));
#4970=EDGE_LOOP('',(#13664,#13665,#13666,#13667));
#4971=EDGE_LOOP('',(#13668,#13669,#13670,#13671));
#4972=EDGE_LOOP('',(#13672,#13673,#13674,#13675));
#4973=EDGE_LOOP('',(#13676,#13677,#13678,#13679));
#4974=EDGE_LOOP('',(#13680,#13681,#13682,#13683));
#4975=EDGE_LOOP('',(#13684,#13685,#13686,#13687));
#4976=EDGE_LOOP('',(#13688,#13689,#13690,#13691));
#4977=EDGE_LOOP('',(#13692,#13693,#13694,#13695));
#4978=EDGE_LOOP('',(#13696,#13697,#13698,#13699));
#4979=EDGE_LOOP('',(#13700,#13701,#13702,#13703));
#4980=EDGE_LOOP('',(#13704,#13705,#13706,#13707));
#4981=EDGE_LOOP('',(#13708,#13709,#13710,#13711));
#4982=EDGE_LOOP('',(#13712,#13713,#13714,#13715));
#4983=EDGE_LOOP('',(#13716,#13717,#13718,#13719));
#4984=EDGE_LOOP('',(#13720,#13721,#13722,#13723));
#4985=EDGE_LOOP('',(#13724,#13725,#13726,#13727));
#4986=EDGE_LOOP('',(#13728,#13729,#13730,#13731));
#4987=EDGE_LOOP('',(#13732,#13733,#13734,#13735));
#4988=EDGE_LOOP('',(#13736,#13737,#13738,#13739));
#4989=EDGE_LOOP('',(#13740,#13741,#13742,#13743));
#4990=EDGE_LOOP('',(#13744,#13745,#13746,#13747));
#4991=EDGE_LOOP('',(#13748,#13749,#13750,#13751));
#4992=EDGE_LOOP('',(#13752,#13753,#13754,#13755));
#4993=EDGE_LOOP('',(#13756,#13757,#13758,#13759));
#4994=EDGE_LOOP('',(#13760,#13761,#13762,#13763));
#4995=EDGE_LOOP('',(#13764,#13765,#13766,#13767,#13768));
#4996=EDGE_LOOP('',(#13769,#13770,#13771,#13772));
#4997=EDGE_LOOP('',(#13773,#13774,#13775,#13776,#13777));
#4998=EDGE_LOOP('',(#13778,#13779,#13780,#13781,#13782));
#4999=EDGE_LOOP('',(#13783,#13784,#13785,#13786));
#5000=EDGE_LOOP('',(#13787,#13788,#13789,#13790,#13791));
#5001=EDGE_LOOP('',(#13792,#13793,#13794,#13795,#13796));
#5002=EDGE_LOOP('',(#13797,#13798,#13799,#13800));
#5003=EDGE_LOOP('',(#13801,#13802,#13803,#13804,#13805));
#5004=EDGE_LOOP('',(#13806,#13807,#13808,#13809,#13810));
#5005=EDGE_LOOP('',(#13811,#13812,#13813,#13814));
#5006=EDGE_LOOP('',(#13815,#13816,#13817,#13818,#13819));
#5007=EDGE_LOOP('',(#13820,#13821,#13822,#13823));
#5008=EDGE_LOOP('',(#13824,#13825,#13826,#13827));
#5009=EDGE_LOOP('',(#13828,#13829,#13830,#13831,#13832,#13833,#13834));
#5010=EDGE_LOOP('',(#13835,#13836,#13837,#13838,#13839));
#5011=EDGE_LOOP('',(#13840,#13841,#13842,#13843,#13844));
#5012=EDGE_LOOP('',(#13845,#13846,#13847,#13848,#13849));
#5013=EDGE_LOOP('',(#13850,#13851,#13852,#13853,#13854));
#5014=EDGE_LOOP('',(#13855,#13856,#13857,#13858));
#5015=EDGE_LOOP('',(#13859,#13860,#13861,#13862,#13863));
#5016=EDGE_LOOP('',(#13864,#13865,#13866,#13867));
#5017=EDGE_LOOP('',(#13868,#13869,#13870,#13871));
#5018=EDGE_LOOP('',(#13872,#13873,#13874,#13875));
#5019=EDGE_LOOP('',(#13876,#13877,#13878,#13879,#13880));
#5020=EDGE_LOOP('',(#13881,#13882,#13883,#13884));
#5021=EDGE_LOOP('',(#13885,#13886,#13887,#13888));
#5022=EDGE_LOOP('',(#13889,#13890,#13891,#13892,#13893,#13894,#13895));
#5023=EDGE_LOOP('',(#13896,#13897,#13898,#13899));
#5024=EDGE_LOOP('',(#13900,#13901,#13902,#13903,#13904));
#5025=EDGE_LOOP('',(#13905,#13906,#13907,#13908,#13909));
#5026=EDGE_LOOP('',(#13910,#13911,#13912,#13913));
#5027=EDGE_LOOP('',(#13914,#13915,#13916,#13917));
#5028=EDGE_LOOP('',(#13918,#13919,#13920,#13921));
#5029=EDGE_LOOP('',(#13922,#13923,#13924,#13925,#13926));
#5030=EDGE_LOOP('',(#13927,#13928,#13929,#13930));
#5031=EDGE_LOOP('',(#13931,#13932,#13933,#13934,#13935));
#5032=EDGE_LOOP('',(#13936,#13937,#13938,#13939));
#5033=EDGE_LOOP('',(#13940,#13941,#13942,#13943));
#5034=EDGE_LOOP('',(#13944,#13945,#13946,#13947));
#5035=EDGE_LOOP('',(#13948,#13949,#13950,#13951,#13952));
#5036=EDGE_LOOP('',(#13953,#13954,#13955,#13956));
#5037=EDGE_LOOP('',(#13957,#13958,#13959,#13960,#13961));
#5038=EDGE_LOOP('',(#13962,#13963,#13964,#13965));
#5039=EDGE_LOOP('',(#13966,#13967,#13968,#13969));
#5040=EDGE_LOOP('',(#13970,#13971,#13972,#13973));
#5041=EDGE_LOOP('',(#13974,#13975,#13976,#13977,#13978));
#5042=EDGE_LOOP('',(#13979,#13980,#13981,#13982));
#5043=EDGE_LOOP('',(#13983,#13984,#13985,#13986,#13987));
#5044=EDGE_LOOP('',(#13988,#13989,#13990,#13991));
#5045=EDGE_LOOP('',(#13992,#13993,#13994,#13995));
#5046=EDGE_LOOP('',(#13996,#13997,#13998,#13999));
#5047=EDGE_LOOP('',(#14000,#14001,#14002,#14003,#14004));
#5048=EDGE_LOOP('',(#14005,#14006,#14007,#14008));
#5049=EDGE_LOOP('',(#14009,#14010,#14011,#14012,#14013));
#5050=EDGE_LOOP('',(#14014,#14015,#14016,#14017));
#5051=EDGE_LOOP('',(#14018,#14019,#14020,#14021));
#5052=EDGE_LOOP('',(#14022,#14023,#14024,#14025));
#5053=EDGE_LOOP('',(#14026,#14027,#14028,#14029,#14030));
#5054=EDGE_LOOP('',(#14031,#14032,#14033,#14034));
#5055=EDGE_LOOP('',(#14035,#14036,#14037,#14038,#14039));
#5056=EDGE_LOOP('',(#14040,#14041,#14042,#14043));
#5057=EDGE_LOOP('',(#14044,#14045,#14046,#14047));
#5058=EDGE_LOOP('',(#14048,#14049,#14050,#14051));
#5059=EDGE_LOOP('',(#14052,#14053,#14054,#14055,#14056));
#5060=EDGE_LOOP('',(#14057,#14058,#14059,#14060));
#5061=EDGE_LOOP('',(#14061,#14062,#14063,#14064,#14065,#14066));
#5062=EDGE_LOOP('',(#14067,#14068,#14069,#14070,#14071));
#5063=EDGE_LOOP('',(#14072,#14073,#14074,#14075));
#5064=EDGE_LOOP('',(#14076,#14077,#14078,#14079));
#5065=EDGE_LOOP('',(#14080,#14081,#14082,#14083,#14084,#14085));
#5066=EDGE_LOOP('',(#14086,#14087,#14088,#14089,#14090));
#5067=EDGE_LOOP('',(#14091,#14092,#14093,#14094,#14095));
#5068=EDGE_LOOP('',(#14096,#14097,#14098,#14099));
#5069=EDGE_LOOP('',(#14100,#14101,#14102,#14103));
#5070=EDGE_LOOP('',(#14104,#14105,#14106,#14107));
#5071=EDGE_LOOP('',(#14108,#14109,#14110,#14111,#14112));
#5072=EDGE_LOOP('',(#14113,#14114,#14115,#14116));
#5073=EDGE_LOOP('',(#14117,#14118,#14119,#14120,#14121));
#5074=EDGE_LOOP('',(#14122,#14123,#14124,#14125));
#5075=EDGE_LOOP('',(#14126,#14127,#14128,#14129));
#5076=EDGE_LOOP('',(#14130,#14131,#14132,#14133));
#5077=EDGE_LOOP('',(#14134,#14135,#14136,#14137,#14138));
#5078=EDGE_LOOP('',(#14139,#14140,#14141,#14142));
#5079=EDGE_LOOP('',(#14143,#14144,#14145,#14146,#14147));
#5080=EDGE_LOOP('',(#14148,#14149,#14150,#14151));
#5081=EDGE_LOOP('',(#14152,#14153,#14154,#14155));
#5082=EDGE_LOOP('',(#14156,#14157,#14158,#14159));
#5083=EDGE_LOOP('',(#14160,#14161,#14162,#14163,#14164));
#5084=EDGE_LOOP('',(#14165,#14166,#14167,#14168));
#5085=EDGE_LOOP('',(#14169,#14170,#14171,#14172,#14173));
#5086=EDGE_LOOP('',(#14174,#14175,#14176,#14177));
#5087=EDGE_LOOP('',(#14178,#14179,#14180,#14181));
#5088=EDGE_LOOP('',(#14182,#14183,#14184,#14185));
#5089=EDGE_LOOP('',(#14186,#14187,#14188,#14189,#14190));
#5090=EDGE_LOOP('',(#14191,#14192,#14193,#14194));
#5091=EDGE_LOOP('',(#14195,#14196,#14197,#14198,#14199));
#5092=EDGE_LOOP('',(#14200,#14201,#14202,#14203));
#5093=EDGE_LOOP('',(#14204,#14205,#14206,#14207));
#5094=EDGE_LOOP('',(#14208,#14209,#14210,#14211));
#5095=EDGE_LOOP('',(#14212,#14213,#14214,#14215,#14216));
#5096=EDGE_LOOP('',(#14217,#14218,#14219,#14220));
#5097=EDGE_LOOP('',(#14221,#14222,#14223,#14224,#14225,#14226));
#5098=EDGE_LOOP('',(#14227,#14228,#14229,#14230,#14231));
#5099=EDGE_LOOP('',(#14232,#14233,#14234,#14235));
#5100=EDGE_LOOP('',(#14236,#14237,#14238,#14239));
#5101=EDGE_LOOP('',(#14240,#14241,#14242,#14243,#14244,#14245));
#5102=EDGE_LOOP('',(#14246,#14247,#14248,#14249,#14250));
#5103=EDGE_LOOP('',(#14251,#14252,#14253,#14254,#14255,#14256));
#5104=EDGE_LOOP('',(#14257,#14258,#14259,#14260,#14261));
#5105=EDGE_LOOP('',(#14262,#14263,#14264,#14265));
#5106=EDGE_LOOP('',(#14266,#14267,#14268,#14269));
#5107=EDGE_LOOP('',(#14270,#14271,#14272,#14273,#14274,#14275));
#5108=EDGE_LOOP('',(#14276,#14277,#14278,#14279,#14280));
#5109=EDGE_LOOP('',(#14281,#14282,#14283,#14284,#14285,#14286));
#5110=EDGE_LOOP('',(#14287,#14288,#14289,#14290,#14291));
#5111=EDGE_LOOP('',(#14292,#14293,#14294,#14295,#14296));
#5112=EDGE_LOOP('',(#14297,#14298,#14299,#14300,#14301));
#5113=EDGE_LOOP('',(#14302,#14303,#14304,#14305,#14306));
#5114=EDGE_LOOP('',(#14307,#14308,#14309,#14310,#14311,#14312,#14313));
#5115=EDGE_LOOP('',(#14314,#14315,#14316,#14317,#14318));
#5116=EDGE_LOOP('',(#14319,#14320,#14321,#14322));
#5117=EDGE_LOOP('',(#14323,#14324,#14325,#14326));
#5118=EDGE_LOOP('',(#14327,#14328,#14329,#14330));
#5119=EDGE_LOOP('',(#14331,#14332,#14333,#14334,#14335,#14336));
#5120=EDGE_LOOP('',(#14337,#14338,#14339,#14340,#14341));
#5121=EDGE_LOOP('',(#14342,#14343,#14344,#14345,#14346));
#5122=EDGE_LOOP('',(#14347,#14348,#14349,#14350));
#5123=EDGE_LOOP('',(#14351,#14352,#14353,#14354));
#5124=EDGE_LOOP('',(#14355,#14356,#14357,#14358,#14359,#14360,#14361,#14362));
#5125=EDGE_LOOP('',(#14363,#14364,#14365,#14366,#14367));
#5126=EDGE_LOOP('',(#14368,#14369,#14370,#14371,#14372));
#5127=EDGE_LOOP('',(#14373,#14374,#14375,#14376,#14377));
#5128=EDGE_LOOP('',(#14378,#14379,#14380,#14381));
#5129=EDGE_LOOP('',(#14382,#14383,#14384,#14385,#14386));
#5130=EDGE_LOOP('',(#14387,#14388,#14389,#14390));
#5131=EDGE_LOOP('',(#14391,#14392,#14393,#14394,#14395));
#5132=EDGE_LOOP('',(#14396,#14397,#14398,#14399));
#5133=EDGE_LOOP('',(#14400,#14401,#14402,#14403,#14404));
#5134=EDGE_LOOP('',(#14405,#14406,#14407,#14408));
#5135=EDGE_LOOP('',(#14409,#14410,#14411,#14412));
#5136=EDGE_LOOP('',(#14413,#14414,#14415,#14416,#14417,#14418));
#5137=EDGE_LOOP('',(#14419,#14420,#14421,#14422));
#5138=EDGE_LOOP('',(#14423,#14424,#14425,#14426));
#5139=EDGE_LOOP('',(#14427,#14428,#14429,#14430));
#5140=EDGE_LOOP('',(#14431,#14432,#14433,#14434));
#5141=EDGE_LOOP('',(#14435,#14436,#14437,#14438));
#5142=EDGE_LOOP('',(#14439,#14440,#14441,#14442,#14443,#14444));
#5143=EDGE_LOOP('',(#14445,#14446,#14447,#14448));
#5144=EDGE_LOOP('',(#14449,#14450,#14451,#14452));
#5145=EDGE_LOOP('',(#14453,#14454,#14455,#14456));
#5146=EDGE_LOOP('',(#14457,#14458,#14459,#14460));
#5147=EDGE_LOOP('',(#14461,#14462,#14463,#14464,#14465));
#5148=EDGE_LOOP('',(#14466,#14467,#14468,#14469));
#5149=EDGE_LOOP('',(#14470,#14471,#14472,#14473,#14474));
#5150=EDGE_LOOP('',(#14475,#14476,#14477,#14478));
#5151=EDGE_LOOP('',(#14479,#14480,#14481,#14482,#14483,#14484));
#5152=EDGE_LOOP('',(#14485,#14486,#14487,#14488));
#5153=EDGE_LOOP('',(#14489,#14490,#14491,#14492,#14493));
#5154=EDGE_LOOP('',(#14494,#14495,#14496,#14497,#14498));
#5155=EDGE_LOOP('',(#14499,#14500,#14501,#14502));
#5156=EDGE_LOOP('',(#14503,#14504,#14505,#14506,#14507,#14508));
#5157=EDGE_LOOP('',(#14509,#14510,#14511,#14512));
#5158=EDGE_LOOP('',(#14513,#14514,#14515,#14516,#14517));
#5159=EDGE_LOOP('',(#14518,#14519,#14520,#14521));
#5160=EDGE_LOOP('',(#14522,#14523,#14524,#14525));
#5161=EDGE_LOOP('',(#14526,#14527,#14528,#14529));
#5162=EDGE_LOOP('',(#14530,#14531,#14532,#14533,#14534));
#5163=EDGE_LOOP('',(#14535,#14536,#14537,#14538,#14539,#14540));
#5164=EDGE_LOOP('',(#14541,#14542,#14543,#14544,#14545,#14546));
#5165=EDGE_LOOP('',(#14547,#14548,#14549,#14550,#14551,#14552));
#5166=EDGE_LOOP('',(#14553,#14554,#14555,#14556));
#6071=CIRCLE('',#18521,0.00407884422956621);
#6072=CIRCLE('',#18522,0.00926353205762594);
#6073=CIRCLE('',#18523,0.00911324794481585);
#6074=CIRCLE('',#18524,0.00911756273482394);
#6075=CIRCLE('',#18526,0.00925178497204344);
#6076=CIRCLE('',#18527,0.00913306539255981);
#6077=CIRCLE('',#18528,0.00926684648530518);
#6078=CIRCLE('',#18529,0.0092508836596066);
#6079=CIRCLE('',#18532,0.00806904972011834);
#6080=CIRCLE('',#18534,0.00806904972011834);
#6081=CIRCLE('',#18537,0.00806904972011834);
#6082=CIRCLE('',#18539,0.00407884422956621);
#6083=CIRCLE('',#18540,0.00407884422999999);
#6084=CIRCLE('',#18541,0.00921926258718324);
#6085=CIRCLE('',#18542,0.00921925444913531);
#6086=CIRCLE('',#18553,0.00816904972011834);
#6087=CIRCLE('',#18556,0.00816904972011834);
#6088=CIRCLE('',#18558,0.00816904972011834);
#6089=CIRCLE('',#18559,9.9999992588795E-5);
#6090=CIRCLE('',#18560,9.99999925874768E-5);
#6091=CIRCLE('',#18563,0.000104492701428376);
#6092=CIRCLE('',#18564,0.0001);
#6093=CIRCLE('',#18567,0.0001);
#6094=CIRCLE('',#18568,0.0001);
#6095=CIRCLE('',#18570,0.000104493909288024);
#6096=CIRCLE('',#18571,9.99999925875666E-5);
#6097=CIRCLE('',#18573,0.000104492715876204);
#6098=CIRCLE('',#18574,9.99999925888095E-5);
#6099=CIRCLE('',#18578,0.0001);
#6100=CIRCLE('',#18580,0.0001);
#6101=CIRCLE('',#18582,9.99999969896661E-5);
#6102=CIRCLE('',#18583,9.99999999999991E-5);
#6103=CIRCLE('',#18584,0.000100000000000023);
#6104=CIRCLE('',#18586,9.99782235912355E-5);
#6105=CIRCLE('',#18587,0.0001);
#6106=CIRCLE('',#18590,0.0001);
#6107=CIRCLE('',#18593,0.0001);
#6108=CIRCLE('',#18595,0.0001);
#6109=CIRCLE('',#18597,0.0001);
#6110=CIRCLE('',#18601,0.0001);
#6111=CIRCLE('',#18602,9.99999999999974E-5);
#6112=CIRCLE('',#18604,9.99999969896684E-5);
#6113=CIRCLE('',#18606,0.0001);
#6114=CIRCLE('',#18608,0.0001);
#6115=CIRCLE('',#18611,9.99999999227393E-5);
#6116=CIRCLE('',#18612,9.99999999233536E-5);
#6117=CIRCLE('',#18613,9.99999999230291E-5);
#6118=CIRCLE('',#18614,9.99999999233779E-5);
#6119=CIRCLE('',#18617,0.00911255899884414);
#6120=CIRCLE('',#18618,0.00911585801383145);
#6972=VERTEX_POINT('',#26001);
#6973=VERTEX_POINT('',#26002);
#6974=VERTEX_POINT('',#26007);
#6975=VERTEX_POINT('',#26027);
#6976=VERTEX_POINT('',#26056);
#6977=VERTEX_POINT('',#26064);
#6978=VERTEX_POINT('',#26069);
#6979=VERTEX_POINT('',#26157);
#6980=VERTEX_POINT('',#26158);
#6981=VERTEX_POINT('',#26161);
#6982=VERTEX_POINT('',#26166);
#6983=VERTEX_POINT('',#26351);
#6984=VERTEX_POINT('',#26357);
#6985=VERTEX_POINT('',#26542);
#6986=VERTEX_POINT('',#26547);
#6987=VERTEX_POINT('',#26550);
#6988=VERTEX_POINT('',#26590);
#6989=VERTEX_POINT('',#26613);
#6990=VERTEX_POINT('',#26678);
#6991=VERTEX_POINT('',#26691);
#6992=VERTEX_POINT('',#26732);
#6993=VERTEX_POINT('',#26867);
#6994=VERTEX_POINT('',#26868);
#6995=VERTEX_POINT('',#26871);
#6996=VERTEX_POINT('',#26914);
#6997=VERTEX_POINT('',#26943);
#6998=VERTEX_POINT('',#26978);
#6999=VERTEX_POINT('',#27004);
#7000=VERTEX_POINT('',#27006);
#7001=VERTEX_POINT('',#27008);
#7002=VERTEX_POINT('',#27019);
#7003=VERTEX_POINT('',#27027);
#7004=VERTEX_POINT('',#27032);
#7005=VERTEX_POINT('',#27061);
#7006=VERTEX_POINT('',#27075);
#7007=VERTEX_POINT('',#27098);
#7008=VERTEX_POINT('',#27115);
#7009=VERTEX_POINT('',#27118);
#7010=VERTEX_POINT('',#27129);
#7011=VERTEX_POINT('',#27141);
#7012=VERTEX_POINT('',#27154);
#7013=VERTEX_POINT('',#27156);
#7014=VERTEX_POINT('',#27169);
#7015=VERTEX_POINT('',#27181);
#7016=VERTEX_POINT('',#27192);
#7017=VERTEX_POINT('',#27195);
#7018=VERTEX_POINT('',#27206);
#7019=VERTEX_POINT('',#27218);
#7020=VERTEX_POINT('',#27231);
#7021=VERTEX_POINT('',#27233);
#7022=VERTEX_POINT('',#27246);
#7023=VERTEX_POINT('',#27258);
#7024=VERTEX_POINT('',#27269);
#7025=VERTEX_POINT('',#27272);
#7026=VERTEX_POINT('',#27283);
#7027=VERTEX_POINT('',#27295);
#7028=VERTEX_POINT('',#27308);
#7029=VERTEX_POINT('',#27340);
#7030=VERTEX_POINT('',#27354);
#7031=VERTEX_POINT('',#27366);
#7032=VERTEX_POINT('',#27377);
#7033=VERTEX_POINT('',#27380);
#7034=VERTEX_POINT('',#27391);
#7035=VERTEX_POINT('',#27396);
#7036=VERTEX_POINT('',#27425);
#7037=VERTEX_POINT('',#27475);
#7038=VERTEX_POINT('',#27483);
#7039=VERTEX_POINT('',#27492);
#7040=VERTEX_POINT('',#27500);
#7041=VERTEX_POINT('',#27529);
#7042=VERTEX_POINT('',#27555);
#7043=VERTEX_POINT('',#27575);
#7044=VERTEX_POINT('',#27578);
#7045=VERTEX_POINT('',#27598);
#7046=VERTEX_POINT('',#27624);
#7047=VERTEX_POINT('',#27653);
#7048=VERTEX_POINT('',#27655);
#7049=VERTEX_POINT('',#27675);
#7050=VERTEX_POINT('',#27685);
#7051=VERTEX_POINT('',#27688);
#7052=VERTEX_POINT('',#27711);
#7053=VERTEX_POINT('',#27770);
#7054=VERTEX_POINT('',#27772);
#7055=VERTEX_POINT('',#27794);
#7056=VERTEX_POINT('',#27805);
#7057=VERTEX_POINT('',#27808);
#7058=VERTEX_POINT('',#27831);
#7059=VERTEX_POINT('',#27890);
#7060=VERTEX_POINT('',#27892);
#7061=VERTEX_POINT('',#27914);
#7062=VERTEX_POINT('',#27925);
#7063=VERTEX_POINT('',#27928);
#7064=VERTEX_POINT('',#27939);
#7065=VERTEX_POINT('',#27998);
#7066=VERTEX_POINT('',#28000);
#7067=VERTEX_POINT('',#28022);
#7068=VERTEX_POINT('',#28033);
#7069=VERTEX_POINT('',#28036);
#7070=VERTEX_POINT('',#28047);
#7071=VERTEX_POINT('',#28106);
#7072=VERTEX_POINT('',#28108);
#7073=VERTEX_POINT('',#28130);
#7074=VERTEX_POINT('',#28141);
#7075=VERTEX_POINT('',#28144);
#7076=VERTEX_POINT('',#28155);
#7077=VERTEX_POINT('',#28177);
#7078=VERTEX_POINT('',#28179);
#7079=VERTEX_POINT('',#28201);
#7080=VERTEX_POINT('',#28212);
#7081=VERTEX_POINT('',#28215);
#7082=VERTEX_POINT('',#28232);
#7083=VERTEX_POINT('',#28254);
#7084=VERTEX_POINT('',#28256);
#7085=VERTEX_POINT('',#28263);
#7086=VERTEX_POINT('',#28273);
#7087=VERTEX_POINT('',#28276);
#7088=VERTEX_POINT('',#28296);
#7089=VERTEX_POINT('',#28349);
#7090=VERTEX_POINT('',#28351);
#7091=VERTEX_POINT('',#28404);
#7092=VERTEX_POINT('',#28414);
#7093=VERTEX_POINT('',#28417);
#7094=VERTEX_POINT('',#28437);
#7095=VERTEX_POINT('',#28490);
#7096=VERTEX_POINT('',#28492);
#7097=VERTEX_POINT('',#28545);
#7098=VERTEX_POINT('',#28555);
#7099=VERTEX_POINT('',#28558);
#7100=VERTEX_POINT('',#28578);
#7101=VERTEX_POINT('',#28631);
#7102=VERTEX_POINT('',#28633);
#7103=VERTEX_POINT('',#28653);
#7104=VERTEX_POINT('',#28663);
#7105=VERTEX_POINT('',#28666);
#7106=VERTEX_POINT('',#28686);
#7107=VERTEX_POINT('',#28739);
#7108=VERTEX_POINT('',#28741);
#7109=VERTEX_POINT('',#28761);
#7110=VERTEX_POINT('',#28771);
#7111=VERTEX_POINT('',#28774);
#7112=VERTEX_POINT('',#28794);
#7113=VERTEX_POINT('',#28847);
#7114=VERTEX_POINT('',#28849);
#7115=VERTEX_POINT('',#28869);
#7116=VERTEX_POINT('',#28879);
#7117=VERTEX_POINT('',#28882);
#7118=VERTEX_POINT('',#28902);
#7119=VERTEX_POINT('',#28907);
#7120=VERTEX_POINT('',#28960);
#7121=VERTEX_POINT('',#28970);
#7122=VERTEX_POINT('',#28980);
#7123=VERTEX_POINT('',#29030);
#7124=VERTEX_POINT('',#29053);
#7125=VERTEX_POINT('',#29056);
#7126=VERTEX_POINT('',#29061);
#7127=VERTEX_POINT('',#29066);
#7128=VERTEX_POINT('',#29080);
#7129=VERTEX_POINT('',#29085);
#7130=VERTEX_POINT('',#29090);
#7131=VERTEX_POINT('',#29108);
#7132=VERTEX_POINT('',#29269);
#7133=VERTEX_POINT('',#29270);
#7134=VERTEX_POINT('',#29275);
#7135=VERTEX_POINT('',#29331);
#7136=VERTEX_POINT('',#29350);
#7137=VERTEX_POINT('',#29421);
#7138=VERTEX_POINT('',#29462);
#7139=VERTEX_POINT('',#29467);
#7140=VERTEX_POINT('',#29475);
#7141=VERTEX_POINT('',#29510);
#7142=VERTEX_POINT('',#29515);
#7143=VERTEX_POINT('',#29526);
#7144=VERTEX_POINT('',#29537);
#7145=VERTEX_POINT('',#29546);
#7146=VERTEX_POINT('',#29553);
#7147=VERTEX_POINT('',#29560);
#7148=VERTEX_POINT('',#29567);
#7149=VERTEX_POINT('',#29574);
#7150=VERTEX_POINT('',#29581);
#7151=VERTEX_POINT('',#29595);
#7152=VERTEX_POINT('',#29669);
#7153=VERTEX_POINT('',#29734);
#7154=VERTEX_POINT('',#29772);
#7155=VERTEX_POINT('',#29779);
#7156=VERTEX_POINT('',#29781);
#7157=VERTEX_POINT('',#29788);
#7158=VERTEX_POINT('',#29790);
#7159=VERTEX_POINT('',#29797);
#7160=VERTEX_POINT('',#29806);
#7161=VERTEX_POINT('',#29814);
#7162=VERTEX_POINT('',#29825);
#7163=VERTEX_POINT('',#29834);
#7164=VERTEX_POINT('',#29841);
#7165=VERTEX_POINT('',#29848);
#7166=VERTEX_POINT('',#29855);
#7167=VERTEX_POINT('',#29862);
#7168=VERTEX_POINT('',#29869);
#7169=VERTEX_POINT('',#29892);
#7170=VERTEX_POINT('',#29893);
#7171=VERTEX_POINT('',#29900);
#7172=VERTEX_POINT('',#29909);
#7173=VERTEX_POINT('',#29985);
#7174=VERTEX_POINT('',#29986);
#7175=VERTEX_POINT('',#29995);
#7176=VERTEX_POINT('',#30002);
#7177=VERTEX_POINT('',#30157);
#7178=VERTEX_POINT('',#30177);
#7179=VERTEX_POINT('',#30304);
#7180=VERTEX_POINT('',#30305);
#7181=VERTEX_POINT('',#30312);
#7182=VERTEX_POINT('',#30325);
#7183=VERTEX_POINT('',#30396);
#7184=VERTEX_POINT('',#30431);
#7185=VERTEX_POINT('',#30436);
#7186=VERTEX_POINT('',#30454);
#7187=VERTEX_POINT('',#30459);
#7188=VERTEX_POINT('',#30473);
#7189=VERTEX_POINT('',#30478);
#7190=VERTEX_POINT('',#30483);
#7191=VERTEX_POINT('',#30501);
#7192=VERTEX_POINT('',#30506);
#7193=VERTEX_POINT('',#30520);
#7194=VERTEX_POINT('',#30542);
#7195=VERTEX_POINT('',#30577);
#7196=VERTEX_POINT('',#30586);
#7197=VERTEX_POINT('',#30596);
#7198=VERTEX_POINT('',#30613);
#7199=VERTEX_POINT('',#30643);
#7200=VERTEX_POINT('',#30658);
#7201=VERTEX_POINT('',#30697);
#7202=VERTEX_POINT('',#30712);
#7203=VERTEX_POINT('',#30751);
#7204=VERTEX_POINT('',#30766);
#7205=VERTEX_POINT('',#30805);
#7206=VERTEX_POINT('',#30820);
#7207=VERTEX_POINT('',#30859);
#7208=VERTEX_POINT('',#30874);
#7209=VERTEX_POINT('',#30913);
#7210=VERTEX_POINT('',#30928);
#7211=VERTEX_POINT('',#30964);
#7212=VERTEX_POINT('',#30980);
#7213=VERTEX_POINT('',#30997);
#7214=VERTEX_POINT('',#31013);
#7215=VERTEX_POINT('',#31030);
#7216=VERTEX_POINT('',#31046);
#7217=VERTEX_POINT('',#31063);
#7218=VERTEX_POINT('',#31079);
#7219=VERTEX_POINT('',#31121);
#7220=VERTEX_POINT('',#31137);
#7221=VERTEX_POINT('',#31179);
#7222=VERTEX_POINT('',#31194);
#7223=VERTEX_POINT('',#31196);
#7224=VERTEX_POINT('',#31235);
#7225=VERTEX_POINT('',#31246);
#7226=VERTEX_POINT('',#31272);
#7227=VERTEX_POINT('',#31281);
#7228=VERTEX_POINT('',#31304);
#7229=VERTEX_POINT('',#31310);
#7230=VERTEX_POINT('',#31323);
#7231=VERTEX_POINT('',#31355);
#7232=VERTEX_POINT('',#31374);
#7233=VERTEX_POINT('',#31380);
#7234=VERTEX_POINT('',#31394);
#7235=VERTEX_POINT('',#31396);
#7236=VERTEX_POINT('',#31414);
#7237=VERTEX_POINT('',#31420);
#7238=VERTEX_POINT('',#31434);
#7239=VERTEX_POINT('',#31436);
#7240=VERTEX_POINT('',#31454);
#7241=VERTEX_POINT('',#31462);
#7242=VERTEX_POINT('',#31479);
#7243=VERTEX_POINT('',#31505);
#7244=VERTEX_POINT('',#31510);
#7245=VERTEX_POINT('',#31518);
#7246=VERTEX_POINT('',#31535);
#7247=VERTEX_POINT('',#31537);
#7248=VERTEX_POINT('',#31539);
#7249=VERTEX_POINT('',#31568);
#7250=VERTEX_POINT('',#31591);
#7251=VERTEX_POINT('',#31608);
#7252=VERTEX_POINT('',#31625);
#7253=VERTEX_POINT('',#31786);
#7254=VERTEX_POINT('',#31840);
#7255=VERTEX_POINT('',#31857);
#7256=VERTEX_POINT('',#31874);
#7257=VERTEX_POINT('',#31897);
#7258=VERTEX_POINT('',#31907);
#7259=VERTEX_POINT('',#31909);
#7260=VERTEX_POINT('',#31911);
#7261=VERTEX_POINT('',#31913);
#7262=VERTEX_POINT('',#31921);
#7263=VERTEX_POINT('',#31926);
#7264=VERTEX_POINT('',#31931);
#7265=VERTEX_POINT('',#31957);
#7266=VERTEX_POINT('',#31971);
#7267=VERTEX_POINT('',#31994);
#7268=VERTEX_POINT('',#32014);
#7269=VERTEX_POINT('',#32028);
#7270=VERTEX_POINT('',#32057);
#7271=VERTEX_POINT('',#32065);
#7272=VERTEX_POINT('',#32076);
#7273=VERTEX_POINT('',#32078);
#7274=VERTEX_POINT('',#32080);
#7275=VERTEX_POINT('',#32088);
#7276=VERTEX_POINT('',#32108);
#7277=VERTEX_POINT('',#32283);
#7278=VERTEX_POINT('',#32284);
#7279=VERTEX_POINT('',#32286);
#7280=VERTEX_POINT('',#32293);
#7281=VERTEX_POINT('',#32313);
#7282=VERTEX_POINT('',#32315);
#7283=VERTEX_POINT('',#32383);
#7284=VERTEX_POINT('',#32384);
#7285=VERTEX_POINT('',#32386);
#7286=VERTEX_POINT('',#32408);
#7287=VERTEX_POINT('',#32430);
#7288=VERTEX_POINT('',#32432);
#7289=VERTEX_POINT('',#32475);
#7290=VERTEX_POINT('',#32476);
#7291=VERTEX_POINT('',#32478);
#7292=VERTEX_POINT('',#32500);
#7293=VERTEX_POINT('',#32522);
#7294=VERTEX_POINT('',#32524);
#7295=VERTEX_POINT('',#32604);
#7296=VERTEX_POINT('',#32605);
#7297=VERTEX_POINT('',#32607);
#7298=VERTEX_POINT('',#32629);
#7299=VERTEX_POINT('',#32651);
#7300=VERTEX_POINT('',#32653);
#7301=VERTEX_POINT('',#32733);
#7302=VERTEX_POINT('',#32734);
#7303=VERTEX_POINT('',#32736);
#7304=VERTEX_POINT('',#32756);
#7305=VERTEX_POINT('',#32776);
#7306=VERTEX_POINT('',#32778);
#7307=VERTEX_POINT('',#32883);
#7308=VERTEX_POINT('',#32884);
#7309=VERTEX_POINT('',#32886);
#7310=VERTEX_POINT('',#32908);
#7311=VERTEX_POINT('',#32930);
#7312=VERTEX_POINT('',#32932);
#7313=VERTEX_POINT('',#33049);
#7314=VERTEX_POINT('',#33050);
#7315=VERTEX_POINT('',#33052);
#7316=VERTEX_POINT('',#33065);
#7317=VERTEX_POINT('',#33077);
#7318=VERTEX_POINT('',#33089);
#7319=VERTEX_POINT('',#33103);
#7320=VERTEX_POINT('',#33105);
#7321=VERTEX_POINT('',#33118);
#7322=VERTEX_POINT('',#33130);
#7323=VERTEX_POINT('',#33154);
#7324=VERTEX_POINT('',#33155);
#7325=VERTEX_POINT('',#33157);
#7326=VERTEX_POINT('',#33179);
#7327=VERTEX_POINT('',#33201);
#7328=VERTEX_POINT('',#33203);
#7329=VERTEX_POINT('',#33320);
#7330=VERTEX_POINT('',#33321);
#7331=VERTEX_POINT('',#33323);
#7332=VERTEX_POINT('',#33343);
#7333=VERTEX_POINT('',#33363);
#7334=VERTEX_POINT('',#33365);
#7335=VERTEX_POINT('',#33470);
#7336=VERTEX_POINT('',#33471);
#7337=VERTEX_POINT('',#33473);
#7338=VERTEX_POINT('',#33493);
#7339=VERTEX_POINT('',#33513);
#7340=VERTEX_POINT('',#33515);
#7341=VERTEX_POINT('',#33620);
#7342=VERTEX_POINT('',#33621);
#7343=VERTEX_POINT('',#33623);
#7344=VERTEX_POINT('',#33643);
#7345=VERTEX_POINT('',#33663);
#7346=VERTEX_POINT('',#33665);
#7347=VERTEX_POINT('',#33770);
#7348=VERTEX_POINT('',#33771);
#7349=VERTEX_POINT('',#33773);
#7350=VERTEX_POINT('',#33793);
#7351=VERTEX_POINT('',#33813);
#7352=VERTEX_POINT('',#33815);
#7353=VERTEX_POINT('',#33920);
#7354=VERTEX_POINT('',#33921);
#7355=VERTEX_POINT('',#33923);
#7356=VERTEX_POINT('',#33936);
#7357=VERTEX_POINT('',#33948);
#7358=VERTEX_POINT('',#33960);
#7359=VERTEX_POINT('',#33974);
#7360=VERTEX_POINT('',#33976);
#7361=VERTEX_POINT('',#33989);
#7362=VERTEX_POINT('',#34001);
#7363=VERTEX_POINT('',#34025);
#7364=VERTEX_POINT('',#34026);
#7365=VERTEX_POINT('',#34058);
#7366=VERTEX_POINT('',#34072);
#7367=VERTEX_POINT('',#34084);
#7368=VERTEX_POINT('',#34096);
#7369=VERTEX_POINT('',#34109);
#7370=VERTEX_POINT('',#34141);
#7371=VERTEX_POINT('',#34154);
#7372=VERTEX_POINT('',#34167);
#7373=VERTEX_POINT('',#34191);
#7374=VERTEX_POINT('',#34192);
#7375=VERTEX_POINT('',#34202);
#7376=VERTEX_POINT('',#34211);
#7377=VERTEX_POINT('',#34243);
#7378=VERTEX_POINT('',#34269);
#7379=VERTEX_POINT('',#34298);
#7380=VERTEX_POINT('',#34324);
#7381=VERTEX_POINT('',#34353);
#7382=VERTEX_POINT('',#34373);
#7383=VERTEX_POINT('',#34378);
#7384=VERTEX_POINT('',#34407);
#7385=VERTEX_POINT('',#34482);
#7386=VERTEX_POINT('',#34483);
#7387=VERTEX_POINT('',#34485);
#7388=VERTEX_POINT('',#34505);
#7389=VERTEX_POINT('',#34525);
#7390=VERTEX_POINT('',#34527);
#7391=VERTEX_POINT('',#34556);
#7392=VERTEX_POINT('',#34582);
#7393=VERTEX_POINT('',#34636);
#7394=VERTEX_POINT('',#34637);
#7395=VERTEX_POINT('',#34732);
#7396=VERTEX_POINT('',#34741);
#7397=VERTEX_POINT('',#34751);
#7398=VERTEX_POINT('',#34768);
#7399=VERTEX_POINT('',#34788);
#7400=VERTEX_POINT('',#34814);
#7401=VERTEX_POINT('',#34819);
#7402=VERTEX_POINT('',#34872);
#7403=VERTEX_POINT('',#34882);
#7404=VERTEX_POINT('',#35096);
#7405=VERTEX_POINT('',#35101);
#7406=VERTEX_POINT('',#35113);
#7407=VERTEX_POINT('',#35125);
#7408=VERTEX_POINT('',#35126);
#7409=VERTEX_POINT('',#35131);
#7410=VERTEX_POINT('',#35133);
#7411=VERTEX_POINT('',#35138);
#7412=VERTEX_POINT('',#35145);
#7413=VERTEX_POINT('',#35146);
#7414=VERTEX_POINT('',#35148);
#7415=VERTEX_POINT('',#35153);
#7416=VERTEX_POINT('',#35158);
#7417=VERTEX_POINT('',#35165);
#7418=VERTEX_POINT('',#35166);
#7419=VERTEX_POINT('',#35168);
#7420=VERTEX_POINT('',#35173);
#7421=VERTEX_POINT('',#35178);
#7422=VERTEX_POINT('',#35196);
#7423=VERTEX_POINT('',#35197);
#7424=VERTEX_POINT('',#35202);
#7425=VERTEX_POINT('',#35204);
#7426=VERTEX_POINT('',#35209);
#7427=VERTEX_POINT('',#35216);
#7428=VERTEX_POINT('',#35385);
#7429=VERTEX_POINT('',#35387);
#7430=VERTEX_POINT('',#35410);
#7431=VERTEX_POINT('',#35433);
#7432=VERTEX_POINT('',#35460);
#7433=VERTEX_POINT('',#35462);
#7434=VERTEX_POINT('',#35470);
#7435=VERTEX_POINT('',#35511);
#7436=VERTEX_POINT('',#35573);
#7437=VERTEX_POINT('',#35602);
#7438=VERTEX_POINT('',#35610);
#7439=VERTEX_POINT('',#35612);
#7440=VERTEX_POINT('',#35620);
#7441=VERTEX_POINT('',#35705);
#7442=VERTEX_POINT('',#35710);
#7443=VERTEX_POINT('',#35715);
#7444=VERTEX_POINT('',#35726);
#7445=VERTEX_POINT('',#35731);
#7446=VERTEX_POINT('',#35742);
#7447=VERTEX_POINT('',#35752);
#7448=VERTEX_POINT('',#35788);
#7449=VERTEX_POINT('',#35822);
#7450=VERTEX_POINT('',#35858);
#7451=VERTEX_POINT('',#35892);
#7452=VERTEX_POINT('',#35897);
#7453=VERTEX_POINT('',#35902);
#7454=VERTEX_POINT('',#35907);
#7455=VERTEX_POINT('',#35912);
#7456=VERTEX_POINT('',#35914);
#7457=VERTEX_POINT('',#35924);
#7458=VERTEX_POINT('',#35925);
#7459=VERTEX_POINT('',#35927);
#7460=VERTEX_POINT('',#35933);
#7461=VERTEX_POINT('',#35938);
#7462=VERTEX_POINT('',#35943);
#7463=VERTEX_POINT('',#35951);
#7464=VERTEX_POINT('',#35979);
#7465=VERTEX_POINT('',#35990);
#7466=VERTEX_POINT('',#36010);
#7467=VERTEX_POINT('',#36027);
#7468=VERTEX_POINT('',#36053);
#7469=VERTEX_POINT('',#36067);
#7470=VERTEX_POINT('',#36069);
#7471=VERTEX_POINT('',#36080);
#7472=VERTEX_POINT('',#36103);
#7473=VERTEX_POINT('',#36120);
#7474=VERTEX_POINT('',#36163);
#7475=VERTEX_POINT('',#36164);
#7476=VERTEX_POINT('',#36166);
#7477=VERTEX_POINT('',#36177);
#7478=VERTEX_POINT('',#36197);
#7479=VERTEX_POINT('',#36214);
#7480=VERTEX_POINT('',#36253);
#7481=VERTEX_POINT('',#36264);
#7482=VERTEX_POINT('',#36287);
#7483=VERTEX_POINT('',#36304);
#7484=VERTEX_POINT('',#36347);
#7485=VERTEX_POINT('',#36353);
#7486=VERTEX_POINT('',#36358);
#7487=VERTEX_POINT('',#36396);
#7488=VERTEX_POINT('',#36404);
#7489=VERTEX_POINT('',#36438);
#7490=VERTEX_POINT('',#36446);
#7491=VERTEX_POINT('',#36468);
#7492=VERTEX_POINT('',#36469);
#7493=VERTEX_POINT('',#36486);
#7494=VERTEX_POINT('',#36494);
#7495=VERTEX_POINT('',#37292);
#7496=VERTEX_POINT('',#37303);
#7497=VERTEX_POINT('',#37310);
#7498=VERTEX_POINT('',#37312);
#7499=VERTEX_POINT('',#37319);
#7500=VERTEX_POINT('',#37321);
#7501=VERTEX_POINT('',#37335);
#7502=VERTEX_POINT('',#37336);
#7503=VERTEX_POINT('',#37354);
#7504=VERTEX_POINT('',#37363);
#7505=VERTEX_POINT('',#37368);
#7506=VERTEX_POINT('',#37386);
#7507=VERTEX_POINT('',#37409);
#7508=VERTEX_POINT('',#37410);
#7509=VERTEX_POINT('',#37428);
#7510=VERTEX_POINT('',#37450);
#7511=VERTEX_POINT('',#37455);
#7512=VERTEX_POINT('',#37473);
#7513=VERTEX_POINT('',#37498);
#7514=VERTEX_POINT('',#37499);
#7515=VERTEX_POINT('',#37549);
#7516=VERTEX_POINT('',#37569);
#7517=VERTEX_POINT('',#37574);
#7518=VERTEX_POINT('',#37594);
#7519=VERTEX_POINT('',#37649);
#7520=VERTEX_POINT('',#37650);
#7521=VERTEX_POINT('',#37700);
#7522=VERTEX_POINT('',#37720);
#7523=VERTEX_POINT('',#37725);
#7524=VERTEX_POINT('',#37775);
#7525=VERTEX_POINT('',#37845);
#7526=VERTEX_POINT('',#37846);
#7527=VERTEX_POINT('',#37864);
#7528=VERTEX_POINT('',#37885);
#7529=VERTEX_POINT('',#37890);
#7530=VERTEX_POINT('',#37909);
#7531=VERTEX_POINT('',#37932);
#7532=VERTEX_POINT('',#37933);
#7533=VERTEX_POINT('',#37953);
#7534=VERTEX_POINT('',#37974);
#7535=VERTEX_POINT('',#37979);
#7536=VERTEX_POINT('',#38032);
#7537=VERTEX_POINT('',#38087);
#7538=VERTEX_POINT('',#38088);
#7539=VERTEX_POINT('',#38107);
#7540=VERTEX_POINT('',#38128);
#7541=VERTEX_POINT('',#38133);
#7542=VERTEX_POINT('',#38154);
#7543=VERTEX_POINT('',#38178);
#7544=VERTEX_POINT('',#38179);
#7545=VERTEX_POINT('',#38199);
#7546=VERTEX_POINT('',#38224);
#7547=VERTEX_POINT('',#38229);
#7548=VERTEX_POINT('',#38279);
#7549=VERTEX_POINT('',#38334);
#7550=VERTEX_POINT('',#38335);
#7551=VERTEX_POINT('',#38353);
#7552=VERTEX_POINT('',#38374);
#7553=VERTEX_POINT('',#38379);
#7554=VERTEX_POINT('',#38399);
#7555=VERTEX_POINT('',#38422);
#7556=VERTEX_POINT('',#38423);
#7557=VERTEX_POINT('',#38441);
#7558=VERTEX_POINT('',#38461);
#7559=VERTEX_POINT('',#38466);
#7560=VERTEX_POINT('',#38485);
#7561=VERTEX_POINT('',#38508);
#7562=VERTEX_POINT('',#38509);
#7563=VERTEX_POINT('',#38527);
#7564=VERTEX_POINT('',#38548);
#7565=VERTEX_POINT('',#38553);
#7566=VERTEX_POINT('',#38573);
#7567=VERTEX_POINT('',#38596);
#7568=VERTEX_POINT('',#38597);
#7569=VERTEX_POINT('',#38615);
#7570=VERTEX_POINT('',#38636);
#7571=VERTEX_POINT('',#38641);
#7572=VERTEX_POINT('',#38660);
#7573=VERTEX_POINT('',#38683);
#7574=VERTEX_POINT('',#38684);
#7575=VERTEX_POINT('',#38703);
#7576=VERTEX_POINT('',#38725);
#7577=VERTEX_POINT('',#38730);
#7578=VERTEX_POINT('',#38752);
#7579=VERTEX_POINT('',#38776);
#7580=VERTEX_POINT('',#38777);
#7581=VERTEX_POINT('',#38795);
#7582=VERTEX_POINT('',#38817);
#7583=VERTEX_POINT('',#38827);
#7584=VERTEX_POINT('',#38848);
#7585=VERTEX_POINT('',#38893);
#7586=VERTEX_POINT('',#38894);
#7587=VERTEX_POINT('',#38912);
#7588=VERTEX_POINT('',#38931);
#7589=VERTEX_POINT('',#38954);
#7590=VERTEX_POINT('',#38963);
#7591=VERTEX_POINT('',#38990);
#7592=VERTEX_POINT('',#38991);
#7593=VERTEX_POINT('',#39009);
#7594=VERTEX_POINT('',#39030);
#7595=VERTEX_POINT('',#39035);
#7596=VERTEX_POINT('',#39053);
#7597=VERTEX_POINT('',#39076);
#7598=VERTEX_POINT('',#39077);
#7599=VERTEX_POINT('',#39086);
#7600=VERTEX_POINT('',#39106);
#7601=VERTEX_POINT('',#39115);
#7602=VERTEX_POINT('',#39122);
#7603=VERTEX_POINT('',#39173);
#7604=VERTEX_POINT('',#39174);
#7605=VERTEX_POINT('',#39192);
#7606=VERTEX_POINT('',#39201);
#7607=VERTEX_POINT('',#39206);
#7608=VERTEX_POINT('',#39224);
#7609=VERTEX_POINT('',#39247);
#7610=VERTEX_POINT('',#39248);
#7611=VERTEX_POINT('',#39266);
#7612=VERTEX_POINT('',#39286);
#7613=VERTEX_POINT('',#39291);
#7614=VERTEX_POINT('',#39311);
#7615=VERTEX_POINT('',#39334);
#7616=VERTEX_POINT('',#39335);
#7617=VERTEX_POINT('',#39385);
#7618=VERTEX_POINT('',#39405);
#7619=VERTEX_POINT('',#39410);
#7620=VERTEX_POINT('',#39460);
#7621=VERTEX_POINT('',#39483);
#7622=VERTEX_POINT('',#39484);
#7623=VERTEX_POINT('',#39534);
#7624=VERTEX_POINT('',#39554);
#7625=VERTEX_POINT('',#39559);
#7626=VERTEX_POINT('',#39609);
#7627=VERTEX_POINT('',#39664);
#7628=VERTEX_POINT('',#39665);
#7629=VERTEX_POINT('',#39683);
#7630=VERTEX_POINT('',#39701);
#7631=VERTEX_POINT('',#39708);
#7632=VERTEX_POINT('',#39726);
#7633=VERTEX_POINT('',#39749);
#7634=VERTEX_POINT('',#39750);
#7635=VERTEX_POINT('',#39770);
#7636=VERTEX_POINT('',#39790);
#7637=VERTEX_POINT('',#39795);
#7638=VERTEX_POINT('',#39845);
#7639=VERTEX_POINT('',#39900);
#7640=VERTEX_POINT('',#39901);
#7641=VERTEX_POINT('',#39920);
#7642=VERTEX_POINT('',#39939);
#7643=VERTEX_POINT('',#39944);
#7644=VERTEX_POINT('',#39963);
#7645=VERTEX_POINT('',#39987);
#7646=VERTEX_POINT('',#39988);
#7647=VERTEX_POINT('',#40008);
#7648=VERTEX_POINT('',#40028);
#7649=VERTEX_POINT('',#40033);
#7650=VERTEX_POINT('',#40083);
#7651=VERTEX_POINT('',#40138);
#7652=VERTEX_POINT('',#40139);
#7653=VERTEX_POINT('',#40157);
#7654=VERTEX_POINT('',#40208);
#7655=VERTEX_POINT('',#40213);
#7656=VERTEX_POINT('',#40231);
#7657=VERTEX_POINT('',#40254);
#7658=VERTEX_POINT('',#40255);
#7659=VERTEX_POINT('',#40273);
#7660=VERTEX_POINT('',#40320);
#7661=VERTEX_POINT('',#40325);
#7662=VERTEX_POINT('',#40343);
#7663=VERTEX_POINT('',#40366);
#7664=VERTEX_POINT('',#40367);
#7665=VERTEX_POINT('',#40385);
#7666=VERTEX_POINT('',#40403);
#7667=VERTEX_POINT('',#40408);
#7668=VERTEX_POINT('',#40426);
#7669=VERTEX_POINT('',#40449);
#7670=VERTEX_POINT('',#40450);
#7671=VERTEX_POINT('',#40468);
#7672=VERTEX_POINT('',#40486);
#7673=VERTEX_POINT('',#40491);
#7674=VERTEX_POINT('',#40509);
#7675=VERTEX_POINT('',#40532);
#7676=VERTEX_POINT('',#40533);
#7677=VERTEX_POINT('',#40552);
#7678=VERTEX_POINT('',#40571);
#7679=VERTEX_POINT('',#40576);
#7680=VERTEX_POINT('',#40595);
#7681=VERTEX_POINT('',#40619);
#7682=VERTEX_POINT('',#40620);
#7683=VERTEX_POINT('',#40638);
#7684=VERTEX_POINT('',#40656);
#7685=VERTEX_POINT('',#40682);
#7686=VERTEX_POINT('',#40701);
#7687=VERTEX_POINT('',#40729);
#7688=VERTEX_POINT('',#40730);
#7689=VERTEX_POINT('',#40748);
#7690=VERTEX_POINT('',#40768);
#7691=VERTEX_POINT('',#40775);
#7692=VERTEX_POINT('',#40784);
#7693=VERTEX_POINT('',#40825);
#7694=VERTEX_POINT('',#40826);
#7695=VERTEX_POINT('',#40844);
#7696=VERTEX_POINT('',#40862);
#7697=VERTEX_POINT('',#40867);
#7698=VERTEX_POINT('',#40885);
#7699=VERTEX_POINT('',#40908);
#7700=VERTEX_POINT('',#40909);
#7701=VERTEX_POINT('',#40929);
#7702=VERTEX_POINT('',#40947);
#7703=VERTEX_POINT('',#40956);
#7704=VERTEX_POINT('',#40976);
#9000=EDGE_CURVE('',#6972,#6973,#365,.T.);
#9001=EDGE_CURVE('',#6972,#6974,#366,.T.);
#9002=EDGE_CURVE('',#6974,#6975,#367,.F.);
#9003=EDGE_CURVE('',#6975,#6976,#368,.T.);
#9004=EDGE_CURVE('',#6976,#6977,#369,.T.);
#9005=EDGE_CURVE('',#6977,#6978,#370,.T.);
#9006=EDGE_CURVE('',#6978,#6973,#6071,.F.);
#9007=EDGE_CURVE('',#6979,#6980,#371,.T.);
#9008=EDGE_CURVE('',#6979,#6981,#372,.F.);
#9009=EDGE_CURVE('',#6981,#6982,#373,.T.);
#9010=EDGE_CURVE('',#6982,#6983,#374,.F.);
#9011=EDGE_CURVE('',#6983,#6984,#375,.T.);
#9012=EDGE_CURVE('',#6984,#6985,#376,.F.);
#9013=EDGE_CURVE('',#6985,#6986,#377,.T.);
#9014=EDGE_CURVE('',#6986,#6987,#378,.T.);
#9015=EDGE_CURVE('',#6987,#6988,#379,.T.);
#9016=EDGE_CURVE('',#6988,#6989,#380,.T.);
#9017=EDGE_CURVE('',#6989,#6990,#381,.T.);
#9018=EDGE_CURVE('',#6990,#6991,#382,.T.);
#9019=EDGE_CURVE('',#6991,#6992,#383,.T.);
#9020=EDGE_CURVE('',#6992,#6980,#384,.T.);
#9021=EDGE_CURVE('',#6993,#6994,#385,.T.);
#9022=EDGE_CURVE('',#6993,#6995,#386,.T.);
#9023=EDGE_CURVE('',#6995,#6996,#387,.T.);
#9024=EDGE_CURVE('',#6996,#6997,#388,.T.);
#9025=EDGE_CURVE('',#6997,#6998,#389,.F.);
#9026=EDGE_CURVE('',#6998,#6999,#6072,.F.);
#9027=EDGE_CURVE('',#6999,#7000,#2017,.F.);
#9028=EDGE_CURVE('',#7000,#7001,#390,.F.);
#9029=EDGE_CURVE('',#7001,#7002,#391,.F.);
#9030=EDGE_CURVE('',#7002,#7003,#392,.F.);
#9031=EDGE_CURVE('',#7003,#7004,#393,.F.);
#9032=EDGE_CURVE('',#7004,#7005,#394,.T.);
#9033=EDGE_CURVE('',#7005,#7006,#395,.T.);
#9034=EDGE_CURVE('',#7006,#7007,#396,.T.);
#9035=EDGE_CURVE('',#7007,#7008,#397,.T.);
#9036=EDGE_CURVE('',#7008,#7009,#398,.T.);
#9037=EDGE_CURVE('',#7009,#7010,#399,.T.);
#9038=EDGE_CURVE('',#7010,#7011,#400,.T.);
#9039=EDGE_CURVE('',#7011,#7012,#2018,.F.);
#9040=EDGE_CURVE('',#7012,#7013,#401,.T.);
#9041=EDGE_CURVE('',#7013,#7014,#402,.T.);
#9042=EDGE_CURVE('',#7014,#7015,#403,.T.);
#9043=EDGE_CURVE('',#7015,#7016,#404,.T.);
#9044=EDGE_CURVE('',#7016,#7017,#405,.T.);
#9045=EDGE_CURVE('',#7017,#7018,#406,.T.);
#9046=EDGE_CURVE('',#7018,#7019,#407,.T.);
#9047=EDGE_CURVE('',#7019,#7020,#2019,.F.);
#9048=EDGE_CURVE('',#7020,#7021,#408,.T.);
#9049=EDGE_CURVE('',#7021,#7022,#409,.T.);
#9050=EDGE_CURVE('',#7022,#7023,#410,.T.);
#9051=EDGE_CURVE('',#7023,#7024,#411,.T.);
#9052=EDGE_CURVE('',#7024,#7025,#412,.T.);
#9053=EDGE_CURVE('',#7025,#7026,#413,.T.);
#9054=EDGE_CURVE('',#7026,#7027,#414,.T.);
#9055=EDGE_CURVE('',#7027,#7028,#415,.T.);
#9056=EDGE_CURVE('',#7028,#7029,#416,.T.);
#9057=EDGE_CURVE('',#7029,#7030,#417,.T.);
#9058=EDGE_CURVE('',#7030,#7031,#418,.T.);
#9059=EDGE_CURVE('',#7031,#7032,#419,.T.);
#9060=EDGE_CURVE('',#7032,#7033,#420,.T.);
#9061=EDGE_CURVE('',#7033,#7034,#421,.F.);
#9062=EDGE_CURVE('',#7034,#7035,#422,.F.);
#9063=EDGE_CURVE('',#7035,#7036,#423,.F.);
#9064=EDGE_CURVE('',#7036,#7037,#424,.F.);
#9065=EDGE_CURVE('',#7037,#7038,#425,.T.);
#9066=EDGE_CURVE('',#7038,#7039,#426,.T.);
#9067=EDGE_CURVE('',#7039,#7040,#427,.T.);
#9068=EDGE_CURVE('',#7040,#7041,#428,.T.);
#9069=EDGE_CURVE('',#7041,#7042,#429,.T.);
#9070=EDGE_CURVE('',#7042,#7043,#430,.T.);
#9071=EDGE_CURVE('',#7043,#7044,#431,.T.);
#9072=EDGE_CURVE('',#7044,#7045,#432,.T.);
#9073=EDGE_CURVE('',#7045,#7046,#433,.T.);
#9074=EDGE_CURVE('',#7046,#7047,#2020,.F.);
#9075=EDGE_CURVE('',#7047,#7048,#434,.T.);
#9076=EDGE_CURVE('',#7048,#7049,#435,.T.);
#9077=EDGE_CURVE('',#7049,#7050,#436,.T.);
#9078=EDGE_CURVE('',#7050,#7051,#437,.T.);
#9079=EDGE_CURVE('',#7051,#7052,#438,.T.);
#9080=EDGE_CURVE('',#7052,#7053,#2021,.T.);
#9081=EDGE_CURVE('',#7053,#7054,#439,.T.);
#9082=EDGE_CURVE('',#7054,#7055,#440,.T.);
#9083=EDGE_CURVE('',#7055,#7056,#441,.T.);
#9084=EDGE_CURVE('',#7056,#7057,#442,.T.);
#9085=EDGE_CURVE('',#7057,#7058,#443,.T.);
#9086=EDGE_CURVE('',#7058,#7059,#2022,.T.);
#9087=EDGE_CURVE('',#7059,#7060,#444,.T.);
#9088=EDGE_CURVE('',#7060,#7061,#445,.T.);
#9089=EDGE_CURVE('',#7061,#7062,#446,.T.);
#9090=EDGE_CURVE('',#7062,#7063,#447,.T.);
#9091=EDGE_CURVE('',#7063,#7064,#448,.T.);
#9092=EDGE_CURVE('',#7064,#7065,#2023,.T.);
#9093=EDGE_CURVE('',#7065,#7066,#449,.T.);
#9094=EDGE_CURVE('',#7066,#7067,#450,.T.);
#9095=EDGE_CURVE('',#7067,#7068,#451,.T.);
#9096=EDGE_CURVE('',#7068,#7069,#452,.T.);
#9097=EDGE_CURVE('',#7069,#7070,#453,.T.);
#9098=EDGE_CURVE('',#7070,#7071,#2024,.T.);
#9099=EDGE_CURVE('',#7071,#7072,#454,.T.);
#9100=EDGE_CURVE('',#7072,#7073,#455,.T.);
#9101=EDGE_CURVE('',#7073,#7074,#456,.T.);
#9102=EDGE_CURVE('',#7074,#7075,#457,.T.);
#9103=EDGE_CURVE('',#7075,#7076,#458,.T.);
#9104=EDGE_CURVE('',#7076,#7077,#2025,.T.);
#9105=EDGE_CURVE('',#7077,#7078,#459,.T.);
#9106=EDGE_CURVE('',#7078,#7079,#460,.T.);
#9107=EDGE_CURVE('',#7079,#7080,#461,.T.);
#9108=EDGE_CURVE('',#7080,#7081,#462,.T.);
#9109=EDGE_CURVE('',#7081,#7082,#463,.T.);
#9110=EDGE_CURVE('',#7082,#7083,#2026,.T.);
#9111=EDGE_CURVE('',#7083,#7084,#464,.F.);
#9112=EDGE_CURVE('',#7084,#7085,#465,.T.);
#9113=EDGE_CURVE('',#7085,#7086,#466,.T.);
#9114=EDGE_CURVE('',#7086,#7087,#467,.T.);
#9115=EDGE_CURVE('',#7087,#7088,#468,.T.);
#9116=EDGE_CURVE('',#7088,#7089,#2027,.T.);
#9117=EDGE_CURVE('',#7089,#7090,#469,.T.);
#9118=EDGE_CURVE('',#7090,#7091,#470,.T.);
#9119=EDGE_CURVE('',#7091,#7092,#471,.T.);
#9120=EDGE_CURVE('',#7092,#7093,#472,.T.);
#9121=EDGE_CURVE('',#7093,#7094,#473,.T.);
#9122=EDGE_CURVE('',#7094,#7095,#2028,.T.);
#9123=EDGE_CURVE('',#7095,#7096,#474,.T.);
#9124=EDGE_CURVE('',#7096,#7097,#475,.T.);
#9125=EDGE_CURVE('',#7097,#7098,#476,.T.);
#9126=EDGE_CURVE('',#7098,#7099,#477,.T.);
#9127=EDGE_CURVE('',#7099,#7100,#478,.T.);
#9128=EDGE_CURVE('',#7100,#7101,#2029,.T.);
#9129=EDGE_CURVE('',#7101,#7102,#479,.T.);
#9130=EDGE_CURVE('',#7102,#7103,#480,.T.);
#9131=EDGE_CURVE('',#7103,#7104,#481,.T.);
#9132=EDGE_CURVE('',#7104,#7105,#482,.T.);
#9133=EDGE_CURVE('',#7105,#7106,#483,.T.);
#9134=EDGE_CURVE('',#7106,#7107,#2030,.T.);
#9135=EDGE_CURVE('',#7107,#7108,#484,.T.);
#9136=EDGE_CURVE('',#7108,#7109,#485,.T.);
#9137=EDGE_CURVE('',#7109,#7110,#486,.T.);
#9138=EDGE_CURVE('',#7110,#7111,#487,.T.);
#9139=EDGE_CURVE('',#7111,#7112,#488,.T.);
#9140=EDGE_CURVE('',#7112,#7113,#2031,.T.);
#9141=EDGE_CURVE('',#7113,#7114,#489,.T.);
#9142=EDGE_CURVE('',#7114,#7115,#490,.T.);
#9143=EDGE_CURVE('',#7115,#7116,#491,.T.);
#9144=EDGE_CURVE('',#7116,#7117,#492,.F.);
#9145=EDGE_CURVE('',#7117,#7118,#493,.F.);
#9146=EDGE_CURVE('',#7118,#7119,#494,.T.);
#9147=EDGE_CURVE('',#7119,#7120,#495,.T.);
#9148=EDGE_CURVE('',#7120,#7121,#496,.T.);
#9149=EDGE_CURVE('',#7121,#7122,#497,.F.);
#9150=EDGE_CURVE('',#7122,#7123,#498,.F.);
#9151=EDGE_CURVE('',#7123,#7124,#499,.T.);
#9152=EDGE_CURVE('',#7124,#7125,#500,.T.);
#9153=EDGE_CURVE('',#7125,#7126,#501,.F.);
#9154=EDGE_CURVE('',#7126,#7127,#502,.F.);
#9155=EDGE_CURVE('',#7127,#7128,#503,.F.);
#9156=EDGE_CURVE('',#7128,#7129,#504,.F.);
#9157=EDGE_CURVE('',#7129,#7130,#505,.T.);
#9158=EDGE_CURVE('',#7130,#7131,#506,.F.);
#9159=EDGE_CURVE('',#7131,#6994,#507,.T.);
#9160=EDGE_CURVE('',#7132,#7133,#508,.T.);
#9161=EDGE_CURVE('',#7134,#7132,#509,.T.);
#9162=EDGE_CURVE('',#7134,#7135,#510,.T.);
#9163=EDGE_CURVE('',#7135,#7136,#511,.T.);
#9164=EDGE_CURVE('',#7137,#7136,#512,.T.);
#9165=EDGE_CURVE('',#7137,#7138,#513,.T.);
#9166=EDGE_CURVE('',#7139,#7138,#514,.T.);
#9167=EDGE_CURVE('',#7139,#7140,#515,.T.);
#9168=EDGE_CURVE('',#7140,#7141,#516,.T.);
#9169=EDGE_CURVE('',#7141,#7142,#517,.T.);
#9170=EDGE_CURVE('',#7142,#7143,#518,.T.);
#9171=EDGE_CURVE('',#7144,#7143,#519,.T.);
#9172=EDGE_CURVE('',#7145,#7144,#520,.T.);
#9173=EDGE_CURVE('',#7145,#7146,#521,.F.);
#9174=EDGE_CURVE('',#7146,#7147,#522,.T.);
#9175=EDGE_CURVE('',#7147,#7148,#523,.F.);
#9176=EDGE_CURVE('',#7149,#7148,#524,.T.);
#9177=EDGE_CURVE('',#7150,#7149,#525,.T.);
#9178=EDGE_CURVE('',#7150,#7151,#526,.T.);
#9179=EDGE_CURVE('',#7151,#7152,#527,.T.);
#9180=EDGE_CURVE('',#7153,#7152,#528,.T.);
#9181=EDGE_CURVE('',#7154,#7153,#529,.T.);
#9182=EDGE_CURVE('',#7155,#7154,#6073,.T.);
#9183=EDGE_CURVE('',#7156,#7155,#530,.T.);
#9184=EDGE_CURVE('',#7157,#7156,#6074,.T.);
#9185=EDGE_CURVE('',#7158,#7157,#531,.T.);
#9186=EDGE_CURVE('',#7159,#7158,#532,.T.);
#9187=EDGE_CURVE('',#7160,#7159,#533,.T.);
#9188=EDGE_CURVE('',#7161,#7160,#534,.T.);
#9189=EDGE_CURVE('',#7161,#7162,#535,.F.);
#9190=EDGE_CURVE('',#7162,#7163,#536,.F.);
#9191=EDGE_CURVE('',#7164,#7163,#537,.T.);
#9192=EDGE_CURVE('',#7165,#7164,#538,.T.);
#9193=EDGE_CURVE('',#7166,#7165,#539,.T.);
#9194=EDGE_CURVE('',#7166,#7167,#540,.F.);
#9195=EDGE_CURVE('',#7167,#7168,#541,.T.);
#9196=EDGE_CURVE('',#7133,#7168,#542,.T.);
#9197=EDGE_CURVE('',#7169,#7170,#543,.F.);
#9198=EDGE_CURVE('',#7171,#7170,#544,.T.);
#9199=EDGE_CURVE('',#7172,#7171,#545,.T.);
#9200=EDGE_CURVE('',#7169,#7172,#546,.T.);
#9201=EDGE_CURVE('',#7173,#7174,#547,.F.);
#9202=EDGE_CURVE('',#7174,#7175,#548,.F.);
#9203=EDGE_CURVE('',#7176,#7175,#549,.T.);
#9204=EDGE_CURVE('',#7176,#7173,#550,.F.);
#9205=EDGE_CURVE('',#7177,#7133,#551,.T.);
#9206=EDGE_CURVE('',#7138,#7177,#552,.T.);
#9207=EDGE_CURVE('',#7178,#7137,#553,.T.);
#9208=EDGE_CURVE('',#7132,#7178,#554,.T.);
#9209=EDGE_CURVE('',#7179,#7180,#555,.F.);
#9210=EDGE_CURVE('',#7181,#7179,#556,.F.);
#9211=EDGE_CURVE('',#7182,#7181,#557,.F.);
#9212=EDGE_CURVE('',#7180,#7182,#558,.F.);
#9213=EDGE_CURVE('',#6994,#7183,#559,.T.);
#9214=EDGE_CURVE('',#7183,#7184,#560,.F.);
#9215=EDGE_CURVE('',#7184,#7185,#561,.T.);
#9216=EDGE_CURVE('',#7185,#7186,#562,.F.);
#9217=EDGE_CURVE('',#7186,#7187,#563,.F.);
#9218=EDGE_CURVE('',#7187,#7188,#564,.F.);
#9219=EDGE_CURVE('',#7188,#7189,#565,.F.);
#9220=EDGE_CURVE('',#7189,#7190,#566,.T.);
#9221=EDGE_CURVE('',#7190,#7191,#567,.F.);
#9222=EDGE_CURVE('',#7191,#7192,#568,.T.);
#9223=EDGE_CURVE('',#7192,#7193,#569,.F.);
#9224=EDGE_CURVE('',#7193,#7124,#570,.T.);
#9225=EDGE_CURVE('',#7123,#7194,#571,.F.);
#9226=EDGE_CURVE('',#7194,#7195,#572,.T.);
#9227=EDGE_CURVE('',#7195,#7196,#573,.T.);
#9228=EDGE_CURVE('',#7196,#7197,#574,.F.);
#9229=EDGE_CURVE('',#7197,#7198,#575,.F.);
#9230=EDGE_CURVE('',#7198,#7116,#576,.F.);
#9231=EDGE_CURVE('',#7115,#7199,#577,.T.);
#9232=EDGE_CURVE('',#7199,#7200,#2032,.T.);
#9233=EDGE_CURVE('',#7200,#7110,#578,.T.);
#9234=EDGE_CURVE('',#7109,#7201,#579,.T.);
#9235=EDGE_CURVE('',#7201,#7202,#2033,.T.);
#9236=EDGE_CURVE('',#7202,#7104,#580,.T.);
#9237=EDGE_CURVE('',#7103,#7203,#581,.T.);
#9238=EDGE_CURVE('',#7203,#7204,#2034,.T.);
#9239=EDGE_CURVE('',#7204,#7098,#582,.T.);
#9240=EDGE_CURVE('',#7097,#7205,#583,.T.);
#9241=EDGE_CURVE('',#7205,#7206,#2035,.T.);
#9242=EDGE_CURVE('',#7206,#7092,#584,.T.);
#9243=EDGE_CURVE('',#7091,#7207,#585,.T.);
#9244=EDGE_CURVE('',#7207,#7208,#2036,.T.);
#9245=EDGE_CURVE('',#7208,#7086,#586,.T.);
#9246=EDGE_CURVE('',#7085,#7209,#587,.T.);
#9247=EDGE_CURVE('',#7209,#7210,#2037,.T.);
#9248=EDGE_CURVE('',#7210,#7080,#588,.T.);
#9249=EDGE_CURVE('',#7079,#7211,#589,.T.);
#9250=EDGE_CURVE('',#7211,#7212,#2038,.T.);
#9251=EDGE_CURVE('',#7212,#7074,#590,.T.);
#9252=EDGE_CURVE('',#7073,#7213,#591,.T.);
#9253=EDGE_CURVE('',#7213,#7214,#2039,.T.);
#9254=EDGE_CURVE('',#7214,#7068,#592,.T.);
#9255=EDGE_CURVE('',#7067,#7215,#593,.T.);
#9256=EDGE_CURVE('',#7215,#7216,#2040,.T.);
#9257=EDGE_CURVE('',#7216,#7062,#594,.T.);
#9258=EDGE_CURVE('',#7061,#7217,#595,.T.);
#9259=EDGE_CURVE('',#7217,#7218,#2041,.T.);
#9260=EDGE_CURVE('',#7218,#7056,#596,.T.);
#9261=EDGE_CURVE('',#7055,#7219,#597,.T.);
#9262=EDGE_CURVE('',#7219,#7220,#2042,.T.);
#9263=EDGE_CURVE('',#7220,#7050,#598,.T.);
#9264=EDGE_CURVE('',#7049,#7221,#599,.T.);
#9265=EDGE_CURVE('',#7221,#7222,#2043,.F.);
#9266=EDGE_CURVE('',#7222,#7223,#600,.T.);
#9267=EDGE_CURVE('',#7223,#7043,#601,.T.);
#9268=EDGE_CURVE('',#7042,#7224,#602,.T.);
#9269=EDGE_CURVE('',#7224,#7225,#603,.T.);
#9270=EDGE_CURVE('',#7225,#7226,#604,.T.);
#9271=EDGE_CURVE('',#7226,#7227,#605,.T.);
#9272=EDGE_CURVE('',#7227,#7032,#606,.T.);
#9273=EDGE_CURVE('',#7031,#7228,#607,.T.);
#9274=EDGE_CURVE('',#7228,#7229,#608,.T.);
#9275=EDGE_CURVE('',#7229,#7230,#609,.T.);
#9276=EDGE_CURVE('',#7230,#7231,#610,.T.);
#9277=EDGE_CURVE('',#7231,#7024,#611,.T.);
#9278=EDGE_CURVE('',#7023,#7232,#612,.T.);
#9279=EDGE_CURVE('',#7232,#7233,#613,.T.);
#9280=EDGE_CURVE('',#7233,#7234,#2044,.F.);
#9281=EDGE_CURVE('',#7234,#7235,#614,.T.);
#9282=EDGE_CURVE('',#7235,#7016,#615,.T.);
#9283=EDGE_CURVE('',#7015,#7236,#616,.T.);
#9284=EDGE_CURVE('',#7236,#7237,#617,.T.);
#9285=EDGE_CURVE('',#7237,#7238,#2045,.F.);
#9286=EDGE_CURVE('',#7238,#7239,#618,.T.);
#9287=EDGE_CURVE('',#7239,#7008,#619,.T.);
#9288=EDGE_CURVE('',#7007,#7240,#620,.T.);
#9289=EDGE_CURVE('',#7240,#7241,#621,.T.);
#9290=EDGE_CURVE('',#7241,#7242,#622,.F.);
#9291=EDGE_CURVE('',#7242,#7243,#623,.F.);
#9292=EDGE_CURVE('',#7243,#7244,#624,.F.);
#9293=EDGE_CURVE('',#7244,#7245,#625,.F.);
#9294=EDGE_CURVE('',#7245,#7246,#2046,.F.);
#9295=EDGE_CURVE('',#7246,#7247,#6075,.F.);
#9296=EDGE_CURVE('',#7247,#7248,#626,.F.);
#9297=EDGE_CURVE('',#7248,#7249,#627,.T.);
#9298=EDGE_CURVE('',#7249,#7250,#628,.T.);
#9299=EDGE_CURVE('',#7250,#7251,#629,.T.);
#9300=EDGE_CURVE('',#7251,#7252,#630,.T.);
#9301=EDGE_CURVE('',#7252,#7253,#631,.T.);
#9302=EDGE_CURVE('',#7253,#7254,#632,.T.);
#9303=EDGE_CURVE('',#7254,#7255,#633,.T.);
#9304=EDGE_CURVE('',#7255,#7256,#634,.T.);
#9305=EDGE_CURVE('',#7256,#7257,#635,.F.);
#9306=EDGE_CURVE('',#7257,#7258,#6076,.F.);
#9307=EDGE_CURVE('',#7258,#7259,#2047,.F.);
#9308=EDGE_CURVE('',#7259,#7260,#6077,.F.);
#9309=EDGE_CURVE('',#7260,#7261,#636,.F.);
#9310=EDGE_CURVE('',#7261,#7262,#637,.F.);
#9311=EDGE_CURVE('',#7262,#7263,#638,.F.);
#9312=EDGE_CURVE('',#7263,#7264,#639,.F.);
#9313=EDGE_CURVE('',#7264,#7265,#640,.T.);
#9314=EDGE_CURVE('',#7265,#7266,#641,.T.);
#9315=EDGE_CURVE('',#7266,#7267,#642,.T.);
#9316=EDGE_CURVE('',#7267,#7268,#643,.T.);
#9317=EDGE_CURVE('',#7268,#7269,#644,.F.);
#9318=EDGE_CURVE('',#7269,#7270,#645,.F.);
#9319=EDGE_CURVE('',#7270,#7271,#646,.F.);
#9320=EDGE_CURVE('',#7271,#7272,#2048,.F.);
#9321=EDGE_CURVE('',#7272,#7273,#6078,.F.);
#9322=EDGE_CURVE('',#7273,#7274,#647,.F.);
#9323=EDGE_CURVE('',#7274,#7275,#648,.T.);
#9324=EDGE_CURVE('',#7275,#7276,#649,.T.);
#9325=EDGE_CURVE('',#7276,#6993,#650,.T.);
#9326=EDGE_CURVE('',#7277,#7278,#2049,.T.);
#9327=EDGE_CURVE('',#7278,#7279,#651,.F.);
#9328=EDGE_CURVE('',#7279,#7280,#652,.T.);
#9329=EDGE_CURVE('',#7280,#7281,#2050,.T.);
#9330=EDGE_CURVE('',#7281,#7282,#653,.T.);
#9331=EDGE_CURVE('',#7282,#7277,#654,.T.);
#9332=EDGE_CURVE('',#7283,#7284,#2051,.T.);
#9333=EDGE_CURVE('',#7284,#7285,#655,.T.);
#9334=EDGE_CURVE('',#7285,#7286,#656,.T.);
#9335=EDGE_CURVE('',#7286,#7287,#2052,.T.);
#9336=EDGE_CURVE('',#7287,#7288,#657,.T.);
#9337=EDGE_CURVE('',#7288,#7283,#658,.T.);
#9338=EDGE_CURVE('',#7289,#7290,#2053,.T.);
#9339=EDGE_CURVE('',#7290,#7291,#659,.T.);
#9340=EDGE_CURVE('',#7291,#7292,#660,.T.);
#9341=EDGE_CURVE('',#7292,#7293,#2054,.T.);
#9342=EDGE_CURVE('',#7293,#7294,#661,.T.);
#9343=EDGE_CURVE('',#7294,#7289,#662,.T.);
#9344=EDGE_CURVE('',#7295,#7296,#2055,.T.);
#9345=EDGE_CURVE('',#7296,#7297,#663,.T.);
#9346=EDGE_CURVE('',#7297,#7298,#664,.T.);
#9347=EDGE_CURVE('',#7298,#7299,#2056,.T.);
#9348=EDGE_CURVE('',#7299,#7300,#665,.T.);
#9349=EDGE_CURVE('',#7300,#7295,#666,.T.);
#9350=EDGE_CURVE('',#7301,#7302,#2057,.T.);
#9351=EDGE_CURVE('',#7302,#7303,#667,.T.);
#9352=EDGE_CURVE('',#7303,#7304,#668,.T.);
#9353=EDGE_CURVE('',#7304,#7305,#2058,.T.);
#9354=EDGE_CURVE('',#7305,#7306,#669,.T.);
#9355=EDGE_CURVE('',#7306,#7301,#670,.T.);
#9356=EDGE_CURVE('',#7307,#7308,#2059,.T.);
#9357=EDGE_CURVE('',#7308,#7309,#671,.T.);
#9358=EDGE_CURVE('',#7309,#7310,#672,.T.);
#9359=EDGE_CURVE('',#7310,#7311,#2060,.T.);
#9360=EDGE_CURVE('',#7311,#7312,#673,.T.);
#9361=EDGE_CURVE('',#7312,#7307,#674,.T.);
#9362=EDGE_CURVE('',#7313,#7314,#2061,.F.);
#9363=EDGE_CURVE('',#7314,#7315,#675,.T.);
#9364=EDGE_CURVE('',#7315,#7316,#676,.T.);
#9365=EDGE_CURVE('',#7316,#7317,#677,.T.);
#9366=EDGE_CURVE('',#7317,#7318,#678,.T.);
#9367=EDGE_CURVE('',#7318,#7319,#2062,.F.);
#9368=EDGE_CURVE('',#7319,#7320,#679,.T.);
#9369=EDGE_CURVE('',#7320,#7321,#680,.T.);
#9370=EDGE_CURVE('',#7321,#7322,#681,.T.);
#9371=EDGE_CURVE('',#7322,#7313,#682,.T.);
#9372=EDGE_CURVE('',#7323,#7324,#2063,.T.);
#9373=EDGE_CURVE('',#7324,#7325,#683,.T.);
#9374=EDGE_CURVE('',#7325,#7326,#684,.T.);
#9375=EDGE_CURVE('',#7326,#7327,#2064,.T.);
#9376=EDGE_CURVE('',#7327,#7328,#685,.T.);
#9377=EDGE_CURVE('',#7328,#7323,#686,.T.);
#9378=EDGE_CURVE('',#7329,#7330,#2065,.T.);
#9379=EDGE_CURVE('',#7330,#7331,#687,.T.);
#9380=EDGE_CURVE('',#7331,#7332,#688,.T.);
#9381=EDGE_CURVE('',#7332,#7333,#2066,.T.);
#9382=EDGE_CURVE('',#7333,#7334,#689,.T.);
#9383=EDGE_CURVE('',#7334,#7329,#690,.T.);
#9384=EDGE_CURVE('',#7335,#7336,#2067,.T.);
#9385=EDGE_CURVE('',#7336,#7337,#691,.T.);
#9386=EDGE_CURVE('',#7337,#7338,#692,.T.);
#9387=EDGE_CURVE('',#7338,#7339,#2068,.T.);
#9388=EDGE_CURVE('',#7339,#7340,#693,.T.);
#9389=EDGE_CURVE('',#7340,#7335,#694,.T.);
#9390=EDGE_CURVE('',#7341,#7342,#2069,.T.);
#9391=EDGE_CURVE('',#7342,#7343,#695,.T.);
#9392=EDGE_CURVE('',#7343,#7344,#696,.T.);
#9393=EDGE_CURVE('',#7344,#7345,#2070,.T.);
#9394=EDGE_CURVE('',#7345,#7346,#697,.T.);
#9395=EDGE_CURVE('',#7346,#7341,#698,.T.);
#9396=EDGE_CURVE('',#7347,#7348,#2071,.T.);
#9397=EDGE_CURVE('',#7348,#7349,#699,.T.);
#9398=EDGE_CURVE('',#7349,#7350,#700,.T.);
#9399=EDGE_CURVE('',#7350,#7351,#2072,.T.);
#9400=EDGE_CURVE('',#7351,#7352,#701,.T.);
#9401=EDGE_CURVE('',#7352,#7347,#702,.T.);
#9402=EDGE_CURVE('',#7353,#7354,#2073,.F.);
#9403=EDGE_CURVE('',#7354,#7355,#703,.T.);
#9404=EDGE_CURVE('',#7355,#7356,#704,.T.);
#9405=EDGE_CURVE('',#7356,#7357,#705,.T.);
#9406=EDGE_CURVE('',#7357,#7358,#706,.T.);
#9407=EDGE_CURVE('',#7358,#7359,#2074,.F.);
#9408=EDGE_CURVE('',#7359,#7360,#707,.T.);
#9409=EDGE_CURVE('',#7360,#7361,#708,.T.);
#9410=EDGE_CURVE('',#7361,#7362,#709,.T.);
#9411=EDGE_CURVE('',#7362,#7353,#710,.T.);
#9412=EDGE_CURVE('',#7363,#7364,#711,.T.);
#9413=EDGE_CURVE('',#7364,#7365,#712,.T.);
#9414=EDGE_CURVE('',#7365,#7366,#713,.T.);
#9415=EDGE_CURVE('',#7366,#7367,#714,.T.);
#9416=EDGE_CURVE('',#7367,#7368,#715,.T.);
#9417=EDGE_CURVE('',#7368,#7369,#716,.T.);
#9418=EDGE_CURVE('',#7369,#7370,#717,.T.);
#9419=EDGE_CURVE('',#7370,#7371,#718,.T.);
#9420=EDGE_CURVE('',#7371,#7372,#719,.T.);
#9421=EDGE_CURVE('',#7372,#7363,#720,.T.);
#9422=EDGE_CURVE('',#7373,#7374,#721,.T.);
#9423=EDGE_CURVE('',#7374,#7375,#722,.T.);
#9424=EDGE_CURVE('',#7375,#7376,#723,.T.);
#9425=EDGE_CURVE('',#7376,#7377,#724,.T.);
#9426=EDGE_CURVE('',#7377,#7378,#725,.T.);
#9427=EDGE_CURVE('',#7378,#7379,#726,.T.);
#9428=EDGE_CURVE('',#7379,#7380,#727,.T.);
#9429=EDGE_CURVE('',#7380,#7381,#728,.T.);
#9430=EDGE_CURVE('',#7381,#7382,#729,.F.);
#9431=EDGE_CURVE('',#7382,#7383,#730,.F.);
#9432=EDGE_CURVE('',#7383,#7384,#731,.F.);
#9433=EDGE_CURVE('',#7384,#7373,#732,.F.);
#9434=EDGE_CURVE('',#7385,#7386,#2075,.F.);
#9435=EDGE_CURVE('',#7386,#7387,#733,.T.);
#9436=EDGE_CURVE('',#7387,#7388,#734,.T.);
#9437=EDGE_CURVE('',#7388,#7389,#2076,.F.);
#9438=EDGE_CURVE('',#7389,#7390,#735,.T.);
#9439=EDGE_CURVE('',#7390,#7391,#736,.T.);
#9440=EDGE_CURVE('',#7391,#7392,#737,.T.);
#9441=EDGE_CURVE('',#7392,#7385,#738,.T.);
#9442=EDGE_CURVE('',#7393,#7394,#739,.F.);
#9443=EDGE_CURVE('',#7394,#7395,#740,.T.);
#9444=EDGE_CURVE('',#7395,#7396,#741,.T.);
#9445=EDGE_CURVE('',#7396,#7397,#742,.F.);
#9446=EDGE_CURVE('',#7397,#7398,#743,.F.);
#9447=EDGE_CURVE('',#7398,#7399,#744,.F.);
#9448=EDGE_CURVE('',#7399,#7400,#745,.F.);
#9449=EDGE_CURVE('',#7400,#7401,#746,.T.);
#9450=EDGE_CURVE('',#7401,#7402,#747,.T.);
#9451=EDGE_CURVE('',#7402,#7403,#748,.T.);
#9452=EDGE_CURVE('',#7403,#7393,#749,.F.);
#9453=EDGE_CURVE('',#6980,#6986,#750,.T.);
#9454=EDGE_CURVE('',#6985,#6979,#751,.F.);
#9455=EDGE_CURVE('',#7169,#7179,#2077,.T.);
#9456=EDGE_CURVE('',#7181,#7172,#2078,.T.);
#9457=EDGE_CURVE('',#7175,#7404,#752,.T.);
#9458=EDGE_CURVE('',#7404,#7405,#753,.F.);
#9459=EDGE_CURVE('',#7176,#7405,#754,.F.);
#9460=EDGE_CURVE('',#7405,#7406,#755,.F.);
#9461=EDGE_CURVE('',#7173,#7406,#756,.F.);
#9462=EDGE_CURVE('',#7407,#7408,#757,.T.);
#9463=EDGE_CURVE('',#7408,#7409,#6079,.F.);
#9464=EDGE_CURVE('',#7409,#7410,#758,.T.);
#9465=EDGE_CURVE('',#7410,#7411,#759,.T.);
#9466=EDGE_CURVE('',#7411,#7407,#2079,.T.);
#9467=EDGE_CURVE('',#7412,#7413,#2080,.T.);
#9468=EDGE_CURVE('',#7413,#7414,#760,.T.);
#9469=EDGE_CURVE('',#7414,#7415,#761,.T.);
#9470=EDGE_CURVE('',#7415,#7416,#6080,.F.);
#9471=EDGE_CURVE('',#7416,#7412,#762,.T.);
#9472=EDGE_CURVE('',#7417,#7418,#2081,.T.);
#9473=EDGE_CURVE('',#7417,#7419,#763,.T.);
#9474=EDGE_CURVE('',#7419,#7420,#764,.T.);
#9475=EDGE_CURVE('',#7420,#7421,#765,.T.);
#9476=EDGE_CURVE('',#7421,#7418,#766,.T.);
#9477=EDGE_CURVE('',#7422,#7423,#767,.T.);
#9478=EDGE_CURVE('',#7423,#7424,#6081,.F.);
#9479=EDGE_CURVE('',#7424,#7425,#768,.T.);
#9480=EDGE_CURVE('',#7425,#7426,#769,.T.);
#9481=EDGE_CURVE('',#7422,#7426,#2082,.T.);
#9482=EDGE_CURVE('',#7427,#7404,#770,.F.);
#9483=EDGE_CURVE('',#7406,#7427,#771,.F.);
#9484=EDGE_CURVE('',#6973,#7428,#6082,.F.);
#9485=EDGE_CURVE('',#7428,#7429,#772,.T.);
#9486=EDGE_CURVE('',#7429,#7430,#773,.T.);
#9487=EDGE_CURVE('',#7430,#7431,#6083,.F.);
#9488=EDGE_CURVE('',#7431,#6977,#774,.T.);
#9489=EDGE_CURVE('',#6976,#7432,#6084,.F.);
#9490=EDGE_CURVE('',#7432,#7433,#775,.T.);
#9491=EDGE_CURVE('',#7433,#7434,#776,.F.);
#9492=EDGE_CURVE('',#7434,#7435,#777,.T.);
#9493=EDGE_CURVE('',#7435,#7436,#778,.F.);
#9494=EDGE_CURVE('',#7436,#7437,#779,.T.);
#9495=EDGE_CURVE('',#7437,#7438,#6085,.F.);
#9496=EDGE_CURVE('',#7438,#7439,#780,.T.);
#9497=EDGE_CURVE('',#7439,#7440,#781,.F.);
#9498=EDGE_CURVE('',#7440,#6972,#782,.T.);
#9499=EDGE_CURVE('',#7127,#7441,#783,.T.);
#9500=EDGE_CURVE('',#7441,#7442,#784,.T.);
#9501=EDGE_CURVE('',#7442,#7443,#785,.F.);
#9502=EDGE_CURVE('',#7443,#7444,#786,.T.);
#9503=EDGE_CURVE('',#7444,#7445,#787,.T.);
#9504=EDGE_CURVE('',#7445,#7446,#788,.T.);
#9505=EDGE_CURVE('',#7446,#7127,#789,.T.);
#9506=EDGE_CURVE('',#7411,#7447,#790,.T.);
#9507=EDGE_CURVE('',#7447,#7417,#791,.T.);
#9508=EDGE_CURVE('',#7418,#7448,#792,.T.);
#9509=EDGE_CURVE('',#7448,#7407,#793,.T.);
#9510=EDGE_CURVE('',#7426,#7449,#794,.T.);
#9511=EDGE_CURVE('',#7449,#7413,#795,.T.);
#9512=EDGE_CURVE('',#7412,#7450,#796,.T.);
#9513=EDGE_CURVE('',#7450,#7422,#797,.T.);
#9514=EDGE_CURVE('',#7187,#7451,#798,.T.);
#9515=EDGE_CURVE('',#7451,#7452,#799,.T.);
#9516=EDGE_CURVE('',#7452,#7453,#800,.F.);
#9517=EDGE_CURVE('',#7453,#7454,#801,.T.);
#9518=EDGE_CURVE('',#7454,#7455,#71,.T.);
#9519=EDGE_CURVE('',#7455,#7456,#802,.T.);
#9520=EDGE_CURVE('',#7456,#7187,#803,.T.);
#9521=EDGE_CURVE('',#7457,#7458,#2083,.T.);
#9522=EDGE_CURVE('',#7458,#7459,#804,.T.);
#9523=EDGE_CURVE('',#7459,#7460,#805,.T.);
#9524=EDGE_CURVE('',#7460,#7461,#806,.T.);
#9525=EDGE_CURVE('',#7461,#7462,#807,.T.);
#9526=EDGE_CURVE('',#7462,#7463,#2084,.T.);
#9527=EDGE_CURVE('',#7463,#7457,#808,.T.);
#9528=EDGE_CURVE('',#7462,#7464,#809,.T.);
#9529=EDGE_CURVE('',#7464,#7465,#810,.T.);
#9530=EDGE_CURVE('',#7465,#7466,#811,.T.);
#9531=EDGE_CURVE('',#7466,#7467,#812,.T.);
#9532=EDGE_CURVE('',#7467,#7468,#813,.T.);
#9533=EDGE_CURVE('',#7468,#7469,#2085,.T.);
#9534=EDGE_CURVE('',#7469,#7470,#814,.T.);
#9535=EDGE_CURVE('',#7470,#7471,#815,.T.);
#9536=EDGE_CURVE('',#7471,#7472,#816,.T.);
#9537=EDGE_CURVE('',#7472,#7473,#817,.T.);
#9538=EDGE_CURVE('',#7473,#7463,#818,.T.);
#9539=EDGE_CURVE('',#7474,#7475,#2086,.T.);
#9540=EDGE_CURVE('',#7475,#7476,#819,.T.);
#9541=EDGE_CURVE('',#7476,#7477,#820,.T.);
#9542=EDGE_CURVE('',#7477,#7478,#821,.T.);
#9543=EDGE_CURVE('',#7478,#7479,#822,.T.);
#9544=EDGE_CURVE('',#7479,#7458,#823,.T.);
#9545=EDGE_CURVE('',#7457,#7480,#824,.T.);
#9546=EDGE_CURVE('',#7480,#7481,#825,.T.);
#9547=EDGE_CURVE('',#7481,#7482,#826,.T.);
#9548=EDGE_CURVE('',#7482,#7483,#827,.T.);
#9549=EDGE_CURVE('',#7483,#7474,#828,.T.);
#9550=EDGE_CURVE('',#7468,#7484,#829,.T.);
#9551=EDGE_CURVE('',#7484,#7485,#830,.T.);
#9552=EDGE_CURVE('',#7485,#7486,#831,.T.);
#9553=EDGE_CURVE('',#7486,#7475,#832,.T.);
#9554=EDGE_CURVE('',#7474,#7469,#833,.T.);
#9555=EDGE_CURVE('',#7451,#7487,#834,.T.);
#9556=EDGE_CURVE('',#7487,#7488,#6086,.T.);
#9557=EDGE_CURVE('',#7488,#7452,#835,.T.);
#9558=EDGE_CURVE('',#7455,#7489,#836,.T.);
#9559=EDGE_CURVE('',#7489,#7490,#837,.T.);
#9560=EDGE_CURVE('',#7490,#7456,#838,.T.);
#9561=EDGE_CURVE('',#7491,#7492,#6087,.T.);
#9562=EDGE_CURVE('',#7492,#7446,#839,.T.);
#9563=EDGE_CURVE('',#7445,#7491,#840,.T.);
#9564=EDGE_CURVE('',#7441,#7493,#841,.T.);
#9565=EDGE_CURVE('',#7493,#7494,#6088,.T.);
#9566=EDGE_CURVE('',#7494,#7442,#842,.T.);
#9567=EDGE_CURVE('',#7407,#7434,#6089,.T.);
#9568=EDGE_CURVE('',#7435,#7418,#6090,.T.);
#9569=EDGE_CURVE('',#7436,#7421,#843,.F.);
#9570=EDGE_CURVE('',#7433,#7408,#6091,.F.);
#9571=EDGE_CURVE('',#7420,#7489,#844,.F.);
#9572=EDGE_CURVE('',#7437,#7454,#845,.T.);
#9573=EDGE_CURVE('',#7494,#7433,#6092,.F.);
#9574=EDGE_CURVE('',#7443,#7432,#846,.T.);
#9575=EDGE_CURVE('',#7438,#7453,#847,.F.);
#9576=EDGE_CURVE('',#7444,#6976,#848,.F.);
#9577=EDGE_CURVE('',#7488,#7439,#6093,.F.);
#9578=EDGE_CURVE('',#6975,#7491,#6094,.T.);
#9579=EDGE_CURVE('',#7439,#7423,#6095,.F.);
#9580=EDGE_CURVE('',#7440,#7422,#6096,.F.);
#9581=EDGE_CURVE('',#7416,#6975,#6097,.F.);
#9582=EDGE_CURVE('',#7412,#6974,#6098,.F.);
#9583=EDGE_CURVE('',#7457,#7428,#849,.T.);
#9584=EDGE_CURVE('',#7430,#7463,#850,.T.);
#9585=EDGE_CURVE('',#7431,#7469,#851,.F.);
#9586=EDGE_CURVE('',#7474,#6978,#852,.F.);
#9587=EDGE_CURVE('',#7491,#7416,#6099,.T.);
#9588=EDGE_CURVE('',#7415,#7492,#6100,.F.);
#9589=EDGE_CURVE('',#7130,#7415,#6101,.T.);
#9590=EDGE_CURVE('',#7131,#7413,#6102,.F.);
#9591=EDGE_CURVE('',#7183,#7426,#6103,.T.);
#9592=EDGE_CURVE('',#7424,#7184,#6104,.T.);
#9593=EDGE_CURVE('',#7193,#7493,#6105,.F.);
#9594=EDGE_CURVE('',#7125,#7441,#853,.T.);
#9595=EDGE_CURVE('',#7129,#7446,#854,.F.);
#9596=EDGE_CURVE('',#7130,#7492,#6106,.T.);
#9597=EDGE_CURVE('',#7451,#7185,#855,.F.);
#9598=EDGE_CURVE('',#7487,#7184,#6107,.T.);
#9599=EDGE_CURVE('',#7487,#7424,#6108,.T.);
#9600=EDGE_CURVE('',#7488,#7423,#6109,.T.);
#9601=EDGE_CURVE('',#7189,#7456,#856,.F.);
#9602=EDGE_CURVE('',#7190,#7490,#857,.T.);
#9603=EDGE_CURVE('',#7191,#7417,#6110,.F.);
#9604=EDGE_CURVE('',#7192,#7411,#6111,.T.);
#9605=EDGE_CURVE('',#7193,#7409,#6112,.F.);
#9606=EDGE_CURVE('',#7493,#7409,#6113,.T.);
#9607=EDGE_CURVE('',#7494,#7408,#6114,.T.);
#9608=EDGE_CURVE('',#6981,#7475,#6115,.F.);
#9609=EDGE_CURVE('',#7458,#6984,#6116,.F.);
#9610=EDGE_CURVE('',#7462,#6983,#6117,.T.);
#9611=EDGE_CURVE('',#6982,#7468,#6118,.T.);
#9612=EDGE_CURVE('',#7427,#7174,#858,.T.);
#9613=EDGE_CURVE('',#7140,#7495,#859,.T.);
#9614=EDGE_CURVE('',#7495,#7496,#860,.F.);
#9615=EDGE_CURVE('',#7496,#7497,#6119,.F.);
#9616=EDGE_CURVE('',#7497,#7498,#861,.T.);
#9617=EDGE_CURVE('',#7498,#7499,#6120,.F.);
#9618=EDGE_CURVE('',#7499,#7500,#862,.F.);
#9619=EDGE_CURVE('',#7500,#7141,#863,.F.);
#9620=EDGE_CURVE('',#7501,#7502,#864,.T.);
#9621=EDGE_CURVE('',#7502,#7503,#865,.T.);
#9622=EDGE_CURVE('',#7503,#7504,#866,.T.);
#9623=EDGE_CURVE('',#7504,#7505,#867,.T.);
#9624=EDGE_CURVE('',#7505,#7506,#868,.T.);
#9625=EDGE_CURVE('',#7506,#7501,#869,.T.);
#9626=EDGE_CURVE('',#7507,#7508,#870,.T.);
#9627=EDGE_CURVE('',#7508,#7509,#871,.T.);
#9628=EDGE_CURVE('',#7509,#7510,#872,.T.);
#9629=EDGE_CURVE('',#7510,#7511,#873,.T.);
#9630=EDGE_CURVE('',#7511,#7512,#874,.T.);
#9631=EDGE_CURVE('',#7512,#7507,#875,.T.);
#9632=EDGE_CURVE('',#7513,#7514,#876,.T.);
#9633=EDGE_CURVE('',#7514,#7515,#877,.T.);
#9634=EDGE_CURVE('',#7515,#7516,#878,.T.);
#9635=EDGE_CURVE('',#7516,#7517,#879,.T.);
#9636=EDGE_CURVE('',#7517,#7518,#880,.T.);
#9637=EDGE_CURVE('',#7518,#7513,#881,.T.);
#9638=EDGE_CURVE('',#7519,#7520,#882,.T.);
#9639=EDGE_CURVE('',#7520,#7521,#883,.T.);
#9640=EDGE_CURVE('',#7521,#7522,#884,.T.);
#9641=EDGE_CURVE('',#7522,#7523,#885,.T.);
#9642=EDGE_CURVE('',#7523,#7524,#886,.T.);
#9643=EDGE_CURVE('',#7524,#7519,#887,.T.);
#9644=EDGE_CURVE('',#7525,#7526,#888,.T.);
#9645=EDGE_CURVE('',#7526,#7527,#889,.T.);
#9646=EDGE_CURVE('',#7527,#7528,#890,.T.);
#9647=EDGE_CURVE('',#7528,#7529,#891,.T.);
#9648=EDGE_CURVE('',#7529,#7530,#892,.T.);
#9649=EDGE_CURVE('',#7530,#7525,#893,.T.);
#9650=EDGE_CURVE('',#7531,#7532,#894,.T.);
#9651=EDGE_CURVE('',#7532,#7533,#895,.T.);
#9652=EDGE_CURVE('',#7533,#7534,#896,.T.);
#9653=EDGE_CURVE('',#7534,#7535,#897,.T.);
#9654=EDGE_CURVE('',#7535,#7536,#898,.T.);
#9655=EDGE_CURVE('',#7536,#7531,#899,.T.);
#9656=EDGE_CURVE('',#7537,#7538,#900,.T.);
#9657=EDGE_CURVE('',#7538,#7539,#901,.T.);
#9658=EDGE_CURVE('',#7539,#7540,#902,.T.);
#9659=EDGE_CURVE('',#7540,#7541,#903,.T.);
#9660=EDGE_CURVE('',#7541,#7542,#904,.T.);
#9661=EDGE_CURVE('',#7542,#7537,#905,.T.);
#9662=EDGE_CURVE('',#7543,#7544,#906,.T.);
#9663=EDGE_CURVE('',#7544,#7545,#907,.T.);
#9664=EDGE_CURVE('',#7545,#7546,#908,.T.);
#9665=EDGE_CURVE('',#7546,#7547,#909,.T.);
#9666=EDGE_CURVE('',#7547,#7548,#910,.T.);
#9667=EDGE_CURVE('',#7548,#7543,#911,.T.);
#9668=EDGE_CURVE('',#7549,#7550,#912,.T.);
#9669=EDGE_CURVE('',#7550,#7551,#913,.T.);
#9670=EDGE_CURVE('',#7551,#7552,#914,.T.);
#9671=EDGE_CURVE('',#7552,#7553,#915,.T.);
#9672=EDGE_CURVE('',#7553,#7554,#916,.T.);
#9673=EDGE_CURVE('',#7554,#7549,#917,.T.);
#9674=EDGE_CURVE('',#7555,#7556,#918,.T.);
#9675=EDGE_CURVE('',#7556,#7557,#919,.T.);
#9676=EDGE_CURVE('',#7557,#7558,#920,.T.);
#9677=EDGE_CURVE('',#7558,#7559,#921,.T.);
#9678=EDGE_CURVE('',#7559,#7560,#922,.T.);
#9679=EDGE_CURVE('',#7560,#7555,#923,.T.);
#9680=EDGE_CURVE('',#7561,#7562,#924,.T.);
#9681=EDGE_CURVE('',#7562,#7563,#925,.T.);
#9682=EDGE_CURVE('',#7563,#7564,#926,.T.);
#9683=EDGE_CURVE('',#7564,#7565,#927,.T.);
#9684=EDGE_CURVE('',#7565,#7566,#928,.T.);
#9685=EDGE_CURVE('',#7566,#7561,#929,.T.);
#9686=EDGE_CURVE('',#7567,#7568,#930,.T.);
#9687=EDGE_CURVE('',#7568,#7569,#931,.T.);
#9688=EDGE_CURVE('',#7569,#7570,#932,.T.);
#9689=EDGE_CURVE('',#7570,#7571,#933,.T.);
#9690=EDGE_CURVE('',#7571,#7572,#934,.T.);
#9691=EDGE_CURVE('',#7572,#7567,#935,.T.);
#9692=EDGE_CURVE('',#7573,#7574,#936,.T.);
#9693=EDGE_CURVE('',#7574,#7575,#937,.T.);
#9694=EDGE_CURVE('',#7575,#7576,#938,.T.);
#9695=EDGE_CURVE('',#7576,#7577,#939,.T.);
#9696=EDGE_CURVE('',#7577,#7578,#940,.T.);
#9697=EDGE_CURVE('',#7578,#7573,#941,.T.);
#9698=EDGE_CURVE('',#7579,#7580,#942,.T.);
#9699=EDGE_CURVE('',#7580,#7581,#943,.T.);
#9700=EDGE_CURVE('',#7581,#7582,#944,.T.);
#9701=EDGE_CURVE('',#7582,#7583,#945,.T.);
#9702=EDGE_CURVE('',#7583,#7584,#946,.T.);
#9703=EDGE_CURVE('',#7584,#7579,#947,.T.);
#9704=EDGE_CURVE('',#7585,#7586,#948,.T.);
#9705=EDGE_CURVE('',#7586,#7587,#949,.T.);
#9706=EDGE_CURVE('',#7587,#7588,#950,.T.);
#9707=EDGE_CURVE('',#7588,#7589,#951,.T.);
#9708=EDGE_CURVE('',#7589,#7590,#952,.T.);
#9709=EDGE_CURVE('',#7590,#7585,#953,.T.);
#9710=EDGE_CURVE('',#7591,#7592,#954,.T.);
#9711=EDGE_CURVE('',#7592,#7593,#955,.T.);
#9712=EDGE_CURVE('',#7593,#7594,#956,.T.);
#9713=EDGE_CURVE('',#7594,#7595,#957,.T.);
#9714=EDGE_CURVE('',#7595,#7596,#958,.T.);
#9715=EDGE_CURVE('',#7596,#7591,#959,.T.);
#9716=EDGE_CURVE('',#7597,#7598,#960,.T.);
#9717=EDGE_CURVE('',#7598,#7599,#961,.T.);
#9718=EDGE_CURVE('',#7599,#7600,#962,.T.);
#9719=EDGE_CURVE('',#7600,#7601,#963,.T.);
#9720=EDGE_CURVE('',#7601,#7602,#964,.T.);
#9721=EDGE_CURVE('',#7602,#7597,#965,.T.);
#9722=EDGE_CURVE('',#7170,#7180,#966,.T.);
#9723=EDGE_CURVE('',#7171,#7182,#967,.F.);
#9724=EDGE_CURVE('',#7603,#7604,#968,.F.);
#9725=EDGE_CURVE('',#7605,#7603,#969,.F.);
#9726=EDGE_CURVE('',#7606,#7605,#970,.F.);
#9727=EDGE_CURVE('',#7607,#7606,#971,.F.);
#9728=EDGE_CURVE('',#7608,#7607,#972,.F.);
#9729=EDGE_CURVE('',#7604,#7608,#973,.F.);
#9730=EDGE_CURVE('',#7609,#7610,#974,.F.);
#9731=EDGE_CURVE('',#7611,#7609,#975,.F.);
#9732=EDGE_CURVE('',#7612,#7611,#976,.F.);
#9733=EDGE_CURVE('',#7613,#7612,#977,.F.);
#9734=EDGE_CURVE('',#7614,#7613,#978,.F.);
#9735=EDGE_CURVE('',#7610,#7614,#979,.F.);
#9736=EDGE_CURVE('',#7615,#7616,#980,.F.);
#9737=EDGE_CURVE('',#7617,#7615,#981,.F.);
#9738=EDGE_CURVE('',#7618,#7617,#982,.F.);
#9739=EDGE_CURVE('',#7619,#7618,#983,.F.);
#9740=EDGE_CURVE('',#7620,#7619,#984,.F.);
#9741=EDGE_CURVE('',#7616,#7620,#985,.F.);
#9742=EDGE_CURVE('',#7621,#7622,#986,.F.);
#9743=EDGE_CURVE('',#7623,#7621,#987,.F.);
#9744=EDGE_CURVE('',#7624,#7623,#988,.F.);
#9745=EDGE_CURVE('',#7625,#7624,#989,.F.);
#9746=EDGE_CURVE('',#7626,#7625,#990,.F.);
#9747=EDGE_CURVE('',#7622,#7626,#991,.F.);
#9748=EDGE_CURVE('',#7627,#7628,#992,.F.);
#9749=EDGE_CURVE('',#7629,#7627,#993,.F.);
#9750=EDGE_CURVE('',#7630,#7629,#994,.F.);
#9751=EDGE_CURVE('',#7631,#7630,#995,.F.);
#9752=EDGE_CURVE('',#7632,#7631,#996,.F.);
#9753=EDGE_CURVE('',#7628,#7632,#997,.F.);
#9754=EDGE_CURVE('',#7633,#7634,#998,.F.);
#9755=EDGE_CURVE('',#7635,#7633,#999,.F.);
#9756=EDGE_CURVE('',#7636,#7635,#1000,.F.);
#9757=EDGE_CURVE('',#7637,#7636,#1001,.F.);
#9758=EDGE_CURVE('',#7638,#7637,#1002,.F.);
#9759=EDGE_CURVE('',#7634,#7638,#1003,.F.);
#9760=EDGE_CURVE('',#7639,#7640,#1004,.F.);
#9761=EDGE_CURVE('',#7641,#7639,#1005,.F.);
#9762=EDGE_CURVE('',#7642,#7641,#1006,.F.);
#9763=EDGE_CURVE('',#7643,#7642,#1007,.F.);
#9764=EDGE_CURVE('',#7644,#7643,#1008,.F.);
#9765=EDGE_CURVE('',#7640,#7644,#1009,.F.);
#9766=EDGE_CURVE('',#7645,#7646,#1010,.F.);
#9767=EDGE_CURVE('',#7647,#7645,#1011,.F.);
#9768=EDGE_CURVE('',#7648,#7647,#1012,.F.);
#9769=EDGE_CURVE('',#7649,#7648,#1013,.F.);
#9770=EDGE_CURVE('',#7650,#7649,#1014,.F.);
#9771=EDGE_CURVE('',#7646,#7650,#1015,.F.);
#9772=EDGE_CURVE('',#7651,#7652,#1016,.F.);
#9773=EDGE_CURVE('',#7653,#7651,#1017,.F.);
#9774=EDGE_CURVE('',#7654,#7653,#1018,.F.);
#9775=EDGE_CURVE('',#7655,#7654,#1019,.F.);
#9776=EDGE_CURVE('',#7656,#7655,#1020,.F.);
#9777=EDGE_CURVE('',#7652,#7656,#1021,.F.);
#9778=EDGE_CURVE('',#7657,#7658,#1022,.F.);
#9779=EDGE_CURVE('',#7659,#7657,#1023,.F.);
#9780=EDGE_CURVE('',#7660,#7659,#1024,.F.);
#9781=EDGE_CURVE('',#7661,#7660,#1025,.F.);
#9782=EDGE_CURVE('',#7662,#7661,#1026,.F.);
#9783=EDGE_CURVE('',#7658,#7662,#1027,.F.);
#9784=EDGE_CURVE('',#7663,#7664,#1028,.F.);
#9785=EDGE_CURVE('',#7665,#7663,#1029,.F.);
#9786=EDGE_CURVE('',#7666,#7665,#1030,.F.);
#9787=EDGE_CURVE('',#7667,#7666,#1031,.F.);
#9788=EDGE_CURVE('',#7668,#7667,#1032,.F.);
#9789=EDGE_CURVE('',#7664,#7668,#1033,.F.);
#9790=EDGE_CURVE('',#7669,#7670,#1034,.F.);
#9791=EDGE_CURVE('',#7671,#7669,#1035,.F.);
#9792=EDGE_CURVE('',#7672,#7671,#1036,.F.);
#9793=EDGE_CURVE('',#7673,#7672,#1037,.F.);
#9794=EDGE_CURVE('',#7674,#7673,#1038,.F.);
#9795=EDGE_CURVE('',#7670,#7674,#1039,.F.);
#9796=EDGE_CURVE('',#7675,#7676,#1040,.F.);
#9797=EDGE_CURVE('',#7677,#7675,#1041,.F.);
#9798=EDGE_CURVE('',#7678,#7677,#1042,.F.);
#9799=EDGE_CURVE('',#7679,#7678,#1043,.F.);
#9800=EDGE_CURVE('',#7680,#7679,#1044,.F.);
#9801=EDGE_CURVE('',#7676,#7680,#1045,.F.);
#9802=EDGE_CURVE('',#7681,#7682,#1046,.F.);
#9803=EDGE_CURVE('',#7683,#7681,#1047,.F.);
#9804=EDGE_CURVE('',#7684,#7683,#1048,.F.);
#9805=EDGE_CURVE('',#7685,#7684,#1049,.F.);
#9806=EDGE_CURVE('',#7686,#7685,#1050,.F.);
#9807=EDGE_CURVE('',#7682,#7686,#1051,.F.);
#9808=EDGE_CURVE('',#7687,#7688,#1052,.F.);
#9809=EDGE_CURVE('',#7689,#7687,#1053,.F.);
#9810=EDGE_CURVE('',#7690,#7689,#1054,.F.);
#9811=EDGE_CURVE('',#7691,#7690,#1055,.F.);
#9812=EDGE_CURVE('',#7692,#7691,#1056,.F.);
#9813=EDGE_CURVE('',#7688,#7692,#1057,.F.);
#9814=EDGE_CURVE('',#7693,#7694,#1058,.F.);
#9815=EDGE_CURVE('',#7695,#7693,#1059,.F.);
#9816=EDGE_CURVE('',#7696,#7695,#1060,.F.);
#9817=EDGE_CURVE('',#7697,#7696,#1061,.F.);
#9818=EDGE_CURVE('',#7698,#7697,#1062,.F.);
#9819=EDGE_CURVE('',#7694,#7698,#1063,.F.);
#9820=EDGE_CURVE('',#7699,#7700,#1064,.F.);
#9821=EDGE_CURVE('',#7701,#7699,#1065,.F.);
#9822=EDGE_CURVE('',#7702,#7701,#1066,.F.);
#9823=EDGE_CURVE('',#7703,#7702,#1067,.F.);
#9824=EDGE_CURVE('',#7704,#7703,#1068,.F.);
#9825=EDGE_CURVE('',#7700,#7704,#1069,.F.);
#9826=EDGE_CURVE('',#7282,#7505,#1070,.F.);
#9827=EDGE_CURVE('',#7506,#7281,#1071,.T.);
#9828=EDGE_CURVE('',#7501,#7280,#1072,.T.);
#9829=EDGE_CURVE('',#7277,#7504,#1073,.T.);
#9830=EDGE_CURVE('',#7502,#7279,#1074,.T.);
#9831=EDGE_CURVE('',#7278,#7503,#1075,.F.);
#9832=EDGE_CURVE('',#7288,#7511,#1076,.F.);
#9833=EDGE_CURVE('',#7512,#7287,#1077,.T.);
#9834=EDGE_CURVE('',#7507,#7286,#1078,.T.);
#9835=EDGE_CURVE('',#7283,#7510,#1079,.T.);
#9836=EDGE_CURVE('',#7508,#7285,#1080,.T.);
#9837=EDGE_CURVE('',#7284,#7509,#1081,.F.);
#9838=EDGE_CURVE('',#7294,#7517,#1082,.F.);
#9839=EDGE_CURVE('',#7518,#7293,#1083,.T.);
#9840=EDGE_CURVE('',#7513,#7292,#1084,.T.);
#9841=EDGE_CURVE('',#7289,#7516,#1085,.T.);
#9842=EDGE_CURVE('',#7514,#7291,#1086,.T.);
#9843=EDGE_CURVE('',#7290,#7515,#1087,.F.);
#9844=EDGE_CURVE('',#7300,#7523,#1088,.F.);
#9845=EDGE_CURVE('',#7524,#7299,#1089,.T.);
#9846=EDGE_CURVE('',#7519,#7298,#1090,.T.);
#9847=EDGE_CURVE('',#7295,#7522,#1091,.T.);
#9848=EDGE_CURVE('',#7520,#7297,#1092,.T.);
#9849=EDGE_CURVE('',#7296,#7521,#1093,.F.);
#9850=EDGE_CURVE('',#7306,#7529,#1094,.F.);
#9851=EDGE_CURVE('',#7530,#7305,#1095,.T.);
#9852=EDGE_CURVE('',#7525,#7304,#1096,.T.);
#9853=EDGE_CURVE('',#7301,#7528,#1097,.T.);
#9854=EDGE_CURVE('',#7526,#7303,#1098,.T.);
#9855=EDGE_CURVE('',#7302,#7527,#1099,.F.);
#9856=EDGE_CURVE('',#7312,#7535,#1100,.F.);
#9857=EDGE_CURVE('',#7536,#7311,#1101,.T.);
#9858=EDGE_CURVE('',#7531,#7310,#1102,.T.);
#9859=EDGE_CURVE('',#7307,#7534,#1103,.T.);
#9860=EDGE_CURVE('',#7532,#7309,#1104,.T.);
#9861=EDGE_CURVE('',#7308,#7533,#1105,.F.);
#9862=EDGE_CURVE('',#7321,#7541,#1106,.F.);
#9863=EDGE_CURVE('',#7542,#7319,#1107,.T.);
#9864=EDGE_CURVE('',#7537,#7318,#1108,.T.);
#9865=EDGE_CURVE('',#7313,#7540,#1109,.T.);
#9866=EDGE_CURVE('',#7538,#7316,#1110,.T.);
#9867=EDGE_CURVE('',#7314,#7539,#1111,.F.);
#9868=EDGE_CURVE('',#7328,#7547,#1112,.F.);
#9869=EDGE_CURVE('',#7548,#7327,#1113,.T.);
#9870=EDGE_CURVE('',#7543,#7326,#1114,.T.);
#9871=EDGE_CURVE('',#7323,#7546,#1115,.T.);
#9872=EDGE_CURVE('',#7544,#7325,#1116,.T.);
#9873=EDGE_CURVE('',#7324,#7545,#1117,.F.);
#9874=EDGE_CURVE('',#7334,#7553,#1118,.F.);
#9875=EDGE_CURVE('',#7554,#7333,#1119,.T.);
#9876=EDGE_CURVE('',#7549,#7332,#1120,.T.);
#9877=EDGE_CURVE('',#7329,#7552,#1121,.T.);
#9878=EDGE_CURVE('',#7550,#7331,#1122,.T.);
#9879=EDGE_CURVE('',#7330,#7551,#1123,.F.);
#9880=EDGE_CURVE('',#7340,#7559,#1124,.F.);
#9881=EDGE_CURVE('',#7560,#7339,#1125,.T.);
#9882=EDGE_CURVE('',#7555,#7338,#1126,.T.);
#9883=EDGE_CURVE('',#7335,#7558,#1127,.T.);
#9884=EDGE_CURVE('',#7556,#7337,#1128,.T.);
#9885=EDGE_CURVE('',#7336,#7557,#1129,.F.);
#9886=EDGE_CURVE('',#7346,#7565,#1130,.F.);
#9887=EDGE_CURVE('',#7566,#7345,#1131,.T.);
#9888=EDGE_CURVE('',#7561,#7344,#1132,.T.);
#9889=EDGE_CURVE('',#7341,#7564,#1133,.T.);
#9890=EDGE_CURVE('',#7562,#7343,#1134,.T.);
#9891=EDGE_CURVE('',#7342,#7563,#1135,.F.);
#9892=EDGE_CURVE('',#7352,#7571,#1136,.F.);
#9893=EDGE_CURVE('',#7572,#7351,#1137,.T.);
#9894=EDGE_CURVE('',#7567,#7350,#1138,.T.);
#9895=EDGE_CURVE('',#7347,#7570,#1139,.T.);
#9896=EDGE_CURVE('',#7568,#7349,#1140,.T.);
#9897=EDGE_CURVE('',#7348,#7569,#1141,.F.);
#9898=EDGE_CURVE('',#7361,#7577,#1142,.F.);
#9899=EDGE_CURVE('',#7578,#7359,#1143,.T.);
#9900=EDGE_CURVE('',#7573,#7358,#1144,.T.);
#9901=EDGE_CURVE('',#7353,#7576,#1145,.T.);
#9902=EDGE_CURVE('',#7574,#7356,#1146,.T.);
#9903=EDGE_CURVE('',#7354,#7575,#1147,.F.);
#9904=EDGE_CURVE('',#7371,#7583,#1148,.F.);
#9905=EDGE_CURVE('',#7584,#7369,#1149,.T.);
#9906=EDGE_CURVE('',#7579,#7368,#1150,.T.);
#9907=EDGE_CURVE('',#7363,#7582,#1151,.F.);
#9908=EDGE_CURVE('',#7580,#7366,#1152,.T.);
#9909=EDGE_CURVE('',#7364,#7581,#1153,.F.);
#9910=EDGE_CURVE('',#7381,#7589,#1154,.T.);
#9911=EDGE_CURVE('',#7590,#7380,#1155,.T.);
#9912=EDGE_CURVE('',#7585,#7379,#1156,.T.);
#9913=EDGE_CURVE('',#7373,#7588,#1157,.F.);
#9914=EDGE_CURVE('',#7586,#7377,#1158,.T.);
#9915=EDGE_CURVE('',#7375,#7587,#1159,.F.);
#9916=EDGE_CURVE('',#7391,#7595,#1160,.F.);
#9917=EDGE_CURVE('',#7596,#7389,#1161,.T.);
#9918=EDGE_CURVE('',#7591,#7388,#1162,.F.);
#9919=EDGE_CURVE('',#7385,#7594,#1163,.T.);
#9920=EDGE_CURVE('',#7592,#7387,#1164,.T.);
#9921=EDGE_CURVE('',#7386,#7593,#1165,.F.);
#9922=EDGE_CURVE('',#7403,#7601,#1166,.T.);
#9923=EDGE_CURVE('',#7602,#7401,#1167,.T.);
#9924=EDGE_CURVE('',#7597,#7400,#1168,.T.);
#9925=EDGE_CURVE('',#7393,#7600,#1169,.F.);
#9926=EDGE_CURVE('',#7598,#7396,#1170,.F.);
#9927=EDGE_CURVE('',#7394,#7599,#1171,.F.);
#9928=EDGE_CURVE('',#7209,#7604,#1172,.T.);
#9929=EDGE_CURVE('',#7603,#7084,#1173,.T.);
#9930=EDGE_CURVE('',#7605,#7083,#1174,.T.);
#9931=EDGE_CURVE('',#7210,#7608,#1175,.F.);
#9932=EDGE_CURVE('',#7606,#7082,#1176,.T.);
#9933=EDGE_CURVE('',#7081,#7607,#1177,.F.);
#9934=EDGE_CURVE('',#7211,#7610,#1178,.T.);
#9935=EDGE_CURVE('',#7609,#7078,#1179,.T.);
#9936=EDGE_CURVE('',#7611,#7077,#1180,.T.);
#9937=EDGE_CURVE('',#7212,#7614,#1181,.F.);
#9938=EDGE_CURVE('',#7612,#7076,#1182,.T.);
#9939=EDGE_CURVE('',#7075,#7613,#1183,.F.);
#9940=EDGE_CURVE('',#7213,#7616,#1184,.T.);
#9941=EDGE_CURVE('',#7615,#7072,#1185,.T.);
#9942=EDGE_CURVE('',#7617,#7071,#1186,.T.);
#9943=EDGE_CURVE('',#7214,#7620,#1187,.F.);
#9944=EDGE_CURVE('',#7618,#7070,#1188,.T.);
#9945=EDGE_CURVE('',#7069,#7619,#1189,.F.);
#9946=EDGE_CURVE('',#7215,#7622,#1190,.T.);
#9947=EDGE_CURVE('',#7621,#7066,#1191,.T.);
#9948=EDGE_CURVE('',#7623,#7065,#1192,.T.);
#9949=EDGE_CURVE('',#7216,#7626,#1193,.F.);
#9950=EDGE_CURVE('',#7624,#7064,#1194,.T.);
#9951=EDGE_CURVE('',#7063,#7625,#1195,.F.);
#9952=EDGE_CURVE('',#7199,#7628,#1196,.T.);
#9953=EDGE_CURVE('',#7627,#7114,#1197,.T.);
#9954=EDGE_CURVE('',#7629,#7113,#1198,.T.);
#9955=EDGE_CURVE('',#7200,#7632,#1199,.F.);
#9956=EDGE_CURVE('',#7630,#7112,#1200,.T.);
#9957=EDGE_CURVE('',#7111,#7631,#1201,.F.);
#9958=EDGE_CURVE('',#7219,#7634,#1202,.T.);
#9959=EDGE_CURVE('',#7633,#7054,#1203,.T.);
#9960=EDGE_CURVE('',#7635,#7053,#1204,.T.);
#9961=EDGE_CURVE('',#7220,#7638,#1205,.F.);
#9962=EDGE_CURVE('',#7636,#7052,#1206,.T.);
#9963=EDGE_CURVE('',#7051,#7637,#1207,.F.);
#9964=EDGE_CURVE('',#7237,#7640,#1208,.T.);
#9965=EDGE_CURVE('',#7639,#7014,#1209,.T.);
#9966=EDGE_CURVE('',#7641,#7012,#1210,.T.);
#9967=EDGE_CURVE('',#7238,#7644,#1211,.F.);
#9968=EDGE_CURVE('',#7642,#7011,#1212,.F.);
#9969=EDGE_CURVE('',#7009,#7643,#1213,.F.);
#9970=EDGE_CURVE('',#7217,#7646,#1214,.T.);
#9971=EDGE_CURVE('',#7645,#7060,#1215,.T.);
#9972=EDGE_CURVE('',#7647,#7059,#1216,.T.);
#9973=EDGE_CURVE('',#7218,#7650,#1217,.F.);
#9974=EDGE_CURVE('',#7648,#7058,#1218,.T.);
#9975=EDGE_CURVE('',#7057,#7649,#1219,.F.);
#9976=EDGE_CURVE('',#7207,#7652,#1220,.T.);
#9977=EDGE_CURVE('',#7651,#7090,#1221,.T.);
#9978=EDGE_CURVE('',#7653,#7089,#1222,.T.);
#9979=EDGE_CURVE('',#7208,#7656,#1223,.F.);
#9980=EDGE_CURVE('',#7654,#7088,#1224,.T.);
#9981=EDGE_CURVE('',#7087,#7655,#1225,.F.);
#9982=EDGE_CURVE('',#7205,#7658,#1226,.T.);
#9983=EDGE_CURVE('',#7657,#7096,#1227,.T.);
#9984=EDGE_CURVE('',#7659,#7095,#1228,.T.);
#9985=EDGE_CURVE('',#7206,#7662,#1229,.F.);
#9986=EDGE_CURVE('',#7660,#7094,#1230,.T.);
#9987=EDGE_CURVE('',#7093,#7661,#1231,.F.);
#9988=EDGE_CURVE('',#7203,#7664,#1232,.T.);
#9989=EDGE_CURVE('',#7663,#7102,#1233,.T.);
#9990=EDGE_CURVE('',#7665,#7101,#1234,.T.);
#9991=EDGE_CURVE('',#7204,#7668,#1235,.F.);
#9992=EDGE_CURVE('',#7666,#7100,#1236,.T.);
#9993=EDGE_CURVE('',#7099,#7667,#1237,.F.);
#9994=EDGE_CURVE('',#7201,#7670,#1238,.T.);
#9995=EDGE_CURVE('',#7669,#7108,#1239,.T.);
#9996=EDGE_CURVE('',#7671,#7107,#1240,.T.);
#9997=EDGE_CURVE('',#7202,#7674,#1241,.F.);
#9998=EDGE_CURVE('',#7672,#7106,#1242,.T.);
#9999=EDGE_CURVE('',#7105,#7673,#1243,.F.);
#10000=EDGE_CURVE('',#7233,#7676,#1244,.T.);
#10001=EDGE_CURVE('',#7675,#7022,#1245,.T.);
#10002=EDGE_CURVE('',#7677,#7020,#1246,.T.);
#10003=EDGE_CURVE('',#7234,#7680,#1247,.F.);
#10004=EDGE_CURVE('',#7678,#7019,#1248,.T.);
#10005=EDGE_CURVE('',#7017,#7679,#1249,.F.);
#10006=EDGE_CURVE('',#7229,#7682,#1250,.F.);
#10007=EDGE_CURVE('',#7681,#7030,#1251,.T.);
#10008=EDGE_CURVE('',#7683,#7028,#1252,.T.);
#10009=EDGE_CURVE('',#7230,#7686,#1253,.F.);
#10010=EDGE_CURVE('',#7684,#7027,#1254,.T.);
#10011=EDGE_CURVE('',#7025,#7685,#1255,.F.);
#10012=EDGE_CURVE('',#7225,#7688,#1256,.F.);
#10013=EDGE_CURVE('',#7687,#7041,#1257,.T.);
#10014=EDGE_CURVE('',#7689,#7039,#1258,.T.);
#10015=EDGE_CURVE('',#7227,#7692,#1259,.F.);
#10016=EDGE_CURVE('',#7690,#7037,#1260,.T.);
#10017=EDGE_CURVE('',#7033,#7691,#1261,.T.);
#10018=EDGE_CURVE('',#7221,#7694,#1262,.T.);
#10019=EDGE_CURVE('',#7693,#7048,#1263,.T.);
#10020=EDGE_CURVE('',#7695,#7047,#1264,.T.);
#10021=EDGE_CURVE('',#7222,#7698,#1265,.F.);
#10022=EDGE_CURVE('',#7696,#7046,#1266,.F.);
#10023=EDGE_CURVE('',#7044,#7697,#1267,.F.);
#10024=EDGE_CURVE('',#7121,#7700,#1268,.T.);
#10025=EDGE_CURVE('',#7699,#7119,#1269,.T.);
#10026=EDGE_CURVE('',#7701,#7118,#1270,.T.);
#10027=EDGE_CURVE('',#7122,#7704,#1271,.F.);
#10028=EDGE_CURVE('',#7702,#7196,#1272,.F.);
#10029=EDGE_CURVE('',#7194,#7703,#1273,.F.);
#10030=EDGE_CURVE('',#7262,#7144,#1274,.F.);
#10031=EDGE_CURVE('',#7145,#7260,#1275,.F.);
#10032=EDGE_CURVE('',#7146,#7259,#1276,.T.);
#10033=EDGE_CURVE('',#7264,#7143,#1277,.F.);
#10034=EDGE_CURVE('',#7147,#7258,#1278,.F.);
#10035=EDGE_CURVE('',#7266,#7142,#1279,.F.);
#10036=EDGE_CURVE('',#7148,#7257,#1280,.F.);
#10037=EDGE_CURVE('',#7268,#7141,#1281,.T.);
#10038=EDGE_CURVE('',#7149,#7256,#1282,.F.);
#10039=EDGE_CURVE('',#7269,#7500,#1283,.F.);
#10040=EDGE_CURVE('',#7150,#7253,#1284,.T.);
#10041=EDGE_CURVE('',#7270,#7499,#1285,.F.);
#10042=EDGE_CURVE('',#7151,#7252,#1286,.T.);
#10043=EDGE_CURVE('',#7271,#7498,#1287,.T.);
#10044=EDGE_CURVE('',#7152,#7251,#1288,.T.);
#10045=EDGE_CURVE('',#7272,#7497,#1289,.F.);
#10046=EDGE_CURVE('',#7153,#7248,#1290,.T.);
#10047=EDGE_CURVE('',#7273,#7496,#1291,.F.);
#10048=EDGE_CURVE('',#7154,#7247,#1292,.F.);
#10049=EDGE_CURVE('',#7274,#7495,#1293,.F.);
#10050=EDGE_CURVE('',#7155,#7246,#1294,.T.);
#10051=EDGE_CURVE('',#7275,#7139,#1295,.F.);
#10052=EDGE_CURVE('',#7156,#7245,#1296,.F.);
#10053=EDGE_CURVE('',#7276,#7177,#1297,.F.);
#10054=EDGE_CURVE('',#7157,#7244,#1298,.F.);
#10055=EDGE_CURVE('',#6995,#7168,#1299,.F.);
#10056=EDGE_CURVE('',#7158,#7243,#1300,.F.);
#10057=EDGE_CURVE('',#6997,#7167,#1301,.T.);
#10058=EDGE_CURVE('',#7159,#7241,#1302,.F.);
#10059=EDGE_CURVE('',#6998,#7166,#1303,.F.);
#10060=EDGE_CURVE('',#7160,#7006,#1304,.T.);
#10061=EDGE_CURVE('',#6999,#7165,#1305,.T.);
#10062=EDGE_CURVE('',#7161,#7004,#1306,.T.);
#10063=EDGE_CURVE('',#7000,#7164,#1307,.F.);
#10064=EDGE_CURVE('',#7162,#7003,#1308,.F.);
#10065=EDGE_CURVE('',#7001,#7163,#1309,.F.);
#10066=EDGE_CURVE('',#6986,#7178,#1310,.F.);
#10067=EDGE_CURVE('',#7134,#6992,#1311,.T.);
#10068=EDGE_CURVE('',#7135,#6989,#1312,.T.);
#10069=EDGE_CURVE('',#6988,#7136,#1313,.F.);
#12417=ORIENTED_EDGE('',*,*,#9000,.F.);
#12418=ORIENTED_EDGE('',*,*,#9001,.T.);
#12419=ORIENTED_EDGE('',*,*,#9002,.T.);
#12420=ORIENTED_EDGE('',*,*,#9003,.T.);
#12421=ORIENTED_EDGE('',*,*,#9004,.T.);
#12422=ORIENTED_EDGE('',*,*,#9005,.T.);
#12423=ORIENTED_EDGE('',*,*,#9006,.T.);
#12424=ORIENTED_EDGE('',*,*,#9007,.F.);
#12425=ORIENTED_EDGE('',*,*,#9008,.T.);
#12426=ORIENTED_EDGE('',*,*,#9009,.T.);
#12427=ORIENTED_EDGE('',*,*,#9010,.T.);
#12428=ORIENTED_EDGE('',*,*,#9011,.T.);
#12429=ORIENTED_EDGE('',*,*,#9012,.T.);
#12430=ORIENTED_EDGE('',*,*,#9013,.T.);
#12431=ORIENTED_EDGE('',*,*,#9014,.T.);
#12432=ORIENTED_EDGE('',*,*,#9015,.T.);
#12433=ORIENTED_EDGE('',*,*,#9016,.T.);
#12434=ORIENTED_EDGE('',*,*,#9017,.T.);
#12435=ORIENTED_EDGE('',*,*,#9018,.T.);
#12436=ORIENTED_EDGE('',*,*,#9019,.T.);
#12437=ORIENTED_EDGE('',*,*,#9020,.T.);
#12438=ORIENTED_EDGE('',*,*,#9021,.F.);
#12439=ORIENTED_EDGE('',*,*,#9022,.T.);
#12440=ORIENTED_EDGE('',*,*,#9023,.T.);
#12441=ORIENTED_EDGE('',*,*,#9024,.T.);
#12442=ORIENTED_EDGE('',*,*,#9025,.T.);
#12443=ORIENTED_EDGE('',*,*,#9026,.T.);
#12444=ORIENTED_EDGE('',*,*,#9027,.T.);
#12445=ORIENTED_EDGE('',*,*,#9028,.T.);
#12446=ORIENTED_EDGE('',*,*,#9029,.T.);
#12447=ORIENTED_EDGE('',*,*,#9030,.T.);
#12448=ORIENTED_EDGE('',*,*,#9031,.T.);
#12449=ORIENTED_EDGE('',*,*,#9032,.T.);
#12450=ORIENTED_EDGE('',*,*,#9033,.T.);
#12451=ORIENTED_EDGE('',*,*,#9034,.T.);
#12452=ORIENTED_EDGE('',*,*,#9035,.T.);
#12453=ORIENTED_EDGE('',*,*,#9036,.T.);
#12454=ORIENTED_EDGE('',*,*,#9037,.T.);
#12455=ORIENTED_EDGE('',*,*,#9038,.T.);
#12456=ORIENTED_EDGE('',*,*,#9039,.T.);
#12457=ORIENTED_EDGE('',*,*,#9040,.T.);
#12458=ORIENTED_EDGE('',*,*,#9041,.T.);
#12459=ORIENTED_EDGE('',*,*,#9042,.T.);
#12460=ORIENTED_EDGE('',*,*,#9043,.T.);
#12461=ORIENTED_EDGE('',*,*,#9044,.T.);
#12462=ORIENTED_EDGE('',*,*,#9045,.T.);
#12463=ORIENTED_EDGE('',*,*,#9046,.T.);
#12464=ORIENTED_EDGE('',*,*,#9047,.T.);
#12465=ORIENTED_EDGE('',*,*,#9048,.T.);
#12466=ORIENTED_EDGE('',*,*,#9049,.T.);
#12467=ORIENTED_EDGE('',*,*,#9050,.T.);
#12468=ORIENTED_EDGE('',*,*,#9051,.T.);
#12469=ORIENTED_EDGE('',*,*,#9052,.T.);
#12470=ORIENTED_EDGE('',*,*,#9053,.T.);
#12471=ORIENTED_EDGE('',*,*,#9054,.T.);
#12472=ORIENTED_EDGE('',*,*,#9055,.T.);
#12473=ORIENTED_EDGE('',*,*,#9056,.T.);
#12474=ORIENTED_EDGE('',*,*,#9057,.T.);
#12475=ORIENTED_EDGE('',*,*,#9058,.T.);
#12476=ORIENTED_EDGE('',*,*,#9059,.T.);
#12477=ORIENTED_EDGE('',*,*,#9060,.T.);
#12478=ORIENTED_EDGE('',*,*,#9061,.T.);
#12479=ORIENTED_EDGE('',*,*,#9062,.T.);
#12480=ORIENTED_EDGE('',*,*,#9063,.T.);
#12481=ORIENTED_EDGE('',*,*,#9064,.T.);
#12482=ORIENTED_EDGE('',*,*,#9065,.T.);
#12483=ORIENTED_EDGE('',*,*,#9066,.T.);
#12484=ORIENTED_EDGE('',*,*,#9067,.T.);
#12485=ORIENTED_EDGE('',*,*,#9068,.T.);
#12486=ORIENTED_EDGE('',*,*,#9069,.T.);
#12487=ORIENTED_EDGE('',*,*,#9070,.T.);
#12488=ORIENTED_EDGE('',*,*,#9071,.T.);
#12489=ORIENTED_EDGE('',*,*,#9072,.T.);
#12490=ORIENTED_EDGE('',*,*,#9073,.T.);
#12491=ORIENTED_EDGE('',*,*,#9074,.T.);
#12492=ORIENTED_EDGE('',*,*,#9075,.T.);
#12493=ORIENTED_EDGE('',*,*,#9076,.T.);
#12494=ORIENTED_EDGE('',*,*,#9077,.T.);
#12495=ORIENTED_EDGE('',*,*,#9078,.T.);
#12496=ORIENTED_EDGE('',*,*,#9079,.T.);
#12497=ORIENTED_EDGE('',*,*,#9080,.T.);
#12498=ORIENTED_EDGE('',*,*,#9081,.T.);
#12499=ORIENTED_EDGE('',*,*,#9082,.T.);
#12500=ORIENTED_EDGE('',*,*,#9083,.T.);
#12501=ORIENTED_EDGE('',*,*,#9084,.T.);
#12502=ORIENTED_EDGE('',*,*,#9085,.T.);
#12503=ORIENTED_EDGE('',*,*,#9086,.T.);
#12504=ORIENTED_EDGE('',*,*,#9087,.T.);
#12505=ORIENTED_EDGE('',*,*,#9088,.T.);
#12506=ORIENTED_EDGE('',*,*,#9089,.T.);
#12507=ORIENTED_EDGE('',*,*,#9090,.T.);
#12508=ORIENTED_EDGE('',*,*,#9091,.T.);
#12509=ORIENTED_EDGE('',*,*,#9092,.T.);
#12510=ORIENTED_EDGE('',*,*,#9093,.T.);
#12511=ORIENTED_EDGE('',*,*,#9094,.T.);
#12512=ORIENTED_EDGE('',*,*,#9095,.T.);
#12513=ORIENTED_EDGE('',*,*,#9096,.T.);
#12514=ORIENTED_EDGE('',*,*,#9097,.T.);
#12515=ORIENTED_EDGE('',*,*,#9098,.T.);
#12516=ORIENTED_EDGE('',*,*,#9099,.T.);
#12517=ORIENTED_EDGE('',*,*,#9100,.T.);
#12518=ORIENTED_EDGE('',*,*,#9101,.T.);
#12519=ORIENTED_EDGE('',*,*,#9102,.T.);
#12520=ORIENTED_EDGE('',*,*,#9103,.T.);
#12521=ORIENTED_EDGE('',*,*,#9104,.T.);
#12522=ORIENTED_EDGE('',*,*,#9105,.T.);
#12523=ORIENTED_EDGE('',*,*,#9106,.T.);
#12524=ORIENTED_EDGE('',*,*,#9107,.T.);
#12525=ORIENTED_EDGE('',*,*,#9108,.T.);
#12526=ORIENTED_EDGE('',*,*,#9109,.T.);
#12527=ORIENTED_EDGE('',*,*,#9110,.T.);
#12528=ORIENTED_EDGE('',*,*,#9111,.T.);
#12529=ORIENTED_EDGE('',*,*,#9112,.T.);
#12530=ORIENTED_EDGE('',*,*,#9113,.T.);
#12531=ORIENTED_EDGE('',*,*,#9114,.T.);
#12532=ORIENTED_EDGE('',*,*,#9115,.T.);
#12533=ORIENTED_EDGE('',*,*,#9116,.T.);
#12534=ORIENTED_EDGE('',*,*,#9117,.T.);
#12535=ORIENTED_EDGE('',*,*,#9118,.T.);
#12536=ORIENTED_EDGE('',*,*,#9119,.T.);
#12537=ORIENTED_EDGE('',*,*,#9120,.T.);
#12538=ORIENTED_EDGE('',*,*,#9121,.T.);
#12539=ORIENTED_EDGE('',*,*,#9122,.T.);
#12540=ORIENTED_EDGE('',*,*,#9123,.T.);
#12541=ORIENTED_EDGE('',*,*,#9124,.T.);
#12542=ORIENTED_EDGE('',*,*,#9125,.T.);
#12543=ORIENTED_EDGE('',*,*,#9126,.T.);
#12544=ORIENTED_EDGE('',*,*,#9127,.T.);
#12545=ORIENTED_EDGE('',*,*,#9128,.T.);
#12546=ORIENTED_EDGE('',*,*,#9129,.T.);
#12547=ORIENTED_EDGE('',*,*,#9130,.T.);
#12548=ORIENTED_EDGE('',*,*,#9131,.T.);
#12549=ORIENTED_EDGE('',*,*,#9132,.T.);
#12550=ORIENTED_EDGE('',*,*,#9133,.T.);
#12551=ORIENTED_EDGE('',*,*,#9134,.T.);
#12552=ORIENTED_EDGE('',*,*,#9135,.T.);
#12553=ORIENTED_EDGE('',*,*,#9136,.T.);
#12554=ORIENTED_EDGE('',*,*,#9137,.T.);
#12555=ORIENTED_EDGE('',*,*,#9138,.T.);
#12556=ORIENTED_EDGE('',*,*,#9139,.T.);
#12557=ORIENTED_EDGE('',*,*,#9140,.T.);
#12558=ORIENTED_EDGE('',*,*,#9141,.T.);
#12559=ORIENTED_EDGE('',*,*,#9142,.T.);
#12560=ORIENTED_EDGE('',*,*,#9143,.T.);
#12561=ORIENTED_EDGE('',*,*,#9144,.T.);
#12562=ORIENTED_EDGE('',*,*,#9145,.T.);
#12563=ORIENTED_EDGE('',*,*,#9146,.T.);
#12564=ORIENTED_EDGE('',*,*,#9147,.T.);
#12565=ORIENTED_EDGE('',*,*,#9148,.T.);
#12566=ORIENTED_EDGE('',*,*,#9149,.T.);
#12567=ORIENTED_EDGE('',*,*,#9150,.T.);
#12568=ORIENTED_EDGE('',*,*,#9151,.T.);
#12569=ORIENTED_EDGE('',*,*,#9152,.T.);
#12570=ORIENTED_EDGE('',*,*,#9153,.T.);
#12571=ORIENTED_EDGE('',*,*,#9154,.T.);
#12572=ORIENTED_EDGE('',*,*,#9155,.T.);
#12573=ORIENTED_EDGE('',*,*,#9156,.T.);
#12574=ORIENTED_EDGE('',*,*,#9157,.T.);
#12575=ORIENTED_EDGE('',*,*,#9158,.T.);
#12576=ORIENTED_EDGE('',*,*,#9159,.T.);
#12577=ORIENTED_EDGE('',*,*,#9160,.F.);
#12578=ORIENTED_EDGE('',*,*,#9161,.F.);
#12579=ORIENTED_EDGE('',*,*,#9162,.T.);
#12580=ORIENTED_EDGE('',*,*,#9163,.T.);
#12581=ORIENTED_EDGE('',*,*,#9164,.F.);
#12582=ORIENTED_EDGE('',*,*,#9165,.T.);
#12583=ORIENTED_EDGE('',*,*,#9166,.F.);
#12584=ORIENTED_EDGE('',*,*,#9167,.T.);
#12585=ORIENTED_EDGE('',*,*,#9168,.T.);
#12586=ORIENTED_EDGE('',*,*,#9169,.T.);
#12587=ORIENTED_EDGE('',*,*,#9170,.T.);
#12588=ORIENTED_EDGE('',*,*,#9171,.F.);
#12589=ORIENTED_EDGE('',*,*,#9172,.F.);
#12590=ORIENTED_EDGE('',*,*,#9173,.T.);
#12591=ORIENTED_EDGE('',*,*,#9174,.T.);
#12592=ORIENTED_EDGE('',*,*,#9175,.T.);
#12593=ORIENTED_EDGE('',*,*,#9176,.F.);
#12594=ORIENTED_EDGE('',*,*,#9177,.F.);
#12595=ORIENTED_EDGE('',*,*,#9178,.T.);
#12596=ORIENTED_EDGE('',*,*,#9179,.T.);
#12597=ORIENTED_EDGE('',*,*,#9180,.F.);
#12598=ORIENTED_EDGE('',*,*,#9181,.F.);
#12599=ORIENTED_EDGE('',*,*,#9182,.F.);
#12600=ORIENTED_EDGE('',*,*,#9183,.F.);
#12601=ORIENTED_EDGE('',*,*,#9184,.F.);
#12602=ORIENTED_EDGE('',*,*,#9185,.F.);
#12603=ORIENTED_EDGE('',*,*,#9186,.F.);
#12604=ORIENTED_EDGE('',*,*,#9187,.F.);
#12605=ORIENTED_EDGE('',*,*,#9188,.F.);
#12606=ORIENTED_EDGE('',*,*,#9189,.T.);
#12607=ORIENTED_EDGE('',*,*,#9190,.T.);
#12608=ORIENTED_EDGE('',*,*,#9191,.F.);
#12609=ORIENTED_EDGE('',*,*,#9192,.F.);
#12610=ORIENTED_EDGE('',*,*,#9193,.F.);
#12611=ORIENTED_EDGE('',*,*,#9194,.T.);
#12612=ORIENTED_EDGE('',*,*,#9195,.T.);
#12613=ORIENTED_EDGE('',*,*,#9196,.F.);
#12614=ORIENTED_EDGE('',*,*,#9197,.T.);
#12615=ORIENTED_EDGE('',*,*,#9198,.F.);
#12616=ORIENTED_EDGE('',*,*,#9199,.F.);
#12617=ORIENTED_EDGE('',*,*,#9200,.F.);
#12618=ORIENTED_EDGE('',*,*,#9201,.T.);
#12619=ORIENTED_EDGE('',*,*,#9202,.T.);
#12620=ORIENTED_EDGE('',*,*,#9203,.F.);
#12621=ORIENTED_EDGE('',*,*,#9204,.T.);
#12622=ORIENTED_EDGE('',*,*,#9160,.T.);
#12623=ORIENTED_EDGE('',*,*,#9205,.F.);
#12624=ORIENTED_EDGE('',*,*,#9206,.F.);
#12625=ORIENTED_EDGE('',*,*,#9165,.F.);
#12626=ORIENTED_EDGE('',*,*,#9207,.F.);
#12627=ORIENTED_EDGE('',*,*,#9208,.F.);
#12628=ORIENTED_EDGE('',*,*,#9209,.F.);
#12629=ORIENTED_EDGE('',*,*,#9210,.F.);
#12630=ORIENTED_EDGE('',*,*,#9211,.F.);
#12631=ORIENTED_EDGE('',*,*,#9212,.F.);
#12632=ORIENTED_EDGE('',*,*,#9021,.T.);
#12633=ORIENTED_EDGE('',*,*,#9213,.T.);
#12634=ORIENTED_EDGE('',*,*,#9214,.T.);
#12635=ORIENTED_EDGE('',*,*,#9215,.T.);
#12636=ORIENTED_EDGE('',*,*,#9216,.T.);
#12637=ORIENTED_EDGE('',*,*,#9217,.T.);
#12638=ORIENTED_EDGE('',*,*,#9218,.T.);
#12639=ORIENTED_EDGE('',*,*,#9219,.T.);
#12640=ORIENTED_EDGE('',*,*,#9220,.T.);
#12641=ORIENTED_EDGE('',*,*,#9221,.T.);
#12642=ORIENTED_EDGE('',*,*,#9222,.T.);
#12643=ORIENTED_EDGE('',*,*,#9223,.T.);
#12644=ORIENTED_EDGE('',*,*,#9224,.T.);
#12645=ORIENTED_EDGE('',*,*,#9151,.F.);
#12646=ORIENTED_EDGE('',*,*,#9225,.T.);
#12647=ORIENTED_EDGE('',*,*,#9226,.T.);
#12648=ORIENTED_EDGE('',*,*,#9227,.T.);
#12649=ORIENTED_EDGE('',*,*,#9228,.T.);
#12650=ORIENTED_EDGE('',*,*,#9229,.T.);
#12651=ORIENTED_EDGE('',*,*,#9230,.T.);
#12652=ORIENTED_EDGE('',*,*,#9143,.F.);
#12653=ORIENTED_EDGE('',*,*,#9231,.T.);
#12654=ORIENTED_EDGE('',*,*,#9232,.T.);
#12655=ORIENTED_EDGE('',*,*,#9233,.T.);
#12656=ORIENTED_EDGE('',*,*,#9137,.F.);
#12657=ORIENTED_EDGE('',*,*,#9234,.T.);
#12658=ORIENTED_EDGE('',*,*,#9235,.T.);
#12659=ORIENTED_EDGE('',*,*,#9236,.T.);
#12660=ORIENTED_EDGE('',*,*,#9131,.F.);
#12661=ORIENTED_EDGE('',*,*,#9237,.T.);
#12662=ORIENTED_EDGE('',*,*,#9238,.T.);
#12663=ORIENTED_EDGE('',*,*,#9239,.T.);
#12664=ORIENTED_EDGE('',*,*,#9125,.F.);
#12665=ORIENTED_EDGE('',*,*,#9240,.T.);
#12666=ORIENTED_EDGE('',*,*,#9241,.T.);
#12667=ORIENTED_EDGE('',*,*,#9242,.T.);
#12668=ORIENTED_EDGE('',*,*,#9119,.F.);
#12669=ORIENTED_EDGE('',*,*,#9243,.T.);
#12670=ORIENTED_EDGE('',*,*,#9244,.T.);
#12671=ORIENTED_EDGE('',*,*,#9245,.T.);
#12672=ORIENTED_EDGE('',*,*,#9113,.F.);
#12673=ORIENTED_EDGE('',*,*,#9246,.T.);
#12674=ORIENTED_EDGE('',*,*,#9247,.T.);
#12675=ORIENTED_EDGE('',*,*,#9248,.T.);
#12676=ORIENTED_EDGE('',*,*,#9107,.F.);
#12677=ORIENTED_EDGE('',*,*,#9249,.T.);
#12678=ORIENTED_EDGE('',*,*,#9250,.T.);
#12679=ORIENTED_EDGE('',*,*,#9251,.T.);
#12680=ORIENTED_EDGE('',*,*,#9101,.F.);
#12681=ORIENTED_EDGE('',*,*,#9252,.T.);
#12682=ORIENTED_EDGE('',*,*,#9253,.T.);
#12683=ORIENTED_EDGE('',*,*,#9254,.T.);
#12684=ORIENTED_EDGE('',*,*,#9095,.F.);
#12685=ORIENTED_EDGE('',*,*,#9255,.T.);
#12686=ORIENTED_EDGE('',*,*,#9256,.T.);
#12687=ORIENTED_EDGE('',*,*,#9257,.T.);
#12688=ORIENTED_EDGE('',*,*,#9089,.F.);
#12689=ORIENTED_EDGE('',*,*,#9258,.T.);
#12690=ORIENTED_EDGE('',*,*,#9259,.T.);
#12691=ORIENTED_EDGE('',*,*,#9260,.T.);
#12692=ORIENTED_EDGE('',*,*,#9083,.F.);
#12693=ORIENTED_EDGE('',*,*,#9261,.T.);
#12694=ORIENTED_EDGE('',*,*,#9262,.T.);
#12695=ORIENTED_EDGE('',*,*,#9263,.T.);
#12696=ORIENTED_EDGE('',*,*,#9077,.F.);
#12697=ORIENTED_EDGE('',*,*,#9264,.T.);
#12698=ORIENTED_EDGE('',*,*,#9265,.T.);
#12699=ORIENTED_EDGE('',*,*,#9266,.T.);
#12700=ORIENTED_EDGE('',*,*,#9267,.T.);
#12701=ORIENTED_EDGE('',*,*,#9070,.F.);
#12702=ORIENTED_EDGE('',*,*,#9268,.T.);
#12703=ORIENTED_EDGE('',*,*,#9269,.T.);
#12704=ORIENTED_EDGE('',*,*,#9270,.T.);
#12705=ORIENTED_EDGE('',*,*,#9271,.T.);
#12706=ORIENTED_EDGE('',*,*,#9272,.T.);
#12707=ORIENTED_EDGE('',*,*,#9059,.F.);
#12708=ORIENTED_EDGE('',*,*,#9273,.T.);
#12709=ORIENTED_EDGE('',*,*,#9274,.T.);
#12710=ORIENTED_EDGE('',*,*,#9275,.T.);
#12711=ORIENTED_EDGE('',*,*,#9276,.T.);
#12712=ORIENTED_EDGE('',*,*,#9277,.T.);
#12713=ORIENTED_EDGE('',*,*,#9051,.F.);
#12714=ORIENTED_EDGE('',*,*,#9278,.T.);
#12715=ORIENTED_EDGE('',*,*,#9279,.T.);
#12716=ORIENTED_EDGE('',*,*,#9280,.T.);
#12717=ORIENTED_EDGE('',*,*,#9281,.T.);
#12718=ORIENTED_EDGE('',*,*,#9282,.T.);
#12719=ORIENTED_EDGE('',*,*,#9043,.F.);
#12720=ORIENTED_EDGE('',*,*,#9283,.T.);
#12721=ORIENTED_EDGE('',*,*,#9284,.T.);
#12722=ORIENTED_EDGE('',*,*,#9285,.T.);
#12723=ORIENTED_EDGE('',*,*,#9286,.T.);
#12724=ORIENTED_EDGE('',*,*,#9287,.T.);
#12725=ORIENTED_EDGE('',*,*,#9035,.F.);
#12726=ORIENTED_EDGE('',*,*,#9288,.T.);
#12727=ORIENTED_EDGE('',*,*,#9289,.T.);
#12728=ORIENTED_EDGE('',*,*,#9290,.T.);
#12729=ORIENTED_EDGE('',*,*,#9291,.T.);
#12730=ORIENTED_EDGE('',*,*,#9292,.T.);
#12731=ORIENTED_EDGE('',*,*,#9293,.T.);
#12732=ORIENTED_EDGE('',*,*,#9294,.T.);
#12733=ORIENTED_EDGE('',*,*,#9295,.T.);
#12734=ORIENTED_EDGE('',*,*,#9296,.T.);
#12735=ORIENTED_EDGE('',*,*,#9297,.T.);
#12736=ORIENTED_EDGE('',*,*,#9298,.T.);
#12737=ORIENTED_EDGE('',*,*,#9299,.T.);
#12738=ORIENTED_EDGE('',*,*,#9300,.T.);
#12739=ORIENTED_EDGE('',*,*,#9301,.T.);
#12740=ORIENTED_EDGE('',*,*,#9302,.T.);
#12741=ORIENTED_EDGE('',*,*,#9303,.T.);
#12742=ORIENTED_EDGE('',*,*,#9304,.T.);
#12743=ORIENTED_EDGE('',*,*,#9305,.T.);
#12744=ORIENTED_EDGE('',*,*,#9306,.T.);
#12745=ORIENTED_EDGE('',*,*,#9307,.T.);
#12746=ORIENTED_EDGE('',*,*,#9308,.T.);
#12747=ORIENTED_EDGE('',*,*,#9309,.T.);
#12748=ORIENTED_EDGE('',*,*,#9310,.T.);
#12749=ORIENTED_EDGE('',*,*,#9311,.T.);
#12750=ORIENTED_EDGE('',*,*,#9312,.T.);
#12751=ORIENTED_EDGE('',*,*,#9313,.T.);
#12752=ORIENTED_EDGE('',*,*,#9314,.T.);
#12753=ORIENTED_EDGE('',*,*,#9315,.T.);
#12754=ORIENTED_EDGE('',*,*,#9316,.T.);
#12755=ORIENTED_EDGE('',*,*,#9317,.T.);
#12756=ORIENTED_EDGE('',*,*,#9318,.T.);
#12757=ORIENTED_EDGE('',*,*,#9319,.T.);
#12758=ORIENTED_EDGE('',*,*,#9320,.T.);
#12759=ORIENTED_EDGE('',*,*,#9321,.T.);
#12760=ORIENTED_EDGE('',*,*,#9322,.T.);
#12761=ORIENTED_EDGE('',*,*,#9323,.T.);
#12762=ORIENTED_EDGE('',*,*,#9324,.T.);
#12763=ORIENTED_EDGE('',*,*,#9325,.T.);
#12764=ORIENTED_EDGE('',*,*,#9326,.T.);
#12765=ORIENTED_EDGE('',*,*,#9327,.T.);
#12766=ORIENTED_EDGE('',*,*,#9328,.T.);
#12767=ORIENTED_EDGE('',*,*,#9329,.T.);
#12768=ORIENTED_EDGE('',*,*,#9330,.T.);
#12769=ORIENTED_EDGE('',*,*,#9331,.T.);
#12770=ORIENTED_EDGE('',*,*,#9332,.T.);
#12771=ORIENTED_EDGE('',*,*,#9333,.T.);
#12772=ORIENTED_EDGE('',*,*,#9334,.T.);
#12773=ORIENTED_EDGE('',*,*,#9335,.T.);
#12774=ORIENTED_EDGE('',*,*,#9336,.T.);
#12775=ORIENTED_EDGE('',*,*,#9337,.T.);
#12776=ORIENTED_EDGE('',*,*,#9338,.T.);
#12777=ORIENTED_EDGE('',*,*,#9339,.T.);
#12778=ORIENTED_EDGE('',*,*,#9340,.T.);
#12779=ORIENTED_EDGE('',*,*,#9341,.T.);
#12780=ORIENTED_EDGE('',*,*,#9342,.T.);
#12781=ORIENTED_EDGE('',*,*,#9343,.T.);
#12782=ORIENTED_EDGE('',*,*,#9344,.T.);
#12783=ORIENTED_EDGE('',*,*,#9345,.T.);
#12784=ORIENTED_EDGE('',*,*,#9346,.T.);
#12785=ORIENTED_EDGE('',*,*,#9347,.T.);
#12786=ORIENTED_EDGE('',*,*,#9348,.T.);
#12787=ORIENTED_EDGE('',*,*,#9349,.T.);
#12788=ORIENTED_EDGE('',*,*,#9350,.T.);
#12789=ORIENTED_EDGE('',*,*,#9351,.T.);
#12790=ORIENTED_EDGE('',*,*,#9352,.T.);
#12791=ORIENTED_EDGE('',*,*,#9353,.T.);
#12792=ORIENTED_EDGE('',*,*,#9354,.T.);
#12793=ORIENTED_EDGE('',*,*,#9355,.T.);
#12794=ORIENTED_EDGE('',*,*,#9356,.T.);
#12795=ORIENTED_EDGE('',*,*,#9357,.T.);
#12796=ORIENTED_EDGE('',*,*,#9358,.T.);
#12797=ORIENTED_EDGE('',*,*,#9359,.T.);
#12798=ORIENTED_EDGE('',*,*,#9360,.T.);
#12799=ORIENTED_EDGE('',*,*,#9361,.T.);
#12800=ORIENTED_EDGE('',*,*,#9362,.T.);
#12801=ORIENTED_EDGE('',*,*,#9363,.T.);
#12802=ORIENTED_EDGE('',*,*,#9364,.T.);
#12803=ORIENTED_EDGE('',*,*,#9365,.T.);
#12804=ORIENTED_EDGE('',*,*,#9366,.T.);
#12805=ORIENTED_EDGE('',*,*,#9367,.T.);
#12806=ORIENTED_EDGE('',*,*,#9368,.T.);
#12807=ORIENTED_EDGE('',*,*,#9369,.T.);
#12808=ORIENTED_EDGE('',*,*,#9370,.T.);
#12809=ORIENTED_EDGE('',*,*,#9371,.T.);
#12810=ORIENTED_EDGE('',*,*,#9372,.T.);
#12811=ORIENTED_EDGE('',*,*,#9373,.T.);
#12812=ORIENTED_EDGE('',*,*,#9374,.T.);
#12813=ORIENTED_EDGE('',*,*,#9375,.T.);
#12814=ORIENTED_EDGE('',*,*,#9376,.T.);
#12815=ORIENTED_EDGE('',*,*,#9377,.T.);
#12816=ORIENTED_EDGE('',*,*,#9378,.T.);
#12817=ORIENTED_EDGE('',*,*,#9379,.T.);
#12818=ORIENTED_EDGE('',*,*,#9380,.T.);
#12819=ORIENTED_EDGE('',*,*,#9381,.T.);
#12820=ORIENTED_EDGE('',*,*,#9382,.T.);
#12821=ORIENTED_EDGE('',*,*,#9383,.T.);
#12822=ORIENTED_EDGE('',*,*,#9384,.T.);
#12823=ORIENTED_EDGE('',*,*,#9385,.T.);
#12824=ORIENTED_EDGE('',*,*,#9386,.T.);
#12825=ORIENTED_EDGE('',*,*,#9387,.T.);
#12826=ORIENTED_EDGE('',*,*,#9388,.T.);
#12827=ORIENTED_EDGE('',*,*,#9389,.T.);
#12828=ORIENTED_EDGE('',*,*,#9390,.T.);
#12829=ORIENTED_EDGE('',*,*,#9391,.T.);
#12830=ORIENTED_EDGE('',*,*,#9392,.T.);
#12831=ORIENTED_EDGE('',*,*,#9393,.T.);
#12832=ORIENTED_EDGE('',*,*,#9394,.T.);
#12833=ORIENTED_EDGE('',*,*,#9395,.T.);
#12834=ORIENTED_EDGE('',*,*,#9396,.T.);
#12835=ORIENTED_EDGE('',*,*,#9397,.T.);
#12836=ORIENTED_EDGE('',*,*,#9398,.T.);
#12837=ORIENTED_EDGE('',*,*,#9399,.T.);
#12838=ORIENTED_EDGE('',*,*,#9400,.T.);
#12839=ORIENTED_EDGE('',*,*,#9401,.T.);
#12840=ORIENTED_EDGE('',*,*,#9402,.T.);
#12841=ORIENTED_EDGE('',*,*,#9403,.T.);
#12842=ORIENTED_EDGE('',*,*,#9404,.T.);
#12843=ORIENTED_EDGE('',*,*,#9405,.T.);
#12844=ORIENTED_EDGE('',*,*,#9406,.T.);
#12845=ORIENTED_EDGE('',*,*,#9407,.T.);
#12846=ORIENTED_EDGE('',*,*,#9408,.T.);
#12847=ORIENTED_EDGE('',*,*,#9409,.T.);
#12848=ORIENTED_EDGE('',*,*,#9410,.T.);
#12849=ORIENTED_EDGE('',*,*,#9411,.T.);
#12850=ORIENTED_EDGE('',*,*,#9412,.T.);
#12851=ORIENTED_EDGE('',*,*,#9413,.T.);
#12852=ORIENTED_EDGE('',*,*,#9414,.T.);
#12853=ORIENTED_EDGE('',*,*,#9415,.T.);
#12854=ORIENTED_EDGE('',*,*,#9416,.T.);
#12855=ORIENTED_EDGE('',*,*,#9417,.T.);
#12856=ORIENTED_EDGE('',*,*,#9418,.T.);
#12857=ORIENTED_EDGE('',*,*,#9419,.T.);
#12858=ORIENTED_EDGE('',*,*,#9420,.T.);
#12859=ORIENTED_EDGE('',*,*,#9421,.T.);
#12860=ORIENTED_EDGE('',*,*,#9422,.T.);
#12861=ORIENTED_EDGE('',*,*,#9423,.T.);
#12862=ORIENTED_EDGE('',*,*,#9424,.T.);
#12863=ORIENTED_EDGE('',*,*,#9425,.T.);
#12864=ORIENTED_EDGE('',*,*,#9426,.T.);
#12865=ORIENTED_EDGE('',*,*,#9427,.T.);
#12866=ORIENTED_EDGE('',*,*,#9428,.T.);
#12867=ORIENTED_EDGE('',*,*,#9429,.T.);
#12868=ORIENTED_EDGE('',*,*,#9430,.T.);
#12869=ORIENTED_EDGE('',*,*,#9431,.T.);
#12870=ORIENTED_EDGE('',*,*,#9432,.T.);
#12871=ORIENTED_EDGE('',*,*,#9433,.T.);
#12872=ORIENTED_EDGE('',*,*,#9434,.T.);
#12873=ORIENTED_EDGE('',*,*,#9435,.T.);
#12874=ORIENTED_EDGE('',*,*,#9436,.T.);
#12875=ORIENTED_EDGE('',*,*,#9437,.T.);
#12876=ORIENTED_EDGE('',*,*,#9438,.T.);
#12877=ORIENTED_EDGE('',*,*,#9439,.T.);
#12878=ORIENTED_EDGE('',*,*,#9440,.T.);
#12879=ORIENTED_EDGE('',*,*,#9441,.T.);
#12880=ORIENTED_EDGE('',*,*,#9442,.T.);
#12881=ORIENTED_EDGE('',*,*,#9443,.T.);
#12882=ORIENTED_EDGE('',*,*,#9444,.T.);
#12883=ORIENTED_EDGE('',*,*,#9445,.T.);
#12884=ORIENTED_EDGE('',*,*,#9446,.T.);
#12885=ORIENTED_EDGE('',*,*,#9447,.T.);
#12886=ORIENTED_EDGE('',*,*,#9448,.T.);
#12887=ORIENTED_EDGE('',*,*,#9449,.T.);
#12888=ORIENTED_EDGE('',*,*,#9450,.T.);
#12889=ORIENTED_EDGE('',*,*,#9451,.T.);
#12890=ORIENTED_EDGE('',*,*,#9452,.T.);
#12891=ORIENTED_EDGE('',*,*,#9007,.T.);
#12892=ORIENTED_EDGE('',*,*,#9453,.T.);
#12893=ORIENTED_EDGE('',*,*,#9013,.F.);
#12894=ORIENTED_EDGE('',*,*,#9454,.T.);
#12895=ORIENTED_EDGE('',*,*,#9455,.F.);
#12896=ORIENTED_EDGE('',*,*,#9200,.T.);
#12897=ORIENTED_EDGE('',*,*,#9456,.F.);
#12898=ORIENTED_EDGE('',*,*,#9210,.T.);
#12899=ORIENTED_EDGE('',*,*,#9203,.T.);
#12900=ORIENTED_EDGE('',*,*,#9457,.T.);
#12901=ORIENTED_EDGE('',*,*,#9458,.T.);
#12902=ORIENTED_EDGE('',*,*,#9459,.F.);
#12903=ORIENTED_EDGE('',*,*,#9204,.F.);
#12904=ORIENTED_EDGE('',*,*,#9459,.T.);
#12905=ORIENTED_EDGE('',*,*,#9460,.T.);
#12906=ORIENTED_EDGE('',*,*,#9461,.F.);
#12907=ORIENTED_EDGE('',*,*,#9462,.T.);
#12908=ORIENTED_EDGE('',*,*,#9463,.T.);
#12909=ORIENTED_EDGE('',*,*,#9464,.T.);
#12910=ORIENTED_EDGE('',*,*,#9465,.T.);
#12911=ORIENTED_EDGE('',*,*,#9466,.T.);
#12912=ORIENTED_EDGE('',*,*,#9467,.T.);
#12913=ORIENTED_EDGE('',*,*,#9468,.T.);
#12914=ORIENTED_EDGE('',*,*,#9469,.T.);
#12915=ORIENTED_EDGE('',*,*,#9470,.T.);
#12916=ORIENTED_EDGE('',*,*,#9471,.T.);
#12917=ORIENTED_EDGE('',*,*,#9472,.F.);
#12918=ORIENTED_EDGE('',*,*,#9473,.T.);
#12919=ORIENTED_EDGE('',*,*,#9474,.T.);
#12920=ORIENTED_EDGE('',*,*,#9475,.T.);
#12921=ORIENTED_EDGE('',*,*,#9476,.T.);
#12922=ORIENTED_EDGE('',*,*,#9477,.T.);
#12923=ORIENTED_EDGE('',*,*,#9478,.T.);
#12924=ORIENTED_EDGE('',*,*,#9479,.T.);
#12925=ORIENTED_EDGE('',*,*,#9480,.T.);
#12926=ORIENTED_EDGE('',*,*,#9481,.F.);
#12927=ORIENTED_EDGE('',*,*,#9482,.F.);
#12928=ORIENTED_EDGE('',*,*,#9483,.F.);
#12929=ORIENTED_EDGE('',*,*,#9460,.F.);
#12930=ORIENTED_EDGE('',*,*,#9458,.F.);
#12931=ORIENTED_EDGE('',*,*,#9000,.T.);
#12932=ORIENTED_EDGE('',*,*,#9484,.T.);
#12933=ORIENTED_EDGE('',*,*,#9485,.T.);
#12934=ORIENTED_EDGE('',*,*,#9486,.T.);
#12935=ORIENTED_EDGE('',*,*,#9487,.T.);
#12936=ORIENTED_EDGE('',*,*,#9488,.T.);
#12937=ORIENTED_EDGE('',*,*,#9004,.F.);
#12938=ORIENTED_EDGE('',*,*,#9489,.T.);
#12939=ORIENTED_EDGE('',*,*,#9490,.T.);
#12940=ORIENTED_EDGE('',*,*,#9491,.T.);
#12941=ORIENTED_EDGE('',*,*,#9492,.T.);
#12942=ORIENTED_EDGE('',*,*,#9493,.T.);
#12943=ORIENTED_EDGE('',*,*,#9494,.T.);
#12944=ORIENTED_EDGE('',*,*,#9495,.T.);
#12945=ORIENTED_EDGE('',*,*,#9496,.T.);
#12946=ORIENTED_EDGE('',*,*,#9497,.T.);
#12947=ORIENTED_EDGE('',*,*,#9498,.T.);
#12948=ORIENTED_EDGE('',*,*,#9499,.T.);
#12949=ORIENTED_EDGE('',*,*,#9500,.T.);
#12950=ORIENTED_EDGE('',*,*,#9501,.T.);
#12951=ORIENTED_EDGE('',*,*,#9502,.T.);
#12952=ORIENTED_EDGE('',*,*,#9503,.T.);
#12953=ORIENTED_EDGE('',*,*,#9504,.T.);
#12954=ORIENTED_EDGE('',*,*,#9505,.T.);
#12955=ORIENTED_EDGE('',*,*,#9466,.F.);
#12956=ORIENTED_EDGE('',*,*,#9506,.T.);
#12957=ORIENTED_EDGE('',*,*,#9507,.T.);
#12958=ORIENTED_EDGE('',*,*,#9472,.T.);
#12959=ORIENTED_EDGE('',*,*,#9508,.T.);
#12960=ORIENTED_EDGE('',*,*,#9509,.T.);
#12961=ORIENTED_EDGE('',*,*,#9481,.T.);
#12962=ORIENTED_EDGE('',*,*,#9510,.T.);
#12963=ORIENTED_EDGE('',*,*,#9511,.T.);
#12964=ORIENTED_EDGE('',*,*,#9467,.F.);
#12965=ORIENTED_EDGE('',*,*,#9512,.T.);
#12966=ORIENTED_EDGE('',*,*,#9513,.T.);
#12967=ORIENTED_EDGE('',*,*,#9514,.T.);
#12968=ORIENTED_EDGE('',*,*,#9515,.T.);
#12969=ORIENTED_EDGE('',*,*,#9516,.T.);
#12970=ORIENTED_EDGE('',*,*,#9517,.T.);
#12971=ORIENTED_EDGE('',*,*,#9518,.T.);
#12972=ORIENTED_EDGE('',*,*,#9519,.T.);
#12973=ORIENTED_EDGE('',*,*,#9520,.T.);
#12974=ORIENTED_EDGE('',*,*,#9521,.T.);
#12975=ORIENTED_EDGE('',*,*,#9522,.T.);
#12976=ORIENTED_EDGE('',*,*,#9523,.T.);
#12977=ORIENTED_EDGE('',*,*,#9524,.T.);
#12978=ORIENTED_EDGE('',*,*,#9525,.T.);
#12979=ORIENTED_EDGE('',*,*,#9526,.T.);
#12980=ORIENTED_EDGE('',*,*,#9527,.T.);
#12981=ORIENTED_EDGE('',*,*,#9526,.F.);
#12982=ORIENTED_EDGE('',*,*,#9528,.T.);
#12983=ORIENTED_EDGE('',*,*,#9529,.T.);
#12984=ORIENTED_EDGE('',*,*,#9530,.T.);
#12985=ORIENTED_EDGE('',*,*,#9531,.T.);
#12986=ORIENTED_EDGE('',*,*,#9532,.T.);
#12987=ORIENTED_EDGE('',*,*,#9533,.T.);
#12988=ORIENTED_EDGE('',*,*,#9534,.T.);
#12989=ORIENTED_EDGE('',*,*,#9535,.T.);
#12990=ORIENTED_EDGE('',*,*,#9536,.T.);
#12991=ORIENTED_EDGE('',*,*,#9537,.T.);
#12992=ORIENTED_EDGE('',*,*,#9538,.T.);
#12993=ORIENTED_EDGE('',*,*,#9539,.T.);
#12994=ORIENTED_EDGE('',*,*,#9540,.T.);
#12995=ORIENTED_EDGE('',*,*,#9541,.T.);
#12996=ORIENTED_EDGE('',*,*,#9542,.T.);
#12997=ORIENTED_EDGE('',*,*,#9543,.T.);
#12998=ORIENTED_EDGE('',*,*,#9544,.T.);
#12999=ORIENTED_EDGE('',*,*,#9521,.F.);
#13000=ORIENTED_EDGE('',*,*,#9545,.T.);
#13001=ORIENTED_EDGE('',*,*,#9546,.T.);
#13002=ORIENTED_EDGE('',*,*,#9547,.T.);
#13003=ORIENTED_EDGE('',*,*,#9548,.T.);
#13004=ORIENTED_EDGE('',*,*,#9549,.T.);
#13005=ORIENTED_EDGE('',*,*,#9533,.F.);
#13006=ORIENTED_EDGE('',*,*,#9550,.T.);
#13007=ORIENTED_EDGE('',*,*,#9551,.T.);
#13008=ORIENTED_EDGE('',*,*,#9552,.T.);
#13009=ORIENTED_EDGE('',*,*,#9553,.T.);
#13010=ORIENTED_EDGE('',*,*,#9539,.F.);
#13011=ORIENTED_EDGE('',*,*,#9554,.T.);
#13012=ORIENTED_EDGE('',*,*,#9555,.T.);
#13013=ORIENTED_EDGE('',*,*,#9556,.T.);
#13014=ORIENTED_EDGE('',*,*,#9557,.T.);
#13015=ORIENTED_EDGE('',*,*,#9515,.F.);
#13016=ORIENTED_EDGE('',*,*,#9558,.T.);
#13017=ORIENTED_EDGE('',*,*,#9559,.T.);
#13018=ORIENTED_EDGE('',*,*,#9560,.T.);
#13019=ORIENTED_EDGE('',*,*,#9519,.F.);
#13020=ORIENTED_EDGE('',*,*,#9561,.T.);
#13021=ORIENTED_EDGE('',*,*,#9562,.T.);
#13022=ORIENTED_EDGE('',*,*,#9504,.F.);
#13023=ORIENTED_EDGE('',*,*,#9563,.T.);
#13024=ORIENTED_EDGE('',*,*,#9564,.T.);
#13025=ORIENTED_EDGE('',*,*,#9565,.T.);
#13026=ORIENTED_EDGE('',*,*,#9566,.T.);
#13027=ORIENTED_EDGE('',*,*,#9500,.F.);
#13028=ORIENTED_EDGE('',*,*,#9567,.F.);
#13029=ORIENTED_EDGE('',*,*,#9509,.F.);
#13030=ORIENTED_EDGE('',*,*,#9508,.F.);
#13031=ORIENTED_EDGE('',*,*,#9568,.F.);
#13032=ORIENTED_EDGE('',*,*,#9492,.F.);
#13033=ORIENTED_EDGE('',*,*,#9568,.T.);
#13034=ORIENTED_EDGE('',*,*,#9476,.F.);
#13035=ORIENTED_EDGE('',*,*,#9569,.F.);
#13036=ORIENTED_EDGE('',*,*,#9493,.F.);
#13037=ORIENTED_EDGE('',*,*,#9491,.F.);
#13038=ORIENTED_EDGE('',*,*,#9570,.T.);
#13039=ORIENTED_EDGE('',*,*,#9462,.F.);
#13040=ORIENTED_EDGE('',*,*,#9567,.T.);
#13041=ORIENTED_EDGE('',*,*,#9475,.F.);
#13042=ORIENTED_EDGE('',*,*,#9571,.T.);
#13043=ORIENTED_EDGE('',*,*,#9558,.F.);
#13044=ORIENTED_EDGE('',*,*,#9518,.F.);
#13045=ORIENTED_EDGE('',*,*,#9572,.F.);
#13046=ORIENTED_EDGE('',*,*,#9494,.F.);
#13047=ORIENTED_EDGE('',*,*,#9569,.T.);
#13048=ORIENTED_EDGE('',*,*,#9566,.F.);
#13049=ORIENTED_EDGE('',*,*,#9573,.T.);
#13050=ORIENTED_EDGE('',*,*,#9490,.F.);
#13051=ORIENTED_EDGE('',*,*,#9574,.F.);
#13052=ORIENTED_EDGE('',*,*,#9501,.F.);
#13053=ORIENTED_EDGE('',*,*,#9572,.T.);
#13054=ORIENTED_EDGE('',*,*,#9517,.F.);
#13055=ORIENTED_EDGE('',*,*,#9575,.F.);
#13056=ORIENTED_EDGE('',*,*,#9495,.F.);
#13057=ORIENTED_EDGE('',*,*,#9574,.T.);
#13058=ORIENTED_EDGE('',*,*,#9489,.F.);
#13059=ORIENTED_EDGE('',*,*,#9576,.F.);
#13060=ORIENTED_EDGE('',*,*,#9502,.F.);
#13061=ORIENTED_EDGE('',*,*,#9557,.F.);
#13062=ORIENTED_EDGE('',*,*,#9577,.T.);
#13063=ORIENTED_EDGE('',*,*,#9496,.F.);
#13064=ORIENTED_EDGE('',*,*,#9575,.T.);
#13065=ORIENTED_EDGE('',*,*,#9516,.F.);
#13066=ORIENTED_EDGE('',*,*,#9003,.F.);
#13067=ORIENTED_EDGE('',*,*,#9578,.T.);
#13068=ORIENTED_EDGE('',*,*,#9563,.F.);
#13069=ORIENTED_EDGE('',*,*,#9503,.F.);
#13070=ORIENTED_EDGE('',*,*,#9576,.T.);
#13071=ORIENTED_EDGE('',*,*,#9497,.F.);
#13072=ORIENTED_EDGE('',*,*,#9579,.T.);
#13073=ORIENTED_EDGE('',*,*,#9477,.F.);
#13074=ORIENTED_EDGE('',*,*,#9580,.F.);
#13075=ORIENTED_EDGE('',*,*,#9471,.F.);
#13076=ORIENTED_EDGE('',*,*,#9581,.T.);
#13077=ORIENTED_EDGE('',*,*,#9002,.F.);
#13078=ORIENTED_EDGE('',*,*,#9582,.F.);
#13079=ORIENTED_EDGE('',*,*,#9580,.T.);
#13080=ORIENTED_EDGE('',*,*,#9513,.F.);
#13081=ORIENTED_EDGE('',*,*,#9512,.F.);
#13082=ORIENTED_EDGE('',*,*,#9582,.T.);
#13083=ORIENTED_EDGE('',*,*,#9001,.F.);
#13084=ORIENTED_EDGE('',*,*,#9498,.F.);
#13085=ORIENTED_EDGE('',*,*,#9583,.F.);
#13086=ORIENTED_EDGE('',*,*,#9527,.F.);
#13087=ORIENTED_EDGE('',*,*,#9584,.F.);
#13088=ORIENTED_EDGE('',*,*,#9486,.F.);
#13089=ORIENTED_EDGE('',*,*,#9485,.F.);
#13090=ORIENTED_EDGE('',*,*,#9584,.T.);
#13091=ORIENTED_EDGE('',*,*,#9538,.F.);
#13092=ORIENTED_EDGE('',*,*,#9537,.F.);
#13093=ORIENTED_EDGE('',*,*,#9536,.F.);
#13094=ORIENTED_EDGE('',*,*,#9535,.F.);
#13095=ORIENTED_EDGE('',*,*,#9534,.F.);
#13096=ORIENTED_EDGE('',*,*,#9585,.F.);
#13097=ORIENTED_EDGE('',*,*,#9487,.F.);
#13098=ORIENTED_EDGE('',*,*,#9583,.T.);
#13099=ORIENTED_EDGE('',*,*,#9484,.F.);
#13100=ORIENTED_EDGE('',*,*,#9006,.F.);
#13101=ORIENTED_EDGE('',*,*,#9586,.F.);
#13102=ORIENTED_EDGE('',*,*,#9549,.F.);
#13103=ORIENTED_EDGE('',*,*,#9548,.F.);
#13104=ORIENTED_EDGE('',*,*,#9547,.F.);
#13105=ORIENTED_EDGE('',*,*,#9546,.F.);
#13106=ORIENTED_EDGE('',*,*,#9545,.F.);
#13107=ORIENTED_EDGE('',*,*,#9585,.T.);
#13108=ORIENTED_EDGE('',*,*,#9554,.F.);
#13109=ORIENTED_EDGE('',*,*,#9586,.T.);
#13110=ORIENTED_EDGE('',*,*,#9005,.F.);
#13111=ORIENTED_EDGE('',*,*,#9488,.F.);
#13112=ORIENTED_EDGE('',*,*,#9587,.F.);
#13113=ORIENTED_EDGE('',*,*,#9578,.F.);
#13114=ORIENTED_EDGE('',*,*,#9581,.F.);
#13115=ORIENTED_EDGE('',*,*,#9470,.F.);
#13116=ORIENTED_EDGE('',*,*,#9588,.T.);
#13117=ORIENTED_EDGE('',*,*,#9561,.F.);
#13118=ORIENTED_EDGE('',*,*,#9587,.T.);
#13119=ORIENTED_EDGE('',*,*,#9158,.F.);
#13120=ORIENTED_EDGE('',*,*,#9589,.T.);
#13121=ORIENTED_EDGE('',*,*,#9469,.F.);
#13122=ORIENTED_EDGE('',*,*,#9468,.F.);
#13123=ORIENTED_EDGE('',*,*,#9590,.F.);
#13124=ORIENTED_EDGE('',*,*,#9590,.T.);
#13125=ORIENTED_EDGE('',*,*,#9511,.F.);
#13126=ORIENTED_EDGE('',*,*,#9510,.F.);
#13127=ORIENTED_EDGE('',*,*,#9591,.F.);
#13128=ORIENTED_EDGE('',*,*,#9213,.F.);
#13129=ORIENTED_EDGE('',*,*,#9159,.F.);
#13130=ORIENTED_EDGE('',*,*,#9479,.F.);
#13131=ORIENTED_EDGE('',*,*,#9592,.T.);
#13132=ORIENTED_EDGE('',*,*,#9214,.F.);
#13133=ORIENTED_EDGE('',*,*,#9591,.T.);
#13134=ORIENTED_EDGE('',*,*,#9480,.F.);
#13135=ORIENTED_EDGE('',*,*,#9224,.F.);
#13136=ORIENTED_EDGE('',*,*,#9593,.T.);
#13137=ORIENTED_EDGE('',*,*,#9564,.F.);
#13138=ORIENTED_EDGE('',*,*,#9594,.F.);
#13139=ORIENTED_EDGE('',*,*,#9152,.F.);
#13140=ORIENTED_EDGE('',*,*,#9499,.F.);
#13141=ORIENTED_EDGE('',*,*,#9154,.F.);
#13142=ORIENTED_EDGE('',*,*,#9153,.F.);
#13143=ORIENTED_EDGE('',*,*,#9594,.T.);
#13144=ORIENTED_EDGE('',*,*,#9155,.F.);
#13145=ORIENTED_EDGE('',*,*,#9505,.F.);
#13146=ORIENTED_EDGE('',*,*,#9595,.F.);
#13147=ORIENTED_EDGE('',*,*,#9156,.F.);
#13148=ORIENTED_EDGE('',*,*,#9596,.F.);
#13149=ORIENTED_EDGE('',*,*,#9157,.F.);
#13150=ORIENTED_EDGE('',*,*,#9595,.T.);
#13151=ORIENTED_EDGE('',*,*,#9562,.F.);
#13152=ORIENTED_EDGE('',*,*,#9596,.T.);
#13153=ORIENTED_EDGE('',*,*,#9588,.F.);
#13154=ORIENTED_EDGE('',*,*,#9589,.F.);
#13155=ORIENTED_EDGE('',*,*,#9514,.F.);
#13156=ORIENTED_EDGE('',*,*,#9217,.F.);
#13157=ORIENTED_EDGE('',*,*,#9216,.F.);
#13158=ORIENTED_EDGE('',*,*,#9597,.F.);
#13159=ORIENTED_EDGE('',*,*,#9597,.T.);
#13160=ORIENTED_EDGE('',*,*,#9215,.F.);
#13161=ORIENTED_EDGE('',*,*,#9598,.F.);
#13162=ORIENTED_EDGE('',*,*,#9555,.F.);
#13163=ORIENTED_EDGE('',*,*,#9598,.T.);
#13164=ORIENTED_EDGE('',*,*,#9592,.F.);
#13165=ORIENTED_EDGE('',*,*,#9599,.F.);
#13166=ORIENTED_EDGE('',*,*,#9600,.F.);
#13167=ORIENTED_EDGE('',*,*,#9556,.F.);
#13168=ORIENTED_EDGE('',*,*,#9599,.T.);
#13169=ORIENTED_EDGE('',*,*,#9478,.F.);
#13170=ORIENTED_EDGE('',*,*,#9579,.F.);
#13171=ORIENTED_EDGE('',*,*,#9577,.F.);
#13172=ORIENTED_EDGE('',*,*,#9600,.T.);
#13173=ORIENTED_EDGE('',*,*,#9218,.F.);
#13174=ORIENTED_EDGE('',*,*,#9520,.F.);
#13175=ORIENTED_EDGE('',*,*,#9601,.F.);
#13176=ORIENTED_EDGE('',*,*,#9219,.F.);
#13177=ORIENTED_EDGE('',*,*,#9601,.T.);
#13178=ORIENTED_EDGE('',*,*,#9560,.F.);
#13179=ORIENTED_EDGE('',*,*,#9602,.F.);
#13180=ORIENTED_EDGE('',*,*,#9220,.F.);
#13181=ORIENTED_EDGE('',*,*,#9571,.F.);
#13182=ORIENTED_EDGE('',*,*,#9474,.F.);
#13183=ORIENTED_EDGE('',*,*,#9473,.F.);
#13184=ORIENTED_EDGE('',*,*,#9603,.F.);
#13185=ORIENTED_EDGE('',*,*,#9221,.F.);
#13186=ORIENTED_EDGE('',*,*,#9602,.T.);
#13187=ORIENTED_EDGE('',*,*,#9559,.F.);
#13188=ORIENTED_EDGE('',*,*,#9603,.T.);
#13189=ORIENTED_EDGE('',*,*,#9507,.F.);
#13190=ORIENTED_EDGE('',*,*,#9506,.F.);
#13191=ORIENTED_EDGE('',*,*,#9604,.F.);
#13192=ORIENTED_EDGE('',*,*,#9222,.F.);
#13193=ORIENTED_EDGE('',*,*,#9605,.F.);
#13194=ORIENTED_EDGE('',*,*,#9223,.F.);
#13195=ORIENTED_EDGE('',*,*,#9604,.T.);
#13196=ORIENTED_EDGE('',*,*,#9465,.F.);
#13197=ORIENTED_EDGE('',*,*,#9464,.F.);
#13198=ORIENTED_EDGE('',*,*,#9593,.F.);
#13199=ORIENTED_EDGE('',*,*,#9605,.T.);
#13200=ORIENTED_EDGE('',*,*,#9606,.F.);
#13201=ORIENTED_EDGE('',*,*,#9607,.F.);
#13202=ORIENTED_EDGE('',*,*,#9565,.F.);
#13203=ORIENTED_EDGE('',*,*,#9606,.T.);
#13204=ORIENTED_EDGE('',*,*,#9463,.F.);
#13205=ORIENTED_EDGE('',*,*,#9607,.T.);
#13206=ORIENTED_EDGE('',*,*,#9570,.F.);
#13207=ORIENTED_EDGE('',*,*,#9573,.F.);
#13208=ORIENTED_EDGE('',*,*,#9608,.F.);
#13209=ORIENTED_EDGE('',*,*,#9008,.F.);
#13210=ORIENTED_EDGE('',*,*,#9454,.F.);
#13211=ORIENTED_EDGE('',*,*,#9012,.F.);
#13212=ORIENTED_EDGE('',*,*,#9609,.F.);
#13213=ORIENTED_EDGE('',*,*,#9544,.F.);
#13214=ORIENTED_EDGE('',*,*,#9543,.F.);
#13215=ORIENTED_EDGE('',*,*,#9542,.F.);
#13216=ORIENTED_EDGE('',*,*,#9541,.F.);
#13217=ORIENTED_EDGE('',*,*,#9540,.F.);
#13218=ORIENTED_EDGE('',*,*,#9609,.T.);
#13219=ORIENTED_EDGE('',*,*,#9011,.F.);
#13220=ORIENTED_EDGE('',*,*,#9610,.F.);
#13221=ORIENTED_EDGE('',*,*,#9525,.F.);
#13222=ORIENTED_EDGE('',*,*,#9524,.F.);
#13223=ORIENTED_EDGE('',*,*,#9523,.F.);
#13224=ORIENTED_EDGE('',*,*,#9522,.F.);
#13225=ORIENTED_EDGE('',*,*,#9608,.T.);
#13226=ORIENTED_EDGE('',*,*,#9553,.F.);
#13227=ORIENTED_EDGE('',*,*,#9552,.F.);
#13228=ORIENTED_EDGE('',*,*,#9551,.F.);
#13229=ORIENTED_EDGE('',*,*,#9550,.F.);
#13230=ORIENTED_EDGE('',*,*,#9611,.F.);
#13231=ORIENTED_EDGE('',*,*,#9009,.F.);
#13232=ORIENTED_EDGE('',*,*,#9610,.T.);
#13233=ORIENTED_EDGE('',*,*,#9010,.F.);
#13234=ORIENTED_EDGE('',*,*,#9611,.T.);
#13235=ORIENTED_EDGE('',*,*,#9532,.F.);
#13236=ORIENTED_EDGE('',*,*,#9531,.F.);
#13237=ORIENTED_EDGE('',*,*,#9530,.F.);
#13238=ORIENTED_EDGE('',*,*,#9529,.F.);
#13239=ORIENTED_EDGE('',*,*,#9528,.F.);
#13240=ORIENTED_EDGE('',*,*,#9483,.T.);
#13241=ORIENTED_EDGE('',*,*,#9612,.T.);
#13242=ORIENTED_EDGE('',*,*,#9201,.F.);
#13243=ORIENTED_EDGE('',*,*,#9461,.T.);
#13244=ORIENTED_EDGE('',*,*,#9168,.F.);
#13245=ORIENTED_EDGE('',*,*,#9613,.T.);
#13246=ORIENTED_EDGE('',*,*,#9614,.T.);
#13247=ORIENTED_EDGE('',*,*,#9615,.T.);
#13248=ORIENTED_EDGE('',*,*,#9616,.T.);
#13249=ORIENTED_EDGE('',*,*,#9617,.T.);
#13250=ORIENTED_EDGE('',*,*,#9618,.T.);
#13251=ORIENTED_EDGE('',*,*,#9619,.T.);
#13252=ORIENTED_EDGE('',*,*,#9620,.T.);
#13253=ORIENTED_EDGE('',*,*,#9621,.T.);
#13254=ORIENTED_EDGE('',*,*,#9622,.T.);
#13255=ORIENTED_EDGE('',*,*,#9623,.T.);
#13256=ORIENTED_EDGE('',*,*,#9624,.T.);
#13257=ORIENTED_EDGE('',*,*,#9625,.T.);
#13258=ORIENTED_EDGE('',*,*,#9626,.T.);
#13259=ORIENTED_EDGE('',*,*,#9627,.T.);
#13260=ORIENTED_EDGE('',*,*,#9628,.T.);
#13261=ORIENTED_EDGE('',*,*,#9629,.T.);
#13262=ORIENTED_EDGE('',*,*,#9630,.T.);
#13263=ORIENTED_EDGE('',*,*,#9631,.T.);
#13264=ORIENTED_EDGE('',*,*,#9632,.T.);
#13265=ORIENTED_EDGE('',*,*,#9633,.T.);
#13266=ORIENTED_EDGE('',*,*,#9634,.T.);
#13267=ORIENTED_EDGE('',*,*,#9635,.T.);
#13268=ORIENTED_EDGE('',*,*,#9636,.T.);
#13269=ORIENTED_EDGE('',*,*,#9637,.T.);
#13270=ORIENTED_EDGE('',*,*,#9638,.T.);
#13271=ORIENTED_EDGE('',*,*,#9639,.T.);
#13272=ORIENTED_EDGE('',*,*,#9640,.T.);
#13273=ORIENTED_EDGE('',*,*,#9641,.T.);
#13274=ORIENTED_EDGE('',*,*,#9642,.T.);
#13275=ORIENTED_EDGE('',*,*,#9643,.T.);
#13276=ORIENTED_EDGE('',*,*,#9644,.T.);
#13277=ORIENTED_EDGE('',*,*,#9645,.T.);
#13278=ORIENTED_EDGE('',*,*,#9646,.T.);
#13279=ORIENTED_EDGE('',*,*,#9647,.T.);
#13280=ORIENTED_EDGE('',*,*,#9648,.T.);
#13281=ORIENTED_EDGE('',*,*,#9649,.T.);
#13282=ORIENTED_EDGE('',*,*,#9650,.T.);
#13283=ORIENTED_EDGE('',*,*,#9651,.T.);
#13284=ORIENTED_EDGE('',*,*,#9652,.T.);
#13285=ORIENTED_EDGE('',*,*,#9653,.T.);
#13286=ORIENTED_EDGE('',*,*,#9654,.T.);
#13287=ORIENTED_EDGE('',*,*,#9655,.T.);
#13288=ORIENTED_EDGE('',*,*,#9656,.T.);
#13289=ORIENTED_EDGE('',*,*,#9657,.T.);
#13290=ORIENTED_EDGE('',*,*,#9658,.T.);
#13291=ORIENTED_EDGE('',*,*,#9659,.T.);
#13292=ORIENTED_EDGE('',*,*,#9660,.T.);
#13293=ORIENTED_EDGE('',*,*,#9661,.T.);
#13294=ORIENTED_EDGE('',*,*,#9662,.T.);
#13295=ORIENTED_EDGE('',*,*,#9663,.T.);
#13296=ORIENTED_EDGE('',*,*,#9664,.T.);
#13297=ORIENTED_EDGE('',*,*,#9665,.T.);
#13298=ORIENTED_EDGE('',*,*,#9666,.T.);
#13299=ORIENTED_EDGE('',*,*,#9667,.T.);
#13300=ORIENTED_EDGE('',*,*,#9668,.T.);
#13301=ORIENTED_EDGE('',*,*,#9669,.T.);
#13302=ORIENTED_EDGE('',*,*,#9670,.T.);
#13303=ORIENTED_EDGE('',*,*,#9671,.T.);
#13304=ORIENTED_EDGE('',*,*,#9672,.T.);
#13305=ORIENTED_EDGE('',*,*,#9673,.T.);
#13306=ORIENTED_EDGE('',*,*,#9674,.T.);
#13307=ORIENTED_EDGE('',*,*,#9675,.T.);
#13308=ORIENTED_EDGE('',*,*,#9676,.T.);
#13309=ORIENTED_EDGE('',*,*,#9677,.T.);
#13310=ORIENTED_EDGE('',*,*,#9678,.T.);
#13311=ORIENTED_EDGE('',*,*,#9679,.T.);
#13312=ORIENTED_EDGE('',*,*,#9680,.T.);
#13313=ORIENTED_EDGE('',*,*,#9681,.T.);
#13314=ORIENTED_EDGE('',*,*,#9682,.T.);
#13315=ORIENTED_EDGE('',*,*,#9683,.T.);
#13316=ORIENTED_EDGE('',*,*,#9684,.T.);
#13317=ORIENTED_EDGE('',*,*,#9685,.T.);
#13318=ORIENTED_EDGE('',*,*,#9686,.T.);
#13319=ORIENTED_EDGE('',*,*,#9687,.T.);
#13320=ORIENTED_EDGE('',*,*,#9688,.T.);
#13321=ORIENTED_EDGE('',*,*,#9689,.T.);
#13322=ORIENTED_EDGE('',*,*,#9690,.T.);
#13323=ORIENTED_EDGE('',*,*,#9691,.T.);
#13324=ORIENTED_EDGE('',*,*,#9692,.T.);
#13325=ORIENTED_EDGE('',*,*,#9693,.T.);
#13326=ORIENTED_EDGE('',*,*,#9694,.T.);
#13327=ORIENTED_EDGE('',*,*,#9695,.T.);
#13328=ORIENTED_EDGE('',*,*,#9696,.T.);
#13329=ORIENTED_EDGE('',*,*,#9697,.T.);
#13330=ORIENTED_EDGE('',*,*,#9698,.T.);
#13331=ORIENTED_EDGE('',*,*,#9699,.T.);
#13332=ORIENTED_EDGE('',*,*,#9700,.T.);
#13333=ORIENTED_EDGE('',*,*,#9701,.T.);
#13334=ORIENTED_EDGE('',*,*,#9702,.T.);
#13335=ORIENTED_EDGE('',*,*,#9703,.T.);
#13336=ORIENTED_EDGE('',*,*,#9704,.T.);
#13337=ORIENTED_EDGE('',*,*,#9705,.T.);
#13338=ORIENTED_EDGE('',*,*,#9706,.T.);
#13339=ORIENTED_EDGE('',*,*,#9707,.T.);
#13340=ORIENTED_EDGE('',*,*,#9708,.T.);
#13341=ORIENTED_EDGE('',*,*,#9709,.T.);
#13342=ORIENTED_EDGE('',*,*,#9710,.T.);
#13343=ORIENTED_EDGE('',*,*,#9711,.T.);
#13344=ORIENTED_EDGE('',*,*,#9712,.T.);
#13345=ORIENTED_EDGE('',*,*,#9713,.T.);
#13346=ORIENTED_EDGE('',*,*,#9714,.T.);
#13347=ORIENTED_EDGE('',*,*,#9715,.T.);
#13348=ORIENTED_EDGE('',*,*,#9716,.T.);
#13349=ORIENTED_EDGE('',*,*,#9717,.T.);
#13350=ORIENTED_EDGE('',*,*,#9718,.T.);
#13351=ORIENTED_EDGE('',*,*,#9719,.T.);
#13352=ORIENTED_EDGE('',*,*,#9720,.T.);
#13353=ORIENTED_EDGE('',*,*,#9721,.T.);
#13354=ORIENTED_EDGE('',*,*,#9198,.T.);
#13355=ORIENTED_EDGE('',*,*,#9722,.T.);
#13356=ORIENTED_EDGE('',*,*,#9212,.T.);
#13357=ORIENTED_EDGE('',*,*,#9723,.F.);
#13358=ORIENTED_EDGE('',*,*,#9211,.T.);
#13359=ORIENTED_EDGE('',*,*,#9456,.T.);
#13360=ORIENTED_EDGE('',*,*,#9199,.T.);
#13361=ORIENTED_EDGE('',*,*,#9723,.T.);
#13362=ORIENTED_EDGE('',*,*,#9724,.F.);
#13363=ORIENTED_EDGE('',*,*,#9725,.F.);
#13364=ORIENTED_EDGE('',*,*,#9726,.F.);
#13365=ORIENTED_EDGE('',*,*,#9727,.F.);
#13366=ORIENTED_EDGE('',*,*,#9728,.F.);
#13367=ORIENTED_EDGE('',*,*,#9729,.F.);
#13368=ORIENTED_EDGE('',*,*,#9730,.F.);
#13369=ORIENTED_EDGE('',*,*,#9731,.F.);
#13370=ORIENTED_EDGE('',*,*,#9732,.F.);
#13371=ORIENTED_EDGE('',*,*,#9733,.F.);
#13372=ORIENTED_EDGE('',*,*,#9734,.F.);
#13373=ORIENTED_EDGE('',*,*,#9735,.F.);
#13374=ORIENTED_EDGE('',*,*,#9736,.F.);
#13375=ORIENTED_EDGE('',*,*,#9737,.F.);
#13376=ORIENTED_EDGE('',*,*,#9738,.F.);
#13377=ORIENTED_EDGE('',*,*,#9739,.F.);
#13378=ORIENTED_EDGE('',*,*,#9740,.F.);
#13379=ORIENTED_EDGE('',*,*,#9741,.F.);
#13380=ORIENTED_EDGE('',*,*,#9742,.F.);
#13381=ORIENTED_EDGE('',*,*,#9743,.F.);
#13382=ORIENTED_EDGE('',*,*,#9744,.F.);
#13383=ORIENTED_EDGE('',*,*,#9745,.F.);
#13384=ORIENTED_EDGE('',*,*,#9746,.F.);
#13385=ORIENTED_EDGE('',*,*,#9747,.F.);
#13386=ORIENTED_EDGE('',*,*,#9748,.F.);
#13387=ORIENTED_EDGE('',*,*,#9749,.F.);
#13388=ORIENTED_EDGE('',*,*,#9750,.F.);
#13389=ORIENTED_EDGE('',*,*,#9751,.F.);
#13390=ORIENTED_EDGE('',*,*,#9752,.F.);
#13391=ORIENTED_EDGE('',*,*,#9753,.F.);
#13392=ORIENTED_EDGE('',*,*,#9754,.F.);
#13393=ORIENTED_EDGE('',*,*,#9755,.F.);
#13394=ORIENTED_EDGE('',*,*,#9756,.F.);
#13395=ORIENTED_EDGE('',*,*,#9757,.F.);
#13396=ORIENTED_EDGE('',*,*,#9758,.F.);
#13397=ORIENTED_EDGE('',*,*,#9759,.F.);
#13398=ORIENTED_EDGE('',*,*,#9760,.F.);
#13399=ORIENTED_EDGE('',*,*,#9761,.F.);
#13400=ORIENTED_EDGE('',*,*,#9762,.F.);
#13401=ORIENTED_EDGE('',*,*,#9763,.F.);
#13402=ORIENTED_EDGE('',*,*,#9764,.F.);
#13403=ORIENTED_EDGE('',*,*,#9765,.F.);
#13404=ORIENTED_EDGE('',*,*,#9766,.F.);
#13405=ORIENTED_EDGE('',*,*,#9767,.F.);
#13406=ORIENTED_EDGE('',*,*,#9768,.F.);
#13407=ORIENTED_EDGE('',*,*,#9769,.F.);
#13408=ORIENTED_EDGE('',*,*,#9770,.F.);
#13409=ORIENTED_EDGE('',*,*,#9771,.F.);
#13410=ORIENTED_EDGE('',*,*,#9772,.F.);
#13411=ORIENTED_EDGE('',*,*,#9773,.F.);
#13412=ORIENTED_EDGE('',*,*,#9774,.F.);
#13413=ORIENTED_EDGE('',*,*,#9775,.F.);
#13414=ORIENTED_EDGE('',*,*,#9776,.F.);
#13415=ORIENTED_EDGE('',*,*,#9777,.F.);
#13416=ORIENTED_EDGE('',*,*,#9778,.F.);
#13417=ORIENTED_EDGE('',*,*,#9779,.F.);
#13418=ORIENTED_EDGE('',*,*,#9780,.F.);
#13419=ORIENTED_EDGE('',*,*,#9781,.F.);
#13420=ORIENTED_EDGE('',*,*,#9782,.F.);
#13421=ORIENTED_EDGE('',*,*,#9783,.F.);
#13422=ORIENTED_EDGE('',*,*,#9784,.F.);
#13423=ORIENTED_EDGE('',*,*,#9785,.F.);
#13424=ORIENTED_EDGE('',*,*,#9786,.F.);
#13425=ORIENTED_EDGE('',*,*,#9787,.F.);
#13426=ORIENTED_EDGE('',*,*,#9788,.F.);
#13427=ORIENTED_EDGE('',*,*,#9789,.F.);
#13428=ORIENTED_EDGE('',*,*,#9790,.F.);
#13429=ORIENTED_EDGE('',*,*,#9791,.F.);
#13430=ORIENTED_EDGE('',*,*,#9792,.F.);
#13431=ORIENTED_EDGE('',*,*,#9793,.F.);
#13432=ORIENTED_EDGE('',*,*,#9794,.F.);
#13433=ORIENTED_EDGE('',*,*,#9795,.F.);
#13434=ORIENTED_EDGE('',*,*,#9796,.F.);
#13435=ORIENTED_EDGE('',*,*,#9797,.F.);
#13436=ORIENTED_EDGE('',*,*,#9798,.F.);
#13437=ORIENTED_EDGE('',*,*,#9799,.F.);
#13438=ORIENTED_EDGE('',*,*,#9800,.F.);
#13439=ORIENTED_EDGE('',*,*,#9801,.F.);
#13440=ORIENTED_EDGE('',*,*,#9802,.F.);
#13441=ORIENTED_EDGE('',*,*,#9803,.F.);
#13442=ORIENTED_EDGE('',*,*,#9804,.F.);
#13443=ORIENTED_EDGE('',*,*,#9805,.F.);
#13444=ORIENTED_EDGE('',*,*,#9806,.F.);
#13445=ORIENTED_EDGE('',*,*,#9807,.F.);
#13446=ORIENTED_EDGE('',*,*,#9808,.F.);
#13447=ORIENTED_EDGE('',*,*,#9809,.F.);
#13448=ORIENTED_EDGE('',*,*,#9810,.F.);
#13449=ORIENTED_EDGE('',*,*,#9811,.F.);
#13450=ORIENTED_EDGE('',*,*,#9812,.F.);
#13451=ORIENTED_EDGE('',*,*,#9813,.F.);
#13452=ORIENTED_EDGE('',*,*,#9814,.F.);
#13453=ORIENTED_EDGE('',*,*,#9815,.F.);
#13454=ORIENTED_EDGE('',*,*,#9816,.F.);
#13455=ORIENTED_EDGE('',*,*,#9817,.F.);
#13456=ORIENTED_EDGE('',*,*,#9818,.F.);
#13457=ORIENTED_EDGE('',*,*,#9819,.F.);
#13458=ORIENTED_EDGE('',*,*,#9820,.F.);
#13459=ORIENTED_EDGE('',*,*,#9821,.F.);
#13460=ORIENTED_EDGE('',*,*,#9822,.F.);
#13461=ORIENTED_EDGE('',*,*,#9823,.F.);
#13462=ORIENTED_EDGE('',*,*,#9824,.F.);
#13463=ORIENTED_EDGE('',*,*,#9825,.F.);
#13464=ORIENTED_EDGE('',*,*,#9612,.F.);
#13465=ORIENTED_EDGE('',*,*,#9482,.T.);
#13466=ORIENTED_EDGE('',*,*,#9457,.F.);
#13467=ORIENTED_EDGE('',*,*,#9202,.F.);
#13468=ORIENTED_EDGE('',*,*,#9197,.F.);
#13469=ORIENTED_EDGE('',*,*,#9455,.T.);
#13470=ORIENTED_EDGE('',*,*,#9209,.T.);
#13471=ORIENTED_EDGE('',*,*,#9722,.F.);
#13472=ORIENTED_EDGE('',*,*,#9826,.F.);
#13473=ORIENTED_EDGE('',*,*,#9330,.F.);
#13474=ORIENTED_EDGE('',*,*,#9827,.F.);
#13475=ORIENTED_EDGE('',*,*,#9624,.F.);
#13476=ORIENTED_EDGE('',*,*,#9827,.T.);
#13477=ORIENTED_EDGE('',*,*,#9329,.F.);
#13478=ORIENTED_EDGE('',*,*,#9828,.F.);
#13479=ORIENTED_EDGE('',*,*,#9625,.F.);
#13480=ORIENTED_EDGE('',*,*,#9826,.T.);
#13481=ORIENTED_EDGE('',*,*,#9623,.F.);
#13482=ORIENTED_EDGE('',*,*,#9829,.F.);
#13483=ORIENTED_EDGE('',*,*,#9331,.F.);
#13484=ORIENTED_EDGE('',*,*,#9828,.T.);
#13485=ORIENTED_EDGE('',*,*,#9328,.F.);
#13486=ORIENTED_EDGE('',*,*,#9830,.F.);
#13487=ORIENTED_EDGE('',*,*,#9620,.F.);
#13488=ORIENTED_EDGE('',*,*,#9829,.T.);
#13489=ORIENTED_EDGE('',*,*,#9622,.F.);
#13490=ORIENTED_EDGE('',*,*,#9831,.F.);
#13491=ORIENTED_EDGE('',*,*,#9326,.F.);
#13492=ORIENTED_EDGE('',*,*,#9830,.T.);
#13493=ORIENTED_EDGE('',*,*,#9327,.F.);
#13494=ORIENTED_EDGE('',*,*,#9831,.T.);
#13495=ORIENTED_EDGE('',*,*,#9621,.F.);
#13496=ORIENTED_EDGE('',*,*,#9832,.F.);
#13497=ORIENTED_EDGE('',*,*,#9336,.F.);
#13498=ORIENTED_EDGE('',*,*,#9833,.F.);
#13499=ORIENTED_EDGE('',*,*,#9630,.F.);
#13500=ORIENTED_EDGE('',*,*,#9833,.T.);
#13501=ORIENTED_EDGE('',*,*,#9335,.F.);
#13502=ORIENTED_EDGE('',*,*,#9834,.F.);
#13503=ORIENTED_EDGE('',*,*,#9631,.F.);
#13504=ORIENTED_EDGE('',*,*,#9832,.T.);
#13505=ORIENTED_EDGE('',*,*,#9629,.F.);
#13506=ORIENTED_EDGE('',*,*,#9835,.F.);
#13507=ORIENTED_EDGE('',*,*,#9337,.F.);
#13508=ORIENTED_EDGE('',*,*,#9834,.T.);
#13509=ORIENTED_EDGE('',*,*,#9334,.F.);
#13510=ORIENTED_EDGE('',*,*,#9836,.F.);
#13511=ORIENTED_EDGE('',*,*,#9626,.F.);
#13512=ORIENTED_EDGE('',*,*,#9835,.T.);
#13513=ORIENTED_EDGE('',*,*,#9628,.F.);
#13514=ORIENTED_EDGE('',*,*,#9837,.F.);
#13515=ORIENTED_EDGE('',*,*,#9332,.F.);
#13516=ORIENTED_EDGE('',*,*,#9836,.T.);
#13517=ORIENTED_EDGE('',*,*,#9333,.F.);
#13518=ORIENTED_EDGE('',*,*,#9837,.T.);
#13519=ORIENTED_EDGE('',*,*,#9627,.F.);
#13520=ORIENTED_EDGE('',*,*,#9838,.F.);
#13521=ORIENTED_EDGE('',*,*,#9342,.F.);
#13522=ORIENTED_EDGE('',*,*,#9839,.F.);
#13523=ORIENTED_EDGE('',*,*,#9636,.F.);
#13524=ORIENTED_EDGE('',*,*,#9839,.T.);
#13525=ORIENTED_EDGE('',*,*,#9341,.F.);
#13526=ORIENTED_EDGE('',*,*,#9840,.F.);
#13527=ORIENTED_EDGE('',*,*,#9637,.F.);
#13528=ORIENTED_EDGE('',*,*,#9838,.T.);
#13529=ORIENTED_EDGE('',*,*,#9635,.F.);
#13530=ORIENTED_EDGE('',*,*,#9841,.F.);
#13531=ORIENTED_EDGE('',*,*,#9343,.F.);
#13532=ORIENTED_EDGE('',*,*,#9840,.T.);
#13533=ORIENTED_EDGE('',*,*,#9340,.F.);
#13534=ORIENTED_EDGE('',*,*,#9842,.F.);
#13535=ORIENTED_EDGE('',*,*,#9632,.F.);
#13536=ORIENTED_EDGE('',*,*,#9841,.T.);
#13537=ORIENTED_EDGE('',*,*,#9634,.F.);
#13538=ORIENTED_EDGE('',*,*,#9843,.F.);
#13539=ORIENTED_EDGE('',*,*,#9338,.F.);
#13540=ORIENTED_EDGE('',*,*,#9842,.T.);
#13541=ORIENTED_EDGE('',*,*,#9339,.F.);
#13542=ORIENTED_EDGE('',*,*,#9843,.T.);
#13543=ORIENTED_EDGE('',*,*,#9633,.F.);
#13544=ORIENTED_EDGE('',*,*,#9844,.F.);
#13545=ORIENTED_EDGE('',*,*,#9348,.F.);
#13546=ORIENTED_EDGE('',*,*,#9845,.F.);
#13547=ORIENTED_EDGE('',*,*,#9642,.F.);
#13548=ORIENTED_EDGE('',*,*,#9845,.T.);
#13549=ORIENTED_EDGE('',*,*,#9347,.F.);
#13550=ORIENTED_EDGE('',*,*,#9846,.F.);
#13551=ORIENTED_EDGE('',*,*,#9643,.F.);
#13552=ORIENTED_EDGE('',*,*,#9844,.T.);
#13553=ORIENTED_EDGE('',*,*,#9641,.F.);
#13554=ORIENTED_EDGE('',*,*,#9847,.F.);
#13555=ORIENTED_EDGE('',*,*,#9349,.F.);
#13556=ORIENTED_EDGE('',*,*,#9846,.T.);
#13557=ORIENTED_EDGE('',*,*,#9346,.F.);
#13558=ORIENTED_EDGE('',*,*,#9848,.F.);
#13559=ORIENTED_EDGE('',*,*,#9638,.F.);
#13560=ORIENTED_EDGE('',*,*,#9847,.T.);
#13561=ORIENTED_EDGE('',*,*,#9640,.F.);
#13562=ORIENTED_EDGE('',*,*,#9849,.F.);
#13563=ORIENTED_EDGE('',*,*,#9344,.F.);
#13564=ORIENTED_EDGE('',*,*,#9848,.T.);
#13565=ORIENTED_EDGE('',*,*,#9345,.F.);
#13566=ORIENTED_EDGE('',*,*,#9849,.T.);
#13567=ORIENTED_EDGE('',*,*,#9639,.F.);
#13568=ORIENTED_EDGE('',*,*,#9850,.F.);
#13569=ORIENTED_EDGE('',*,*,#9354,.F.);
#13570=ORIENTED_EDGE('',*,*,#9851,.F.);
#13571=ORIENTED_EDGE('',*,*,#9648,.F.);
#13572=ORIENTED_EDGE('',*,*,#9851,.T.);
#13573=ORIENTED_EDGE('',*,*,#9353,.F.);
#13574=ORIENTED_EDGE('',*,*,#9852,.F.);
#13575=ORIENTED_EDGE('',*,*,#9649,.F.);
#13576=ORIENTED_EDGE('',*,*,#9850,.T.);
#13577=ORIENTED_EDGE('',*,*,#9647,.F.);
#13578=ORIENTED_EDGE('',*,*,#9853,.F.);
#13579=ORIENTED_EDGE('',*,*,#9355,.F.);
#13580=ORIENTED_EDGE('',*,*,#9852,.T.);
#13581=ORIENTED_EDGE('',*,*,#9352,.F.);
#13582=ORIENTED_EDGE('',*,*,#9854,.F.);
#13583=ORIENTED_EDGE('',*,*,#9644,.F.);
#13584=ORIENTED_EDGE('',*,*,#9853,.T.);
#13585=ORIENTED_EDGE('',*,*,#9646,.F.);
#13586=ORIENTED_EDGE('',*,*,#9855,.F.);
#13587=ORIENTED_EDGE('',*,*,#9350,.F.);
#13588=ORIENTED_EDGE('',*,*,#9854,.T.);
#13589=ORIENTED_EDGE('',*,*,#9351,.F.);
#13590=ORIENTED_EDGE('',*,*,#9855,.T.);
#13591=ORIENTED_EDGE('',*,*,#9645,.F.);
#13592=ORIENTED_EDGE('',*,*,#9856,.F.);
#13593=ORIENTED_EDGE('',*,*,#9360,.F.);
#13594=ORIENTED_EDGE('',*,*,#9857,.F.);
#13595=ORIENTED_EDGE('',*,*,#9654,.F.);
#13596=ORIENTED_EDGE('',*,*,#9857,.T.);
#13597=ORIENTED_EDGE('',*,*,#9359,.F.);
#13598=ORIENTED_EDGE('',*,*,#9858,.F.);
#13599=ORIENTED_EDGE('',*,*,#9655,.F.);
#13600=ORIENTED_EDGE('',*,*,#9856,.T.);
#13601=ORIENTED_EDGE('',*,*,#9653,.F.);
#13602=ORIENTED_EDGE('',*,*,#9859,.F.);
#13603=ORIENTED_EDGE('',*,*,#9361,.F.);
#13604=ORIENTED_EDGE('',*,*,#9858,.T.);
#13605=ORIENTED_EDGE('',*,*,#9358,.F.);
#13606=ORIENTED_EDGE('',*,*,#9860,.F.);
#13607=ORIENTED_EDGE('',*,*,#9650,.F.);
#13608=ORIENTED_EDGE('',*,*,#9859,.T.);
#13609=ORIENTED_EDGE('',*,*,#9652,.F.);
#13610=ORIENTED_EDGE('',*,*,#9861,.F.);
#13611=ORIENTED_EDGE('',*,*,#9356,.F.);
#13612=ORIENTED_EDGE('',*,*,#9860,.T.);
#13613=ORIENTED_EDGE('',*,*,#9357,.F.);
#13614=ORIENTED_EDGE('',*,*,#9861,.T.);
#13615=ORIENTED_EDGE('',*,*,#9651,.F.);
#13616=ORIENTED_EDGE('',*,*,#9862,.F.);
#13617=ORIENTED_EDGE('',*,*,#9369,.F.);
#13618=ORIENTED_EDGE('',*,*,#9368,.F.);
#13619=ORIENTED_EDGE('',*,*,#9863,.F.);
#13620=ORIENTED_EDGE('',*,*,#9660,.F.);
#13621=ORIENTED_EDGE('',*,*,#9863,.T.);
#13622=ORIENTED_EDGE('',*,*,#9367,.F.);
#13623=ORIENTED_EDGE('',*,*,#9864,.F.);
#13624=ORIENTED_EDGE('',*,*,#9661,.F.);
#13625=ORIENTED_EDGE('',*,*,#9862,.T.);
#13626=ORIENTED_EDGE('',*,*,#9659,.F.);
#13627=ORIENTED_EDGE('',*,*,#9865,.F.);
#13628=ORIENTED_EDGE('',*,*,#9371,.F.);
#13629=ORIENTED_EDGE('',*,*,#9370,.F.);
#13630=ORIENTED_EDGE('',*,*,#9864,.T.);
#13631=ORIENTED_EDGE('',*,*,#9366,.F.);
#13632=ORIENTED_EDGE('',*,*,#9365,.F.);
#13633=ORIENTED_EDGE('',*,*,#9866,.F.);
#13634=ORIENTED_EDGE('',*,*,#9656,.F.);
#13635=ORIENTED_EDGE('',*,*,#9865,.T.);
#13636=ORIENTED_EDGE('',*,*,#9658,.F.);
#13637=ORIENTED_EDGE('',*,*,#9867,.F.);
#13638=ORIENTED_EDGE('',*,*,#9362,.F.);
#13639=ORIENTED_EDGE('',*,*,#9866,.T.);
#13640=ORIENTED_EDGE('',*,*,#9364,.F.);
#13641=ORIENTED_EDGE('',*,*,#9363,.F.);
#13642=ORIENTED_EDGE('',*,*,#9867,.T.);
#13643=ORIENTED_EDGE('',*,*,#9657,.F.);
#13644=ORIENTED_EDGE('',*,*,#9868,.F.);
#13645=ORIENTED_EDGE('',*,*,#9376,.F.);
#13646=ORIENTED_EDGE('',*,*,#9869,.F.);
#13647=ORIENTED_EDGE('',*,*,#9666,.F.);
#13648=ORIENTED_EDGE('',*,*,#9869,.T.);
#13649=ORIENTED_EDGE('',*,*,#9375,.F.);
#13650=ORIENTED_EDGE('',*,*,#9870,.F.);
#13651=ORIENTED_EDGE('',*,*,#9667,.F.);
#13652=ORIENTED_EDGE('',*,*,#9868,.T.);
#13653=ORIENTED_EDGE('',*,*,#9665,.F.);
#13654=ORIENTED_EDGE('',*,*,#9871,.F.);
#13655=ORIENTED_EDGE('',*,*,#9377,.F.);
#13656=ORIENTED_EDGE('',*,*,#9870,.T.);
#13657=ORIENTED_EDGE('',*,*,#9374,.F.);
#13658=ORIENTED_EDGE('',*,*,#9872,.F.);
#13659=ORIENTED_EDGE('',*,*,#9662,.F.);
#13660=ORIENTED_EDGE('',*,*,#9871,.T.);
#13661=ORIENTED_EDGE('',*,*,#9664,.F.);
#13662=ORIENTED_EDGE('',*,*,#9873,.F.);
#13663=ORIENTED_EDGE('',*,*,#9372,.F.);
#13664=ORIENTED_EDGE('',*,*,#9872,.T.);
#13665=ORIENTED_EDGE('',*,*,#9373,.F.);
#13666=ORIENTED_EDGE('',*,*,#9873,.T.);
#13667=ORIENTED_EDGE('',*,*,#9663,.F.);
#13668=ORIENTED_EDGE('',*,*,#9874,.F.);
#13669=ORIENTED_EDGE('',*,*,#9382,.F.);
#13670=ORIENTED_EDGE('',*,*,#9875,.F.);
#13671=ORIENTED_EDGE('',*,*,#9672,.F.);
#13672=ORIENTED_EDGE('',*,*,#9875,.T.);
#13673=ORIENTED_EDGE('',*,*,#9381,.F.);
#13674=ORIENTED_EDGE('',*,*,#9876,.F.);
#13675=ORIENTED_EDGE('',*,*,#9673,.F.);
#13676=ORIENTED_EDGE('',*,*,#9874,.T.);
#13677=ORIENTED_EDGE('',*,*,#9671,.F.);
#13678=ORIENTED_EDGE('',*,*,#9877,.F.);
#13679=ORIENTED_EDGE('',*,*,#9383,.F.);
#13680=ORIENTED_EDGE('',*,*,#9876,.T.);
#13681=ORIENTED_EDGE('',*,*,#9380,.F.);
#13682=ORIENTED_EDGE('',*,*,#9878,.F.);
#13683=ORIENTED_EDGE('',*,*,#9668,.F.);
#13684=ORIENTED_EDGE('',*,*,#9877,.T.);
#13685=ORIENTED_EDGE('',*,*,#9670,.F.);
#13686=ORIENTED_EDGE('',*,*,#9879,.F.);
#13687=ORIENTED_EDGE('',*,*,#9378,.F.);
#13688=ORIENTED_EDGE('',*,*,#9878,.T.);
#13689=ORIENTED_EDGE('',*,*,#9379,.F.);
#13690=ORIENTED_EDGE('',*,*,#9879,.T.);
#13691=ORIENTED_EDGE('',*,*,#9669,.F.);
#13692=ORIENTED_EDGE('',*,*,#9880,.F.);
#13693=ORIENTED_EDGE('',*,*,#9388,.F.);
#13694=ORIENTED_EDGE('',*,*,#9881,.F.);
#13695=ORIENTED_EDGE('',*,*,#9678,.F.);
#13696=ORIENTED_EDGE('',*,*,#9881,.T.);
#13697=ORIENTED_EDGE('',*,*,#9387,.F.);
#13698=ORIENTED_EDGE('',*,*,#9882,.F.);
#13699=ORIENTED_EDGE('',*,*,#9679,.F.);
#13700=ORIENTED_EDGE('',*,*,#9880,.T.);
#13701=ORIENTED_EDGE('',*,*,#9677,.F.);
#13702=ORIENTED_EDGE('',*,*,#9883,.F.);
#13703=ORIENTED_EDGE('',*,*,#9389,.F.);
#13704=ORIENTED_EDGE('',*,*,#9882,.T.);
#13705=ORIENTED_EDGE('',*,*,#9386,.F.);
#13706=ORIENTED_EDGE('',*,*,#9884,.F.);
#13707=ORIENTED_EDGE('',*,*,#9674,.F.);
#13708=ORIENTED_EDGE('',*,*,#9883,.T.);
#13709=ORIENTED_EDGE('',*,*,#9676,.F.);
#13710=ORIENTED_EDGE('',*,*,#9885,.F.);
#13711=ORIENTED_EDGE('',*,*,#9384,.F.);
#13712=ORIENTED_EDGE('',*,*,#9884,.T.);
#13713=ORIENTED_EDGE('',*,*,#9385,.F.);
#13714=ORIENTED_EDGE('',*,*,#9885,.T.);
#13715=ORIENTED_EDGE('',*,*,#9675,.F.);
#13716=ORIENTED_EDGE('',*,*,#9886,.F.);
#13717=ORIENTED_EDGE('',*,*,#9394,.F.);
#13718=ORIENTED_EDGE('',*,*,#9887,.F.);
#13719=ORIENTED_EDGE('',*,*,#9684,.F.);
#13720=ORIENTED_EDGE('',*,*,#9887,.T.);
#13721=ORIENTED_EDGE('',*,*,#9393,.F.);
#13722=ORIENTED_EDGE('',*,*,#9888,.F.);
#13723=ORIENTED_EDGE('',*,*,#9685,.F.);
#13724=ORIENTED_EDGE('',*,*,#9886,.T.);
#13725=ORIENTED_EDGE('',*,*,#9683,.F.);
#13726=ORIENTED_EDGE('',*,*,#9889,.F.);
#13727=ORIENTED_EDGE('',*,*,#9395,.F.);
#13728=ORIENTED_EDGE('',*,*,#9888,.T.);
#13729=ORIENTED_EDGE('',*,*,#9392,.F.);
#13730=ORIENTED_EDGE('',*,*,#9890,.F.);
#13731=ORIENTED_EDGE('',*,*,#9680,.F.);
#13732=ORIENTED_EDGE('',*,*,#9889,.T.);
#13733=ORIENTED_EDGE('',*,*,#9682,.F.);
#13734=ORIENTED_EDGE('',*,*,#9891,.F.);
#13735=ORIENTED_EDGE('',*,*,#9390,.F.);
#13736=ORIENTED_EDGE('',*,*,#9890,.T.);
#13737=ORIENTED_EDGE('',*,*,#9391,.F.);
#13738=ORIENTED_EDGE('',*,*,#9891,.T.);
#13739=ORIENTED_EDGE('',*,*,#9681,.F.);
#13740=ORIENTED_EDGE('',*,*,#9892,.F.);
#13741=ORIENTED_EDGE('',*,*,#9400,.F.);
#13742=ORIENTED_EDGE('',*,*,#9893,.F.);
#13743=ORIENTED_EDGE('',*,*,#9690,.F.);
#13744=ORIENTED_EDGE('',*,*,#9893,.T.);
#13745=ORIENTED_EDGE('',*,*,#9399,.F.);
#13746=ORIENTED_EDGE('',*,*,#9894,.F.);
#13747=ORIENTED_EDGE('',*,*,#9691,.F.);
#13748=ORIENTED_EDGE('',*,*,#9892,.T.);
#13749=ORIENTED_EDGE('',*,*,#9689,.F.);
#13750=ORIENTED_EDGE('',*,*,#9895,.F.);
#13751=ORIENTED_EDGE('',*,*,#9401,.F.);
#13752=ORIENTED_EDGE('',*,*,#9894,.T.);
#13753=ORIENTED_EDGE('',*,*,#9398,.F.);
#13754=ORIENTED_EDGE('',*,*,#9896,.F.);
#13755=ORIENTED_EDGE('',*,*,#9686,.F.);
#13756=ORIENTED_EDGE('',*,*,#9895,.T.);
#13757=ORIENTED_EDGE('',*,*,#9688,.F.);
#13758=ORIENTED_EDGE('',*,*,#9897,.F.);
#13759=ORIENTED_EDGE('',*,*,#9396,.F.);
#13760=ORIENTED_EDGE('',*,*,#9896,.T.);
#13761=ORIENTED_EDGE('',*,*,#9397,.F.);
#13762=ORIENTED_EDGE('',*,*,#9897,.T.);
#13763=ORIENTED_EDGE('',*,*,#9687,.F.);
#13764=ORIENTED_EDGE('',*,*,#9898,.F.);
#13765=ORIENTED_EDGE('',*,*,#9409,.F.);
#13766=ORIENTED_EDGE('',*,*,#9408,.F.);
#13767=ORIENTED_EDGE('',*,*,#9899,.F.);
#13768=ORIENTED_EDGE('',*,*,#9696,.F.);
#13769=ORIENTED_EDGE('',*,*,#9899,.T.);
#13770=ORIENTED_EDGE('',*,*,#9407,.F.);
#13771=ORIENTED_EDGE('',*,*,#9900,.F.);
#13772=ORIENTED_EDGE('',*,*,#9697,.F.);
#13773=ORIENTED_EDGE('',*,*,#9898,.T.);
#13774=ORIENTED_EDGE('',*,*,#9695,.F.);
#13775=ORIENTED_EDGE('',*,*,#9901,.F.);
#13776=ORIENTED_EDGE('',*,*,#9411,.F.);
#13777=ORIENTED_EDGE('',*,*,#9410,.F.);
#13778=ORIENTED_EDGE('',*,*,#9900,.T.);
#13779=ORIENTED_EDGE('',*,*,#9406,.F.);
#13780=ORIENTED_EDGE('',*,*,#9405,.F.);
#13781=ORIENTED_EDGE('',*,*,#9902,.F.);
#13782=ORIENTED_EDGE('',*,*,#9692,.F.);
#13783=ORIENTED_EDGE('',*,*,#9901,.T.);
#13784=ORIENTED_EDGE('',*,*,#9694,.F.);
#13785=ORIENTED_EDGE('',*,*,#9903,.F.);
#13786=ORIENTED_EDGE('',*,*,#9402,.F.);
#13787=ORIENTED_EDGE('',*,*,#9902,.T.);
#13788=ORIENTED_EDGE('',*,*,#9404,.F.);
#13789=ORIENTED_EDGE('',*,*,#9403,.F.);
#13790=ORIENTED_EDGE('',*,*,#9903,.T.);
#13791=ORIENTED_EDGE('',*,*,#9693,.F.);
#13792=ORIENTED_EDGE('',*,*,#9904,.F.);
#13793=ORIENTED_EDGE('',*,*,#9419,.F.);
#13794=ORIENTED_EDGE('',*,*,#9418,.F.);
#13795=ORIENTED_EDGE('',*,*,#9905,.F.);
#13796=ORIENTED_EDGE('',*,*,#9702,.F.);
#13797=ORIENTED_EDGE('',*,*,#9905,.T.);
#13798=ORIENTED_EDGE('',*,*,#9417,.F.);
#13799=ORIENTED_EDGE('',*,*,#9906,.F.);
#13800=ORIENTED_EDGE('',*,*,#9703,.F.);
#13801=ORIENTED_EDGE('',*,*,#9904,.T.);
#13802=ORIENTED_EDGE('',*,*,#9701,.F.);
#13803=ORIENTED_EDGE('',*,*,#9907,.F.);
#13804=ORIENTED_EDGE('',*,*,#9421,.F.);
#13805=ORIENTED_EDGE('',*,*,#9420,.F.);
#13806=ORIENTED_EDGE('',*,*,#9906,.T.);
#13807=ORIENTED_EDGE('',*,*,#9416,.F.);
#13808=ORIENTED_EDGE('',*,*,#9415,.F.);
#13809=ORIENTED_EDGE('',*,*,#9908,.F.);
#13810=ORIENTED_EDGE('',*,*,#9698,.F.);
#13811=ORIENTED_EDGE('',*,*,#9907,.T.);
#13812=ORIENTED_EDGE('',*,*,#9700,.F.);
#13813=ORIENTED_EDGE('',*,*,#9909,.F.);
#13814=ORIENTED_EDGE('',*,*,#9412,.F.);
#13815=ORIENTED_EDGE('',*,*,#9908,.T.);
#13816=ORIENTED_EDGE('',*,*,#9414,.F.);
#13817=ORIENTED_EDGE('',*,*,#9413,.F.);
#13818=ORIENTED_EDGE('',*,*,#9909,.T.);
#13819=ORIENTED_EDGE('',*,*,#9699,.F.);
#13820=ORIENTED_EDGE('',*,*,#9910,.F.);
#13821=ORIENTED_EDGE('',*,*,#9429,.F.);
#13822=ORIENTED_EDGE('',*,*,#9911,.F.);
#13823=ORIENTED_EDGE('',*,*,#9708,.F.);
#13824=ORIENTED_EDGE('',*,*,#9911,.T.);
#13825=ORIENTED_EDGE('',*,*,#9428,.F.);
#13826=ORIENTED_EDGE('',*,*,#9912,.F.);
#13827=ORIENTED_EDGE('',*,*,#9709,.F.);
#13828=ORIENTED_EDGE('',*,*,#9910,.T.);
#13829=ORIENTED_EDGE('',*,*,#9707,.F.);
#13830=ORIENTED_EDGE('',*,*,#9913,.F.);
#13831=ORIENTED_EDGE('',*,*,#9433,.F.);
#13832=ORIENTED_EDGE('',*,*,#9432,.F.);
#13833=ORIENTED_EDGE('',*,*,#9431,.F.);
#13834=ORIENTED_EDGE('',*,*,#9430,.F.);
#13835=ORIENTED_EDGE('',*,*,#9912,.T.);
#13836=ORIENTED_EDGE('',*,*,#9427,.F.);
#13837=ORIENTED_EDGE('',*,*,#9426,.F.);
#13838=ORIENTED_EDGE('',*,*,#9914,.F.);
#13839=ORIENTED_EDGE('',*,*,#9704,.F.);
#13840=ORIENTED_EDGE('',*,*,#9913,.T.);
#13841=ORIENTED_EDGE('',*,*,#9706,.F.);
#13842=ORIENTED_EDGE('',*,*,#9915,.F.);
#13843=ORIENTED_EDGE('',*,*,#9423,.F.);
#13844=ORIENTED_EDGE('',*,*,#9422,.F.);
#13845=ORIENTED_EDGE('',*,*,#9914,.T.);
#13846=ORIENTED_EDGE('',*,*,#9425,.F.);
#13847=ORIENTED_EDGE('',*,*,#9424,.F.);
#13848=ORIENTED_EDGE('',*,*,#9915,.T.);
#13849=ORIENTED_EDGE('',*,*,#9705,.F.);
#13850=ORIENTED_EDGE('',*,*,#9916,.F.);
#13851=ORIENTED_EDGE('',*,*,#9439,.F.);
#13852=ORIENTED_EDGE('',*,*,#9438,.F.);
#13853=ORIENTED_EDGE('',*,*,#9917,.F.);
#13854=ORIENTED_EDGE('',*,*,#9714,.F.);
#13855=ORIENTED_EDGE('',*,*,#9917,.T.);
#13856=ORIENTED_EDGE('',*,*,#9437,.F.);
#13857=ORIENTED_EDGE('',*,*,#9918,.F.);
#13858=ORIENTED_EDGE('',*,*,#9715,.F.);
#13859=ORIENTED_EDGE('',*,*,#9916,.T.);
#13860=ORIENTED_EDGE('',*,*,#9713,.F.);
#13861=ORIENTED_EDGE('',*,*,#9919,.F.);
#13862=ORIENTED_EDGE('',*,*,#9441,.F.);
#13863=ORIENTED_EDGE('',*,*,#9440,.F.);
#13864=ORIENTED_EDGE('',*,*,#9918,.T.);
#13865=ORIENTED_EDGE('',*,*,#9436,.F.);
#13866=ORIENTED_EDGE('',*,*,#9920,.F.);
#13867=ORIENTED_EDGE('',*,*,#9710,.F.);
#13868=ORIENTED_EDGE('',*,*,#9919,.T.);
#13869=ORIENTED_EDGE('',*,*,#9712,.F.);
#13870=ORIENTED_EDGE('',*,*,#9921,.F.);
#13871=ORIENTED_EDGE('',*,*,#9434,.F.);
#13872=ORIENTED_EDGE('',*,*,#9920,.T.);
#13873=ORIENTED_EDGE('',*,*,#9435,.F.);
#13874=ORIENTED_EDGE('',*,*,#9921,.T.);
#13875=ORIENTED_EDGE('',*,*,#9711,.F.);
#13876=ORIENTED_EDGE('',*,*,#9922,.F.);
#13877=ORIENTED_EDGE('',*,*,#9451,.F.);
#13878=ORIENTED_EDGE('',*,*,#9450,.F.);
#13879=ORIENTED_EDGE('',*,*,#9923,.F.);
#13880=ORIENTED_EDGE('',*,*,#9720,.F.);
#13881=ORIENTED_EDGE('',*,*,#9923,.T.);
#13882=ORIENTED_EDGE('',*,*,#9449,.F.);
#13883=ORIENTED_EDGE('',*,*,#9924,.F.);
#13884=ORIENTED_EDGE('',*,*,#9721,.F.);
#13885=ORIENTED_EDGE('',*,*,#9922,.T.);
#13886=ORIENTED_EDGE('',*,*,#9719,.F.);
#13887=ORIENTED_EDGE('',*,*,#9925,.F.);
#13888=ORIENTED_EDGE('',*,*,#9452,.F.);
#13889=ORIENTED_EDGE('',*,*,#9924,.T.);
#13890=ORIENTED_EDGE('',*,*,#9448,.F.);
#13891=ORIENTED_EDGE('',*,*,#9447,.F.);
#13892=ORIENTED_EDGE('',*,*,#9446,.F.);
#13893=ORIENTED_EDGE('',*,*,#9445,.F.);
#13894=ORIENTED_EDGE('',*,*,#9926,.F.);
#13895=ORIENTED_EDGE('',*,*,#9716,.F.);
#13896=ORIENTED_EDGE('',*,*,#9925,.T.);
#13897=ORIENTED_EDGE('',*,*,#9718,.F.);
#13898=ORIENTED_EDGE('',*,*,#9927,.F.);
#13899=ORIENTED_EDGE('',*,*,#9442,.F.);
#13900=ORIENTED_EDGE('',*,*,#9926,.T.);
#13901=ORIENTED_EDGE('',*,*,#9444,.F.);
#13902=ORIENTED_EDGE('',*,*,#9443,.F.);
#13903=ORIENTED_EDGE('',*,*,#9927,.T.);
#13904=ORIENTED_EDGE('',*,*,#9717,.F.);
#13905=ORIENTED_EDGE('',*,*,#9928,.F.);
#13906=ORIENTED_EDGE('',*,*,#9246,.F.);
#13907=ORIENTED_EDGE('',*,*,#9112,.F.);
#13908=ORIENTED_EDGE('',*,*,#9929,.F.);
#13909=ORIENTED_EDGE('',*,*,#9724,.T.);
#13910=ORIENTED_EDGE('',*,*,#9929,.T.);
#13911=ORIENTED_EDGE('',*,*,#9111,.F.);
#13912=ORIENTED_EDGE('',*,*,#9930,.F.);
#13913=ORIENTED_EDGE('',*,*,#9725,.T.);
#13914=ORIENTED_EDGE('',*,*,#9928,.T.);
#13915=ORIENTED_EDGE('',*,*,#9729,.T.);
#13916=ORIENTED_EDGE('',*,*,#9931,.F.);
#13917=ORIENTED_EDGE('',*,*,#9247,.F.);
#13918=ORIENTED_EDGE('',*,*,#9930,.T.);
#13919=ORIENTED_EDGE('',*,*,#9110,.F.);
#13920=ORIENTED_EDGE('',*,*,#9932,.F.);
#13921=ORIENTED_EDGE('',*,*,#9726,.T.);
#13922=ORIENTED_EDGE('',*,*,#9931,.T.);
#13923=ORIENTED_EDGE('',*,*,#9728,.T.);
#13924=ORIENTED_EDGE('',*,*,#9933,.F.);
#13925=ORIENTED_EDGE('',*,*,#9108,.F.);
#13926=ORIENTED_EDGE('',*,*,#9248,.F.);
#13927=ORIENTED_EDGE('',*,*,#9932,.T.);
#13928=ORIENTED_EDGE('',*,*,#9109,.F.);
#13929=ORIENTED_EDGE('',*,*,#9933,.T.);
#13930=ORIENTED_EDGE('',*,*,#9727,.T.);
#13931=ORIENTED_EDGE('',*,*,#9934,.F.);
#13932=ORIENTED_EDGE('',*,*,#9249,.F.);
#13933=ORIENTED_EDGE('',*,*,#9106,.F.);
#13934=ORIENTED_EDGE('',*,*,#9935,.F.);
#13935=ORIENTED_EDGE('',*,*,#9730,.T.);
#13936=ORIENTED_EDGE('',*,*,#9935,.T.);
#13937=ORIENTED_EDGE('',*,*,#9105,.F.);
#13938=ORIENTED_EDGE('',*,*,#9936,.F.);
#13939=ORIENTED_EDGE('',*,*,#9731,.T.);
#13940=ORIENTED_EDGE('',*,*,#9934,.T.);
#13941=ORIENTED_EDGE('',*,*,#9735,.T.);
#13942=ORIENTED_EDGE('',*,*,#9937,.F.);
#13943=ORIENTED_EDGE('',*,*,#9250,.F.);
#13944=ORIENTED_EDGE('',*,*,#9936,.T.);
#13945=ORIENTED_EDGE('',*,*,#9104,.F.);
#13946=ORIENTED_EDGE('',*,*,#9938,.F.);
#13947=ORIENTED_EDGE('',*,*,#9732,.T.);
#13948=ORIENTED_EDGE('',*,*,#9937,.T.);
#13949=ORIENTED_EDGE('',*,*,#9734,.T.);
#13950=ORIENTED_EDGE('',*,*,#9939,.F.);
#13951=ORIENTED_EDGE('',*,*,#9102,.F.);
#13952=ORIENTED_EDGE('',*,*,#9251,.F.);
#13953=ORIENTED_EDGE('',*,*,#9938,.T.);
#13954=ORIENTED_EDGE('',*,*,#9103,.F.);
#13955=ORIENTED_EDGE('',*,*,#9939,.T.);
#13956=ORIENTED_EDGE('',*,*,#9733,.T.);
#13957=ORIENTED_EDGE('',*,*,#9940,.F.);
#13958=ORIENTED_EDGE('',*,*,#9252,.F.);
#13959=ORIENTED_EDGE('',*,*,#9100,.F.);
#13960=ORIENTED_EDGE('',*,*,#9941,.F.);
#13961=ORIENTED_EDGE('',*,*,#9736,.T.);
#13962=ORIENTED_EDGE('',*,*,#9941,.T.);
#13963=ORIENTED_EDGE('',*,*,#9099,.F.);
#13964=ORIENTED_EDGE('',*,*,#9942,.F.);
#13965=ORIENTED_EDGE('',*,*,#9737,.T.);
#13966=ORIENTED_EDGE('',*,*,#9940,.T.);
#13967=ORIENTED_EDGE('',*,*,#9741,.T.);
#13968=ORIENTED_EDGE('',*,*,#9943,.F.);
#13969=ORIENTED_EDGE('',*,*,#9253,.F.);
#13970=ORIENTED_EDGE('',*,*,#9942,.T.);
#13971=ORIENTED_EDGE('',*,*,#9098,.F.);
#13972=ORIENTED_EDGE('',*,*,#9944,.F.);
#13973=ORIENTED_EDGE('',*,*,#9738,.T.);
#13974=ORIENTED_EDGE('',*,*,#9943,.T.);
#13975=ORIENTED_EDGE('',*,*,#9740,.T.);
#13976=ORIENTED_EDGE('',*,*,#9945,.F.);
#13977=ORIENTED_EDGE('',*,*,#9096,.F.);
#13978=ORIENTED_EDGE('',*,*,#9254,.F.);
#13979=ORIENTED_EDGE('',*,*,#9944,.T.);
#13980=ORIENTED_EDGE('',*,*,#9097,.F.);
#13981=ORIENTED_EDGE('',*,*,#9945,.T.);
#13982=ORIENTED_EDGE('',*,*,#9739,.T.);
#13983=ORIENTED_EDGE('',*,*,#9946,.F.);
#13984=ORIENTED_EDGE('',*,*,#9255,.F.);
#13985=ORIENTED_EDGE('',*,*,#9094,.F.);
#13986=ORIENTED_EDGE('',*,*,#9947,.F.);
#13987=ORIENTED_EDGE('',*,*,#9742,.T.);
#13988=ORIENTED_EDGE('',*,*,#9947,.T.);
#13989=ORIENTED_EDGE('',*,*,#9093,.F.);
#13990=ORIENTED_EDGE('',*,*,#9948,.F.);
#13991=ORIENTED_EDGE('',*,*,#9743,.T.);
#13992=ORIENTED_EDGE('',*,*,#9946,.T.);
#13993=ORIENTED_EDGE('',*,*,#9747,.T.);
#13994=ORIENTED_EDGE('',*,*,#9949,.F.);
#13995=ORIENTED_EDGE('',*,*,#9256,.F.);
#13996=ORIENTED_EDGE('',*,*,#9948,.T.);
#13997=ORIENTED_EDGE('',*,*,#9092,.F.);
#13998=ORIENTED_EDGE('',*,*,#9950,.F.);
#13999=ORIENTED_EDGE('',*,*,#9744,.T.);
#14000=ORIENTED_EDGE('',*,*,#9949,.T.);
#14001=ORIENTED_EDGE('',*,*,#9746,.T.);
#14002=ORIENTED_EDGE('',*,*,#9951,.F.);
#14003=ORIENTED_EDGE('',*,*,#9090,.F.);
#14004=ORIENTED_EDGE('',*,*,#9257,.F.);
#14005=ORIENTED_EDGE('',*,*,#9950,.T.);
#14006=ORIENTED_EDGE('',*,*,#9091,.F.);
#14007=ORIENTED_EDGE('',*,*,#9951,.T.);
#14008=ORIENTED_EDGE('',*,*,#9745,.T.);
#14009=ORIENTED_EDGE('',*,*,#9952,.F.);
#14010=ORIENTED_EDGE('',*,*,#9231,.F.);
#14011=ORIENTED_EDGE('',*,*,#9142,.F.);
#14012=ORIENTED_EDGE('',*,*,#9953,.F.);
#14013=ORIENTED_EDGE('',*,*,#9748,.T.);
#14014=ORIENTED_EDGE('',*,*,#9953,.T.);
#14015=ORIENTED_EDGE('',*,*,#9141,.F.);
#14016=ORIENTED_EDGE('',*,*,#9954,.F.);
#14017=ORIENTED_EDGE('',*,*,#9749,.T.);
#14018=ORIENTED_EDGE('',*,*,#9952,.T.);
#14019=ORIENTED_EDGE('',*,*,#9753,.T.);
#14020=ORIENTED_EDGE('',*,*,#9955,.F.);
#14021=ORIENTED_EDGE('',*,*,#9232,.F.);
#14022=ORIENTED_EDGE('',*,*,#9954,.T.);
#14023=ORIENTED_EDGE('',*,*,#9140,.F.);
#14024=ORIENTED_EDGE('',*,*,#9956,.F.);
#14025=ORIENTED_EDGE('',*,*,#9750,.T.);
#14026=ORIENTED_EDGE('',*,*,#9955,.T.);
#14027=ORIENTED_EDGE('',*,*,#9752,.T.);
#14028=ORIENTED_EDGE('',*,*,#9957,.F.);
#14029=ORIENTED_EDGE('',*,*,#9138,.F.);
#14030=ORIENTED_EDGE('',*,*,#9233,.F.);
#14031=ORIENTED_EDGE('',*,*,#9956,.T.);
#14032=ORIENTED_EDGE('',*,*,#9139,.F.);
#14033=ORIENTED_EDGE('',*,*,#9957,.T.);
#14034=ORIENTED_EDGE('',*,*,#9751,.T.);
#14035=ORIENTED_EDGE('',*,*,#9958,.F.);
#14036=ORIENTED_EDGE('',*,*,#9261,.F.);
#14037=ORIENTED_EDGE('',*,*,#9082,.F.);
#14038=ORIENTED_EDGE('',*,*,#9959,.F.);
#14039=ORIENTED_EDGE('',*,*,#9754,.T.);
#14040=ORIENTED_EDGE('',*,*,#9959,.T.);
#14041=ORIENTED_EDGE('',*,*,#9081,.F.);
#14042=ORIENTED_EDGE('',*,*,#9960,.F.);
#14043=ORIENTED_EDGE('',*,*,#9755,.T.);
#14044=ORIENTED_EDGE('',*,*,#9958,.T.);
#14045=ORIENTED_EDGE('',*,*,#9759,.T.);
#14046=ORIENTED_EDGE('',*,*,#9961,.F.);
#14047=ORIENTED_EDGE('',*,*,#9262,.F.);
#14048=ORIENTED_EDGE('',*,*,#9960,.T.);
#14049=ORIENTED_EDGE('',*,*,#9080,.F.);
#14050=ORIENTED_EDGE('',*,*,#9962,.F.);
#14051=ORIENTED_EDGE('',*,*,#9756,.T.);
#14052=ORIENTED_EDGE('',*,*,#9961,.T.);
#14053=ORIENTED_EDGE('',*,*,#9758,.T.);
#14054=ORIENTED_EDGE('',*,*,#9963,.F.);
#14055=ORIENTED_EDGE('',*,*,#9078,.F.);
#14056=ORIENTED_EDGE('',*,*,#9263,.F.);
#14057=ORIENTED_EDGE('',*,*,#9962,.T.);
#14058=ORIENTED_EDGE('',*,*,#9079,.F.);
#14059=ORIENTED_EDGE('',*,*,#9963,.T.);
#14060=ORIENTED_EDGE('',*,*,#9757,.T.);
#14061=ORIENTED_EDGE('',*,*,#9964,.F.);
#14062=ORIENTED_EDGE('',*,*,#9284,.F.);
#14063=ORIENTED_EDGE('',*,*,#9283,.F.);
#14064=ORIENTED_EDGE('',*,*,#9042,.F.);
#14065=ORIENTED_EDGE('',*,*,#9965,.F.);
#14066=ORIENTED_EDGE('',*,*,#9760,.T.);
#14067=ORIENTED_EDGE('',*,*,#9965,.T.);
#14068=ORIENTED_EDGE('',*,*,#9041,.F.);
#14069=ORIENTED_EDGE('',*,*,#9040,.F.);
#14070=ORIENTED_EDGE('',*,*,#9966,.F.);
#14071=ORIENTED_EDGE('',*,*,#9761,.T.);
#14072=ORIENTED_EDGE('',*,*,#9964,.T.);
#14073=ORIENTED_EDGE('',*,*,#9765,.T.);
#14074=ORIENTED_EDGE('',*,*,#9967,.F.);
#14075=ORIENTED_EDGE('',*,*,#9285,.F.);
#14076=ORIENTED_EDGE('',*,*,#9966,.T.);
#14077=ORIENTED_EDGE('',*,*,#9039,.F.);
#14078=ORIENTED_EDGE('',*,*,#9968,.F.);
#14079=ORIENTED_EDGE('',*,*,#9762,.T.);
#14080=ORIENTED_EDGE('',*,*,#9967,.T.);
#14081=ORIENTED_EDGE('',*,*,#9764,.T.);
#14082=ORIENTED_EDGE('',*,*,#9969,.F.);
#14083=ORIENTED_EDGE('',*,*,#9036,.F.);
#14084=ORIENTED_EDGE('',*,*,#9287,.F.);
#14085=ORIENTED_EDGE('',*,*,#9286,.F.);
#14086=ORIENTED_EDGE('',*,*,#9968,.T.);
#14087=ORIENTED_EDGE('',*,*,#9038,.F.);
#14088=ORIENTED_EDGE('',*,*,#9037,.F.);
#14089=ORIENTED_EDGE('',*,*,#9969,.T.);
#14090=ORIENTED_EDGE('',*,*,#9763,.T.);
#14091=ORIENTED_EDGE('',*,*,#9970,.F.);
#14092=ORIENTED_EDGE('',*,*,#9258,.F.);
#14093=ORIENTED_EDGE('',*,*,#9088,.F.);
#14094=ORIENTED_EDGE('',*,*,#9971,.F.);
#14095=ORIENTED_EDGE('',*,*,#9766,.T.);
#14096=ORIENTED_EDGE('',*,*,#9971,.T.);
#14097=ORIENTED_EDGE('',*,*,#9087,.F.);
#14098=ORIENTED_EDGE('',*,*,#9972,.F.);
#14099=ORIENTED_EDGE('',*,*,#9767,.T.);
#14100=ORIENTED_EDGE('',*,*,#9970,.T.);
#14101=ORIENTED_EDGE('',*,*,#9771,.T.);
#14102=ORIENTED_EDGE('',*,*,#9973,.F.);
#14103=ORIENTED_EDGE('',*,*,#9259,.F.);
#14104=ORIENTED_EDGE('',*,*,#9972,.T.);
#14105=ORIENTED_EDGE('',*,*,#9086,.F.);
#14106=ORIENTED_EDGE('',*,*,#9974,.F.);
#14107=ORIENTED_EDGE('',*,*,#9768,.T.);
#14108=ORIENTED_EDGE('',*,*,#9973,.T.);
#14109=ORIENTED_EDGE('',*,*,#9770,.T.);
#14110=ORIENTED_EDGE('',*,*,#9975,.F.);
#14111=ORIENTED_EDGE('',*,*,#9084,.F.);
#14112=ORIENTED_EDGE('',*,*,#9260,.F.);
#14113=ORIENTED_EDGE('',*,*,#9974,.T.);
#14114=ORIENTED_EDGE('',*,*,#9085,.F.);
#14115=ORIENTED_EDGE('',*,*,#9975,.T.);
#14116=ORIENTED_EDGE('',*,*,#9769,.T.);
#14117=ORIENTED_EDGE('',*,*,#9976,.F.);
#14118=ORIENTED_EDGE('',*,*,#9243,.F.);
#14119=ORIENTED_EDGE('',*,*,#9118,.F.);
#14120=ORIENTED_EDGE('',*,*,#9977,.F.);
#14121=ORIENTED_EDGE('',*,*,#9772,.T.);
#14122=ORIENTED_EDGE('',*,*,#9977,.T.);
#14123=ORIENTED_EDGE('',*,*,#9117,.F.);
#14124=ORIENTED_EDGE('',*,*,#9978,.F.);
#14125=ORIENTED_EDGE('',*,*,#9773,.T.);
#14126=ORIENTED_EDGE('',*,*,#9976,.T.);
#14127=ORIENTED_EDGE('',*,*,#9777,.T.);
#14128=ORIENTED_EDGE('',*,*,#9979,.F.);
#14129=ORIENTED_EDGE('',*,*,#9244,.F.);
#14130=ORIENTED_EDGE('',*,*,#9978,.T.);
#14131=ORIENTED_EDGE('',*,*,#9116,.F.);
#14132=ORIENTED_EDGE('',*,*,#9980,.F.);
#14133=ORIENTED_EDGE('',*,*,#9774,.T.);
#14134=ORIENTED_EDGE('',*,*,#9979,.T.);
#14135=ORIENTED_EDGE('',*,*,#9776,.T.);
#14136=ORIENTED_EDGE('',*,*,#9981,.F.);
#14137=ORIENTED_EDGE('',*,*,#9114,.F.);
#14138=ORIENTED_EDGE('',*,*,#9245,.F.);
#14139=ORIENTED_EDGE('',*,*,#9980,.T.);
#14140=ORIENTED_EDGE('',*,*,#9115,.F.);
#14141=ORIENTED_EDGE('',*,*,#9981,.T.);
#14142=ORIENTED_EDGE('',*,*,#9775,.T.);
#14143=ORIENTED_EDGE('',*,*,#9982,.F.);
#14144=ORIENTED_EDGE('',*,*,#9240,.F.);
#14145=ORIENTED_EDGE('',*,*,#9124,.F.);
#14146=ORIENTED_EDGE('',*,*,#9983,.F.);
#14147=ORIENTED_EDGE('',*,*,#9778,.T.);
#14148=ORIENTED_EDGE('',*,*,#9983,.T.);
#14149=ORIENTED_EDGE('',*,*,#9123,.F.);
#14150=ORIENTED_EDGE('',*,*,#9984,.F.);
#14151=ORIENTED_EDGE('',*,*,#9779,.T.);
#14152=ORIENTED_EDGE('',*,*,#9982,.T.);
#14153=ORIENTED_EDGE('',*,*,#9783,.T.);
#14154=ORIENTED_EDGE('',*,*,#9985,.F.);
#14155=ORIENTED_EDGE('',*,*,#9241,.F.);
#14156=ORIENTED_EDGE('',*,*,#9984,.T.);
#14157=ORIENTED_EDGE('',*,*,#9122,.F.);
#14158=ORIENTED_EDGE('',*,*,#9986,.F.);
#14159=ORIENTED_EDGE('',*,*,#9780,.T.);
#14160=ORIENTED_EDGE('',*,*,#9985,.T.);
#14161=ORIENTED_EDGE('',*,*,#9782,.T.);
#14162=ORIENTED_EDGE('',*,*,#9987,.F.);
#14163=ORIENTED_EDGE('',*,*,#9120,.F.);
#14164=ORIENTED_EDGE('',*,*,#9242,.F.);
#14165=ORIENTED_EDGE('',*,*,#9986,.T.);
#14166=ORIENTED_EDGE('',*,*,#9121,.F.);
#14167=ORIENTED_EDGE('',*,*,#9987,.T.);
#14168=ORIENTED_EDGE('',*,*,#9781,.T.);
#14169=ORIENTED_EDGE('',*,*,#9988,.F.);
#14170=ORIENTED_EDGE('',*,*,#9237,.F.);
#14171=ORIENTED_EDGE('',*,*,#9130,.F.);
#14172=ORIENTED_EDGE('',*,*,#9989,.F.);
#14173=ORIENTED_EDGE('',*,*,#9784,.T.);
#14174=ORIENTED_EDGE('',*,*,#9989,.T.);
#14175=ORIENTED_EDGE('',*,*,#9129,.F.);
#14176=ORIENTED_EDGE('',*,*,#9990,.F.);
#14177=ORIENTED_EDGE('',*,*,#9785,.T.);
#14178=ORIENTED_EDGE('',*,*,#9988,.T.);
#14179=ORIENTED_EDGE('',*,*,#9789,.T.);
#14180=ORIENTED_EDGE('',*,*,#9991,.F.);
#14181=ORIENTED_EDGE('',*,*,#9238,.F.);
#14182=ORIENTED_EDGE('',*,*,#9990,.T.);
#14183=ORIENTED_EDGE('',*,*,#9128,.F.);
#14184=ORIENTED_EDGE('',*,*,#9992,.F.);
#14185=ORIENTED_EDGE('',*,*,#9786,.T.);
#14186=ORIENTED_EDGE('',*,*,#9991,.T.);
#14187=ORIENTED_EDGE('',*,*,#9788,.T.);
#14188=ORIENTED_EDGE('',*,*,#9993,.F.);
#14189=ORIENTED_EDGE('',*,*,#9126,.F.);
#14190=ORIENTED_EDGE('',*,*,#9239,.F.);
#14191=ORIENTED_EDGE('',*,*,#9992,.T.);
#14192=ORIENTED_EDGE('',*,*,#9127,.F.);
#14193=ORIENTED_EDGE('',*,*,#9993,.T.);
#14194=ORIENTED_EDGE('',*,*,#9787,.T.);
#14195=ORIENTED_EDGE('',*,*,#9994,.F.);
#14196=ORIENTED_EDGE('',*,*,#9234,.F.);
#14197=ORIENTED_EDGE('',*,*,#9136,.F.);
#14198=ORIENTED_EDGE('',*,*,#9995,.F.);
#14199=ORIENTED_EDGE('',*,*,#9790,.T.);
#14200=ORIENTED_EDGE('',*,*,#9995,.T.);
#14201=ORIENTED_EDGE('',*,*,#9135,.F.);
#14202=ORIENTED_EDGE('',*,*,#9996,.F.);
#14203=ORIENTED_EDGE('',*,*,#9791,.T.);
#14204=ORIENTED_EDGE('',*,*,#9994,.T.);
#14205=ORIENTED_EDGE('',*,*,#9795,.T.);
#14206=ORIENTED_EDGE('',*,*,#9997,.F.);
#14207=ORIENTED_EDGE('',*,*,#9235,.F.);
#14208=ORIENTED_EDGE('',*,*,#9996,.T.);
#14209=ORIENTED_EDGE('',*,*,#9134,.F.);
#14210=ORIENTED_EDGE('',*,*,#9998,.F.);
#14211=ORIENTED_EDGE('',*,*,#9792,.T.);
#14212=ORIENTED_EDGE('',*,*,#9997,.T.);
#14213=ORIENTED_EDGE('',*,*,#9794,.T.);
#14214=ORIENTED_EDGE('',*,*,#9999,.F.);
#14215=ORIENTED_EDGE('',*,*,#9132,.F.);
#14216=ORIENTED_EDGE('',*,*,#9236,.F.);
#14217=ORIENTED_EDGE('',*,*,#9998,.T.);
#14218=ORIENTED_EDGE('',*,*,#9133,.F.);
#14219=ORIENTED_EDGE('',*,*,#9999,.T.);
#14220=ORIENTED_EDGE('',*,*,#9793,.T.);
#14221=ORIENTED_EDGE('',*,*,#10000,.F.);
#14222=ORIENTED_EDGE('',*,*,#9279,.F.);
#14223=ORIENTED_EDGE('',*,*,#9278,.F.);
#14224=ORIENTED_EDGE('',*,*,#9050,.F.);
#14225=ORIENTED_EDGE('',*,*,#10001,.F.);
#14226=ORIENTED_EDGE('',*,*,#9796,.T.);
#14227=ORIENTED_EDGE('',*,*,#10001,.T.);
#14228=ORIENTED_EDGE('',*,*,#9049,.F.);
#14229=ORIENTED_EDGE('',*,*,#9048,.F.);
#14230=ORIENTED_EDGE('',*,*,#10002,.F.);
#14231=ORIENTED_EDGE('',*,*,#9797,.T.);
#14232=ORIENTED_EDGE('',*,*,#10000,.T.);
#14233=ORIENTED_EDGE('',*,*,#9801,.T.);
#14234=ORIENTED_EDGE('',*,*,#10003,.F.);
#14235=ORIENTED_EDGE('',*,*,#9280,.F.);
#14236=ORIENTED_EDGE('',*,*,#10002,.T.);
#14237=ORIENTED_EDGE('',*,*,#9047,.F.);
#14238=ORIENTED_EDGE('',*,*,#10004,.F.);
#14239=ORIENTED_EDGE('',*,*,#9798,.T.);
#14240=ORIENTED_EDGE('',*,*,#10003,.T.);
#14241=ORIENTED_EDGE('',*,*,#9800,.T.);
#14242=ORIENTED_EDGE('',*,*,#10005,.F.);
#14243=ORIENTED_EDGE('',*,*,#9044,.F.);
#14244=ORIENTED_EDGE('',*,*,#9282,.F.);
#14245=ORIENTED_EDGE('',*,*,#9281,.F.);
#14246=ORIENTED_EDGE('',*,*,#10004,.T.);
#14247=ORIENTED_EDGE('',*,*,#9046,.F.);
#14248=ORIENTED_EDGE('',*,*,#9045,.F.);
#14249=ORIENTED_EDGE('',*,*,#10005,.T.);
#14250=ORIENTED_EDGE('',*,*,#9799,.T.);
#14251=ORIENTED_EDGE('',*,*,#10006,.F.);
#14252=ORIENTED_EDGE('',*,*,#9274,.F.);
#14253=ORIENTED_EDGE('',*,*,#9273,.F.);
#14254=ORIENTED_EDGE('',*,*,#9058,.F.);
#14255=ORIENTED_EDGE('',*,*,#10007,.F.);
#14256=ORIENTED_EDGE('',*,*,#9802,.T.);
#14257=ORIENTED_EDGE('',*,*,#10007,.T.);
#14258=ORIENTED_EDGE('',*,*,#9057,.F.);
#14259=ORIENTED_EDGE('',*,*,#9056,.F.);
#14260=ORIENTED_EDGE('',*,*,#10008,.F.);
#14261=ORIENTED_EDGE('',*,*,#9803,.T.);
#14262=ORIENTED_EDGE('',*,*,#10006,.T.);
#14263=ORIENTED_EDGE('',*,*,#9807,.T.);
#14264=ORIENTED_EDGE('',*,*,#10009,.F.);
#14265=ORIENTED_EDGE('',*,*,#9275,.F.);
#14266=ORIENTED_EDGE('',*,*,#10008,.T.);
#14267=ORIENTED_EDGE('',*,*,#9055,.F.);
#14268=ORIENTED_EDGE('',*,*,#10010,.F.);
#14269=ORIENTED_EDGE('',*,*,#9804,.T.);
#14270=ORIENTED_EDGE('',*,*,#10009,.T.);
#14271=ORIENTED_EDGE('',*,*,#9806,.T.);
#14272=ORIENTED_EDGE('',*,*,#10011,.F.);
#14273=ORIENTED_EDGE('',*,*,#9052,.F.);
#14274=ORIENTED_EDGE('',*,*,#9277,.F.);
#14275=ORIENTED_EDGE('',*,*,#9276,.F.);
#14276=ORIENTED_EDGE('',*,*,#10010,.T.);
#14277=ORIENTED_EDGE('',*,*,#9054,.F.);
#14278=ORIENTED_EDGE('',*,*,#9053,.F.);
#14279=ORIENTED_EDGE('',*,*,#10011,.T.);
#14280=ORIENTED_EDGE('',*,*,#9805,.T.);
#14281=ORIENTED_EDGE('',*,*,#10012,.F.);
#14282=ORIENTED_EDGE('',*,*,#9269,.F.);
#14283=ORIENTED_EDGE('',*,*,#9268,.F.);
#14284=ORIENTED_EDGE('',*,*,#9069,.F.);
#14285=ORIENTED_EDGE('',*,*,#10013,.F.);
#14286=ORIENTED_EDGE('',*,*,#9808,.T.);
#14287=ORIENTED_EDGE('',*,*,#10013,.T.);
#14288=ORIENTED_EDGE('',*,*,#9068,.F.);
#14289=ORIENTED_EDGE('',*,*,#9067,.F.);
#14290=ORIENTED_EDGE('',*,*,#10014,.F.);
#14291=ORIENTED_EDGE('',*,*,#9809,.T.);
#14292=ORIENTED_EDGE('',*,*,#10012,.T.);
#14293=ORIENTED_EDGE('',*,*,#9813,.T.);
#14294=ORIENTED_EDGE('',*,*,#10015,.F.);
#14295=ORIENTED_EDGE('',*,*,#9271,.F.);
#14296=ORIENTED_EDGE('',*,*,#9270,.F.);
#14297=ORIENTED_EDGE('',*,*,#10014,.T.);
#14298=ORIENTED_EDGE('',*,*,#9066,.F.);
#14299=ORIENTED_EDGE('',*,*,#9065,.F.);
#14300=ORIENTED_EDGE('',*,*,#10016,.F.);
#14301=ORIENTED_EDGE('',*,*,#9810,.T.);
#14302=ORIENTED_EDGE('',*,*,#10015,.T.);
#14303=ORIENTED_EDGE('',*,*,#9812,.T.);
#14304=ORIENTED_EDGE('',*,*,#10017,.F.);
#14305=ORIENTED_EDGE('',*,*,#9060,.F.);
#14306=ORIENTED_EDGE('',*,*,#9272,.F.);
#14307=ORIENTED_EDGE('',*,*,#10016,.T.);
#14308=ORIENTED_EDGE('',*,*,#9064,.F.);
#14309=ORIENTED_EDGE('',*,*,#9063,.F.);
#14310=ORIENTED_EDGE('',*,*,#9062,.F.);
#14311=ORIENTED_EDGE('',*,*,#9061,.F.);
#14312=ORIENTED_EDGE('',*,*,#10017,.T.);
#14313=ORIENTED_EDGE('',*,*,#9811,.T.);
#14314=ORIENTED_EDGE('',*,*,#10018,.F.);
#14315=ORIENTED_EDGE('',*,*,#9264,.F.);
#14316=ORIENTED_EDGE('',*,*,#9076,.F.);
#14317=ORIENTED_EDGE('',*,*,#10019,.F.);
#14318=ORIENTED_EDGE('',*,*,#9814,.T.);
#14319=ORIENTED_EDGE('',*,*,#10019,.T.);
#14320=ORIENTED_EDGE('',*,*,#9075,.F.);
#14321=ORIENTED_EDGE('',*,*,#10020,.F.);
#14322=ORIENTED_EDGE('',*,*,#9815,.T.);
#14323=ORIENTED_EDGE('',*,*,#10018,.T.);
#14324=ORIENTED_EDGE('',*,*,#9819,.T.);
#14325=ORIENTED_EDGE('',*,*,#10021,.F.);
#14326=ORIENTED_EDGE('',*,*,#9265,.F.);
#14327=ORIENTED_EDGE('',*,*,#10020,.T.);
#14328=ORIENTED_EDGE('',*,*,#9074,.F.);
#14329=ORIENTED_EDGE('',*,*,#10022,.F.);
#14330=ORIENTED_EDGE('',*,*,#9816,.T.);
#14331=ORIENTED_EDGE('',*,*,#10021,.T.);
#14332=ORIENTED_EDGE('',*,*,#9818,.T.);
#14333=ORIENTED_EDGE('',*,*,#10023,.F.);
#14334=ORIENTED_EDGE('',*,*,#9071,.F.);
#14335=ORIENTED_EDGE('',*,*,#9267,.F.);
#14336=ORIENTED_EDGE('',*,*,#9266,.F.);
#14337=ORIENTED_EDGE('',*,*,#10022,.T.);
#14338=ORIENTED_EDGE('',*,*,#9073,.F.);
#14339=ORIENTED_EDGE('',*,*,#9072,.F.);
#14340=ORIENTED_EDGE('',*,*,#10023,.T.);
#14341=ORIENTED_EDGE('',*,*,#9817,.T.);
#14342=ORIENTED_EDGE('',*,*,#10024,.F.);
#14343=ORIENTED_EDGE('',*,*,#9148,.F.);
#14344=ORIENTED_EDGE('',*,*,#9147,.F.);
#14345=ORIENTED_EDGE('',*,*,#10025,.F.);
#14346=ORIENTED_EDGE('',*,*,#9820,.T.);
#14347=ORIENTED_EDGE('',*,*,#10025,.T.);
#14348=ORIENTED_EDGE('',*,*,#9146,.F.);
#14349=ORIENTED_EDGE('',*,*,#10026,.F.);
#14350=ORIENTED_EDGE('',*,*,#9821,.T.);
#14351=ORIENTED_EDGE('',*,*,#10024,.T.);
#14352=ORIENTED_EDGE('',*,*,#9825,.T.);
#14353=ORIENTED_EDGE('',*,*,#10027,.F.);
#14354=ORIENTED_EDGE('',*,*,#9149,.F.);
#14355=ORIENTED_EDGE('',*,*,#10026,.T.);
#14356=ORIENTED_EDGE('',*,*,#9145,.F.);
#14357=ORIENTED_EDGE('',*,*,#9144,.F.);
#14358=ORIENTED_EDGE('',*,*,#9230,.F.);
#14359=ORIENTED_EDGE('',*,*,#9229,.F.);
#14360=ORIENTED_EDGE('',*,*,#9228,.F.);
#14361=ORIENTED_EDGE('',*,*,#10028,.F.);
#14362=ORIENTED_EDGE('',*,*,#9822,.T.);
#14363=ORIENTED_EDGE('',*,*,#10027,.T.);
#14364=ORIENTED_EDGE('',*,*,#9824,.T.);
#14365=ORIENTED_EDGE('',*,*,#10029,.F.);
#14366=ORIENTED_EDGE('',*,*,#9225,.F.);
#14367=ORIENTED_EDGE('',*,*,#9150,.F.);
#14368=ORIENTED_EDGE('',*,*,#10028,.T.);
#14369=ORIENTED_EDGE('',*,*,#9227,.F.);
#14370=ORIENTED_EDGE('',*,*,#9226,.F.);
#14371=ORIENTED_EDGE('',*,*,#10029,.T.);
#14372=ORIENTED_EDGE('',*,*,#9823,.T.);
#14373=ORIENTED_EDGE('',*,*,#10030,.F.);
#14374=ORIENTED_EDGE('',*,*,#9310,.F.);
#14375=ORIENTED_EDGE('',*,*,#9309,.F.);
#14376=ORIENTED_EDGE('',*,*,#10031,.F.);
#14377=ORIENTED_EDGE('',*,*,#9172,.T.);
#14378=ORIENTED_EDGE('',*,*,#10031,.T.);
#14379=ORIENTED_EDGE('',*,*,#9308,.F.);
#14380=ORIENTED_EDGE('',*,*,#10032,.F.);
#14381=ORIENTED_EDGE('',*,*,#9173,.F.);
#14382=ORIENTED_EDGE('',*,*,#10030,.T.);
#14383=ORIENTED_EDGE('',*,*,#9171,.T.);
#14384=ORIENTED_EDGE('',*,*,#10033,.F.);
#14385=ORIENTED_EDGE('',*,*,#9312,.F.);
#14386=ORIENTED_EDGE('',*,*,#9311,.F.);
#14387=ORIENTED_EDGE('',*,*,#10032,.T.);
#14388=ORIENTED_EDGE('',*,*,#9307,.F.);
#14389=ORIENTED_EDGE('',*,*,#10034,.F.);
#14390=ORIENTED_EDGE('',*,*,#9174,.F.);
#14391=ORIENTED_EDGE('',*,*,#10033,.T.);
#14392=ORIENTED_EDGE('',*,*,#9170,.F.);
#14393=ORIENTED_EDGE('',*,*,#10035,.F.);
#14394=ORIENTED_EDGE('',*,*,#9314,.F.);
#14395=ORIENTED_EDGE('',*,*,#9313,.F.);
#14396=ORIENTED_EDGE('',*,*,#10034,.T.);
#14397=ORIENTED_EDGE('',*,*,#9306,.F.);
#14398=ORIENTED_EDGE('',*,*,#10036,.F.);
#14399=ORIENTED_EDGE('',*,*,#9175,.F.);
#14400=ORIENTED_EDGE('',*,*,#10035,.T.);
#14401=ORIENTED_EDGE('',*,*,#9169,.F.);
#14402=ORIENTED_EDGE('',*,*,#10037,.F.);
#14403=ORIENTED_EDGE('',*,*,#9316,.F.);
#14404=ORIENTED_EDGE('',*,*,#9315,.F.);
#14405=ORIENTED_EDGE('',*,*,#10036,.T.);
#14406=ORIENTED_EDGE('',*,*,#9305,.F.);
#14407=ORIENTED_EDGE('',*,*,#10038,.F.);
#14408=ORIENTED_EDGE('',*,*,#9176,.T.);
#14409=ORIENTED_EDGE('',*,*,#10037,.T.);
#14410=ORIENTED_EDGE('',*,*,#9619,.F.);
#14411=ORIENTED_EDGE('',*,*,#10039,.F.);
#14412=ORIENTED_EDGE('',*,*,#9317,.F.);
#14413=ORIENTED_EDGE('',*,*,#10038,.T.);
#14414=ORIENTED_EDGE('',*,*,#9304,.F.);
#14415=ORIENTED_EDGE('',*,*,#9303,.F.);
#14416=ORIENTED_EDGE('',*,*,#9302,.F.);
#14417=ORIENTED_EDGE('',*,*,#10040,.F.);
#14418=ORIENTED_EDGE('',*,*,#9177,.T.);
#14419=ORIENTED_EDGE('',*,*,#10039,.T.);
#14420=ORIENTED_EDGE('',*,*,#9618,.F.);
#14421=ORIENTED_EDGE('',*,*,#10041,.F.);
#14422=ORIENTED_EDGE('',*,*,#9318,.F.);
#14423=ORIENTED_EDGE('',*,*,#10040,.T.);
#14424=ORIENTED_EDGE('',*,*,#9301,.F.);
#14425=ORIENTED_EDGE('',*,*,#10042,.F.);
#14426=ORIENTED_EDGE('',*,*,#9178,.F.);
#14427=ORIENTED_EDGE('',*,*,#10041,.T.);
#14428=ORIENTED_EDGE('',*,*,#9617,.F.);
#14429=ORIENTED_EDGE('',*,*,#10043,.F.);
#14430=ORIENTED_EDGE('',*,*,#9319,.F.);
#14431=ORIENTED_EDGE('',*,*,#10042,.T.);
#14432=ORIENTED_EDGE('',*,*,#9300,.F.);
#14433=ORIENTED_EDGE('',*,*,#10044,.F.);
#14434=ORIENTED_EDGE('',*,*,#9179,.F.);
#14435=ORIENTED_EDGE('',*,*,#10043,.T.);
#14436=ORIENTED_EDGE('',*,*,#9616,.F.);
#14437=ORIENTED_EDGE('',*,*,#10045,.F.);
#14438=ORIENTED_EDGE('',*,*,#9320,.F.);
#14439=ORIENTED_EDGE('',*,*,#10044,.T.);
#14440=ORIENTED_EDGE('',*,*,#9299,.F.);
#14441=ORIENTED_EDGE('',*,*,#9298,.F.);
#14442=ORIENTED_EDGE('',*,*,#9297,.F.);
#14443=ORIENTED_EDGE('',*,*,#10046,.F.);
#14444=ORIENTED_EDGE('',*,*,#9180,.T.);
#14445=ORIENTED_EDGE('',*,*,#10045,.T.);
#14446=ORIENTED_EDGE('',*,*,#9615,.F.);
#14447=ORIENTED_EDGE('',*,*,#10047,.F.);
#14448=ORIENTED_EDGE('',*,*,#9321,.F.);
#14449=ORIENTED_EDGE('',*,*,#10046,.T.);
#14450=ORIENTED_EDGE('',*,*,#9296,.F.);
#14451=ORIENTED_EDGE('',*,*,#10048,.F.);
#14452=ORIENTED_EDGE('',*,*,#9181,.T.);
#14453=ORIENTED_EDGE('',*,*,#10047,.T.);
#14454=ORIENTED_EDGE('',*,*,#9614,.F.);
#14455=ORIENTED_EDGE('',*,*,#10049,.F.);
#14456=ORIENTED_EDGE('',*,*,#9322,.F.);
#14457=ORIENTED_EDGE('',*,*,#10048,.T.);
#14458=ORIENTED_EDGE('',*,*,#9295,.F.);
#14459=ORIENTED_EDGE('',*,*,#10050,.F.);
#14460=ORIENTED_EDGE('',*,*,#9182,.T.);
#14461=ORIENTED_EDGE('',*,*,#10049,.T.);
#14462=ORIENTED_EDGE('',*,*,#9613,.F.);
#14463=ORIENTED_EDGE('',*,*,#9167,.F.);
#14464=ORIENTED_EDGE('',*,*,#10051,.F.);
#14465=ORIENTED_EDGE('',*,*,#9323,.F.);
#14466=ORIENTED_EDGE('',*,*,#10050,.T.);
#14467=ORIENTED_EDGE('',*,*,#9294,.F.);
#14468=ORIENTED_EDGE('',*,*,#10052,.F.);
#14469=ORIENTED_EDGE('',*,*,#9183,.T.);
#14470=ORIENTED_EDGE('',*,*,#10051,.T.);
#14471=ORIENTED_EDGE('',*,*,#9166,.T.);
#14472=ORIENTED_EDGE('',*,*,#9206,.T.);
#14473=ORIENTED_EDGE('',*,*,#10053,.F.);
#14474=ORIENTED_EDGE('',*,*,#9324,.F.);
#14475=ORIENTED_EDGE('',*,*,#10052,.T.);
#14476=ORIENTED_EDGE('',*,*,#9293,.F.);
#14477=ORIENTED_EDGE('',*,*,#10054,.F.);
#14478=ORIENTED_EDGE('',*,*,#9184,.T.);
#14479=ORIENTED_EDGE('',*,*,#10053,.T.);
#14480=ORIENTED_EDGE('',*,*,#9205,.T.);
#14481=ORIENTED_EDGE('',*,*,#9196,.T.);
#14482=ORIENTED_EDGE('',*,*,#10055,.F.);
#14483=ORIENTED_EDGE('',*,*,#9022,.F.);
#14484=ORIENTED_EDGE('',*,*,#9325,.F.);
#14485=ORIENTED_EDGE('',*,*,#10054,.T.);
#14486=ORIENTED_EDGE('',*,*,#9292,.F.);
#14487=ORIENTED_EDGE('',*,*,#10056,.F.);
#14488=ORIENTED_EDGE('',*,*,#9185,.T.);
#14489=ORIENTED_EDGE('',*,*,#10055,.T.);
#14490=ORIENTED_EDGE('',*,*,#9195,.F.);
#14491=ORIENTED_EDGE('',*,*,#10057,.F.);
#14492=ORIENTED_EDGE('',*,*,#9024,.F.);
#14493=ORIENTED_EDGE('',*,*,#9023,.F.);
#14494=ORIENTED_EDGE('',*,*,#10056,.T.);
#14495=ORIENTED_EDGE('',*,*,#9291,.F.);
#14496=ORIENTED_EDGE('',*,*,#9290,.F.);
#14497=ORIENTED_EDGE('',*,*,#10058,.F.);
#14498=ORIENTED_EDGE('',*,*,#9186,.T.);
#14499=ORIENTED_EDGE('',*,*,#10057,.T.);
#14500=ORIENTED_EDGE('',*,*,#9194,.F.);
#14501=ORIENTED_EDGE('',*,*,#10059,.F.);
#14502=ORIENTED_EDGE('',*,*,#9025,.F.);
#14503=ORIENTED_EDGE('',*,*,#10058,.T.);
#14504=ORIENTED_EDGE('',*,*,#9289,.F.);
#14505=ORIENTED_EDGE('',*,*,#9288,.F.);
#14506=ORIENTED_EDGE('',*,*,#9034,.F.);
#14507=ORIENTED_EDGE('',*,*,#10060,.F.);
#14508=ORIENTED_EDGE('',*,*,#9187,.T.);
#14509=ORIENTED_EDGE('',*,*,#10059,.T.);
#14510=ORIENTED_EDGE('',*,*,#9193,.T.);
#14511=ORIENTED_EDGE('',*,*,#10061,.F.);
#14512=ORIENTED_EDGE('',*,*,#9026,.F.);
#14513=ORIENTED_EDGE('',*,*,#10060,.T.);
#14514=ORIENTED_EDGE('',*,*,#9033,.F.);
#14515=ORIENTED_EDGE('',*,*,#9032,.F.);
#14516=ORIENTED_EDGE('',*,*,#10062,.F.);
#14517=ORIENTED_EDGE('',*,*,#9188,.T.);
#14518=ORIENTED_EDGE('',*,*,#10061,.T.);
#14519=ORIENTED_EDGE('',*,*,#9192,.T.);
#14520=ORIENTED_EDGE('',*,*,#10063,.F.);
#14521=ORIENTED_EDGE('',*,*,#9027,.F.);
#14522=ORIENTED_EDGE('',*,*,#10062,.T.);
#14523=ORIENTED_EDGE('',*,*,#9031,.F.);
#14524=ORIENTED_EDGE('',*,*,#10064,.F.);
#14525=ORIENTED_EDGE('',*,*,#9189,.F.);
#14526=ORIENTED_EDGE('',*,*,#10063,.T.);
#14527=ORIENTED_EDGE('',*,*,#9191,.T.);
#14528=ORIENTED_EDGE('',*,*,#10065,.F.);
#14529=ORIENTED_EDGE('',*,*,#9028,.F.);
#14530=ORIENTED_EDGE('',*,*,#10064,.T.);
#14531=ORIENTED_EDGE('',*,*,#9030,.F.);
#14532=ORIENTED_EDGE('',*,*,#9029,.F.);
#14533=ORIENTED_EDGE('',*,*,#10065,.T.);
#14534=ORIENTED_EDGE('',*,*,#9190,.F.);
#14535=ORIENTED_EDGE('',*,*,#10066,.F.);
#14536=ORIENTED_EDGE('',*,*,#9453,.F.);
#14537=ORIENTED_EDGE('',*,*,#9020,.F.);
#14538=ORIENTED_EDGE('',*,*,#10067,.F.);
#14539=ORIENTED_EDGE('',*,*,#9161,.T.);
#14540=ORIENTED_EDGE('',*,*,#9208,.T.);
#14541=ORIENTED_EDGE('',*,*,#10067,.T.);
#14542=ORIENTED_EDGE('',*,*,#9019,.F.);
#14543=ORIENTED_EDGE('',*,*,#9018,.F.);
#14544=ORIENTED_EDGE('',*,*,#9017,.F.);
#14545=ORIENTED_EDGE('',*,*,#10068,.F.);
#14546=ORIENTED_EDGE('',*,*,#9162,.F.);
#14547=ORIENTED_EDGE('',*,*,#10066,.T.);
#14548=ORIENTED_EDGE('',*,*,#9207,.T.);
#14549=ORIENTED_EDGE('',*,*,#9164,.T.);
#14550=ORIENTED_EDGE('',*,*,#10069,.F.);
#14551=ORIENTED_EDGE('',*,*,#9015,.F.);
#14552=ORIENTED_EDGE('',*,*,#9014,.F.);
#14553=ORIENTED_EDGE('',*,*,#10068,.T.);
#14554=ORIENTED_EDGE('',*,*,#9016,.F.);
#14555=ORIENTED_EDGE('',*,*,#10069,.T.);
#14556=ORIENTED_EDGE('',*,*,#9163,.F.);
#16562=PLANE('',#18531);
#16563=PLANE('',#18533);
#16564=PLANE('',#18535);
#16565=PLANE('',#18536);
#16566=PLANE('',#18548);
#16567=PLANE('',#18551);
#16897=ADVANCED_FACE('',(#3781),#325,.F.);
#16898=ADVANCED_FACE('',(#3782),#326,.T.);
#16899=ADVANCED_FACE('',(#3783),#327,.T.);
#16900=ADVANCED_FACE('',(#3784,#3482,#3483),#328,.T.);
#16901=ADVANCED_FACE('',(#3785),#329,.T.);
#16902=ADVANCED_FACE('',(#3786),#3205,.T.);
#16903=ADVANCED_FACE('',(#3787,#3484,#3485,#3486,#3487,#3488,#3489,#3490,
#3491,#3492,#3493,#3494,#3495,#3496,#3497,#3498,#3499,#3500),#330,.T.);
#16904=ADVANCED_FACE('',(#3788),#331,.T.);
#16905=ADVANCED_FACE('',(#3789),#332,.T.);
#16906=ADVANCED_FACE('',(#3790),#1532,.T.);
#16907=ADVANCED_FACE('',(#3791),#131,.T.);
#16908=ADVANCED_FACE('',(#3792),#16562,.F.);
#16909=ADVANCED_FACE('',(#3793),#16563,.F.);
#16910=ADVANCED_FACE('',(#3794),#16564,.F.);
#16911=ADVANCED_FACE('',(#3795),#16565,.F.);
#16912=ADVANCED_FACE('',(#3796),#3206,.T.);
#16913=ADVANCED_FACE('',(#3797),#333,.F.);
#16914=ADVANCED_FACE('',(#3798),#3207,.T.);
#16915=ADVANCED_FACE('',(#3799),#3208,.F.);
#16916=ADVANCED_FACE('',(#3800),#3209,.F.);
#16917=ADVANCED_FACE('',(#3801),#3210,.T.);
#16918=ADVANCED_FACE('',(#3802),#16566,.F.);
#16919=ADVANCED_FACE('',(#3803),#3211,.F.);
#16920=ADVANCED_FACE('',(#3804),#3212,.F.);
#16921=ADVANCED_FACE('',(#3805),#16567,.F.);
#16922=ADVANCED_FACE('',(#3806),#3213,.T.);
#16923=ADVANCED_FACE('',(#3807),#3214,.T.);
#16924=ADVANCED_FACE('',(#3808),#3215,.T.);
#16925=ADVANCED_FACE('',(#3809),#3216,.T.);
#16926=ADVANCED_FACE('',(#3810),#1533,.T.);
#16927=ADVANCED_FACE('',(#3811),#192,.F.);
#16928=ADVANCED_FACE('',(#3812),#193,.F.);
#16929=ADVANCED_FACE('',(#3813),#1534,.T.);
#16930=ADVANCED_FACE('',(#3814),#1535,.T.);
#16931=ADVANCED_FACE('',(#3815),#194,.T.);
#16932=ADVANCED_FACE('',(#3816),#195,.T.);
#16933=ADVANCED_FACE('',(#3817),#1536,.T.);
#16934=ADVANCED_FACE('',(#3818),#1537,.T.);
#16935=ADVANCED_FACE('',(#3819),#196,.F.);
#16936=ADVANCED_FACE('',(#3820),#197,.F.);
#16937=ADVANCED_FACE('',(#3821),#1538,.T.);
#16938=ADVANCED_FACE('',(#3822),#1539,.T.);
#16939=ADVANCED_FACE('',(#3823),#198,.T.);
#16940=ADVANCED_FACE('',(#3824),#199,.T.);
#16941=ADVANCED_FACE('',(#3825),#1540,.T.);
#16942=ADVANCED_FACE('',(#3826),#143,.T.);
#16943=ADVANCED_FACE('',(#3827),#200,.T.);
#16944=ADVANCED_FACE('',(#3828),#3217,.T.);
#16945=ADVANCED_FACE('',(#3829),#1541,.T.);
#16946=ADVANCED_FACE('',(#3830),#3218,.T.);
#16947=ADVANCED_FACE('',(#3831),#1542,.T.);
#16948=ADVANCED_FACE('',(#3832),#132,.T.);
#16949=ADVANCED_FACE('',(#3833),#133,.T.);
#16950=ADVANCED_FACE('',(#3834),#1543,.T.);
#16951=ADVANCED_FACE('',(#3835),#144,.T.);
#16952=ADVANCED_FACE('',(#3836),#134,.T.);
#16953=ADVANCED_FACE('',(#3837),#1544,.T.);
#16954=ADVANCED_FACE('',(#3838),#145,.T.);
#16955=ADVANCED_FACE('',(#3839),#201,.T.);
#16956=ADVANCED_FACE('',(#3840),#146,.T.);
#16957=ADVANCED_FACE('',(#3841),#135,.T.);
#16958=ADVANCED_FACE('',(#3842),#1545,.T.);
#16959=ADVANCED_FACE('',(#3843),#3219,.T.);
#16960=ADVANCED_FACE('',(#3844),#1546,.T.);
#16961=ADVANCED_FACE('',(#3845),#3220,.T.);
#16962=ADVANCED_FACE('',(#3846),#147,.T.);
#16963=ADVANCED_FACE('',(#3847),#202,.T.);
#16964=ADVANCED_FACE('',(#3848),#148,.T.);
#16965=ADVANCED_FACE('',(#3849),#203,.T.);
#16966=ADVANCED_FACE('',(#3850),#1547,.T.);
#16967=ADVANCED_FACE('',(#3851),#1548,.T.);
#16968=ADVANCED_FACE('',(#3852),#204,.T.);
#16969=ADVANCED_FACE('',(#3853),#136,.T.);
#16970=ADVANCED_FACE('',(#3854),#334,.T.);
#16971=ADVANCED_FACE('',(#3855),#3221,.T.);
#16972=ADVANCED_FACE('',(#3856),#3222,.T.);
#16973=ADVANCED_FACE('',(#3857),#3223,.T.);
#16974=ADVANCED_FACE('',(#3858),#3224,.T.);
#16975=ADVANCED_FACE('',(#3859),#3225,.T.);
#16976=ADVANCED_FACE('',(#3860),#3226,.T.);
#16977=ADVANCED_FACE('',(#3861),#3227,.T.);
#16978=ADVANCED_FACE('',(#3862),#3228,.T.);
#16979=ADVANCED_FACE('',(#3863),#3229,.T.);
#16980=ADVANCED_FACE('',(#3864),#3230,.T.);
#16981=ADVANCED_FACE('',(#3865),#3231,.T.);
#16982=ADVANCED_FACE('',(#3866),#3232,.T.);
#16983=ADVANCED_FACE('',(#3867),#3233,.T.);
#16984=ADVANCED_FACE('',(#3868),#3234,.T.);
#16985=ADVANCED_FACE('',(#3869),#3235,.T.);
#16986=ADVANCED_FACE('',(#3870),#3236,.T.);
#16987=ADVANCED_FACE('',(#3871),#3237,.T.);
#16988=ADVANCED_FACE('',(#3872),#137,.T.);
#16989=ADVANCED_FACE('',(#3873),#138,.T.);
#16990=ADVANCED_FACE('',(#3874),#3238,.T.);
#16991=ADVANCED_FACE('',(#3875),#3239,.T.);
#16992=ADVANCED_FACE('',(#3876),#3240,.T.);
#16993=ADVANCED_FACE('',(#3877),#3241,.T.);
#16994=ADVANCED_FACE('',(#3878),#3242,.T.);
#16995=ADVANCED_FACE('',(#3879),#3243,.T.);
#16996=ADVANCED_FACE('',(#3880),#3244,.T.);
#16997=ADVANCED_FACE('',(#3881),#3245,.T.);
#16998=ADVANCED_FACE('',(#3882),#3246,.T.);
#16999=ADVANCED_FACE('',(#3883),#3247,.T.);
#17000=ADVANCED_FACE('',(#3884),#3248,.T.);
#17001=ADVANCED_FACE('',(#3885),#3249,.T.);
#17002=ADVANCED_FACE('',(#3886),#3250,.T.);
#17003=ADVANCED_FACE('',(#3887),#3251,.T.);
#17004=ADVANCED_FACE('',(#3888),#3252,.T.);
#17005=ADVANCED_FACE('',(#3889),#3253,.T.);
#17006=ADVANCED_FACE('',(#3890),#3254,.T.);
#17007=ADVANCED_FACE('',(#3891),#139,.F.);
#17008=ADVANCED_FACE('',(#3892),#140,.F.);
#17009=ADVANCED_FACE('',(#3893),#1549,.T.);
#17010=ADVANCED_FACE('',(#3894),#3255,.T.);
#17011=ADVANCED_FACE('',(#3895),#1550,.T.);
#17012=ADVANCED_FACE('',(#3896),#1551,.T.);
#17013=ADVANCED_FACE('',(#3897),#3256,.T.);
#17014=ADVANCED_FACE('',(#3898),#205,.T.);
#17015=ADVANCED_FACE('',(#3899),#1552,.T.);
#17016=ADVANCED_FACE('',(#3900),#3257,.T.);
#17017=ADVANCED_FACE('',(#3901),#1553,.T.);
#17018=ADVANCED_FACE('',(#3902),#1554,.T.);
#17019=ADVANCED_FACE('',(#3903),#3258,.T.);
#17020=ADVANCED_FACE('',(#3904),#1555,.T.);
#17021=ADVANCED_FACE('',(#3905),#1556,.T.);
#17022=ADVANCED_FACE('',(#3906),#3259,.T.);
#17023=ADVANCED_FACE('',(#3907),#1557,.T.);
#17024=ADVANCED_FACE('',(#3908),#1558,.T.);
#17025=ADVANCED_FACE('',(#3909),#3260,.T.);
#17026=ADVANCED_FACE('',(#3910),#1559,.T.);
#17027=ADVANCED_FACE('',(#3911),#1560,.T.);
#17028=ADVANCED_FACE('',(#3912),#3261,.T.);
#17029=ADVANCED_FACE('',(#3913),#1561,.T.);
#17030=ADVANCED_FACE('',(#3914),#1562,.T.);
#17031=ADVANCED_FACE('',(#3915),#3262,.T.);
#17032=ADVANCED_FACE('',(#3916),#1563,.T.);
#17033=ADVANCED_FACE('',(#3917),#1564,.T.);
#17034=ADVANCED_FACE('',(#3918),#3263,.T.);
#17035=ADVANCED_FACE('',(#3919),#1565,.T.);
#17036=ADVANCED_FACE('',(#3920),#1566,.T.);
#17037=ADVANCED_FACE('',(#3921),#3264,.T.);
#17038=ADVANCED_FACE('',(#3922),#1567,.T.);
#17039=ADVANCED_FACE('',(#3923),#1568,.T.);
#17040=ADVANCED_FACE('',(#3924),#3265,.T.);
#17041=ADVANCED_FACE('',(#3925),#1569,.T.);
#17042=ADVANCED_FACE('',(#3926),#1570,.T.);
#17043=ADVANCED_FACE('',(#3927),#3266,.T.);
#17044=ADVANCED_FACE('',(#3928),#1571,.T.);
#17045=ADVANCED_FACE('',(#3929),#1572,.T.);
#17046=ADVANCED_FACE('',(#3930),#3267,.T.);
#17047=ADVANCED_FACE('',(#3931),#1573,.T.);
#17048=ADVANCED_FACE('',(#3932),#1574,.T.);
#17049=ADVANCED_FACE('',(#3933),#3268,.T.);
#17050=ADVANCED_FACE('',(#3934),#1575,.T.);
#17051=ADVANCED_FACE('',(#3935),#1576,.T.);
#17052=ADVANCED_FACE('',(#3936),#3269,.T.);
#17053=ADVANCED_FACE('',(#3937),#1577,.T.);
#17054=ADVANCED_FACE('',(#3938),#1578,.T.);
#17055=ADVANCED_FACE('',(#3939),#3270,.T.);
#17056=ADVANCED_FACE('',(#3940),#1579,.T.);
#17057=ADVANCED_FACE('',(#3941),#1580,.T.);
#17058=ADVANCED_FACE('',(#3942),#3271,.T.);
#17059=ADVANCED_FACE('',(#3943),#1581,.T.);
#17060=ADVANCED_FACE('',(#3944),#1582,.T.);
#17061=ADVANCED_FACE('',(#3945),#3272,.T.);
#17062=ADVANCED_FACE('',(#3946),#1583,.T.);
#17063=ADVANCED_FACE('',(#3947),#1584,.T.);
#17064=ADVANCED_FACE('',(#3948),#3273,.T.);
#17065=ADVANCED_FACE('',(#3949),#1585,.T.);
#17066=ADVANCED_FACE('',(#3950),#1586,.T.);
#17067=ADVANCED_FACE('',(#3951),#3274,.T.);
#17068=ADVANCED_FACE('',(#3952),#1587,.T.);
#17069=ADVANCED_FACE('',(#3953),#1588,.T.);
#17070=ADVANCED_FACE('',(#3954),#3275,.T.);
#17071=ADVANCED_FACE('',(#3955),#1589,.T.);
#17072=ADVANCED_FACE('',(#3956),#1590,.T.);
#17073=ADVANCED_FACE('',(#3957),#3276,.T.);
#17074=ADVANCED_FACE('',(#3958),#1591,.T.);
#17075=ADVANCED_FACE('',(#3959),#1592,.T.);
#17076=ADVANCED_FACE('',(#3960),#3277,.T.);
#17077=ADVANCED_FACE('',(#3961),#1593,.T.);
#17078=ADVANCED_FACE('',(#3962),#1594,.T.);
#17079=ADVANCED_FACE('',(#3963),#3278,.T.);
#17080=ADVANCED_FACE('',(#3964),#1595,.T.);
#17081=ADVANCED_FACE('',(#3965),#1596,.T.);
#17082=ADVANCED_FACE('',(#3966),#3279,.T.);
#17083=ADVANCED_FACE('',(#3967),#1597,.T.);
#17084=ADVANCED_FACE('',(#3968),#1598,.T.);
#17085=ADVANCED_FACE('',(#3969),#3280,.T.);
#17086=ADVANCED_FACE('',(#3970),#1599,.T.);
#17087=ADVANCED_FACE('',(#3971),#1600,.T.);
#17088=ADVANCED_FACE('',(#3972),#1601,.T.);
#17089=ADVANCED_FACE('',(#3973),#1602,.T.);
#17090=ADVANCED_FACE('',(#3974),#1603,.T.);
#17091=ADVANCED_FACE('',(#3975),#1604,.T.);
#17092=ADVANCED_FACE('',(#3976),#1605,.T.);
#17093=ADVANCED_FACE('',(#3977),#1606,.T.);
#17094=ADVANCED_FACE('',(#3978),#1607,.T.);
#17095=ADVANCED_FACE('',(#3979),#206,.T.);
#17096=ADVANCED_FACE('',(#3980),#1608,.T.);
#17097=ADVANCED_FACE('',(#3981),#1609,.T.);
#17098=ADVANCED_FACE('',(#3982),#1610,.T.);
#17099=ADVANCED_FACE('',(#3983),#1611,.T.);
#17100=ADVANCED_FACE('',(#3984),#3281,.T.);
#17101=ADVANCED_FACE('',(#3985),#1612,.T.);
#17102=ADVANCED_FACE('',(#3986),#1613,.T.);
#17103=ADVANCED_FACE('',(#3987),#3282,.T.);
#17104=ADVANCED_FACE('',(#3988),#1614,.T.);
#17105=ADVANCED_FACE('',(#3989),#1615,.T.);
#17106=ADVANCED_FACE('',(#3990),#1616,.T.);
#17107=ADVANCED_FACE('',(#3991),#207,.T.);
#17108=ADVANCED_FACE('',(#3992),#208,.T.);
#17109=ADVANCED_FACE('',(#3993),#209,.T.);
#17110=ADVANCED_FACE('',(#3994),#1617,.T.);
#17111=ADVANCED_FACE('',(#3995),#1618,.T.);
#17112=ADVANCED_FACE('',(#3996),#210,.T.);
#17113=ADVANCED_FACE('',(#3997),#3283,.T.);
#17114=ADVANCED_FACE('',(#3998),#3284,.T.);
#17115=ADVANCED_FACE('',(#3999),#1619,.T.);
#17116=ADVANCED_FACE('',(#4000),#1620,.T.);
#17117=ADVANCED_FACE('',(#4001),#1621,.T.);
#17118=ADVANCED_FACE('',(#4002),#1622,.T.);
#17119=ADVANCED_FACE('',(#4003),#3285,.T.);
#17120=ADVANCED_FACE('',(#4004),#3286,.T.);
#17121=ADVANCED_FACE('',(#4005),#1623,.T.);
#17122=ADVANCED_FACE('',(#4006),#1624,.T.);
#17123=ADVANCED_FACE('',(#4007),#1625,.T.);
#17124=ADVANCED_FACE('',(#4008),#1626,.T.);
#17125=ADVANCED_FACE('',(#4009),#3287,.T.);
#17126=ADVANCED_FACE('',(#4010),#3288,.T.);
#17127=ADVANCED_FACE('',(#4011),#1627,.T.);
#17128=ADVANCED_FACE('',(#4012),#1628,.T.);
#17129=ADVANCED_FACE('',(#4013),#1629,.T.);
#17130=ADVANCED_FACE('',(#4014),#1630,.T.);
#17131=ADVANCED_FACE('',(#4015),#3289,.T.);
#17132=ADVANCED_FACE('',(#4016),#3290,.T.);
#17133=ADVANCED_FACE('',(#4017),#1631,.T.);
#17134=ADVANCED_FACE('',(#4018),#1632,.T.);
#17135=ADVANCED_FACE('',(#4019),#1633,.T.);
#17136=ADVANCED_FACE('',(#4020),#1634,.T.);
#17137=ADVANCED_FACE('',(#4021),#3291,.T.);
#17138=ADVANCED_FACE('',(#4022),#3292,.T.);
#17139=ADVANCED_FACE('',(#4023),#1635,.T.);
#17140=ADVANCED_FACE('',(#4024),#1636,.T.);
#17141=ADVANCED_FACE('',(#4025),#1637,.T.);
#17142=ADVANCED_FACE('',(#4026),#1638,.T.);
#17143=ADVANCED_FACE('',(#4027),#3293,.T.);
#17144=ADVANCED_FACE('',(#4028),#3294,.T.);
#17145=ADVANCED_FACE('',(#4029),#1639,.T.);
#17146=ADVANCED_FACE('',(#4030),#1640,.T.);
#17147=ADVANCED_FACE('',(#4031),#1641,.T.);
#17148=ADVANCED_FACE('',(#4032),#1642,.T.);
#17149=ADVANCED_FACE('',(#4033),#3295,.T.);
#17150=ADVANCED_FACE('',(#4034),#3296,.T.);
#17151=ADVANCED_FACE('',(#4035),#1643,.T.);
#17152=ADVANCED_FACE('',(#4036),#1644,.T.);
#17153=ADVANCED_FACE('',(#4037),#1645,.T.);
#17154=ADVANCED_FACE('',(#4038),#1646,.T.);
#17155=ADVANCED_FACE('',(#4039),#3297,.T.);
#17156=ADVANCED_FACE('',(#4040),#3298,.T.);
#17157=ADVANCED_FACE('',(#4041),#1647,.T.);
#17158=ADVANCED_FACE('',(#4042),#1648,.T.);
#17159=ADVANCED_FACE('',(#4043),#1649,.T.);
#17160=ADVANCED_FACE('',(#4044),#335,.T.);
#17161=ADVANCED_FACE('',(#4045),#3299,.T.);
#17162=ADVANCED_FACE('',(#4046),#3300,.T.);
#17163=ADVANCED_FACE('',(#4047),#1650,.T.);
#17164=ADVANCED_FACE('',(#4048),#1651,.T.);
#17165=ADVANCED_FACE('',(#4049),#1652,.T.);
#17166=ADVANCED_FACE('',(#4050),#336,.T.);
#17167=ADVANCED_FACE('',(#4051),#3301,.T.);
#17168=ADVANCED_FACE('',(#4052),#3302,.T.);
#17169=ADVANCED_FACE('',(#4053),#1653,.T.);
#17170=ADVANCED_FACE('',(#4054),#1654,.T.);
#17171=ADVANCED_FACE('',(#4055),#1655,.T.);
#17172=ADVANCED_FACE('',(#4056),#1656,.T.);
#17173=ADVANCED_FACE('',(#4057),#3303,.T.);
#17174=ADVANCED_FACE('',(#4058),#3304,.T.);
#17175=ADVANCED_FACE('',(#4059),#1657,.T.);
#17176=ADVANCED_FACE('',(#4060),#1658,.T.);
#17177=ADVANCED_FACE('',(#4061),#1659,.T.);
#17178=ADVANCED_FACE('',(#4062),#1660,.T.);
#17179=ADVANCED_FACE('',(#4063),#3305,.T.);
#17180=ADVANCED_FACE('',(#4064),#3306,.T.);
#17181=ADVANCED_FACE('',(#4065),#1661,.T.);
#17182=ADVANCED_FACE('',(#4066),#1662,.T.);
#17183=ADVANCED_FACE('',(#4067),#1663,.T.);
#17184=ADVANCED_FACE('',(#4068),#1664,.T.);
#17185=ADVANCED_FACE('',(#4069),#3307,.T.);
#17186=ADVANCED_FACE('',(#4070),#3308,.T.);
#17187=ADVANCED_FACE('',(#4071),#1665,.T.);
#17188=ADVANCED_FACE('',(#4072),#1666,.T.);
#17189=ADVANCED_FACE('',(#4073),#1667,.T.);
#17190=ADVANCED_FACE('',(#4074),#1668,.T.);
#17191=ADVANCED_FACE('',(#4075),#1669,.T.);
#17192=ADVANCED_FACE('',(#4076),#1670,.T.);
#17193=ADVANCED_FACE('',(#4077),#1671,.T.);
#17194=ADVANCED_FACE('',(#4078),#1672,.T.);
#17195=ADVANCED_FACE('',(#4079),#1673,.T.);
#17196=ADVANCED_FACE('',(#4080),#1674,.T.);
#17197=ADVANCED_FACE('',(#4081),#1675,.T.);
#17198=ADVANCED_FACE('',(#4082),#1676,.T.);
#17199=ADVANCED_FACE('',(#4083),#1677,.T.);
#17200=ADVANCED_FACE('',(#4084),#211,.T.);
#17201=ADVANCED_FACE('',(#4085),#1678,.T.);
#17202=ADVANCED_FACE('',(#4086),#1679,.T.);
#17203=ADVANCED_FACE('',(#4087),#3309,.T.);
#17204=ADVANCED_FACE('',(#4088),#3310,.T.);
#17205=ADVANCED_FACE('',(#4089),#1680,.T.);
#17206=ADVANCED_FACE('',(#4090),#1681,.T.);
#17207=ADVANCED_FACE('',(#4091),#1682,.T.);
#17208=ADVANCED_FACE('',(#4092),#1683,.T.);
#17209=ADVANCED_FACE('',(#4093),#212,.T.);
#17210=ADVANCED_FACE('',(#4094),#213,.T.);
#17211=ADVANCED_FACE('',(#4095),#214,.T.);
#17212=ADVANCED_FACE('',(#4096),#1684,.T.);
#17213=ADVANCED_FACE('',(#4097),#215,.T.);
#17214=ADVANCED_FACE('',(#4098),#216,.T.);
#17215=ADVANCED_FACE('',(#4099),#217,.T.);
#17216=ADVANCED_FACE('',(#4100),#3311,.T.);
#17217=ADVANCED_FACE('',(#4101),#1685,.T.);
#17218=ADVANCED_FACE('',(#4102),#218,.T.);
#17219=ADVANCED_FACE('',(#4103),#1686,.T.);
#17220=ADVANCED_FACE('',(#4104),#219,.T.);
#17221=ADVANCED_FACE('',(#4105),#220,.T.);
#17222=ADVANCED_FACE('',(#4106),#1687,.T.);
#17223=ADVANCED_FACE('',(#4107),#221,.T.);
#17224=ADVANCED_FACE('',(#4108),#1688,.T.);
#17225=ADVANCED_FACE('',(#4109),#222,.T.);
#17226=ADVANCED_FACE('',(#4110),#1689,.T.);
#17227=ADVANCED_FACE('',(#4111),#3312,.T.);
#17228=ADVANCED_FACE('',(#4112),#1690,.T.);
#17229=ADVANCED_FACE('',(#4113),#223,.T.);
#17230=ADVANCED_FACE('',(#4114),#224,.T.);
#17231=ADVANCED_FACE('',(#4115),#225,.T.);
#17232=ADVANCED_FACE('',(#4116),#226,.T.);
#17233=ADVANCED_FACE('',(#4117),#1691,.T.);
#17234=ADVANCED_FACE('',(#4118),#3313,.T.);
#17235=ADVANCED_FACE('',(#4119),#1692,.T.);
#17236=ADVANCED_FACE('',(#4120),#227,.T.);
#17237=ADVANCED_FACE('',(#4121),#1693,.T.);
#17238=ADVANCED_FACE('',(#4122),#228,.T.);
#17239=ADVANCED_FACE('',(#4123),#1694,.T.);
#17240=ADVANCED_FACE('',(#4124),#229,.T.);
#17241=ADVANCED_FACE('',(#4125),#230,.T.);
#17242=ADVANCED_FACE('',(#4126),#1695,.T.);
#17243=ADVANCED_FACE('',(#4127),#231,.T.);
#17244=ADVANCED_FACE('',(#4128),#1696,.T.);
#17245=ADVANCED_FACE('',(#4129),#3314,.T.);
#17246=ADVANCED_FACE('',(#4130),#232,.T.);
#17247=ADVANCED_FACE('',(#4131),#233,.T.);
#17248=ADVANCED_FACE('',(#4132),#234,.T.);
#17249=ADVANCED_FACE('',(#4133),#1697,.T.);
#17250=ADVANCED_FACE('',(#4134),#1698,.T.);
#17251=ADVANCED_FACE('',(#4135),#1699,.T.);
#17252=ADVANCED_FACE('',(#4136),#1700,.T.);
#17669=CLOSED_SHELL('',(#16897,#16898,#16899,#16900,#16901,#16902,#16903,
#16904,#16905,#16906,#16907,#16908,#16909,#16910,#16911,#16912,#16913,#16914,
#16915,#16916,#16917,#16918,#16919,#16920,#16921,#16922,#16923,#16924,#16925,
#16926,#16927,#16928,#16929,#16930,#16931,#16932,#16933,#16934,#16935,#16936,
#16937,#16938,#16939,#16940,#16941,#16942,#16943,#16944,#16945,#16946,#16947,
#16948,#16949,#16950,#16951,#16952,#16953,#16954,#16955,#16956,#16957,#16958,
#16959,#16960,#16961,#16962,#16963,#16964,#16965,#16966,#16967,#16968,#16969,
#16970,#16971,#16972,#16973,#16974,#16975,#16976,#16977,#16978,#16979,#16980,
#16981,#16982,#16983,#16984,#16985,#16986,#16987,#16988,#16989,#16990,#16991,
#16992,#16993,#16994,#16995,#16996,#16997,#16998,#16999,#17000,#17001,#17002,
#17003,#17004,#17005,#17006,#17007,#17008,#17009,#17010,#17011,#17012,#17013,
#17014,#17015,#17016,#17017,#17018,#17019,#17020,#17021,#17022,#17023,#17024,
#17025,#17026,#17027,#17028,#17029,#17030,#17031,#17032,#17033,#17034,#17035,
#17036,#17037,#17038,#17039,#17040,#17041,#17042,#17043,#17044,#17045,#17046,
#17047,#17048,#17049,#17050,#17051,#17052,#17053,#17054,#17055,#17056,#17057,
#17058,#17059,#17060,#17061,#17062,#17063,#17064,#17065,#17066,#17067,#17068,
#17069,#17070,#17071,#17072,#17073,#17074,#17075,#17076,#17077,#17078,#17079,
#17080,#17081,#17082,#17083,#17084,#17085,#17086,#17087,#17088,#17089,#17090,
#17091,#17092,#17093,#17094,#17095,#17096,#17097,#17098,#17099,#17100,#17101,
#17102,#17103,#17104,#17105,#17106,#17107,#17108,#17109,#17110,#17111,#17112,
#17113,#17114,#17115,#17116,#17117,#17118,#17119,#17120,#17121,#17122,#17123,
#17124,#17125,#17126,#17127,#17128,#17129,#17130,#17131,#17132,#17133,#17134,
#17135,#17136,#17137,#17138,#17139,#17140,#17141,#17142,#17143,#17144,#17145,
#17146,#17147,#17148,#17149,#17150,#17151,#17152,#17153,#17154,#17155,#17156,
#17157,#17158,#17159,#17160,#17161,#17162,#17163,#17164,#17165,#17166,#17167,
#17168,#17169,#17170,#17171,#17172,#17173,#17174,#17175,#17176,#17177,#17178,
#17179,#17180,#17181,#17182,#17183,#17184,#17185,#17186,#17187,#17188,#17189,
#17190,#17191,#17192,#17193,#17194,#17195,#17196,#17197,#17198,#17199,#17200,
#17201,#17202,#17203,#17204,#17205,#17206,#17207,#17208,#17209,#17210,#17211,
#17212,#17213,#17214,#17215,#17216,#17217,#17218,#17219,#17220,#17221,#17222,
#17223,#17224,#17225,#17226,#17227,#17228,#17229,#17230,#17231,#17232,#17233,
#17234,#17235,#17236,#17237,#17238,#17239,#17240,#17241,#17242,#17243,#17244,
#17245,#17246,#17247,#17248,#17249,#17250,#17251,#17252));
#18520=AXIS2_PLACEMENT_3D('',#25844,#21173,#21174);
#18521=AXIS2_PLACEMENT_3D('',#26092,#21175,#21176);
#18522=AXIS2_PLACEMENT_3D('',#27005,#21177,#21178);
#18523=AXIS2_PLACEMENT_3D('',#29780,#21194,#21195);
#18524=AXIS2_PLACEMENT_3D('',#29789,#21196,#21197);
#18525=AXIS2_PLACEMENT_3D('',#30303,#21198,#21199);
#18526=AXIS2_PLACEMENT_3D('',#31538,#21215,#21216);
#18527=AXIS2_PLACEMENT_3D('',#31908,#21217,#21218);
#18528=AXIS2_PLACEMENT_3D('',#31912,#21220,#21221);
#18529=AXIS2_PLACEMENT_3D('',#32079,#21223,#21224);
#18530=AXIS2_PLACEMENT_3D('',#35112,#21255,#21256);
#18531=AXIS2_PLACEMENT_3D('',#35124,#21257,#21258);
#18532=AXIS2_PLACEMENT_3D('',#35132,#21259,#21260);
#18533=AXIS2_PLACEMENT_3D('',#35144,#21262,#21263);
#18534=AXIS2_PLACEMENT_3D('',#35159,#21265,#21266);
#18535=AXIS2_PLACEMENT_3D('',#35164,#21267,#21268);
#18536=AXIS2_PLACEMENT_3D('',#35195,#21270,#21271);
#18537=AXIS2_PLACEMENT_3D('',#35203,#21272,#21273);
#18538=AXIS2_PLACEMENT_3D('',#35215,#21275,#21276);
#18539=AXIS2_PLACEMENT_3D('',#35386,#21277,#21278);
#18540=AXIS2_PLACEMENT_3D('',#35434,#21279,#21280);
#18541=AXIS2_PLACEMENT_3D('',#35461,#21281,#21282);
#18542=AXIS2_PLACEMENT_3D('',#35611,#21283,#21284);
#18543=AXIS2_PLACEMENT_3D('',#35704,#21285,#21286);
#18544=AXIS2_PLACEMENT_3D('',#35751,#21287,#21288);
#18545=AXIS2_PLACEMENT_3D('',#35821,#21289,#21290);
#18546=AXIS2_PLACEMENT_3D('',#35891,#21291,#21292);
#18547=AXIS2_PLACEMENT_3D('',#35913,#21293,#21294);
#18548=AXIS2_PLACEMENT_3D('',#35923,#21295,#21296);
#18549=AXIS2_PLACEMENT_3D('',#35978,#21299,#21300);
#18550=AXIS2_PLACEMENT_3D('',#36162,#21302,#21303);
#18551=AXIS2_PLACEMENT_3D('',#36346,#21305,#21306);
#18552=AXIS2_PLACEMENT_3D('',#36395,#21307,#21308);
#18553=AXIS2_PLACEMENT_3D('',#36405,#21309,#21310);
#18554=AXIS2_PLACEMENT_3D('',#36437,#21311,#21312);
#18555=AXIS2_PLACEMENT_3D('',#36467,#21313,#21314);
#18556=AXIS2_PLACEMENT_3D('',#36470,#21315,#21316);
#18557=AXIS2_PLACEMENT_3D('',#36485,#21317,#21318);
#18558=AXIS2_PLACEMENT_3D('',#36495,#21319,#21320);
#18559=AXIS2_PLACEMENT_3D('',#36566,#21321,#21322);
#18560=AXIS2_PLACEMENT_3D('',#36567,#21323,#21324);
#18561=AXIS2_PLACEMENT_3D('',#36568,#21325,#21326);
#18562=AXIS2_PLACEMENT_3D('',#36576,#21327,#21328);
#18563=AXIS2_PLACEMENT_3D('',#36577,#21329,#21330);
#18564=AXIS2_PLACEMENT_3D('',#36633,#21331,#21332);
#18565=AXIS2_PLACEMENT_3D('',#36641,#21333,#21334);
#18566=AXIS2_PLACEMENT_3D('',#36649,#21335,#21336);
#18567=AXIS2_PLACEMENT_3D('',#36678,#21337,#21338);
#18568=AXIS2_PLACEMENT_3D('',#36700,#21339,#21340);
#18569=AXIS2_PLACEMENT_3D('',#36701,#21341,#21342);
#18570=AXIS2_PLACEMENT_3D('',#36702,#21343,#21344);
#18571=AXIS2_PLACEMENT_3D('',#36703,#21345,#21346);
#18572=AXIS2_PLACEMENT_3D('',#36704,#21347,#21348);
#18573=AXIS2_PLACEMENT_3D('',#36705,#21349,#21350);
#18574=AXIS2_PLACEMENT_3D('',#36706,#21351,#21352);
#18575=AXIS2_PLACEMENT_3D('',#36793,#21353,#21354);
#18576=AXIS2_PLACEMENT_3D('',#36801,#21355,#21356);
#18577=AXIS2_PLACEMENT_3D('',#36842,#21357,#21358);
#18578=AXIS2_PLACEMENT_3D('',#36843,#21359,#21360);
#18579=AXIS2_PLACEMENT_3D('',#36844,#21361,#21362);
#18580=AXIS2_PLACEMENT_3D('',#36845,#21363,#21364);
#18581=AXIS2_PLACEMENT_3D('',#36846,#21365,#21366);
#18582=AXIS2_PLACEMENT_3D('',#36847,#21367,#21368);
#18583=AXIS2_PLACEMENT_3D('',#36848,#21369,#21370);
#18584=AXIS2_PLACEMENT_3D('',#36888,#21371,#21372);
#18585=AXIS2_PLACEMENT_3D('',#36889,#21373,#21374);
#18586=AXIS2_PLACEMENT_3D('',#36890,#21375,#21376);
#18587=AXIS2_PLACEMENT_3D('',#36912,#21377,#21378);
#18588=AXIS2_PLACEMENT_3D('',#36920,#21379,#21380);
#18589=AXIS2_PLACEMENT_3D('',#36921,#21381,#21382);
#18590=AXIS2_PLACEMENT_3D('',#36950,#21383,#21384);
#18591=AXIS2_PLACEMENT_3D('',#36951,#21385,#21386);
#18592=AXIS2_PLACEMENT_3D('',#36952,#21387,#21388);
#18593=AXIS2_PLACEMENT_3D('',#36981,#21389,#21390);
#18594=AXIS2_PLACEMENT_3D('',#36982,#21391,#21392);
#18595=AXIS2_PLACEMENT_3D('',#36983,#21393,#21394);
#18596=AXIS2_PLACEMENT_3D('',#36984,#21395,#21396);
#18597=AXIS2_PLACEMENT_3D('',#36985,#21397,#21398);
#18598=AXIS2_PLACEMENT_3D('',#36986,#21399,#21400);
#18599=AXIS2_PLACEMENT_3D('',#36987,#21401,#21402);
#18600=AXIS2_PLACEMENT_3D('',#37020,#21403,#21404);
#18601=AXIS2_PLACEMENT_3D('',#37021,#21405,#21406);
#18602=AXIS2_PLACEMENT_3D('',#37061,#21407,#21408);
#18603=AXIS2_PLACEMENT_3D('',#37062,#21409,#21410);
#18604=AXIS2_PLACEMENT_3D('',#37063,#21411,#21412);
#18605=AXIS2_PLACEMENT_3D('',#37064,#21413,#21414);
#18606=AXIS2_PLACEMENT_3D('',#37065,#21415,#21416);
#18607=AXIS2_PLACEMENT_3D('',#37066,#21417,#21418);
#18608=AXIS2_PLACEMENT_3D('',#37067,#21419,#21420);
#18609=AXIS2_PLACEMENT_3D('',#37068,#21421,#21422);
#18610=AXIS2_PLACEMENT_3D('',#37069,#21423,#21424);
#18611=AXIS2_PLACEMENT_3D('',#37070,#21425,#21426);
#18612=AXIS2_PLACEMENT_3D('',#37071,#21427,#21428);
#18613=AXIS2_PLACEMENT_3D('',#37108,#21429,#21430);
#18614=AXIS2_PLACEMENT_3D('',#37145,#21431,#21432);
#18615=AXIS2_PLACEMENT_3D('',#37146,#21433,#21434);
#18616=AXIS2_PLACEMENT_3D('',#37147,#21435,#21436);
#18617=AXIS2_PLACEMENT_3D('',#37311,#21437,#21438);
#18618=AXIS2_PLACEMENT_3D('',#37320,#21439,#21440);
#18619=AXIS2_PLACEMENT_3D('',#37334,#21441,#21442);
#18620=AXIS2_PLACEMENT_3D('',#37408,#21443,#21444);
#18621=AXIS2_PLACEMENT_3D('',#37497,#21445,#21446);
#18622=AXIS2_PLACEMENT_3D('',#37648,#21447,#21448);
#18623=AXIS2_PLACEMENT_3D('',#37844,#21449,#21450);
#18624=AXIS2_PLACEMENT_3D('',#37931,#21451,#21452);
#18625=AXIS2_PLACEMENT_3D('',#38086,#21453,#21454);
#18626=AXIS2_PLACEMENT_3D('',#38177,#21455,#21456);
#18627=AXIS2_PLACEMENT_3D('',#38333,#21457,#21458);
#18628=AXIS2_PLACEMENT_3D('',#38421,#21459,#21460);
#18629=AXIS2_PLACEMENT_3D('',#38507,#21461,#21462);
#18630=AXIS2_PLACEMENT_3D('',#38595,#21463,#21464);
#18631=AXIS2_PLACEMENT_3D('',#38682,#21465,#21466);
#18632=AXIS2_PLACEMENT_3D('',#38775,#21467,#21468);
#18633=AXIS2_PLACEMENT_3D('',#38892,#21469,#21470);
#18634=AXIS2_PLACEMENT_3D('',#38989,#21471,#21472);
#18635=AXIS2_PLACEMENT_3D('',#39075,#21473,#21474);
#18636=AXIS2_PLACEMENT_3D('',#39162,#21475,#21476);
#18637=AXIS2_PLACEMENT_3D('',#39171,#21477,#21478);
#18638=AXIS2_PLACEMENT_3D('',#39172,#21479,#21480);
#18639=AXIS2_PLACEMENT_3D('',#39246,#21481,#21482);
#18640=AXIS2_PLACEMENT_3D('',#39333,#21483,#21484);
#18641=AXIS2_PLACEMENT_3D('',#39482,#21485,#21486);
#18642=AXIS2_PLACEMENT_3D('',#39663,#21487,#21488);
#18643=AXIS2_PLACEMENT_3D('',#39748,#21489,#21490);
#18644=AXIS2_PLACEMENT_3D('',#39899,#21491,#21492);
#18645=AXIS2_PLACEMENT_3D('',#39986,#21493,#21494);
#18646=AXIS2_PLACEMENT_3D('',#40137,#21495,#21496);
#18647=AXIS2_PLACEMENT_3D('',#40253,#21497,#21498);
#18648=AXIS2_PLACEMENT_3D('',#40365,#21499,#21500);
#18649=AXIS2_PLACEMENT_3D('',#40448,#21501,#21502);
#18650=AXIS2_PLACEMENT_3D('',#40531,#21503,#21504);
#18651=AXIS2_PLACEMENT_3D('',#40618,#21505,#21506);
#18652=AXIS2_PLACEMENT_3D('',#40728,#21507,#21508);
#18653=AXIS2_PLACEMENT_3D('',#40824,#21509,#21510);
#18654=AXIS2_PLACEMENT_3D('',#40907,#21511,#21512);
#18655=AXIS2_PLACEMENT_3D('',#40989,#21513,#21514);
#18656=AXIS2_PLACEMENT_3D('',#40990,#21515,#21516);
#18657=AXIS2_PLACEMENT_3D('',#41035,#21517,#21518);
#18658=AXIS2_PLACEMENT_3D('',#41107,#21519,#21520);
#18659=AXIS2_PLACEMENT_3D('',#41124,#21521,#21522);
#18660=AXIS2_PLACEMENT_3D('',#41169,#21523,#21524);
#18661=AXIS2_PLACEMENT_3D('',#41244,#21525,#21526);
#18662=AXIS2_PLACEMENT_3D('',#41317,#21527,#21528);
#18663=AXIS2_PLACEMENT_3D('',#41392,#21529,#21530);
#18664=AXIS2_PLACEMENT_3D('',#41465,#21531,#21532);
#18665=AXIS2_PLACEMENT_3D('',#41540,#21533,#21534);
#18666=AXIS2_PLACEMENT_3D('',#41613,#21535,#21536);
#18667=AXIS2_PLACEMENT_3D('',#41687,#21537,#21538);
#18668=AXIS2_PLACEMENT_3D('',#41762,#21539,#21540);
#18669=AXIS2_PLACEMENT_3D('',#41838,#21541,#21542);
#18670=AXIS2_PLACEMENT_3D('',#41915,#21543,#21544);
#18671=AXIS2_PLACEMENT_3D('',#42001,#21545,#21546);
#18672=AXIS2_PLACEMENT_3D('',#42079,#21547,#21548);
#18673=AXIS2_PLACEMENT_3D('',#42154,#21549,#21550);
#18674=AXIS2_PLACEMENT_3D('',#42227,#21551,#21552);
#18675=AXIS2_PLACEMENT_3D('',#42301,#21553,#21554);
#18676=AXIS2_PLACEMENT_3D('',#42375,#21555,#21556);
#18677=AXIS2_PLACEMENT_3D('',#42449,#21557,#21558);
#18678=AXIS2_PLACEMENT_3D('',#42523,#21559,#21560);
#18679=AXIS2_PLACEMENT_3D('',#42597,#21561,#21562);
#18680=AXIS2_PLACEMENT_3D('',#42671,#21563,#21564);
#18681=AXIS2_PLACEMENT_3D('',#42745,#21565,#21566);
#18682=AXIS2_PLACEMENT_3D('',#42816,#21567,#21568);
#18683=AXIS2_PLACEMENT_3D('',#42892,#21569,#21570);
#18684=AXIS2_PLACEMENT_3D('',#43204,#21571,#21572);
#18685=AXIS2_PLACEMENT_3D('',#43350,#21573,#21574);
#18686=AXIS2_PLACEMENT_3D('',#43419,#21575,#21576);
#18687=AXIS2_PLACEMENT_3D('',#43512,#21577,#21578);
#18688=AXIS2_PLACEMENT_3D('',#43520,#21579,#21580);
#18689=AXIS2_PLACEMENT_3D('',#43545,#21581,#21582);
#18690=AXIS2_PLACEMENT_3D('',#43605,#21583,#21584);
#18691=AXIS2_PLACEMENT_3D('',#43622,#21585,#21586);
#18692=AXIS2_PLACEMENT_3D('',#43638,#21587,#21588);
#18693=AXIS2_PLACEMENT_3D('',#43771,#21589,#21590);
#18694=AXIS2_PLACEMENT_3D('',#43787,#21591,#21592);
#18695=AXIS2_PLACEMENT_3D('',#43920,#21593,#21594);
#18696=AXIS2_PLACEMENT_3D('',#43935,#21595,#21596);
#18697=AXIS2_PLACEMENT_3D('',#44068,#21597,#21598);
#18698=AXIS2_PLACEMENT_3D('',#44083,#21599,#21600);
#18699=AXIS2_PLACEMENT_3D('',#44216,#21601,#21602);
#18700=AXIS2_PLACEMENT_3D('',#44232,#21603,#21604);
#18701=AXIS2_PLACEMENT_3D('',#44366,#21605,#21606);
#18702=AXIS2_PLACEMENT_3D('',#44382,#21607,#21608);
#18703=AXIS2_PLACEMENT_3D('',#44520,#21609,#21610);
#18704=AXIS2_PLACEMENT_3D('',#44536,#21611,#21612);
#18705=AXIS2_PLACEMENT_3D('',#44687,#21613,#21614);
#18706=AXIS2_PLACEMENT_3D('',#44703,#21615,#21616);
#18707=AXIS2_PLACEMENT_3D('',#44849,#21617,#21618);
#18708=AXIS2_PLACEMENT_3D('',#44865,#21619,#21620);
#18709=AXIS2_PLACEMENT_3D('',#45010,#21621,#21622);
#18710=AXIS2_PLACEMENT_3D('',#45026,#21623,#21624);
#18711=AXIS2_PLACEMENT_3D('',#45158,#21625,#21626);
#18712=AXIS2_PLACEMENT_3D('',#45174,#21627,#21628);
#18713=AXIS2_PLACEMENT_3D('',#45301,#21629,#21630);
#18714=AXIS2_PLACEMENT_3D('',#45317,#21631,#21632);
#18715=AXIS2_PLACEMENT_3D('',#45455,#21633,#21634);
#18716=AXIS2_PLACEMENT_3D('',#45470,#21635,#21636);
#18717=AXIS2_PLACEMENT_3D('',#45882,#21637,#21638);
#18718=AXIS2_PLACEMENT_3D('',#45948,#21639,#21640);
#18719=AXIS2_PLACEMENT_3D('',#45962,#21641,#21642);
#18720=AXIS2_PLACEMENT_3D('',#46088,#21643,#21644);
#18721=AXIS2_PLACEMENT_3D('',#46093,#21645,#21646);
#18722=AXIS2_PLACEMENT_3D('',#46116,#21647,#21648);
#18723=AXIS2_PLACEMENT_3D('',#46139,#21649,#21650);
#18724=AXIS2_PLACEMENT_3D('',#46154,#21651,#21652);
#18725=AXIS2_PLACEMENT_3D('',#46165,#21653,#21654);
#18726=AXIS2_PLACEMENT_3D('',#46173,#21655,#21656);
#18727=AXIS2_PLACEMENT_3D('',#46215,#21657,#21658);
#18728=AXIS2_PLACEMENT_3D('',#46251,#21659,#21660);
#18729=AXIS2_PLACEMENT_3D('',#46262,#21661,#21662);
#18730=AXIS2_PLACEMENT_3D('',#46292,#21663,#21664);
#18731=AXIS2_PLACEMENT_3D('',#46372,#21665,#21666);
#18732=AXIS2_PLACEMENT_3D('',#46456,#21667,#21668);
#18733=AXIS2_PLACEMENT_3D('',#46499,#21669,#21670);
#18734=AXIS2_PLACEMENT_3D('',#46515,#21671,#21672);
#18735=AXIS2_PLACEMENT_3D('',#46532,#21673,#21674);
#18736=AXIS2_PLACEMENT_3D('',#46548,#21675,#21676);
#18737=AXIS2_PLACEMENT_3D('',#46598,#21677,#21678);
#18738=AXIS2_PLACEMENT_3D('',#46698,#21679,#21680);
#18739=AXIS2_PLACEMENT_3D('',#46767,#21681,#21682);
#18740=AXIS2_PLACEMENT_3D('',#46830,#21683,#21684);
#18741=AXIS2_PLACEMENT_3D('',#46838,#21685,#21686);
#18742=AXIS2_PLACEMENT_3D('',#46880,#21687,#21688);
#18743=AXIS2_PLACEMENT_3D('',#46913,#21689,#21690);
#18744=AXIS2_PLACEMENT_3D('',#46924,#21691,#21692);
#18745=AXIS2_PLACEMENT_3D('',#46932,#21693,#21694);
#18746=AXIS2_PLACEMENT_3D('',#46940,#21695,#21696);
#21173=DIRECTION('axis',(0.,0.,1.));
#21174=DIRECTION('refdir',(1.,0.,0.));
#21175=DIRECTION('center_axis',(0.0825919163630432,-0.996583451272946,6.19384420193564E-7));
#21176=DIRECTION('ref_axis',(0.765754157887476,0.0634623218806236,0.639994611992603));
#21177=DIRECTION('center_axis',(0.966179703385848,0.0733338853286848,-0.247222414088678));
#21178=DIRECTION('ref_axis',(0.153476402600925,0.606887091524721,0.779828860703003));
#21179=DIRECTION('',(-0.999797265210905,-0.00157571520789441,0.0200735048852593));
#21180=DIRECTION('',(-0.999795009940132,-0.00177423967236348,0.0201690399472964));
#21181=DIRECTION('',(-0.999814419433609,-0.00074299116254352,0.0192503157576034));
#21182=DIRECTION('',(-0.99930375064088,0.0370923483029995,-0.00402139931355867));
#21183=DIRECTION('',(0.999799569502936,0.000143273756301408,-0.0200199973619988));
#21184=DIRECTION('',(0.999795159155772,0.000550483968732209,-0.0202320709786369));
#21185=DIRECTION('',(0.999794381564603,0.000677070304206123,-0.0202666269432168));
#21186=DIRECTION('',(0.999794667552926,0.00072470430475225,-0.0202508650779472));
#21187=DIRECTION('',(0.99979559762733,0.000724626511420293,-0.0202048974614902));
#21188=DIRECTION('',(0.999794934842533,0.000845975517364629,-0.0202329579804895));
#21189=DIRECTION('',(0.999795478082445,0.000877544516035547,-0.0202047499741565));
#21190=DIRECTION('',(0.999792750698211,0.00115574151218025,-0.02032535148188));
#21191=DIRECTION('',(0.999796795370114,0.000927130164533834,-0.0201372390686534));
#21192=DIRECTION('',(0.999789554301239,0.00153991797600282,-0.0204566801499491));
#21193=DIRECTION('',(0.999799696863398,0.000859242700217791,-0.0199956958828443));
#21194=DIRECTION('center_axis',(-0.966520755854356,0.0727166375962521,0.246068931641969));
#21195=DIRECTION('ref_axis',(0.15568482121692,-0.596109982412235,0.787664348127514));
#21196=DIRECTION('center_axis',(0.965616313298931,-0.0694925699401865,-0.250511313545094));
#21197=DIRECTION('ref_axis',(0.147415368320144,-0.647349895074982,0.747801325573475));
#21198=DIRECTION('center_axis',(0.999750119804914,-3.4619426304031E-5,-0.0223538979051964));
#21199=DIRECTION('ref_axis',(0.0223537576222625,-0.00231815432474148,0.999747435946045));
#21200=DIRECTION('',(-0.999798518286744,0.000907194296559704,0.0200524270386368));
#21201=DIRECTION('',(-0.999797847151546,0.000882664687892492,0.0200869543281969));
#21202=DIRECTION('',(-0.999794527097293,0.00105818090835443,0.020243118323649));
#21203=DIRECTION('',(-0.999793960532759,0.00102594036328993,0.0202727385567707));
#21204=DIRECTION('',(-0.99979281884068,0.00103697298612291,0.0203284057819104));
#21205=DIRECTION('',(-0.999790073544858,0.00116543286722787,0.0204560652961453));
#21206=DIRECTION('',(-0.999792172359634,0.000941112379170086,0.0203648323315679));
#21207=DIRECTION('',(-0.999792286411407,0.000862374111952732,0.0203627194436703));
#21208=DIRECTION('',(-0.999788908874571,0.00103939132471049,0.0205196821873228));
#21209=DIRECTION('',(-0.999783724751033,0.00133812018306296,0.0207536299794865));
#21210=DIRECTION('',(-0.999792998568771,0.000603868432621,0.0203370439292827));
#21211=DIRECTION('',(0.999255736399573,0.0382175248776868,0.00523393396688128));
#21212=DIRECTION('',(0.999811045660937,-0.000922877743517363,-0.019417035588743));
#21213=DIRECTION('',(0.999809716706824,-0.000927106074859977,-0.0194851444168618));
#21214=DIRECTION('',(0.999816314546287,-0.000464324184849131,-0.0191604167525331));
#21215=DIRECTION('center_axis',(0.96683239686865,-0.0708748078028809,-0.245381087258425));
#21216=DIRECTION('ref_axis',(0.140042328661989,-0.656336014011258,0.741357661924891));
#21217=DIRECTION('center_axis',(0.957113823248678,-0.0400659616184508,0.286928297778184));
#21218=DIRECTION('ref_axis',(0.204108305786598,-0.609609959396545,-0.765973561497698));
#21219=DIRECTION('',(-0.999796968581146,0.00159150450853508,-0.0200870288830814));
#21220=DIRECTION('center_axis',(-0.965247781539032,0.0691046739050647,-0.252034252192936));
#21221=DIRECTION('ref_axis',(0.146842758004779,-0.654350158212197,-0.741797192546064));
#21222=DIRECTION('',(0.999816280485641,0.000465769226166559,0.0191621589307047));
#21223=DIRECTION('center_axis',(0.966757680149406,0.0705404390428106,0.245771508380827));
#21224=DIRECTION('ref_axis',(0.140547052978298,0.656363572024975,-0.741237740011753));
#21225=DIRECTION('',(0.999794903114167,-0.000848133911591957,0.0202344353961459));
#21226=DIRECTION('',(-0.999790098322183,-0.00116340831296703,-0.020454969518826));
#21227=DIRECTION('',(0.999795574158484,-0.000726169871118148,0.02020600332638));
#21228=DIRECTION('',(-0.999792175797662,-0.000940634061937126,-0.0203646856430204));
#21229=DIRECTION('',(0.999794642017327,-0.000726392539479541,0.0202520652607186));
#21230=DIRECTION('',(-0.999792264776137,-0.000863745000872394,-0.0203637235881719));
#21231=DIRECTION('',(0.999794385721742,-0.000676521551207557,0.0202664401875626));
#21232=DIRECTION('',(-0.999788865344958,-0.00104230550305824,-0.0205216551837372));
#21233=DIRECTION('',(0.999799527208902,-0.000872277300359709,0.0200036128028985));
#21234=DIRECTION('',(-0.9997980790357,-0.000940170020731757,-0.0200727984311172));
#21235=DIRECTION('',(0.999799571229728,-0.000142906932253215,0.0200199137476009));
#21236=DIRECTION('',(-0.999792941420028,-0.000607873253951516,-0.0203397339411044));
#21237=DIRECTION('',(-0.99979517235786,0.00176498749919714,-0.020161799251162));
#21238=DIRECTION('',(0.999809462767171,0.000941297182692076,0.0194974901162665));
#21239=DIRECTION('',(0.999795158107842,-0.000550333259916924,0.0202321268634491));
#21240=DIRECTION('',(-0.999783669579685,-0.00134174073953075,-0.020756053901623));
#21241=DIRECTION('',(0.999795442584518,-0.000879999821241033,0.020206399667981));
#21242=DIRECTION('',(-0.999792869478343,-0.00103298086046051,-0.0203261184391759));
#21243=DIRECTION('',(0.999792702399425,-0.00115909618973122,0.0203275361241377));
#21244=DIRECTION('',(-0.999794065485702,-0.00101784417227304,-0.0202679701206788));
#21245=DIRECTION('',(0.999796734453382,-0.000931561542189858,0.0201400588243195));
#21246=DIRECTION('',(-0.999794878993418,-0.00103154307653973,-0.0202271069957695));
#21247=DIRECTION('',(0.99978945409093,-0.00154695287703341,0.020461046536212));
#21248=DIRECTION('',(-0.99979917188903,-0.00078031983021078,-0.0200251589500104));
#21249=DIRECTION('',(-0.999814422778328,0.000742280540990978,-0.0192501694547673));
#21250=DIRECTION('',(0.999810938682864,0.000928619335546645,0.0194222695949644));
#21251=DIRECTION('',(-0.999303691614598,-0.0370938856343022,0.00402188686874901));
#21252=DIRECTION('',(0.999255934071334,-0.0382128842081673,-0.0052300768368433));
#21253=DIRECTION('',(0.0225950194900106,-0.0017788380133363,0.999743117420454));
#21254=DIRECTION('',(-0.0208097837600092,0.313767956481563,-0.94927162729392));
#21255=DIRECTION('center_axis',(-0.974667565771182,0.0286954385344785,-0.221810072000784));
#21256=DIRECTION('ref_axis',(-0.221901450770903,4.90925569561603E-18,0.975069098139085));
#21257=DIRECTION('center_axis',(6.93889390390723E-16,0.,1.));
#21258=DIRECTION('ref_axis',(1.,0.,-6.93889390390723E-16));
#21259=DIRECTION('center_axis',(6.93889390390723E-16,0.,1.));
#21260=DIRECTION('ref_axis',(1.,0.,-6.93889390390723E-16));
#21261=DIRECTION('',(0.,1.,0.));
#21262=DIRECTION('center_axis',(6.93889390390723E-16,0.,1.));
#21263=DIRECTION('ref_axis',(1.,0.,-6.93889390390723E-16));
#21264=DIRECTION('',(0.,1.,0.));
#21265=DIRECTION('center_axis',(6.93889390390723E-16,0.,1.));
#21266=DIRECTION('ref_axis',(1.,0.,-6.93889390390723E-16));
#21267=DIRECTION('center_axis',(6.93889390390723E-16,0.,-1.));
#21268=DIRECTION('ref_axis',(-1.,0.,-6.93889390390723E-16));
#21269=DIRECTION('',(0.,1.,0.));
#21270=DIRECTION('center_axis',(6.93889390390723E-16,0.,-1.));
#21271=DIRECTION('ref_axis',(-1.,0.,-6.93889390390723E-16));
#21272=DIRECTION('center_axis',(6.93889390390723E-16,0.,-1.));
#21273=DIRECTION('ref_axis',(-1.,0.,-6.93889390390723E-16));
#21274=DIRECTION('',(0.,1.,0.));
#21275=DIRECTION('center_axis',(0.999750166148961,-4.73635043611131E-5,
0.0223518017578594));
#21276=DIRECTION('ref_axis',(0.0223518017829303,3.33694979789914E-21,-0.999750167270332));
#21277=DIRECTION('center_axis',(0.0825919163630432,-0.996583451272946,6.19384420193564E-7));
#21278=DIRECTION('ref_axis',(0.765754157887476,0.0634623218806236,0.639994611992603));
#21279=DIRECTION('center_axis',(0.0825919165140713,0.996583451260439,-6.0402864252192E-7));
#21280=DIRECTION('ref_axis',(0.765754157790578,-0.0634623121281307,-0.639994613075606));
#21281=DIRECTION('center_axis',(-0.98075579440661,5.32973170040097E-6,0.195238499557471));
#21282=DIRECTION('ref_axis',(0.19443017895973,0.0909288071299902,0.976692816367359));
#21283=DIRECTION('center_axis',(-0.981482829121148,-3.75634276483288E-6,
-0.191550139979688));
#21284=DIRECTION('ref_axis',(0.190757106872796,-0.0909203347980143,-0.977417627679048));
#21285=DIRECTION('center_axis',(-4.86886864449402E-15,1.,-2.1379377376203E-14));
#21286=DIRECTION('ref_axis',(-4.04680781916367E-45,2.1379377376203E-14,
1.));
#21287=DIRECTION('center_axis',(0.,1.,0.));
#21288=DIRECTION('ref_axis',(-1.,0.,-4.22123945207479E-11));
#21289=DIRECTION('center_axis',(0.,1.,0.));
#21290=DIRECTION('ref_axis',(-1.,0.,-2.83604770904466E-14));
#21291=DIRECTION('center_axis',(1.47522099208952E-16,1.,-6.09726439183545E-15));
#21292=DIRECTION('ref_axis',(8.40782393547547E-47,6.09726439183545E-15,
1.));
#21293=DIRECTION('center_axis',(0.982692008587054,-0.00050387605033863,
0.185246220927898));
#21294=DIRECTION('ref_axis',(-0.0160368225195314,-0.996473482954562,0.0823615085575891));
#21295=DIRECTION('center_axis',(0.76964097577498,0.,-0.638476912979738));
#21296=DIRECTION('ref_axis',(-0.638476912979738,0.,-0.76964097577498));
#21297=DIRECTION('',(0.,1.,0.));
#21298=DIRECTION('',(0.,1.,0.));
#21299=DIRECTION('center_axis',(0.,1.,0.));
#21300=DIRECTION('ref_axis',(0.,0.,1.));
#21301=DIRECTION('',(0.,1.,0.));
#21302=DIRECTION('center_axis',(0.,1.,0.));
#21303=DIRECTION('ref_axis',(0.,0.,1.));
#21304=DIRECTION('',(0.,1.,0.));
#21305=DIRECTION('center_axis',(0.76964097577498,0.,0.638476912979738));
#21306=DIRECTION('ref_axis',(0.638476912979738,0.,-0.76964097577498));
#21307=DIRECTION('center_axis',(0.,0.,1.));
#21308=DIRECTION('ref_axis',(1.,0.,0.));
#21309=DIRECTION('center_axis',(6.93889390390723E-16,0.,-1.));
#21310=DIRECTION('ref_axis',(-1.,0.,-6.93889390390723E-16));
#21311=DIRECTION('center_axis',(0.,0.,1.));
#21312=DIRECTION('ref_axis',(1.,0.,0.));
#21313=DIRECTION('center_axis',(0.,0.,1.));
#21314=DIRECTION('ref_axis',(1.,0.,0.));
#21315=DIRECTION('center_axis',(6.93889390390723E-16,0.,1.));
#21316=DIRECTION('ref_axis',(1.,0.,-6.93889390390723E-16));
#21317=DIRECTION('center_axis',(0.,0.,1.));
#21318=DIRECTION('ref_axis',(1.,0.,0.));
#21319=DIRECTION('center_axis',(6.93889390390723E-16,0.,1.));
#21320=DIRECTION('ref_axis',(1.,0.,-6.93889390390723E-16));
#21321=DIRECTION('center_axis',(0.999993789125747,0.00350648594152928,-0.000355339658387565));
#21322=DIRECTION('ref_axis',(-0.00326396958594675,0.883331083394255,-0.468738246372188));
#21323=DIRECTION('center_axis',(0.99999378903564,0.00350650862306363,0.00035536941415181));
#21324=DIRECTION('ref_axis',(-0.000355367205935845,-1.25282104470708E-6,
0.999999936856288));
#21325=DIRECTION('center_axis',(0.999992536376844,0.00385800221437534,0.000207387369863947));
#21326=DIRECTION('ref_axis',(-0.00385800229734076,0.999992557881444,0.));
#21327=DIRECTION('center_axis',(0.999992536598678,0.00385794601180392,-0.000207363237830676));
#21328=DIRECTION('ref_axis',(-0.00385794609474882,0.999992558098274,0.));
#21329=DIRECTION('center_axis',(0.999990310769996,0.00440207548560395,-9.87651888418822E-6));
#21330=DIRECTION('ref_axis',(-0.0036207108715852,0.821212665146659,-0.570610768436336));
#21331=DIRECTION('center_axis',(-0.909784343381186,-0.228750702611131,-0.346360454719326));
#21332=DIRECTION('ref_axis',(-0.355794328393026,3.2321890514358E-17,0.93456428130084));
#21333=DIRECTION('center_axis',(0.981482840368801,6.94690961148907E-5,0.191550069787602));
#21334=DIRECTION('ref_axis',(0.191550070249807,0.,-0.981482842737098));
#21335=DIRECTION('center_axis',(0.98075583355353,-0.000125702323698021,
-0.195238262514414));
#21336=DIRECTION('ref_axis',(0.195238265280273,1.00024838000881E-5,0.980755841007485));
#21337=DIRECTION('center_axis',(-0.909784105944603,0.228750295766247,0.346361347089185));
#21338=DIRECTION('ref_axis',(0.355795210127735,-5.10614014417012E-17,0.934563945618576));
#21339=DIRECTION('center_axis',(0.909784343381305,-0.228750702611003,0.346360454719098));
#21340=DIRECTION('ref_axis',(0.355794328392781,1.06760012694273E-16,-0.934564281300933));
#21341=DIRECTION('center_axis',(0.999992536382172,-0.00385800090220185,
0.000207386085645872));
#21342=DIRECTION('ref_axis',(0.00385800098516621,0.999992557886507,0.));
#21343=DIRECTION('center_axis',(0.999990310574524,-0.00440211987885248,
9.88122079760886E-6));
#21344=DIRECTION('ref_axis',(-0.00362072769721535,-0.821207579688302,0.570618087159375));
#21345=DIRECTION('center_axis',(0.999993789045476,-0.00350650580089381,
0.000355369583883258));
#21346=DIRECTION('ref_axis',(-0.00326400780572816,-0.883333427384614,0.468733828860255));
#21347=DIRECTION('center_axis',(0.999992536601163,-0.0038579454128945,-0.000207362394964344));
#21348=DIRECTION('ref_axis',(0.00385794549583871,0.999992558100585,0.));
#21349=DIRECTION('center_axis',(0.999990310770151,-0.00440207545088307,
-9.87630342248303E-6));
#21350=DIRECTION('ref_axis',(-5.67743328359544E-5,-0.0106536201675253,-0.999943246966547));
#21351=DIRECTION('center_axis',(0.999993789133264,-0.00350648377631366,
-0.000355339871731304));
#21352=DIRECTION('ref_axis',(-0.000355337663693595,1.25270705322677E-6,
-0.999999936866786));
#21353=DIRECTION('center_axis',(0.0825919165140834,0.996583451260439,-6.02271343951247E-7));
#21354=DIRECTION('ref_axis',(0.996583451260621,-0.082591916514075,3.89962523269363E-8));
#21355=DIRECTION('center_axis',(-0.0825919163630573,0.996583451272945,-6.20081085572316E-7));
#21356=DIRECTION('ref_axis',(0.996583451273137,0.0825919163630472,-4.26522010047437E-8));
#21357=DIRECTION('center_axis',(1.,0.,0.));
#21358=DIRECTION('ref_axis',(0.,-1.,0.));
#21359=DIRECTION('center_axis',(-0.969814393901857,0.243844297412866,-1.75042618129133E-12));
#21360=DIRECTION('ref_axis',(-0.243844297412866,-0.969814393901857,-1.66055871266714E-29));
#21361=DIRECTION('center_axis',(6.93889390390723E-16,0.,1.));
#21362=DIRECTION('ref_axis',(1.,0.,-6.37059463001412E-16));
#21363=DIRECTION('center_axis',(-0.984842147348564,0.173453004603174,6.83371517254786E-16));
#21364=DIRECTION('ref_axis',(-0.173453004603174,-0.984842147348564,7.55355110189228E-33));
#21365=DIRECTION('center_axis',(0.999993711234398,-0.00354647500652752,
-2.58533075644835E-6));
#21366=DIRECTION('ref_axis',(0.00354647500653937,0.99999371123774,-7.29885891232207E-24));
#21367=DIRECTION('center_axis',(-0.999993447039029,0.00361187934263431,
0.000245370360983865));
#21368=DIRECTION('ref_axis',(-0.000245366581733725,1.4894891990769E-6,-0.999999969896511));
#21369=DIRECTION('center_axis',(0.999995302234954,-0.00306520929522128,
-3.17016093720866E-13));
#21370=DIRECTION('ref_axis',(0.00271824782984711,0.88680243276121,0.462140732220754));
#21371=DIRECTION('center_axis',(0.999995302242941,-0.00306520668935977,
1.41267078951194E-12));
#21372=DIRECTION('ref_axis',(2.87570856016762E-8,9.38219006929373E-6,0.999999999955987));
#21373=DIRECTION('center_axis',(0.999993711188974,-0.00354648781441971,
2.58552001539276E-6));
#21374=DIRECTION('ref_axis',(0.00354648781443156,0.999993711192317,-1.16816817935139E-23));
#21375=DIRECTION('center_axis',(-0.999993257216905,0.00366579675322716,
-0.00021784143289343));
#21376=DIRECTION('ref_axis',(0.00319184891825971,0.838306860871718,-0.545189342445255));
#21377=DIRECTION('center_axis',(-0.951640608285474,-0.167605461698958,-0.25746565182706));
#21378=DIRECTION('ref_axis',(-0.261159981199218,7.93998114470773E-18,0.965295532062603));
#21379=DIRECTION('center_axis',(-0.244892111977192,-0.956154896867404,-0.160610294464068));
#21380=DIRECTION('ref_axis',(0.968731061165788,-0.248113141797458,1.27019149305754E-16));
#21381=DIRECTION('center_axis',(-0.244864748752396,0.95616063541462,-0.160617851130988));
#21382=DIRECTION('ref_axis',(-0.968738082088973,-0.24808572774462,-1.42728691652663E-16));
#21383=DIRECTION('center_axis',(-0.951640608283787,0.167605461701957,-0.257465651831341));
#21384=DIRECTION('ref_axis',(-0.261159981203695,8.13263164653001E-17,0.965295532061392));
#21385=DIRECTION('center_axis',(1.,0.,0.));
#21386=DIRECTION('ref_axis',(0.,0.876535239907724,-0.481337691439087));
#21387=DIRECTION('center_axis',(-0.244892182585915,0.956154863195271,0.160610387261659));
#21388=DIRECTION('ref_axis',(-0.968731041871288,-0.248113217130746,-1.42505471275098E-17));
#21389=DIRECTION('center_axis',(-0.951640551025411,0.167605051542164,0.257466130474672));
#21390=DIRECTION('ref_axis',(0.261160448242619,4.15284970329584E-18,0.965295405704241));
#21391=DIRECTION('center_axis',(1.,0.,0.));
#21392=DIRECTION('ref_axis',(0.,0.87657024749419,0.481273935724733));
#21393=DIRECTION('center_axis',(0.984842218075142,-0.173452603026977,-9.02676907320607E-15));
#21394=DIRECTION('ref_axis',(0.173452603026977,0.984842218075142,2.17217989749286E-31));
#21395=DIRECTION('center_axis',(6.93889390390723E-16,0.,-1.));
#21396=DIRECTION('ref_axis',(-1.,0.,-6.37059463001412E-16));
#21397=DIRECTION('center_axis',(0.96981448141323,-0.243843949363496,2.90327682891753E-13));
#21398=DIRECTION('ref_axis',(0.243843949363496,0.96981448141323,4.72120435553235E-31));
#21399=DIRECTION('center_axis',(1.,0.,0.));
#21400=DIRECTION('ref_axis',(0.,-1.,0.));
#21401=DIRECTION('center_axis',(-0.244864821889913,-0.956160598919634,0.16061795688673));
#21402=DIRECTION('ref_axis',(0.968738062004926,-0.248085806169841,3.77743453549349E-19));
#21403=DIRECTION('center_axis',(0.999993662978143,0.00356005563298786,2.72893016458924E-6));
#21404=DIRECTION('ref_axis',(0.00311111586717999,-0.874261870422573,0.485444644509841));
#21405=DIRECTION('center_axis',(0.999995302242957,0.00306520668415282,-1.74781900008877E-12));
#21406=DIRECTION('ref_axis',(0.00271825281217274,-0.886804813943252,-0.462136162909508));
#21407=DIRECTION('center_axis',(0.999995302234954,0.00306520929503774,1.39698738163942E-14));
#21408=DIRECTION('ref_axis',(2.8755664516212E-8,-9.38124145866162E-6,-0.999999999955996));
#21409=DIRECTION('center_axis',(0.999993711234403,0.00354647500511862,-2.58533131823476E-6));
#21410=DIRECTION('ref_axis',(0.0031007485640922,-0.874666312378887,-0.484715614920607));
#21411=DIRECTION('center_axis',(-0.999993447038901,-0.00361187937971174,
0.000245370340625091));
#21412=DIRECTION('ref_axis',(0.00317944976032623,-0.843814728946945,0.536625189784654));
#21413=DIRECTION('center_axis',(1.,0.,0.));
#21414=DIRECTION('ref_axis',(0.,-1.,0.));
#21415=DIRECTION('center_axis',(0.984842147375681,0.173453004449208,-1.64841417546653E-10));
#21416=DIRECTION('ref_axis',(-0.173453004449208,0.984842147375681,-1.94987819100897E-27));
#21417=DIRECTION('center_axis',(6.93889390390723E-16,0.,1.));
#21418=DIRECTION('ref_axis',(1.,0.,-6.37059463001412E-16));
#21419=DIRECTION('center_axis',(0.969814393902275,0.243844297411202,-2.84511405416877E-13));
#21420=DIRECTION('ref_axis',(-0.243844297411202,0.969814393902275,1.27098327284467E-30));
#21421=DIRECTION('center_axis',(1.,0.,0.));
#21422=DIRECTION('ref_axis',(0.,-1.,0.));
#21423=DIRECTION('center_axis',(-0.0823386574739372,0.996604407719049,5.95150216138491E-7));
#21424=DIRECTION('ref_axis',(0.996604407719226,0.0823386574739416,1.7269978458749E-8));
#21425=DIRECTION('center_axis',(0.63736849112035,0.0611262158547342,-0.768130843191607));
#21426=DIRECTION('ref_axis',(-0.00927097489734817,0.997384807118265,0.0716770224975518));
#21427=DIRECTION('center_axis',(0.637368185944156,0.0611271411090484,0.768131022785885));
#21428=DIRECTION('ref_axis',(-0.769570799631323,1.71699639970919E-5,0.638561495910925));
#21429=DIRECTION('center_axis',(0.637368456188137,-0.0611270399883367,0.768130806593913));
#21430=DIRECTION('ref_axis',(-0.00927098015071904,-0.997384730640923,-0.0716780859913101));
#21431=DIRECTION('center_axis',(0.637368220895556,-0.0611263169692591,-0.768131059368262));
#21432=DIRECTION('ref_axis',(-0.769570797403229,-1.717109277194E-5,-0.638561498596111));
#21433=DIRECTION('center_axis',(0.0823386573805061,0.996604407726757,6.13355466221133E-7));
#21434=DIRECTION('ref_axis',(0.996604407726945,-0.082338657380496,-4.12451842793918E-8));
#21435=DIRECTION('center_axis',(-0.975990677738216,-0.0251890228193663,
-0.216350895763117));
#21436=DIRECTION('ref_axis',(-0.216419564343231,-5.31751016061812E-18,0.976300451792114));
#21437=DIRECTION('center_axis',(-0.966447028925014,-0.0723817684077612,
-0.246456933122562));
#21438=DIRECTION('ref_axis',(0.156314970820748,0.595634525008648,-0.787899195655783));
#21439=DIRECTION('center_axis',(0.965411969008708,0.0686536407204188,0.251528144967043));
#21440=DIRECTION('ref_axis',(0.148704659736293,0.64743602524561,-0.747471415765767));
#21441=DIRECTION('center_axis',(0.999764710177655,4.72949843663878E-6,0.0216915711976085));
#21442=DIRECTION('ref_axis',(0.0216915711978511,3.37899635702931E-23,-0.999764710188837));
#21443=DIRECTION('center_axis',(0.99976438521954,4.08870955359827E-6,0.0217065434806438));
#21444=DIRECTION('ref_axis',(0.0217065434808252,-2.19008514488595E-22,-0.999764385227897));
#21445=DIRECTION('center_axis',(0.999764064843307,3.40730474217083E-6,0.0217212945373594));
#21446=DIRECTION('ref_axis',(0.0217212945374855,-7.6410513036406E-23,-0.99976406484911));
#21447=DIRECTION('center_axis',(0.99976374924311,2.90109501624487E-6,0.0217358158564165));
#21448=DIRECTION('ref_axis',(0.021735815856508,-1.05284018011641E-22,-0.999763749247317));
#21449=DIRECTION('center_axis',(0.99976640399297,4.0363566896332E-6,0.0216133623176406));
#21450=DIRECTION('ref_axis',(0.0216133623178167,-1.60742745341573E-22,-0.999766404001114));
#21451=DIRECTION('center_axis',(0.999763129384452,8.25018479049991E-7,0.0217643084596511));
#21452=DIRECTION('ref_axis',(0.0217643084596585,2.45472806930464E-24,-0.999763129384792));
#21453=DIRECTION('center_axis',(0.999769417791993,1.50007309598972E-5,0.0214734958224482));
#21454=DIRECTION('ref_axis',(0.0214734958248642,5.20388214323119E-24,-0.999769417904478));
#21455=DIRECTION('center_axis',(0.999763438172819,2.16269669590136E-6,0.0217501192683182));
#21456=DIRECTION('ref_axis',(0.0217501192683691,-1.26685871371197E-22,-0.999763438175157));
#21457=DIRECTION('center_axis',(0.99976503922338,5.12733989460498E-6,0.0216764000789616));
#21458=DIRECTION('ref_axis',(0.0216764000792465,1.99825578127218E-22,-0.999765039236522));
#21459=DIRECTION('center_axis',(0.999765375453303,5.10299320466825E-6,0.0216608868395403));
#21460=DIRECTION('ref_axis',(0.0216608868398223,1.61235729862652E-22,-0.99976537546632));
#21461=DIRECTION('center_axis',(0.999765713346224,5.51245434595147E-6,0.0216452855589496));
#21462=DIRECTION('ref_axis',(0.0216452855592785,-1.64937072290126E-22,-0.999765713361414));
#21463=DIRECTION('center_axis',(0.999766057463275,4.50676636095009E-6,0.0216293856599718));
#21464=DIRECTION('ref_axis',(0.0216293856601915,-1.13137331017225E-22,-0.999766057473429));
#21465=DIRECTION('center_axis',(0.999769839153505,1.40781112176933E-5,0.0214538695992536));
#21466=DIRECTION('ref_axis',(0.0214538696013796,1.23674150965502E-22,-0.999769839252579));
#21467=DIRECTION('center_axis',(0.999770358169119,3.64750266020402E-5,0.0214296429266803));
#21468=DIRECTION('ref_axis',(0.0214296429409356,4.42227884678903E-22,-0.99977035883418));
#21469=DIRECTION('center_axis',(0.999766032799768,2.3287275843937E-5,0.0216305135749479));
#21470=DIRECTION('ref_axis',(0.021630513580813,-4.12908816846881E-22,-0.999766033070853));
#21471=DIRECTION('center_axis',(0.999763745028459,3.66762269207557E-6,0.0217360095974351));
#21472=DIRECTION('ref_axis',(0.0217360095975813,-5.4425946294211E-23,-0.999763745035183));
#21473=DIRECTION('center_axis',(0.999763972772618,7.80388041093266E-6,0.0217255307187726));
#21474=DIRECTION('ref_axis',(0.0217255307194341,-4.1126736519674E-22,-0.999763972803061));
#21475=DIRECTION('center_axis',(-0.974671768615882,-0.0286863516212842,
0.221792778723403));
#21476=DIRECTION('ref_axis',(0.221884092473798,-2.88678970212481E-17,0.975073048292834));
#21477=DIRECTION('center_axis',(-0.975976237722848,0.0252188885886727,0.216412548293086));
#21478=DIRECTION('ref_axis',(0.216481399498132,-2.06557536366637E-17,0.976286742546128));
#21479=DIRECTION('center_axis',(0.999764709262297,-4.73662963717919E-6,
-0.0216916133848715));
#21480=DIRECTION('ref_axis',(0.0216916112630805,-0.000274958271209076,0.999764671509631));
#21481=DIRECTION('center_axis',(0.999764384264301,-4.08849168619633E-6,
-0.0217065874772601));
#21482=DIRECTION('ref_axis',(0.0217065858809087,-0.000238963614421796,0.999764355748786));
#21483=DIRECTION('center_axis',(0.999764063905754,-3.40534231195707E-6,
-0.0217213376902918));
#21484=DIRECTION('ref_axis',(0.0217213365462412,-0.000203702899778933,0.999764043184077));
#21485=DIRECTION('center_axis',(0.999763748332528,-2.89897229151112E-6,
-0.0217358577399271));
#21486=DIRECTION('ref_axis',(0.0217358569031682,-0.000174525088592317,0.99976373312182));
#21487=DIRECTION('center_axis',(0.999766403501999,-4.31175631876197E-6,
-0.0216133849751954));
#21488=DIRECTION('ref_axis',(0.0216133834966834,-0.000220804919340372,0.999766379160158));
#21489=DIRECTION('center_axis',(0.999763128353256,-8.40752198221754E-7,
-0.0217643558279152));
#21490=DIRECTION('ref_axis',(0.0217643558021162,-2.35325148120707E-5,0.999763128077216));
#21491=DIRECTION('center_axis',(0.999769418060103,-1.50448636207487E-5,
-0.0214734833088371));
#21492=DIRECTION('ref_axis',(0.0214734544646323,-0.00108205437596858,0.999768833236805));
#21493=DIRECTION('center_axis',(0.999763437260841,-2.16801141837553E-6,
-0.0217501611876457));
#21494=DIRECTION('ref_axis',(0.0217501607491883,-0.000124518145035359,0.999763429518512));
#21495=DIRECTION('center_axis',(0.999765038344753,-5.14904944543397E-6,
-0.0216764405980732));
#21496=DIRECTION('ref_axis',(0.0216764381689193,-0.000292188339262183,0.999764995713634));
#21497=DIRECTION('center_axis',(0.999765374632217,-5.15081959904467E-6,
-0.0216609247256913));
#21498=DIRECTION('ref_axis',(0.0216609223653019,-0.000286176218006351,0.999765333738601));
#21499=DIRECTION('center_axis',(0.99976571267043,-5.61582566448302E-6,-0.0216453167463528));
#21500=DIRECTION('ref_axis',(0.0216453140457445,-0.000303503805251101,0.999765666676597));
#21501=DIRECTION('center_axis',(0.999766057204937,-4.76013267136721E-6,
-0.0216293975467653));
#21502=DIRECTION('ref_axis',(0.0216293956773392,-0.00025039306212543,0.999766025901034));
#21503=DIRECTION('center_axis',(0.999769839441945,-1.4088563379705E-5,-0.0214538561508182));
#21504=DIRECTION('ref_axis',(0.0214538329403548,-0.000954360151552805,0.999769384532687));
#21505=DIRECTION('center_axis',(0.999770360412419,9.34322212250805E-6,-0.0214295672734342));
#21506=DIRECTION('ref_axis',(0.0214295545404625,0.000738176847933698,0.999770088213855));
#21507=DIRECTION('center_axis',(0.999766031866939,9.65877267560661E-6,-0.0216305670693989));
#21508=DIRECTION('ref_axis',(0.0216305539828126,0.000740752816224304,0.999765757775121));
#21509=DIRECTION('center_axis',(0.999763744304182,-3.6972435022485E-6,-0.021736042906044));
#21510=DIRECTION('ref_axis',(0.021736041333449,-0.000246635043159153,0.999763713923598));
#21511=DIRECTION('center_axis',(0.999763970269845,-7.60123828743992E-6,
-0.0217256459627287));
#21512=DIRECTION('ref_axis',(0.0217256434705418,-0.000243365665931261,0.999763940732483));
#21513=DIRECTION('center_axis',(-0.861920942122417,0.0166890382046472,-0.506767960248681));
#21514=DIRECTION('ref_axis',(-0.506838548513134,-4.00833851573235E-18,0.862041000034859));
#21515=DIRECTION('center_axis',(-0.871379853789596,0.0464998923150909,0.488400358747111));
#21516=DIRECTION('ref_axis',(0.48892923596368,1.37760753029074E-17,0.872323450458585));
#21517=DIRECTION('center_axis',(0.9997889250661,0.00124823490811798,0.0205072481036904));
#21518=DIRECTION('ref_axis',(0.0205072640797821,-9.63206510880043E-20,-0.999789703947766));
#21519=DIRECTION('center_axis',(0.999793850535689,-0.000926913239675538,
0.0202829303323548));
#21520=DIRECTION('ref_axis',(0.0202829390455843,-1.54023260780225E-20,-0.999794280031484));
#21521=DIRECTION('center_axis',(-0.888474164973873,-0.110685117325802,-0.44537901048046));
#21522=DIRECTION('ref_axis',(0.458638632717905,-0.248526491485849,-0.8531618765559));
#21523=DIRECTION('center_axis',(0.999791013008113,0.00102608806371862,0.0204175770231834));
#21524=DIRECTION('ref_axis',(0.0204175877715834,1.36199942924005E-20,-0.999791539326869));
#21525=DIRECTION('center_axis',(0.999794530784448,-0.000804757388187486,
0.0202545940233657));
#21526=DIRECTION('ref_axis',(0.0202546005821554,-4.98364828404734E-20,-0.999794854535298));
#21527=DIRECTION('center_axis',(0.999791115031614,0.000948396434230425,
0.020416337772641));
#21528=DIRECTION('ref_axis',(0.0204163469544439,-1.5274753026493E-20,-0.999791564665874));
#21529=DIRECTION('center_axis',(0.999793613160936,-0.000803410291055622,
0.0202998919825738));
#21530=DIRECTION('ref_axis',(0.0202998985340433,-3.79381199126813E-21,-0.999793935828532));
#21531=DIRECTION('center_axis',(0.999787734476799,0.00112360919993097,0.0205723963630029));
#21532=DIRECTION('ref_axis',(0.0205724093493161,-5.07154029360286E-20,-0.999788365592221));
#21533=DIRECTION('center_axis',(0.999793368904827,-0.00075256783557933,
0.020313865599363));
#21534=DIRECTION('ref_axis',(0.0203138713518291,-8.43310052312757E-21,-0.999793652025607));
#21535=DIRECTION('center_axis',(0.999796830831292,0.00103544519085822,0.0201301990293868));
#21536=DIRECTION('ref_axis',(0.0201302098206591,-8.26905179960667E-20,-0.99979736679618));
#21537=DIRECTION('center_axis',(0.999798400909155,-0.000959085530652312,
0.0200558643404188));
#21538=DIRECTION('ref_axis',(0.020055873564569,-8.57107583407826E-20,-0.99979886073928));
#21539=DIRECTION('center_axis',(0.999791828846322,0.000690509182037432,
0.0203917181521609));
#21540=DIRECTION('ref_axis',(0.0203917230135781,1.36073098268412E-20,-0.999792067198244));
#21541=DIRECTION('center_axis',(0.999798557733554,-0.000222129791565017,
0.0200697437019374));
#21542=DIRECTION('ref_axis',(0.0200697441970745,8.00806346724806E-22,-0.999798582399407));
#21543=DIRECTION('center_axis',(0.999807998093897,0.00102627949949861,0.0195681807499801));
#21544=DIRECTION('ref_axis',(0.0195681910550776,1.13196871364439E-20,-0.999808524618005));
#21545=DIRECTION('center_axis',(0.999793956365789,-0.00183064297990715,
0.0202161707730065));
#21546=DIRECTION('ref_axis',(0.0202162046478504,2.20102616963072E-20,-0.999795631651607));
#21547=DIRECTION('center_axis',(0.999782564221964,0.00141848170254525,0.0208041387087796));
#21548=DIRECTION('ref_axis',(0.0208041596387145,-5.80397643032026E-20,-0.999783570049902));
#21549=DIRECTION('center_axis',(0.999794149235583,-0.0006263178055023,0.0202797159818387));
#21550=DIRECTION('ref_axis',(0.0202797199594425,-3.1734126612677E-20,-0.999794345332262));
#21551=DIRECTION('center_axis',(0.999791678956523,0.0011207187498946,0.0203799577718084));
#21552=DIRECTION('ref_axis',(0.0203799705705411,-1.6022026816592E-21,-0.999792306831546));
#21553=DIRECTION('center_axis',(0.999794376483078,-0.000960029259732881,
0.0202554460981016));
#21554=DIRECTION('ref_axis',(0.0202554554323866,1.86296831220422E-20,-0.999794837216729));
#21555=DIRECTION('center_axis',(0.99979286009161,0.00110736634622207,0.0203226634478307));
#21556=DIRECTION('ref_axis',(0.0203226759082791,-1.33088630109754E-19,-0.999793473095282));
#21557=DIRECTION('center_axis',(0.999791633273466,-0.00123760086048944,
0.0203754357127787));
#21558=DIRECTION('ref_axis',(0.0203754513168747,2.79319123752651E-20,-0.999792398942717));
#21559=DIRECTION('center_axis',(0.999793659198503,0.00112258096642959,0.0202824761417586));
#21560=DIRECTION('ref_axis',(0.0202824889216375,8.64084697903419E-20,-0.999794289163098));
#21561=DIRECTION('center_axis',(0.999795640224913,-0.00101430853326898,
0.0201903186070843));
#21562=DIRECTION('ref_axis',(0.0201903289932123,-8.52295535382801E-20,-0.999796154531085));
#21563=DIRECTION('center_axis',(0.999797937496759,0.00087548785669098,0.0200827711793035));
#21564=DIRECTION('ref_axis',(0.020082778875819,-2.87508323961054E-20,-0.999798320659034));
#21565=DIRECTION('center_axis',(0.999788371198081,-0.00162444407414253,
0.0205079008808463));
#21566=DIRECTION('ref_axis',(0.0205079279392145,3.37598965323948E-21,-0.999789690330741));
#21567=DIRECTION('center_axis',(0.999809454916367,0.00101543101890164,0.0194941724544518));
#21568=DIRECTION('ref_axis',(0.0194941825046817,8.09901741121448E-20,-0.999809970368607));
#21569=DIRECTION('center_axis',(0.999813094544414,-0.000821842795898232,
0.0193158109314898));
#21570=DIRECTION('ref_axis',(0.0193158174546895,7.39417849148241E-20,-0.999813432194256));
#21571=DIRECTION('center_axis',(-0.894413399787221,-0.108947147830865,-0.433768589527394));
#21572=DIRECTION('ref_axis',(0.446107570363565,-0.286335917882665,-0.847938546001188));
#21573=DIRECTION('center_axis',(0.999275730732793,-0.0377336078180166,-0.00491821202049895));
#21574=DIRECTION('ref_axis',(0.0377340641918212,0.999287816597184,1.18406610643697E-20));
#21575=DIRECTION('center_axis',(0.9993238879154,0.0365809086693469,-0.00368838210782324));
#21576=DIRECTION('ref_axis',(-0.0365811574982001,0.999330685467074,5.68996066554659E-19));
#21577=DIRECTION('center_axis',(-0.9071068036828,-0.0997526098957014,-0.408909114023362));
#21578=DIRECTION('ref_axis',(0.420735592379569,-0.187704192648809,-0.887552081495544));
#21579=DIRECTION('center_axis',(-0.892779367153904,0.107912754414502,-0.437378370543114));
#21580=DIRECTION('ref_axis',(0.450437289746274,0.229260614961514,-0.862870684652979));
#21581=DIRECTION('center_axis',(-0.906179467397534,0.100126013659033,-0.410869266623671));
#21582=DIRECTION('ref_axis',(0.422740553915488,0.188359688277069,-0.88645984224182));
#21583=DIRECTION('center_axis',(-0.888442770560192,0.11072537147098,0.445431628369544));
#21584=DIRECTION('ref_axis',(0.458700410018584,0.248506250715052,0.853134559846412));
#21585=DIRECTION('center_axis',(0.999788900090079,-0.00125025659902504,
-0.0205083425733733));
#21586=DIRECTION('ref_axis',(0.0202248090182454,0.2357985529214,0.971591477700556));
#21587=DIRECTION('center_axis',(0.999793881909161,0.000924798772571727,
-0.020281480326686));
#21588=DIRECTION('ref_axis',(0.0199249195804614,-0.236470906870714,0.971434252939155));
#21589=DIRECTION('center_axis',(0.999791009341069,-0.00102657885440262,
-0.0204177319167002));
#21590=DIRECTION('ref_axis',(0.0200915076707316,0.233881095299282,0.972057593242872));
#21591=DIRECTION('center_axis',(0.999794553926456,0.000803250983560136,
-0.0202535114697604));
#21592=DIRECTION('ref_axis',(0.0198773395977057,-0.234440014181946,0.971927348684502));
#21593=DIRECTION('center_axis',(0.999791136401335,-0.000947056551401116,
-0.020415353467797));
#21594=DIRECTION('ref_axis',(0.0200780696682136,0.231986423030301,0.972511784323462));
#21595=DIRECTION('center_axis',(0.999793638354371,0.000801760735019295,
-0.0202987163597241));
#21596=DIRECTION('ref_axis',(0.0199289344184095,-0.232475550901422,0.972398043913102));
#21597=DIRECTION('center_axis',(0.999787777679922,-0.00112074158813577,
-0.0205704530853312));
#21598=DIRECTION('ref_axis',(0.0202762490552125,0.230120557335461,0.972950873793671));
#21599=DIRECTION('center_axis',(0.999793364511817,0.000753129469705107,
-0.0203140609958707));
#21600=DIRECTION('ref_axis',(0.019940463145563,-0.230537759819647,0.972859043863436));
#21601=DIRECTION('center_axis',(0.999797269820169,-0.00100281307594856,
-0.0201100379430304));
#21602=DIRECTION('ref_axis',(0.0197388213428965,0.245971495490712,0.969076056013178));
#21603=DIRECTION('center_axis',(0.999798569975224,0.000946215735264768,
-0.0200480460713516));
#21604=DIRECTION('ref_axis',(0.0196627093866498,-0.246479167651138,0.968948604299309));
#21605=DIRECTION('center_axis',(0.999791885662076,-0.000686562352684949,
-0.0203890656089599));
#21606=DIRECTION('ref_axis',(0.0200146371369503,0.226504667176284,0.973804420840056));
#21607=DIRECTION('center_axis',(0.99979855577085,0.000222511329138727,-0.0200698372497246));
#21608=DIRECTION('ref_axis',(0.0195979526674169,-0.226653390542104,0.973778291402624));
#21609=DIRECTION('center_axis',(0.999808251227011,-0.0010122534972086,-0.0195559740551144));
#21610=DIRECTION('ref_axis',(0.019561740686774,0.097217177687249,0.995070931473646));
#21611=DIRECTION('center_axis',(0.999793794637041,0.00183980383449,-0.0202233362014672));
#21612=DIRECTION('ref_axis',(0.0203061294301529,-0.0989747175626273,0.994882740020634));
#21613=DIRECTION('center_axis',(0.999782618994953,-0.0014149149279061,-0.0208017492374791));
#21614=DIRECTION('ref_axis',(0.0205754110187433,0.228287297878377,0.973376372267582));
#21615=DIRECTION('center_axis',(0.999794150030209,0.00062648588613381,-0.0202796716148505));
#21616=DIRECTION('ref_axis',(0.0198859134073932,-0.228587973036081,0.973320136969954));
#21617=DIRECTION('center_axis',(0.999791628136578,-0.0011246887331621,-0.0203822320481515));
#21618=DIRECTION('ref_axis',(0.0200651399814408,0.237752804753668,0.971118424286806));
#21619=DIRECTION('center_axis',(0.999794411622241,0.000957621136659537,
-0.0202538255817547));
#21620=DIRECTION('ref_axis',(0.0198979725293028,-0.238433414014752,0.970954982360404));
#21621=DIRECTION('center_axis',(0.999792754982158,-0.00111540024855146,
-0.0203273945077252));
#21622=DIRECTION('ref_axis',(0.0200019923075789,0.239729634175733,0.970633619241419));
#21623=DIRECTION('center_axis',(0.999791681155371,0.00123430342639552,-0.0203732861259386));
#21624=DIRECTION('ref_axis',(0.0200723578644585,-0.240436401635085,0.970457334053658));
#21625=DIRECTION('center_axis',(0.999793307262561,-0.00114897474535068,
-0.0202983400805286));
#21626=DIRECTION('ref_axis',(0.0199739827107701,0.241749830888139,0.970133011127972));
#21627=DIRECTION('center_axis',(0.999795700732705,0.00100994630042123,-0.0201875408326533));
#21628=DIRECTION('ref_axis',(0.0198300396982846,-0.242451180930935,0.969960924156617));
#21629=DIRECTION('center_axis',(0.999796612386705,-0.00097684807480299,
-0.0201439724956925));
#21630=DIRECTION('ref_axis',(0.0197741222240788,0.243832457525914,0.969615757270446));
#21631=DIRECTION('center_axis',(0.999788470786211,0.00161750735550819,-0.0205035936588081));
#21632=DIRECTION('ref_axis',(0.020276847625652,-0.24446333162905,0.969446506486661));
#21633=DIRECTION('center_axis',(0.999809561437771,-0.00100976586465744,
-0.0194890028095292));
#21634=DIRECTION('ref_axis',(0.0194928865433859,0.0993568624144647,0.994860915538127));
#21635=DIRECTION('center_axis',(0.999813090956489,0.000822563171989843,
-0.0193159659830663));
#21636=DIRECTION('ref_axis',(0.019299902172773,-0.101315362126067,0.994667135866761));
#21637=DIRECTION('center_axis',(-0.894513307027751,0.108908998607699,0.433572108849894));
#21638=DIRECTION('ref_axis',(0.445950796796345,0.285094269409663,0.848439240244389));
#21639=DIRECTION('center_axis',(0.999275539368059,0.0377381791903952,0.00492201707314082));
#21640=DIRECTION('ref_axis',(-0.0377386363260221,0.999287643938547,1.44659142945742E-19));
#21641=DIRECTION('center_axis',(0.999323945968658,-0.0365793722937842,0.00368789048421688));
#21642=DIRECTION('ref_axis',(0.0365796210458605,0.99933074170874,5.48310762901686E-20));
#21643=DIRECTION('center_axis',(-0.899913319397339,0.103764596224201,0.423543299016396));
#21644=DIRECTION('ref_axis',(0.435882629579717,0.185666942346874,0.880644150466142));
#21645=DIRECTION('center_axis',(-0.892850412212971,-0.107873925346478,0.437242904621071));
#21646=DIRECTION('ref_axis',(0.450296527273034,-0.22926177676768,0.862943842459735));
#21647=DIRECTION('center_axis',(-0.902455495465162,-0.102686894907543,0.418365247503871));
#21648=DIRECTION('ref_axis',(0.430605675709258,-0.18716164862259,0.882920873766074));
#21649=DIRECTION('center_axis',(-0.0158981576952788,0.585858710763356,0.81025725520022));
#21650=DIRECTION('ref_axis',(-0.128366775809462,-0.804849591107076,0.579429984176739));
#21651=DIRECTION('center_axis',(0.964785017122322,-0.0707010746474826,0.253359879973077));
#21652=DIRECTION('ref_axis',(0.253995491527146,0.,-0.967205402323562));
#21653=DIRECTION('center_axis',(-0.4517890859873,0.439366663897523,0.776430007430368));
#21654=DIRECTION('ref_axis',(0.864325114912213,0.,0.502933490366261));
#21655=DIRECTION('center_axis',(0.99979575798624,-0.00165747969236773,0.0201418736414786));
#21656=DIRECTION('ref_axis',(0.0201419013088053,-6.91947263585986E-21,-0.999797131327984));
#21657=DIRECTION('center_axis',(0.957670107909995,-0.0378387209059063,0.285370278087721));
#21658=DIRECTION('ref_axis',(0.285574789854396,0.,-0.958356426075193));
#21659=DIRECTION('center_axis',(-0.0157867627303391,0.591490281443045,0.806157568395238));
#21660=DIRECTION('ref_axis',(0.,-0.806258043227403,0.591564001382031));
#21661=DIRECTION('center_axis',(-0.574815246048694,-0.372435393183957,0.72861465179743));
#21662=DIRECTION('ref_axis',(0.785095927168427,0.,0.619374188309093));
#21663=DIRECTION('center_axis',(-0.0158858783442597,-0.585584495916129,
0.81045569713087));
#21664=DIRECTION('ref_axis',(-0.103891727389854,0.807137326320615,0.581150449918059));
#21665=DIRECTION('center_axis',(0.965326993626903,0.0677101640932514,0.252109359313991));
#21666=DIRECTION('ref_axis',(0.252689272754282,0.,-0.967547482780516));
#21667=DIRECTION('center_axis',(0.999814819167062,0.000554045269651598,
0.0192359145292012));
#21668=DIRECTION('ref_axis',(0.0192359174815893,-7.65610025019835E-21,-0.999814972621755));
#21669=DIRECTION('center_axis',(0.966303505500391,0.0721331810984261,0.24709176320201));
#21670=DIRECTION('ref_axis',(0.247737116134259,0.,-0.968827291775722));
#21671=DIRECTION('center_axis',(0.0157842736068064,-0.591588197507761,0.806085765459373));
#21672=DIRECTION('ref_axis',(0.,-0.806186199657785,-0.591661906397004));
#21673=DIRECTION('center_axis',(-0.0157863871158359,-0.591180316731151,
0.806384910009783));
#21674=DIRECTION('ref_axis',(0.0315820058328888,0.80578818841723,0.591361118365801));
#21675=DIRECTION('center_axis',(0.966378069659036,-0.0724684750264558,-0.246701736129714));
#21676=DIRECTION('ref_axis',(-0.247352098144654,0.,-0.968925662547668));
#21677=DIRECTION('center_axis',(0.999814852905107,-0.000552632782769883,
-0.01923420150011));
#21678=DIRECTION('ref_axis',(0.0192033195060585,0.092118786496819,0.995562836637799));
#21679=DIRECTION('center_axis',(0.965531741233883,-0.0685504202901476,-0.251096189831526));
#21680=DIRECTION('ref_axis',(-0.251688247883278,0.,-0.967808362165489));
#21681=DIRECTION('center_axis',(0.0158782835274792,-0.586533726279538,0.809769144910363));
#21682=DIRECTION('ref_axis',(-0.123819524012861,-0.804790948205936,-0.5805000044436));
#21683=DIRECTION('center_axis',(0.438823103950365,-0.445656359684007,0.780272191297733));
#21684=DIRECTION('ref_axis',(0.,-0.868345456619373,-0.495959845117014));
#21685=DIRECTION('center_axis',(0.0157906183176418,0.591381310212439,0.806237435439812));
#21686=DIRECTION('ref_axis',(0.0301303812059224,0.805690346002935,-0.591570136573895));
#21687=DIRECTION('center_axis',(0.965712986386173,0.0749508725835839,-0.248557427215642));
#21688=DIRECTION('ref_axis',(-0.249258534766396,0.,-0.968436979284718));
#21689=DIRECTION('center_axis',(0.999796052573138,0.00164189776482789,-0.0201285228196576));
#21690=DIRECTION('ref_axis',(0.020193557109576,-0.0946575785765395,0.995305060305276));
#21691=DIRECTION('center_axis',(0.526294582686482,0.401383271747728,0.749603549481958));
#21692=DIRECTION('ref_axis',(0.818424732890698,0.,-0.57461374556548));
#21693=DIRECTION('center_axis',(0.964696696273675,0.0703284210564187,-0.253799522045191));
#21694=DIRECTION('ref_axis',(-0.254429517253042,0.,-0.967091319757542));
#21695=DIRECTION('center_axis',(0.0158966842261725,0.585482599575022,0.810529099431654));
#21696=DIRECTION('ref_axis',(-0.114192359427942,0.806390651605264,-0.580253584264602));
#25844=CARTESIAN_POINT('',(0.,0.,0.));
#25845=CARTESIAN_POINT('Ctrl Pts',(-0.185819463593633,0.0166104930553049,
0.00236863820262676));
#25846=CARTESIAN_POINT('Ctrl Pts',(-0.203223508587672,0.0164247592890707,
0.00234416866113263));
#25847=CARTESIAN_POINT('Ctrl Pts',(-0.220627582451438,0.0162418056983084,
0.00231971009381821));
#25848=CARTESIAN_POINT('Ctrl Pts',(-0.238031675744303,0.0160611171225611,
0.00229373846137714));
#25849=CARTESIAN_POINT('Ctrl Pts',(-0.18581926440362,0.0166461165277183,
0.00221607060080922));
#25850=CARTESIAN_POINT('Ctrl Pts',(-0.203223313044138,0.0164497831264032,
0.00218726310900855));
#25851=CARTESIAN_POINT('Ctrl Pts',(-0.220627389279833,0.0162559154123599,
0.00215868502272393));
#25852=CARTESIAN_POINT('Ctrl Pts',(-0.238031485810861,0.0160641905057161,
0.0021289558365353));
#25853=CARTESIAN_POINT('Ctrl Pts',(-0.185818880874426,0.0167106984888996,
0.00190682671781972));
#25854=CARTESIAN_POINT('Ctrl Pts',(-0.203222934036142,0.0164938099422013,
0.00186885154579339));
#25855=CARTESIAN_POINT('Ctrl Pts',(-0.220627006269502,0.016278128585195,
0.00183193650018925));
#25856=CARTESIAN_POINT('Ctrl Pts',(-0.238031099947329,0.0160640878015832,
0.00179531454904686));
#25857=CARTESIAN_POINT('Ctrl Pts',(-0.185818335405062,0.0168157482814852,
0.00126613919744405));
#25858=CARTESIAN_POINT('Ctrl Pts',(-0.203222383696577,0.0165663597906042,
0.00122992539721983));
#25859=CARTESIAN_POINT('Ctrl Pts',(-0.220626440719063,0.016317358802535,
0.00119476376827596));
#25860=CARTESIAN_POINT('Ctrl Pts',(-0.238030512988197,0.0160691276034975,
0.00116079870997399));
#25861=CARTESIAN_POINT('Ctrl Pts',(-0.185817827209109,0.0169242355148058,
9.8641936611403E-5));
#25862=CARTESIAN_POINT('Ctrl Pts',(-0.203221858920215,0.0166409437466787,
9.11218039920294E-5));
#25863=CARTESIAN_POINT('Ctrl Pts',(-0.220625885580743,0.0163575362327447,
8.39196676156386E-5));
#25864=CARTESIAN_POINT('Ctrl Pts',(-0.238029902001653,0.0160736640759679,
7.73368998092213E-5));
#25865=CARTESIAN_POINT('Ctrl Pts',(-0.185818130580629,0.0168405937503755,
-0.00127155898818726));
#25866=CARTESIAN_POINT('Ctrl Pts',(-0.20322218710562,0.0165814424082619,
-0.00122048351610829));
#25867=CARTESIAN_POINT('Ctrl Pts',(-0.220626248932598,0.0163217805675101,
-0.0011714081373514));
#25868=CARTESIAN_POINT('Ctrl Pts',(-0.238030331796423,0.0160627645050436,
-0.00112492380137579));
#25869=CARTESIAN_POINT('Ctrl Pts',(-0.185819629874682,0.0165908497836556,
-0.00251327778772927));
#25870=CARTESIAN_POINT('Ctrl Pts',(-0.203223673996629,0.0164148787644927,
-0.00249147144795656));
#25871=CARTESIAN_POINT('Ctrl Pts',(-0.220627751907747,0.0162423115134214,
-0.00246930645840148));
#25872=CARTESIAN_POINT('Ctrl Pts',(-0.238031849291733,0.0160723190230807,
-0.00244485415145052));
#25873=CARTESIAN_POINT('Ctrl Pts',(-0.185821321884765,0.016234179304769,
-0.00369798898814236));
#25874=CARTESIAN_POINT('Ctrl Pts',(-0.203225319480993,0.0161450945583953,
-0.00371151425360031));
#25875=CARTESIAN_POINT('Ctrl Pts',(-0.220629323053567,0.0160579626760164,
-0.0037253545768972));
#25876=CARTESIAN_POINT('Ctrl Pts',(-0.238033334942443,0.0159726607261184,
-0.00373864195256771));
#25877=CARTESIAN_POINT('Ctrl Pts',(-0.185823245401148,0.0155679236134438,
-0.00510694903431088));
#25878=CARTESIAN_POINT('Ctrl Pts',(-0.203227224653483,0.0155630775790093,
-0.00518221799309441));
#25879=CARTESIAN_POINT('Ctrl Pts',(-0.220631203569159,0.0155602580016752,
-0.00525755181874107));
#25880=CARTESIAN_POINT('Ctrl Pts',(-0.238035184380882,0.0155591988240479,
-0.00533210507472633));
#25881=CARTESIAN_POINT('Ctrl Pts',(-0.185825309557818,0.0144549166529026,
-0.00659829769408909));
#25882=CARTESIAN_POINT('Ctrl Pts',(-0.203229286524981,0.0145155596341981,
-0.00676015088892623));
#25883=CARTESIAN_POINT('Ctrl Pts',(-0.22063325576454,0.0145775956365756,
-0.00692214625038456));
#25884=CARTESIAN_POINT('Ctrl Pts',(-0.238037222353744,0.0146408934228599,
-0.00708388886226514));
#25885=CARTESIAN_POINT('Ctrl Pts',(-0.185827024933535,0.0130736100782548,
-0.00784141832828519));
#25886=CARTESIAN_POINT('Ctrl Pts',(-0.203231018325486,0.0131627927804585,
-0.00809004931086922));
#25887=CARTESIAN_POINT('Ctrl Pts',(-0.220635004750871,0.0132529981228345,
-0.00833876091410667));
#25888=CARTESIAN_POINT('Ctrl Pts',(-0.238038987871232,0.0133440928006999,
-0.00858734922546909));
#25889=CARTESIAN_POINT('Ctrl Pts',(-0.18582832438757,0.0114765605098063,
-0.00878674958056091));
#25890=CARTESIAN_POINT('Ctrl Pts',(-0.203232338232321,0.0115609317972438,
-0.00910975493295771));
#25891=CARTESIAN_POINT('Ctrl Pts',(-0.220636347717917,0.011645972461393,
-0.00943280869850027));
#25892=CARTESIAN_POINT('Ctrl Pts',(-0.238040354954934,0.011731574352546,
-0.00975583575545302));
#25893=CARTESIAN_POINT('Ctrl Pts',(-0.185829453345315,0.0091451966229997,
-0.0096057242773119));
#25894=CARTESIAN_POINT('Ctrl Pts',(-0.203233491880005,0.00919013323193661,
-0.00999827176177371));
#25895=CARTESIAN_POINT('Ctrl Pts',(-0.220637530309762,0.00923531471374497,
-0.010390817424762));
#25896=CARTESIAN_POINT('Ctrl Pts',(-0.23804156864792,0.00928068353228921,
-0.0107833654056958));
#25897=CARTESIAN_POINT('Ctrl Pts',(-0.185829632293992,0.00601552622584051,
-0.00973743542872093));
#25898=CARTESIAN_POINT('Ctrl Pts',(-0.203233675322875,0.00597352188698778,
-0.0101422781507738));
#25899=CARTESIAN_POINT('Ctrl Pts',(-0.220637719137517,0.00593129183613322,
-0.0105471134497117));
#25900=CARTESIAN_POINT('Ctrl Pts',(-0.238041763362071,0.00588889329790392,
-0.0109519477983446));
#25901=CARTESIAN_POINT('Ctrl Pts',(-0.185828144842012,0.0030739290209801,
-0.00865481883805552));
#25902=CARTESIAN_POINT('Ctrl Pts',(-0.203232153522101,0.0029784477533647,
-0.00896475560878426));
#25903=CARTESIAN_POINT('Ctrl Pts',(-0.22063615670017,0.00288224573504626,
-0.00927474912637149));
#25904=CARTESIAN_POINT('Ctrl Pts',(-0.23804015699596,0.00278543581335185,
-0.00958473005637672));
#25905=CARTESIAN_POINT('Ctrl Pts',(-0.185826082022641,0.00110130832095057,
-0.00715935834428723));
#25906=CARTESIAN_POINT('Ctrl Pts',(-0.203230064435315,0.00102431113527,
-0.00735889669894074));
#25907=CARTESIAN_POINT('Ctrl Pts',(-0.220634039193033,0.000946044449726581,
-0.00755853937500263));
#25908=CARTESIAN_POINT('Ctrl Pts',(-0.238038010705833,0.000866655562235164,
-0.00775795997137017));
#25909=CARTESIAN_POINT('Ctrl Pts',(-0.185824164055499,-0.00013244480670859,
-0.0057658502018965));
#25910=CARTESIAN_POINT('Ctrl Pts',(-0.20322813912978,-0.000160334959886128,
-0.00587671276434198));
#25911=CARTESIAN_POINT('Ctrl Pts',(-0.220632108537853,-0.000189837833944718,
-0.0059877445582653));
#25912=CARTESIAN_POINT('Ctrl Pts',(-0.238036077190852,-0.000220820008254192,
-0.00609839080888522));
#25913=CARTESIAN_POINT('Ctrl Pts',(-0.185822299173595,-0.000912009378582172,
-0.00442360049681092));
#25914=CARTESIAN_POINT('Ctrl Pts',(-0.203226287658242,-0.000866786568362782,
-0.00446783414154759));
#25915=CARTESIAN_POINT('Ctrl Pts',(-0.220630281624252,-0.00082387334949089,
-0.00451207377872994));
#25916=CARTESIAN_POINT('Ctrl Pts',(-0.23803428087264,-0.000782904229550054,
-0.00455527877134414));
#25917=CARTESIAN_POINT('Ctrl Pts',(-0.185820718130017,-0.00137009218103609,
-0.00326760896710645));
#25918=CARTESIAN_POINT('Ctrl Pts',(-0.203224730158278,-0.00125053240292857,
-0.00326719962044019));
#25919=CARTESIAN_POINT('Ctrl Pts',(-0.220628754805288,-0.00113312156821255,
-0.00326706607813972));
#25920=CARTESIAN_POINT('Ctrl Pts',(-0.23803279135031,-0.00101767765869665,
-0.00326612878115765));
#25921=CARTESIAN_POINT('Ctrl Pts',(-0.185819647933685,-0.00158153457958364,
-0.00252531449976026));
#25922=CARTESIAN_POINT('Ctrl Pts',(-0.203223692052988,-0.00140575636354931,
-0.00250567473614365));
#25923=CARTESIAN_POINT('Ctrl Pts',(-0.220627772291069,-0.00123370234183487,
-0.00248543365897305));
#25924=CARTESIAN_POINT('Ctrl Pts',(-0.238031871675392,-0.001064293369006,
-0.00246259728183289));
#25925=CARTESIAN_POINT('Ctrl Pts',(-0.185818880874262,-0.00171069848643351,
-0.00190682671492207));
#25926=CARTESIAN_POINT('Ctrl Pts',(-0.203222934035982,-0.0014938099322336,
-0.00186885153402852));
#25927=CARTESIAN_POINT('Ctrl Pts',(-0.220627006269333,-0.00127812856598612,
-0.00183193647922556));
#25928=CARTESIAN_POINT('Ctrl Pts',(-0.238031099947143,-0.00106408777175675,
-0.00179531451994465));
#25929=CARTESIAN_POINT('Ctrl Pts',(-0.185818335405171,-0.0018157482831674,
-0.00126613919912989));
#25930=CARTESIAN_POINT('Ctrl Pts',(-0.203222383696684,-0.00156635979742609,
-0.00122992540382135));
#25931=CARTESIAN_POINT('Ctrl Pts',(-0.220626440719173,-0.00131735881546124,
-0.00119476377996408));
#25932=CARTESIAN_POINT('Ctrl Pts',(-0.238030512988314,-0.00106912762331005,
-0.00116079872610497));
#25933=CARTESIAN_POINT('Ctrl Pts',(-0.185817827208834,-0.00192423551004945,
-9.86419358357781E-5));
#25934=CARTESIAN_POINT('Ctrl Pts',(-0.203221858919953,-0.00164094372766557,
-9.11218007194661E-5));
#25935=CARTESIAN_POINT('Ctrl Pts',(-0.220625885580502,-0.00135753619911081,
-8.39196619480522E-5));
#25936=CARTESIAN_POINT('Ctrl Pts',(-0.238029902001436,-0.00107366402718548,
-7.73368926939811E-5));
#25937=CARTESIAN_POINT('Ctrl Pts',(-0.185818130581901,-0.00184059377323484,
0.00127155899038818));
#25938=CARTESIAN_POINT('Ctrl Pts',(-0.20322218710682,-0.00158144249928501,
0.00122048352511737));
#25939=CARTESIAN_POINT('Ctrl Pts',(-0.220626248933645,-0.00132178072462663,
0.0011714081546043));
#25940=CARTESIAN_POINT('Ctrl Pts',(-0.238030331797288,-0.00106276472807202,
0.00112492383001885));
#25941=CARTESIAN_POINT('Ctrl Pts',(-0.185819629872525,-0.00159084974486086,
0.00251327778358106));
#25942=CARTESIAN_POINT('Ctrl Pts',(-0.203223673994595,-0.00141487860996912,
0.00249147143135548));
#25943=CARTESIAN_POINT('Ctrl Pts',(-0.220627751905974,-0.00124231124688325,
0.00246930642685937));
#25944=CARTESIAN_POINT('Ctrl Pts',(-0.238031849290273,-0.00107231864497727,
0.00244485409969644));
#25945=CARTESIAN_POINT('Ctrl Pts',(-0.185821321898498,-0.00123417951568875,
0.00369798917224086));
#25946=CARTESIAN_POINT('Ctrl Pts',(-0.203225319494204,-0.00114509540859564,
0.003711514992569));
#25947=CARTESIAN_POINT('Ctrl Pts',(-0.22062932306665,-0.00105796426044417,
0.00372535589828007));
#25948=CARTESIAN_POINT('Ctrl Pts',(-0.238033334955726,-0.000972663126262614,
0.00373864380762799));
#25949=CARTESIAN_POINT('Ctrl Pts',(-0.185823245436368,-0.000567924396732498,
0.00510694905821607));
#25950=CARTESIAN_POINT('Ctrl Pts',(-0.203227224690427,-0.000563080693363035,
0.00518221807967137));
#25951=CARTESIAN_POINT('Ctrl Pts',(-0.220631203607128,-0.000560263335972913,
0.00525755189961067));
#25952=CARTESIAN_POINT('Ctrl Pts',(-0.238035184419129,-0.000559206262722732,
0.00533210518716677));
#25953=CARTESIAN_POINT('Ctrl Pts',(-0.185825309451763,0.000545085685742881,
0.00659829745055551));
#25954=CARTESIAN_POINT('Ctrl Pts',(-0.203229286420574,0.000484449699432902,
0.00676014989093362));
#25955=CARTESIAN_POINT('Ctrl Pts',(-0.220633255665466,0.000422420785569872,
0.00692214425104443));
#25956=CARTESIAN_POINT('Ctrl Pts',(-0.238037222262465,0.000359130275923251,
0.00708388576133197));
#25957=CARTESIAN_POINT('Ctrl Pts',(-0.18582702479622,0.00192639486310074,
0.00784141870119505));
#25958=CARTESIAN_POINT('Ctrl Pts',(-0.203231018176613,0.00183722692142162,
0.00809005081566443));
#25959=CARTESIAN_POINT('Ctrl Pts',(-0.22063500458984,0.00174703627304292,
0.00833876365528797));
#25960=CARTESIAN_POINT('Ctrl Pts',(-0.238038987697963,0.00165595618969436,
0.00858735323957588));
#25961=CARTESIAN_POINT('Ctrl Pts',(-0.185828324413572,0.00352344076961579,
0.00878675040966002));
#25962=CARTESIAN_POINT('Ctrl Pts',(-0.203232338254504,0.00343907331273139,
0.00910975824932868));
#25963=CARTESIAN_POINT('Ctrl Pts',(-0.220636347734676,0.00335403651878359,
0.00943281459138894));
#25964=CARTESIAN_POINT('Ctrl Pts',(-0.238040354964937,0.00326843848901562,
0.00975584429234039));
#25965=CARTESIAN_POINT('Ctrl Pts',(-0.185829453384424,0.00585480099283502,
0.00960572462550227));
#25966=CARTESIAN_POINT('Ctrl Pts',(-0.203233491922009,0.00580985725942693,
0.00999827314311295));
#25967=CARTESIAN_POINT('Ctrl Pts',(-0.220637530355488,0.00576466867020715,
0.0103908197967745));
#25968=CARTESIAN_POINT('Ctrl Pts',(-0.238041568698001,0.00571929278241239,
0.01078336873748));
#25969=CARTESIAN_POINT('Ctrl Pts',(-0.185829632324535,0.00898447703279034,
0.00973743551044517));
#25970=CARTESIAN_POINT('Ctrl Pts',(-0.20323367535712,0.00902649110858287,
0.0101422784667701));
#25971=CARTESIAN_POINT('Ctrl Pts',(-0.220637719176512,0.00906873086433049,
0.0105471139309657));
#25972=CARTESIAN_POINT('Ctrl Pts',(-0.238041763406542,0.00911113903768637,
0.0109519484055942));
#25973=CARTESIAN_POINT('Ctrl Pts',(-0.185828144821879,0.0119260676124901,
0.00865481978154805));
#25974=CARTESIAN_POINT('Ctrl Pts',(-0.203232153491178,0.0120215388163693,
0.00896475940006844));
#25975=CARTESIAN_POINT('Ctrl Pts',(-0.220636156655006,0.0121177307814799,
0.00927475599174944));
#25976=CARTESIAN_POINT('Ctrl Pts',(-0.238040156934043,0.0122145307595023,
0.00958474013175701));
#25977=CARTESIAN_POINT('Ctrl Pts',(-0.185826081864447,0.0138986875060143,
0.0071593582727713));
#25978=CARTESIAN_POINT('Ctrl Pts',(-0.203230064272376,0.0139756722252048,
0.00735889640414339));
#25979=CARTESIAN_POINT('Ctrl Pts',(-0.22063403902823,0.0140539264607635,
0.00755853873522353));
#25980=CARTESIAN_POINT('Ctrl Pts',(-0.238038010541502,0.0141333028562059,
0.00775795890451245));
#25981=CARTESIAN_POINT('Ctrl Pts',(-0.185824164045733,0.0151324448001649,
0.00576585000582876));
#25982=CARTESIAN_POINT('Ctrl Pts',(-0.203228139124408,0.0151603349181088,
0.00587671195695743));
#25983=CARTESIAN_POINT('Ctrl Pts',(-0.220632108538343,0.0151898375748212,
0.00598774292639455));
#25984=CARTESIAN_POINT('Ctrl Pts',(-0.238036077197705,0.0152208192897305,
0.00609838833446442));
#25985=CARTESIAN_POINT('Ctrl Pts',(-0.185822299200829,0.01591200987427,
0.00442360064358258));
#25986=CARTESIAN_POINT('Ctrl Pts',(-0.203226287685109,0.0158667885469009,
0.00446783472845091));
#25987=CARTESIAN_POINT('Ctrl Pts',(-0.220630281650178,0.0158238768216512,
0.00451207481602829));
#25988=CARTESIAN_POINT('Ctrl Pts',(-0.238034280897302,0.0157829092105071,
0.00455528026393975));
#25989=CARTESIAN_POINT('Ctrl Pts',(-0.185820718137045,0.0163700922862437,
0.00326760909611432));
#25990=CARTESIAN_POINT('Ctrl Pts',(-0.203224730165169,0.0162505328296095,
0.00326720013800919));
#25991=CARTESIAN_POINT('Ctrl Pts',(-0.220628754812585,0.0161331223929292,
0.00326706699899929));
#25992=CARTESIAN_POINT('Ctrl Pts',(-0.238032791358368,0.016017678941859,
0.00326613005920909));
#25993=CARTESIAN_POINT('Ctrl Pts',(-0.18581986197366,0.0165392461104783,
0.00267377340626184));
#25994=CARTESIAN_POINT('Ctrl Pts',(-0.203223899674741,0.0163747116144059,
0.00265797976538081));
#25995=CARTESIAN_POINT('Ctrl Pts',(-0.220627968794648,0.0162135862702056,
0.00264176023600675));
#25996=CARTESIAN_POINT('Ctrl Pts',(-0.238032055611188,0.016054970356251,
0.00262330371106081));
#25997=CARTESIAN_POINT('Ctrl Pts',(-0.185819463593633,0.0166104930553049,
0.00236863820262676));
#25998=CARTESIAN_POINT('Ctrl Pts',(-0.203223508587672,0.0164247592890707,
0.00234416866113263));
#25999=CARTESIAN_POINT('Ctrl Pts',(-0.220627582451438,0.0162418056983084,
0.00231971009381821));
#26000=CARTESIAN_POINT('Ctrl Pts',(-0.238031675744303,0.0160611171225611,
0.00229373846137714));
#26001=CARTESIAN_POINT('',(-0.220091864350141,0.0162481906744713,0.00232003547938548));
#26002=CARTESIAN_POINT('',(-0.230613780455036,0.0161371732180366,0.00230566860537552));
#26003=CARTESIAN_POINT('Ctrl Pts',(-0.220091864350141,0.0162481906744713,
0.00232003547938548));
#26004=CARTESIAN_POINT('Ctrl Pts',(-0.223599172161426,0.0162114519962125,
0.0023149748956921));
#26005=CARTESIAN_POINT('Ctrl Pts',(-0.227106480893481,0.016174812491324,
0.00230987413069827));
#26006=CARTESIAN_POINT('Ctrl Pts',(-0.230613790469045,0.0161382679437046,
0.00230472071158295));
#26007=CARTESIAN_POINT('',(-0.21500029174819,0.0153240929662069,0.00555316308125546));
#26008=CARTESIAN_POINT('Ctrl Pts',(-0.220091864350141,0.0162481906744713,
0.00232003547938548));
#26009=CARTESIAN_POINT('Ctrl Pts',(-0.219964032121089,0.0162246503855585,
0.00259808795516262));
#26010=CARTESIAN_POINT('Ctrl Pts',(-0.219813080900817,0.0161920738263575,
0.002863235307656));
#26011=CARTESIAN_POINT('Ctrl Pts',(-0.219641753631267,0.016149773489234,
0.00311424188670563));
#26012=CARTESIAN_POINT('Ctrl Pts',(-0.219606803621251,0.0161411444063679,
0.00316544612567476));
#26013=CARTESIAN_POINT('Ctrl Pts',(-0.219571005329045,0.0161321311914261,
0.003216013187459));
#26014=CARTESIAN_POINT('Ctrl Pts',(-0.219534386818884,0.01612274284289,
0.00326596109874446));
#26015=CARTESIAN_POINT('Ctrl Pts',(-0.219355791305947,0.016076954062432,
0.00350956666317138));
#26016=CARTESIAN_POINT('Ctrl Pts',(-0.21915768525195,0.0160222778157506,
0.00373830735842303));
#26017=CARTESIAN_POINT('Ctrl Pts',(-0.218943331145544,0.0159637685900893,
0.00394877190880269));
#26018=CARTESIAN_POINT('Ctrl Pts',(-0.21885802655045,0.0159404841945253,
0.00403252861191818));
#26019=CARTESIAN_POINT('Ctrl Pts',(-0.218770149187462,0.0159165696614574,
0.00411347490234016));
#26020=CARTESIAN_POINT('Ctrl Pts',(-0.218679854877443,0.0158923302275234,
0.00419142907760536));
#26021=CARTESIAN_POINT('Ctrl Pts',(-0.218223322396706,0.0157697744551469,
0.00458556922896357));
#26022=CARTESIAN_POINT('Ctrl Pts',(-0.217705003227418,0.0156391436947526,
0.00490281618706478));
#26023=CARTESIAN_POINT('Ctrl Pts',(-0.217145035305693,0.0155351186744745,
0.00513162883065141));
#26024=CARTESIAN_POINT('Ctrl Pts',(-0.216474315366188,0.0154105192954726,
0.00540569667723717));
#26025=CARTESIAN_POINT('Ctrl Pts',(-0.215743833615192,0.0153264023738546,
0.00555341322890043));
#26026=CARTESIAN_POINT('Ctrl Pts',(-0.21500029174819,0.0153240929662069,
0.00555316308125546));
#26027=CARTESIAN_POINT('',(-0.192201188944086,0.015241534078835,0.00554549074872928));
#26028=CARTESIAN_POINT('Ctrl Pts',(-0.192201188944086,0.015241534078835,
0.00554549074872928));
#26029=CARTESIAN_POINT('Ctrl Pts',(-0.192678589700584,0.0152435315770371,
0.00554564496900607));
#26030=CARTESIAN_POINT('Ctrl Pts',(-0.193156755420166,0.0152455145072555,
0.00554579898090145));
#26031=CARTESIAN_POINT('Ctrl Pts',(-0.193630507624624,0.0152474620561553,
0.00554595109465557));
#26032=CARTESIAN_POINT('Ctrl Pts',(-0.194104259909824,0.0152494096053871,
0.00554610320843563));
#26033=CARTESIAN_POINT('Ctrl Pts',(-0.194573598676706,0.0152513221215489,
0.0055462536667817));
#26034=CARTESIAN_POINT('Ctrl Pts',(-0.195054059361393,0.0152532621127367,
0.00554640792672152));
#26035=CARTESIAN_POINT('Ctrl Pts',(-0.195294289703737,0.0152542321083306,
0.00554648505669144));
#26036=CARTESIAN_POINT('Ctrl Pts',(-0.195537300526605,0.015255208744483,
0.00554656298160729));
#26037=CARTESIAN_POINT('Ctrl Pts',(-0.195763672529165,0.0152561146772,0.00554663556632508));
#26038=CARTESIAN_POINT('Ctrl Pts',(-0.195990044531725,0.0152570206099169,
0.00554670815104287));
#26039=CARTESIAN_POINT('Ctrl Pts',(-0.196199777712581,0.0152578561399587,
0.00554677559870816));
#26040=CARTESIAN_POINT('Ctrl Pts',(-0.196410704370724,0.0152586930485431,
0.00554684374511567));
#26041=CARTESIAN_POINT('Ctrl Pts',(-0.19683255768701,0.0152603668657118,
0.00554698003793067));
#26042=CARTESIAN_POINT('Ctrl Pts',(-0.197259184915049,0.0152620456340052,
0.00554711874688127));
#26043=CARTESIAN_POINT('Ctrl Pts',(-0.197689893504854,0.0152637260387762,
0.00554725953304577));
#26044=CARTESIAN_POINT('Ctrl Pts',(-0.198551310684465,0.0152670868483182,
0.00554754110537476));
#26045=CARTESIAN_POINT('Ctrl Pts',(-0.199429053310939,0.0152704542694656,
0.00554783101954003));
#26046=CARTESIAN_POINT('Ctrl Pts',(-0.200323661272974,0.0152738264707178,
0.00554812786352896));
#26047=CARTESIAN_POINT('Ctrl Pts',(-0.201218269235009,0.01527719867197,
0.0055484247075179));
#26048=CARTESIAN_POINT('Ctrl Pts',(-0.2021297425327,0.0152805756302453,
0.00554872846691666));
#26049=CARTESIAN_POINT('Ctrl Pts',(-0.2030579484167,0.0152839525550071,
0.00554903797343471));
#26050=CARTESIAN_POINT('Ctrl Pts',(-0.204914360184699,0.0152907064045306,
0.00554965698647082));
#26051=CARTESIAN_POINT('Ctrl Pts',(-0.206837702298988,0.0152974601561509,
0.00555029886425079));
#26052=CARTESIAN_POINT('Ctrl Pts',(-0.208828081024599,0.0153041762029342,
0.00555096151666457));
#26053=CARTESIAN_POINT('Ctrl Pts',(-0.21081845965904,0.0153108922494098,
0.00555162416904801));
#26054=CARTESIAN_POINT('Ctrl Pts',(-0.212875874899139,0.015317570478775,
0.00555230751522824));
#26055=CARTESIAN_POINT('Ctrl Pts',(-0.215000291390286,0.0153241679289001,
0.00555302111108408));
#26056=CARTESIAN_POINT('',(-0.186146181814525,0.00833801480660534,0.00957679076147885));
#26057=CARTESIAN_POINT('Ctrl Pts',(-0.192201188668275,0.0152415940904861,
0.00554556725774743));
#26058=CARTESIAN_POINT('Ctrl Pts',(-0.191385429512063,0.0150388003056731,
0.00585256287769953));
#26059=CARTESIAN_POINT('Ctrl Pts',(-0.189924359857282,0.0144159207087289,
0.00669446943947488));
#26060=CARTESIAN_POINT('Ctrl Pts',(-0.188118588226452,0.0129535683023105,
0.0079971734865383));
#26061=CARTESIAN_POINT('Ctrl Pts',(-0.186728499480259,0.0109160101219197,
0.00909799313116123));
#26062=CARTESIAN_POINT('Ctrl Pts',(-0.186240928505495,0.00922649890739429,
0.00949868329865868));
#26063=CARTESIAN_POINT('Ctrl Pts',(-0.186146181814525,0.00833801480660534,
0.00957679076147885));
#26064=CARTESIAN_POINT('',(-0.237657867810474,0.00839975141101414,0.0107287568273012));
#26065=CARTESIAN_POINT('Ctrl Pts',(-0.186146188570675,0.00833798789827216,
0.00957649060684295));
#26066=CARTESIAN_POINT('Ctrl Pts',(-0.203316735846858,0.0083585159298715,
0.0099611404338935));
#26067=CARTESIAN_POINT('Ctrl Pts',(-0.220487282901184,0.00837917464529529,
0.0103457920140646));
#26068=CARTESIAN_POINT('Ctrl Pts',(-0.237657829826327,0.00839993762480588,
0.010730442320928));
#26069=CARTESIAN_POINT('',(-0.230843542079246,0.0161181318983597,0.00261043863931786));
#26070=CARTESIAN_POINT('Ctrl Pts',(-0.237657867810474,0.00839975141101414,
0.0107287568273012));
#26071=CARTESIAN_POINT('Ctrl Pts',(-0.237628040172413,0.00871804736541609,
0.0106932259604992));
#26072=CARTESIAN_POINT('Ctrl Pts',(-0.237583075320134,0.00903375586220757,
0.0106396630368088));
#26073=CARTESIAN_POINT('Ctrl Pts',(-0.237524354422287,0.00934381631424547,
0.0105697131231371));
#26074=CARTESIAN_POINT('Ctrl Pts',(-0.237409875404356,0.0099482930397302,
0.0104333426363938));
#26075=CARTESIAN_POINT('Ctrl Pts',(-0.237243104297146,0.0105312772939824,
0.0102346798484156));
#26076=CARTESIAN_POINT('Ctrl Pts',(-0.237034426717481,0.0110700480166096,
0.00998606499931368));
#26077=CARTESIAN_POINT('Ctrl Pts',(-0.236825749137817,0.0116088187392369,
0.00973745015021171));
#26078=CARTESIAN_POINT('Ctrl Pts',(-0.236575218375409,0.0121034354127291,
0.00943895128259336));
#26079=CARTESIAN_POINT('Ctrl Pts',(-0.236294502051235,0.0125537967820148,
0.00910454953732754));
#26080=CARTESIAN_POINT('Ctrl Pts',(-0.236015363399207,0.0130016270459575,
0.00877202718514883));
#26081=CARTESIAN_POINT('Ctrl Pts',(-0.235706378926574,0.013405701518213,
0.00840399539865004));
#26082=CARTESIAN_POINT('Ctrl Pts',(-0.235379076902145,0.0137658122240604,
0.00801408434478435));
#26083=CARTESIAN_POINT('Ctrl Pts',(-0.235377227013985,0.0137678475445937,
0.00801188059476749));
#26084=CARTESIAN_POINT('Ctrl Pts',(-0.235375376540491,0.0137698814606867,
0.00800967614545206));
#26085=CARTESIAN_POINT('Ctrl Pts',(-0.235373525482602,0.0137719139727705,
0.0080074709979345));
#26086=CARTESIAN_POINT('Ctrl Pts',(-0.234714805396164,0.0144952066067006,
0.00722274407358542));
#26087=CARTESIAN_POINT('Ctrl Pts',(-0.233982176786342,0.0150406056960837,
0.00634992635599267));
#26088=CARTESIAN_POINT('Ctrl Pts',(-0.233216594643784,0.0154272463887169,
0.00543780883209741));
#26089=CARTESIAN_POINT('Ctrl Pts',(-0.232451013528585,0.0158138865625047,
0.00452569253220128));
#26090=CARTESIAN_POINT('Ctrl Pts',(-0.231652435338367,0.0160415300380187,
0.00357419085672357));
#26091=CARTESIAN_POINT('Ctrl Pts',(-0.230843549352499,0.0161191166093656,
0.0026105069458129));
#26092=CARTESIAN_POINT('Origin',(-0.233966934007412,0.0158592789729621,
3.09238363249698E-10));
#26093=CARTESIAN_POINT('Ctrl Pts',(-0.227150244243996,0.0165409512347104,
-9.63953309535137E-15));
#26094=CARTESIAN_POINT('Ctrl Pts',(-0.237845216608682,0.0163742849350107,
-4.07145020822619E-16));
#26095=CARTESIAN_POINT('Ctrl Pts',(-0.227150244243996,0.01654095123471,
-0.000381994959333103));
#26096=CARTESIAN_POINT('Ctrl Pts',(-0.237845216608682,0.0163742849350106,
-0.000371791760088174));
#26097=CARTESIAN_POINT('Ctrl Pts',(-0.227150244243997,0.0165287121322335,
-0.00114598487798004));
#26098=CARTESIAN_POINT('Ctrl Pts',(-0.237845216608682,0.0163722325524407,
-0.00111537528026388));
#26099=CARTESIAN_POINT('Ctrl Pts',(-0.227150244243996,0.0164948323843552,
-0.00192393728847136));
#26100=CARTESIAN_POINT('Ctrl Pts',(-0.237845216608682,0.0163665512368254,
-0.00188927901278524));
#26101=CARTESIAN_POINT('Ctrl Pts',(-0.227150244243996,0.0164156764744566,
-0.00344935006783133));
#26102=CARTESIAN_POINT('Ctrl Pts',(-0.237845216608682,0.0163532775339462,
-0.0034371522067016));
#26103=CARTESIAN_POINT('Ctrl Pts',(-0.227150244243997,0.0158708078188047,
-0.00568348814190198));
#26104=CARTESIAN_POINT('Ctrl Pts',(-0.237845216608683,0.0158878089324482,
-0.00572426400319885));
#26105=CARTESIAN_POINT('Ctrl Pts',(-0.227150244243996,0.0138592003117079,
-0.00851222286772063));
#26106=CARTESIAN_POINT('Ctrl Pts',(-0.237845216608682,0.0139254525795067,
-0.00865325189315152));
#26107=CARTESIAN_POINT('Ctrl Pts',(-0.227150244243997,0.0109293641084061,
-0.0103996324725637));
#26108=CARTESIAN_POINT('Ctrl Pts',(-0.237845216608683,0.0109812780384655,
-0.0106210180177305));
#26109=CARTESIAN_POINT('Ctrl Pts',(-0.227150244243996,0.0074999999998714,
-0.0110623240930123));
#26110=CARTESIAN_POINT('Ctrl Pts',(-0.237845216608682,0.00749999999987136,
-0.01131420416039));
#26111=CARTESIAN_POINT('Ctrl Pts',(-0.227150244243997,0.00407063589135525,
-0.0103996324724683));
#26112=CARTESIAN_POINT('Ctrl Pts',(-0.237845216608683,0.00401872196129691,
-0.0106210180176321));
#26113=CARTESIAN_POINT('Ctrl Pts',(-0.227150244243996,0.00114079968810594,
-0.00851222286754358));
#26114=CARTESIAN_POINT('Ctrl Pts',(-0.237845216608682,0.00107454742031117,
-0.00865325189296982));
#26115=CARTESIAN_POINT('Ctrl Pts',(-0.227150244243997,-0.000870807818911773,
-0.00568348814166902));
#26116=CARTESIAN_POINT('Ctrl Pts',(-0.237845216608682,-0.00088780893254747,
-0.00572426400296157));
#26117=CARTESIAN_POINT('Ctrl Pts',(-0.227150244243996,-0.00141567647450146,
-0.00344935006758328));
#26118=CARTESIAN_POINT('Ctrl Pts',(-0.237845216608682,-0.00135327753398082,
-0.00343715220645101));
#26119=CARTESIAN_POINT('Ctrl Pts',(-0.227150244243996,-0.00149483238436559,
-0.00192393728824214));
#26120=CARTESIAN_POINT('Ctrl Pts',(-0.237845216608682,-0.00136655123682709,
-0.00188927901255543));
#26121=CARTESIAN_POINT('Ctrl Pts',(-0.227150244243996,-0.0015287121322383,
-0.00114598487779204));
#26122=CARTESIAN_POINT('Ctrl Pts',(-0.237845216608682,-0.00137223255244152,
-0.0011153752800763));
#26123=CARTESIAN_POINT('Ctrl Pts',(-0.227150244243997,-0.00154707078594764,
1.16062262795529E-13));
#26124=CARTESIAN_POINT('Ctrl Pts',(-0.237845216608682,-0.00137531112629545,
1.24505090562086E-13));
#26125=CARTESIAN_POINT('Ctrl Pts',(-0.227150244243996,-0.00152871213223388,
0.00114598487802365));
#26126=CARTESIAN_POINT('Ctrl Pts',(-0.237845216608682,-0.00137223255244077,
0.00111537528032471));
#26127=CARTESIAN_POINT('Ctrl Pts',(-0.227150244243996,-0.0014948323843583,
0.00192393728847254));
#26128=CARTESIAN_POINT('Ctrl Pts',(-0.237845216608682,-0.00136655123682587,
0.00188927901280252));
#26129=CARTESIAN_POINT('Ctrl Pts',(-0.227150244243996,-0.00141567647446389,
0.00344935006836688));
#26130=CARTESIAN_POINT('Ctrl Pts',(-0.237845216608682,-0.00135327753394768,
0.00343715220737864));
#26131=CARTESIAN_POINT('Ctrl Pts',(-0.227150244243997,-0.000870821762961343,
0.00568349039573915));
#26132=CARTESIAN_POINT('Ctrl Pts',(-0.237845216608682,-0.000887826039510656,
0.00572426676828764));
#26133=CARTESIAN_POINT('Ctrl Pts',(-0.227150244243997,0.00114085439618864,
0.00851222287679413));
#26134=CARTESIAN_POINT('Ctrl Pts',(-0.237845216608682,0.0010746145376654,
0.00865325190429854));
#26135=CARTESIAN_POINT('Ctrl Pts',(-0.227150244243996,0.00407062011024736,
0.0103996408584618));
#26136=CARTESIAN_POINT('Ctrl Pts',(-0.237845216608682,0.00401870260056976,
0.0106210283057897));
#26137=CARTESIAN_POINT('Ctrl Pts',(-0.227150244243997,0.00750000000000013,
0.0110623211795783));
#26138=CARTESIAN_POINT('Ctrl Pts',(-0.237845216608683,0.00749999999999948,
0.0113142005861093));
#26139=CARTESIAN_POINT('Ctrl Pts',(-0.227150244243996,0.0109293798897529,
0.0103996408584618));
#26140=CARTESIAN_POINT('Ctrl Pts',(-0.237845216608681,0.0109812973994292,
0.0106210283057901));
#26141=CARTESIAN_POINT('Ctrl Pts',(-0.227150244243997,0.0138591456038116,
0.00851222287679417));
#26142=CARTESIAN_POINT('Ctrl Pts',(-0.237845216608683,0.0139253854623337,
0.00865325190429944));
#26143=CARTESIAN_POINT('Ctrl Pts',(-0.227150244243997,0.0158708217629616,
0.00568349039573924));
#26144=CARTESIAN_POINT('Ctrl Pts',(-0.237845216608682,0.0158878260395101,
0.00572426676828895));
#26145=CARTESIAN_POINT('Ctrl Pts',(-0.227150244243996,0.0164156764744642,
0.00344935006836702));
#26146=CARTESIAN_POINT('Ctrl Pts',(-0.237845216608682,0.0163532775339475,
0.00343715220738017));
#26147=CARTESIAN_POINT('Ctrl Pts',(-0.227150244243996,0.0164740029315869,
0.00232534147293065));
#26148=CARTESIAN_POINT('Ctrl Pts',(-0.237845216608682,0.0163630583331681,
0.0022965935348158));
#26149=CARTESIAN_POINT('Ctrl Pts',(-0.227150244243996,0.0164948323843597,
0.00192393728845175));
#26150=CARTESIAN_POINT('Ctrl Pts',(-0.237845216608682,0.0163665512368261,
0.0018892790127829));
#26151=CARTESIAN_POINT('Ctrl Pts',(-0.227150244243996,0.0165287121322363,
0.00114598487796074));
#26152=CARTESIAN_POINT('Ctrl Pts',(-0.237845216608682,0.0163722325524412,
0.00111537528026272));
#26153=CARTESIAN_POINT('Ctrl Pts',(-0.227150244243996,0.0165409512347109,
0.000381994959313824));
#26154=CARTESIAN_POINT('Ctrl Pts',(-0.237845216608682,0.0163742849350108,
0.00037179176008736));
#26155=CARTESIAN_POINT('Ctrl Pts',(-0.227150244243996,0.0165409512347104,
-9.63953309535137E-15));
#26156=CARTESIAN_POINT('Ctrl Pts',(-0.237845216608682,0.0163742849350107,
-4.07145020822619E-16));
#26157=CARTESIAN_POINT('',(-0.230613689225592,0.0164370167296803,0.00231666183293797));
#26158=CARTESIAN_POINT('',(-0.228219847986792,0.016461711610013,0.00232234304728458));
#26159=CARTESIAN_POINT('Ctrl Pts',(-0.230613698506742,0.0164380746908005,
0.00231603175567153));
#26160=CARTESIAN_POINT('Ctrl Pts',(-0.228219860721099,0.0164629072347989,
0.00232246635860196));
#26161=CARTESIAN_POINT('',(-0.230845404656383,0.01641869106371,0.00262492038517608));
#26162=CARTESIAN_POINT('Ctrl Pts',(-0.230845397055334,0.0164178730318222,
0.0026248611718336));
#26163=CARTESIAN_POINT('Ctrl Pts',(-0.230763233312891,0.0164246613929725,
0.00252596184206025));
#26164=CARTESIAN_POINT('Ctrl Pts',(-0.230685933491642,0.0164310479032495,
0.0024230472437672));
#26165=CARTESIAN_POINT('Ctrl Pts',(-0.230613689225592,0.0164370167296803,
0.00231666183293795));
#26166=CARTESIAN_POINT('',(-0.230845404654042,-0.00141869264250409,0.0026249204784827));
#26167=CARTESIAN_POINT('Ctrl Pts',(-0.230845406155635,0.0164188524145726,
0.00262493206457884));
#26168=CARTESIAN_POINT('Ctrl Pts',(-0.231100300338632,0.016394135408487,
0.00293573688999021));
#26169=CARTESIAN_POINT('Ctrl Pts',(-0.231330253084667,0.0163562988156621,
0.00321637191052311));
#26170=CARTESIAN_POINT('Ctrl Pts',(-0.231531680676482,0.016314511634419,
0.00346194554495639));
#26171=CARTESIAN_POINT('Ctrl Pts',(-0.231632395191451,0.0162936178946247,
0.0035847332388272));
#26172=CARTESIAN_POINT('Ctrl Pts',(-0.231725978785969,0.0162717928171178,
0.00369876105724253));
#26173=CARTESIAN_POINT('Ctrl Pts',(-0.231816013844249,0.0162489000359078,
0.00380848773826119));
#26174=CARTESIAN_POINT('Ctrl Pts',(-0.231861031373389,0.0162374536453028,
0.00386335107877052));
#26175=CARTESIAN_POINT('Ctrl Pts',(-0.231905161506138,0.016225692875953,
0.00391713038034571));
#26176=CARTESIAN_POINT('Ctrl Pts',(-0.231943478722522,0.0162151366678332,
0.00396380508855938));
#26177=CARTESIAN_POINT('Ctrl Pts',(-0.231981795938907,0.0162045804597134,
0.00401047979677305));
#26178=CARTESIAN_POINT('Ctrl Pts',(-0.232014300953749,0.0161953870895132,
0.00405008402747138));
#26179=CARTESIAN_POINT('Ctrl Pts',(-0.232061142463723,0.0161815297542121,
0.00410721922519355));
#26180=CARTESIAN_POINT('Ctrl Pts',(-0.232107983973697,0.0161676724189111,
0.00416435442291572));
#26181=CARTESIAN_POINT('Ctrl Pts',(-0.232169160847613,0.0161488560231783,
0.00423895076719931));
#26182=CARTESIAN_POINT('Ctrl Pts',(-0.232225616581178,0.0161305642422028,
0.00430777306797529));
#26183=CARTESIAN_POINT('Ctrl Pts',(-0.232282072314744,0.0161122724612272,
0.00437659536875126));
#26184=CARTESIAN_POINT('Ctrl Pts',(-0.232333807470107,0.0160947133906112,
0.00443970018976271));
#26185=CARTESIAN_POINT('Ctrl Pts',(-0.232385377331384,0.0160765467528926,
0.00450260334417301));
#26186=CARTESIAN_POINT('Ctrl Pts',(-0.232488517053936,0.0160402134774552,
0.00462840965299361));
#26187=CARTESIAN_POINT('Ctrl Pts',(-0.232590995510011,0.0160012622260062,
0.00475334511963562));
#26188=CARTESIAN_POINT('Ctrl Pts',(-0.232690758730041,0.0159606000393275,
0.00487499945630557));
#26189=CARTESIAN_POINT('Ctrl Pts',(-0.232790521950071,0.0159199378526488,
0.00499665379297553));
#26190=CARTESIAN_POINT('Ctrl Pts',(-0.232887569522866,0.0158775169648435,
0.00511502319888208));
#26191=CARTESIAN_POINT('Ctrl Pts',(-0.232977286659695,0.0158360935819725,
0.0052243323902255));
#26192=CARTESIAN_POINT('Ctrl Pts',(-0.233067003796523,0.0157946701991014,
0.00533364158156891));
#26193=CARTESIAN_POINT('Ctrl Pts',(-0.23314939055768,0.0157546441706645,
0.00543403165986536));
#26194=CARTESIAN_POINT('Ctrl Pts',(-0.233244961120346,0.0157052982799395,
0.00555069044803048));
#26195=CARTESIAN_POINT('Ctrl Pts',(-0.233263930412106,0.0156955038770163,
0.00557384542930724));
#26196=CARTESIAN_POINT('Ctrl Pts',(-0.233283419144619,0.0156853288434712,
0.00559763514898268));
#26197=CARTESIAN_POINT('Ctrl Pts',(-0.233303270872681,0.0156748394500476,
0.00562186377880468));
#26198=CARTESIAN_POINT('Ctrl Pts',(-0.233383435573525,0.0156324814707721,
0.0057197031636423));
#26199=CARTESIAN_POINT('Ctrl Pts',(-0.23346951958345,0.0155848560910614,
0.00582464387515683));
#26200=CARTESIAN_POINT('Ctrl Pts',(-0.233551221014356,0.0155374303604521,
0.00592420294833371));
#26201=CARTESIAN_POINT('Ctrl Pts',(-0.233653154724202,0.0154782602748176,
0.00604841650940856));
#26202=CARTESIAN_POINT('Ctrl Pts',(-0.233748264657028,0.0154197330280522,
0.006164431229071));
#26203=CARTESIAN_POINT('Ctrl Pts',(-0.233842820452025,0.0153585628948797,
0.00627980759476657));
#26204=CARTESIAN_POINT('Ctrl Pts',(-0.233937376247022,0.0152973927617072,
0.00639518396046214));
#26205=CARTESIAN_POINT('Ctrl Pts',(-0.234031378989655,0.0152333870670153,
0.00650981630376789));
#26206=CARTESIAN_POINT('Ctrl Pts',(-0.234119759433353,0.0151704480417673,
0.0066174646559021));
#26207=CARTESIAN_POINT('Ctrl Pts',(-0.23420813987705,0.0151075090165192,
0.00672511300803631));
#26208=CARTESIAN_POINT('Ctrl Pts',(-0.234290895921197,0.0150459592772678,
0.00682596426023255));
#26209=CARTESIAN_POINT('Ctrl Pts',(-0.23438203795834,0.0149747376617064,
0.00693722683716703));
#26210=CARTESIAN_POINT('Ctrl Pts',(-0.234473179995482,0.014903516046145,
0.00704848941410152));
#26211=CARTESIAN_POINT('Ctrl Pts',(-0.234572712055863,0.0148221387927767,
0.0071698520102151));
#26212=CARTESIAN_POINT('Ctrl Pts',(-0.234666614521964,0.0147414320966982,
0.00728423838151296));
#26213=CARTESIAN_POINT('Ctrl Pts',(-0.234760516988065,0.0146607254006198,
0.00739862475281083));
#26214=CARTESIAN_POINT('Ctrl Pts',(-0.234848786350016,0.0145810186683803,
0.00750627424136947));
#26215=CARTESIAN_POINT('Ctrl Pts',(-0.234936248176809,0.0144983824900823,
0.00761302947121143));
#26216=CARTESIAN_POINT('Ctrl Pts',(-0.235023710003601,0.0144157463117844,
0.00771978470105339));
#26217=CARTESIAN_POINT('Ctrl Pts',(-0.23511036646589,0.0143299974330337,
0.00782550470042646));
#26218=CARTESIAN_POINT('Ctrl Pts',(-0.235190938922874,0.014247020334218,
0.00792356544252254));
#26219=CARTESIAN_POINT('Ctrl Pts',(-0.235271511379857,0.0141640432354024,
0.00802162618461862));
#26220=CARTESIAN_POINT('Ctrl Pts',(-0.235345994424314,0.0140842359024048,
0.00811235964384396));
#26221=CARTESIAN_POINT('Ctrl Pts',(-0.235430686760159,0.0139887033941303,
0.00821589281443685));
#26222=CARTESIAN_POINT('Ctrl Pts',(-0.235495095996826,0.0139160501147822,
0.00829463066504644));
#26223=CARTESIAN_POINT('Ctrl Pts',(-0.235565415763708,0.0138340266016512,
0.00838051344444797));
#26224=CARTESIAN_POINT('Ctrl Pts',(-0.235634425112979,0.0137502746078903,
0.00846458329314199));
#26225=CARTESIAN_POINT('Ctrl Pts',(-0.235656156832651,0.0137239002851413,
0.00849105771152119));
#26226=CARTESIAN_POINT('Ctrl Pts',(-0.235677758600599,0.0136973642359917,
0.00851736083439707));
#26227=CARTESIAN_POINT('Ctrl Pts',(-0.235699004913631,0.0136709329854625,
0.00854323862301745));
#26228=CARTESIAN_POINT('Ctrl Pts',(-0.235787719161043,0.0135605689662904,
0.00865129165502526));
#26229=CARTESIAN_POINT('Ctrl Pts',(-0.235870228407553,0.0134521030844415,
0.00875205385374006));
#26230=CARTESIAN_POINT('Ctrl Pts',(-0.235950605571676,0.0133411714387136,
0.00885026140620821));
#26231=CARTESIAN_POINT('Ctrl Pts',(-0.236111359899922,0.0131193081472577,
0.0090466765111445));
#26232=CARTESIAN_POINT('Ctrl Pts',(-0.236263595884827,0.0128871731417065,
0.0092323612018346));
#26233=CARTESIAN_POINT('Ctrl Pts',(-0.236403654401485,0.0126515670091865,
0.0094029129604812));
#26234=CARTESIAN_POINT('Ctrl Pts',(-0.236543712918143,0.0124159608766665,
0.0095734647191278));
#26235=CARTESIAN_POINT('Ctrl Pts',(-0.236671587059248,0.0121771237877737,
0.00972922544746999));
#26236=CARTESIAN_POINT('Ctrl Pts',(-0.236789833249587,0.0119311450822871,
0.00987356375454342));
#26237=CARTESIAN_POINT('Ctrl Pts',(-0.236848956344757,0.0118081557295438,
0.00994573290808013));
#26238=CARTESIAN_POINT('Ctrl Pts',(-0.23690567511583,0.0116833001634472,
0.0100149174696784));
#26239=CARTESIAN_POINT('Ctrl Pts',(-0.236957846430498,0.0115626181380559,
0.0100782504702421));
#26240=CARTESIAN_POINT('Ctrl Pts',(-0.237010017745166,0.0114419361126645,
0.0101415834708057));
#26241=CARTESIAN_POINT('Ctrl Pts',(-0.237057632216303,0.011325666949853,
0.0101995095969159));
#26242=CARTESIAN_POINT('Ctrl Pts',(-0.237109142115983,0.0111901477257744,
0.0102626567192974));
#26243=CARTESIAN_POINT('Ctrl Pts',(-0.237144692626639,0.0110966166249623,
0.0103062388745939));
#26244=CARTESIAN_POINT('Ctrl Pts',(-0.237182106718332,0.0109937916041834,
0.0103520374018463));
#26245=CARTESIAN_POINT('Ctrl Pts',(-0.237218322025799,0.0108890866011028,
0.0103961046392556));
#26246=CARTESIAN_POINT('Ctrl Pts',(-0.237234579856412,0.0108420822727267,
0.0104158873701364));
#26247=CARTESIAN_POINT('Ctrl Pts',(-0.23725059609541,0.010794706184345,
0.0104353353011454));
#26248=CARTESIAN_POINT('Ctrl Pts',(-0.237266093686358,0.0107476642246503,
0.010454168061085));
#26249=CARTESIAN_POINT('Ctrl Pts',(-0.237316113104637,0.0105958334358221,
0.0105149519403283));
#26250=CARTESIAN_POINT('Ctrl Pts',(-0.237360717689318,0.0104475103219917,
0.0105694881860006));
#26251=CARTESIAN_POINT('Ctrl Pts',(-0.237402188197519,0.0102972373788654,
0.010620255747033));
#26252=CARTESIAN_POINT('Ctrl Pts',(-0.237485129213922,0.0099966914926128,
0.0107217908690978));
#26253=CARTESIAN_POINT('Ctrl Pts',(-0.237555547649754,0.00968817545869758,
0.0108076341360598));
#26254=CARTESIAN_POINT('Ctrl Pts',(-0.237611806042195,0.00937864054540575,
0.0108759601364871));
#26255=CARTESIAN_POINT('Ctrl Pts',(-0.237724322827076,0.00875957071882208,
0.0110126121373416));
#26256=CARTESIAN_POINT('Ctrl Pts',(-0.237780162569082,0.00813666054908404,
0.0110808280399472));
#26257=CARTESIAN_POINT('Ctrl Pts',(-0.237780757020967,0.00751171081608989,
0.0110816784755926));
#26258=CARTESIAN_POINT('Ctrl Pts',(-0.237780760734013,0.00750780727624916,
0.011081683787555));
#26259=CARTESIAN_POINT('Ctrl Pts',(-0.237780762292029,0.00750390367038639,
0.0110816864372711));
#26260=CARTESIAN_POINT('Ctrl Pts',(-0.237780761694531,0.00749999999999945,
0.0110816864237671));
#26261=CARTESIAN_POINT('Ctrl Pts',(-0.23778066663381,0.00687893303717793,
0.0110816842753144));
#26262=CARTESIAN_POINT('Ctrl Pts',(-0.237726010708986,0.00625608202678869,
0.0110147767774946));
#26263=CARTESIAN_POINT('Ctrl Pts',(-0.237614845441578,0.00563821530166374,
0.0108796632942073));
#26264=CARTESIAN_POINT('Ctrl Pts',(-0.237558913447348,0.00532734016133628,
0.0108116819296686));
#26265=CARTESIAN_POINT('Ctrl Pts',(-0.237488683165496,0.00501775189075729,
0.0107261184353061));
#26266=CARTESIAN_POINT('Ctrl Pts',(-0.237405879976365,0.00471612119147505,
0.0106247571095187));
#26267=CARTESIAN_POINT('Ctrl Pts',(-0.2373644783818,0.00456530584183393,
0.0105740764466251));
#26268=CARTESIAN_POINT('Ctrl Pts',(-0.237319930103575,0.00441643903893137,
0.0105196014633509));
#26269=CARTESIAN_POINT('Ctrl Pts',(-0.237269894824879,0.00426394159912891,
0.0104588043597344));
#26270=CARTESIAN_POINT('Ctrl Pts',(-0.237253190953929,0.00421303156882405,
0.0104385077410399));
#26271=CARTESIAN_POINT('Ctrl Pts',(-0.237235876931987,0.00416172022874334,
0.0104174873363778));
#26272=CARTESIAN_POINT('Ctrl Pts',(-0.237218307823531,0.00411091345951884,
0.0103961043563028));
#26273=CARTESIAN_POINT('Ctrl Pts',(-0.237183249894779,0.00400953210029451,
0.0103534361131266));
#26274=CARTESIAN_POINT('Ctrl Pts',(-0.237147176277473,0.00391018939539668,
0.0103092664206609));
#26275=CARTESIAN_POINT('Ctrl Pts',(-0.237112908060806,0.00381972380657039,
0.0102672494712808));
#26276=CARTESIAN_POINT('Ctrl Pts',(-0.237061466496008,0.00368392183313235,
0.0102041759345063));
#26277=CARTESIAN_POINT('Ctrl Pts',(-0.237014075859274,0.00356786256094538,
0.0101465240645061));
#26278=CARTESIAN_POINT('Ctrl Pts',(-0.236962091075866,0.00344725418310079,
0.0100834231132401));
#26279=CARTESIAN_POINT('Ctrl Pts',(-0.236910106292458,0.00332664580525621,
0.0100203221619742));
#26280=CARTESIAN_POINT('Ctrl Pts',(-0.236853536995318,0.003201733163161,
0.00995131596519577));
#26281=CARTESIAN_POINT('Ctrl Pts',(-0.236794570856648,0.0030787040364747,
0.00987933488154406));
#26282=CARTESIAN_POINT('Ctrl Pts',(-0.236676638579308,0.00283264578310208,
0.00973537271424062));
#26283=CARTESIAN_POINT('Ctrl Pts',(-0.236549108070154,0.00259379182280089,
0.0095800372046828));
#26284=CARTESIAN_POINT('Ctrl Pts',(-0.23640942071538,0.00235815034729726,
0.00940993731667735));
#26285=CARTESIAN_POINT('Ctrl Pts',(-0.236269733360606,0.00212250887179363,
0.0092398374286719));
#26286=CARTESIAN_POINT('Ctrl Pts',(-0.236117896002483,0.00189031920890611,
0.00905463410525447));
#26287=CARTESIAN_POINT('Ctrl Pts',(-0.235957457637001,0.00166827584739166,
0.00885861358605071));
#26288=CARTESIAN_POINT('Ctrl Pts',(-0.23587723845426,0.00155725416663443,
0.00876060332644883));
#26289=CARTESIAN_POINT('Ctrl Pts',(-0.235794866603536,0.00144867026152674,
0.00866001258255653));
#26290=CARTESIAN_POINT('Ctrl Pts',(-0.235706421246396,0.00133831736827609,
0.00855228205242222));
#26291=CARTESIAN_POINT('Ctrl Pts',(-0.235682754877842,0.00130878894160599,
0.00852345532241545));
#26292=CARTESIAN_POINT('Ctrl Pts',(-0.235658654177629,0.00127913904841267,
0.0084941084536834));
#26293=CARTESIAN_POINT('Ctrl Pts',(-0.235634421754154,0.00124972540958528,
0.00846458324989155));
#26294=CARTESIAN_POINT('Ctrl Pts',(-0.235568093374281,0.00116921513739988,
0.00838376760489224));
#26295=CARTESIAN_POINT('Ctrl Pts',(-0.235500778107123,0.00109055246370788,
0.00830154828174661));
#26296=CARTESIAN_POINT('Ctrl Pts',(-0.235438681621512,0.00102030581655116,
0.00822564249980966));
#26297=CARTESIAN_POINT('Ctrl Pts',(-0.235353898793518,0.000924395245373119,
0.00812200528442701));
#26298=CARTESIAN_POINT('Ctrl Pts',(-0.235278834910607,0.000843726368531342,
0.00803055897729168));
#26299=CARTESIAN_POINT('Ctrl Pts',(-0.235197751777394,0.000760017919507905,
0.00793187284909972));
#26300=CARTESIAN_POINT('Ctrl Pts',(-0.235116668644181,0.000676309470484467,
0.00783318672090776));
#26301=CARTESIAN_POINT('Ctrl Pts',(-0.235029571572779,0.000589949806240253,
0.00772693550362108));
#26302=CARTESIAN_POINT('Ctrl Pts',(-0.234941674231112,0.000506744595351982,
0.00761964685648566));
#26303=CARTESIAN_POINT('Ctrl Pts',(-0.234853776889444,0.000423539384463711,
0.00751235820935023));
#26304=CARTESIAN_POINT('Ctrl Pts',(-0.234765077020754,0.000343301382149936,
0.00740417759734143));
#26305=CARTESIAN_POINT('Ctrl Pts',(-0.234670448982667,0.000261869893349022,
0.00728891518395673));
#26306=CARTESIAN_POINT('Ctrl Pts',(-0.234575820944579,0.000180438404548108,
0.00717365277057203));
#26307=CARTESIAN_POINT('Ctrl Pts',(-0.23447526857943,9.81717754813013E-5,
0.00705104731107811));
#26308=CARTESIAN_POINT('Ctrl Pts',(-0.234384076032058,2.68535732625788E-5,
0.00693971183174857));
#26309=CARTESIAN_POINT('Ctrl Pts',(-0.234292883484686,-4.44646289561437E-5,
0.00682837635241903));
#26310=CARTESIAN_POINT('Ctrl Pts',(-0.234211046367837,-0.000105360993591713,
0.00672864972887943));
#26311=CARTESIAN_POINT('Ctrl Pts',(-0.23412337118657,-0.00016787228663261,
0.00662186731835593));
#26312=CARTESIAN_POINT('Ctrl Pts',(-0.234035696005303,-0.000230383579673508,
0.00651508490783243));
#26313=CARTESIAN_POINT('Ctrl Pts',(-0.233942184999647,-0.000294164288529817,
0.00640104689092552));
#26314=CARTESIAN_POINT('Ctrl Pts',(-0.233848164561004,-0.000355105177677982,
0.00628632317533926));
#26315=CARTESIAN_POINT('Ctrl Pts',(-0.233754144122361,-0.000416046066826147,
0.00617159945975299));
#26316=CARTESIAN_POINT('Ctrl Pts',(-0.233659613180542,-0.000474341316365998,
0.00605629571904232));
#26317=CARTESIAN_POINT('Ctrl Pts',(-0.233558456155359,-0.000533221594720501,
0.00593302620228869));
#26318=CARTESIAN_POINT('Ctrl Pts',(-0.233474310049849,-0.000582200359229365,
0.00583048611924345));
#26319=CARTESIAN_POINT('Ctrl Pts',(-0.233385580249099,-0.000631352225649045,
0.00572231156613564));
#26320=CARTESIAN_POINT('Ctrl Pts',(-0.233303279983003,-0.000674839454613146,
0.00562186381649031));
#26321=CARTESIAN_POINT('Ctrl Pts',(-0.233286642216975,-0.00068363080335406,
0.0056015573674843));
#26322=CARTESIAN_POINT('Ctrl Pts',(-0.233270267215688,-0.000692197111540543,
0.00558156925020403));
#26323=CARTESIAN_POINT('Ctrl Pts',(-0.233254245969635,-0.000700499830582056,
0.00556201347580956));
#26324=CARTESIAN_POINT('Ctrl Pts',(-0.233158974131218,-0.000749872726069023,
0.00544572323396024));
#26325=CARTESIAN_POINT('Ctrl Pts',(-0.233076210545331,-0.000790248603855624,
0.0053448711035504));
#26326=CARTESIAN_POINT('Ctrl Pts',(-0.232986293433231,-0.00083192370727539,
0.00523531504586229));
#26327=CARTESIAN_POINT('Ctrl Pts',(-0.232896376321131,-0.000873598810695155,
0.00512575898817417));
#26328=CARTESIAN_POINT('Ctrl Pts',(-0.232799305640179,-0.000916189568014474,
0.00500736315149536));
#26329=CARTESIAN_POINT('Ctrl Pts',(-0.232699475480134,-0.000957040429939678,
0.00488562808656381));
#26330=CARTESIAN_POINT('Ctrl Pts',(-0.23259964532009,-0.000997891291864883,
0.00476389302163227));
#26331=CARTESIAN_POINT('Ctrl Pts',(-0.232497056076894,-0.0010370458356378,
0.00463882151690649));
#26332=CARTESIAN_POINT('Ctrl Pts',(-0.232393792110345,-0.00107357729545367,
0.00451286349182803));
#26333=CARTESIAN_POINT('Ctrl Pts',(-0.232342160127071,-0.0010918430253616,
0.0044498844792888));
#26334=CARTESIAN_POINT('Ctrl Pts',(-0.232290359484728,-0.00110949976706081,
0.00438669985428264));
#26335=CARTESIAN_POINT('Ctrl Pts',(-0.23223387589419,-0.00112788179208304,
0.00431784339824848));
#26336=CARTESIAN_POINT('Ctrl Pts',(-0.232177392303652,-0.00114626381710528,
0.00424898694221432));
#26337=CARTESIAN_POINT('Ctrl Pts',(-0.232116225215548,-0.00116516478536523,
0.00417440231650458));
#26338=CARTESIAN_POINT('Ctrl Pts',(-0.232069243323862,-0.00117912866891544,
0.00411709598246582));
#26339=CARTESIAN_POINT('Ctrl Pts',(-0.232022261432176,-0.00119309255246565,
0.00405978964842705));
#26340=CARTESIAN_POINT('Ctrl Pts',(-0.231989465850055,-0.00120241270487414,
0.00401983136596938));
#26341=CARTESIAN_POINT('Ctrl Pts',(-0.231950878638839,-0.00121309140983481,
0.00397282798321303));
#26342=CARTESIAN_POINT('Ctrl Pts',(-0.231912291427624,-0.00122377011479549,
0.00392582460045668));
#26343=CARTESIAN_POINT('Ctrl Pts',(-0.231867911879468,-0.00123564945038949,
0.00387174191318196));
#26344=CARTESIAN_POINT('Ctrl Pts',(-0.231822623769973,-0.00124721447752194,
0.00381654936798492));
#26345=CARTESIAN_POINT('Ctrl Pts',(-0.231732047550984,-0.00127034453178683,
0.00370616427759082));
#26346=CARTESIAN_POINT('Ctrl Pts',(-0.231637838129472,-0.00129240691549724,
0.00359137488292652));
#26347=CARTESIAN_POINT('Ctrl Pts',(-0.231536443480711,-0.00131352075345898,
0.00346775798194196));
#26348=CARTESIAN_POINT('Ctrl Pts',(-0.231333655616239,-0.00135574813097255,
0.00322052592709761));
#26349=CARTESIAN_POINT('Ctrl Pts',(-0.231102125386862,-0.00139395843488747,
0.00293796225972129));
#26350=CARTESIAN_POINT('Ctrl Pts',(-0.23084540613858,-0.0014188524162263,
0.00262493204378136));
#26351=CARTESIAN_POINT('',(-0.230845404651119,-0.00141869028668481,-0.00262492044785718));
#26352=CARTESIAN_POINT('Ctrl Pts',(-0.23084539705679,-0.00141787297644972,
-0.00262486128582299));
#26353=CARTESIAN_POINT('Ctrl Pts',(-0.230239453773023,-0.00146793597280632,
-0.00189549595714672));
#26354=CARTESIAN_POINT('Ctrl Pts',(-0.229556645639841,-0.00152435019813871,
-2.99121385213125E-11));
#26355=CARTESIAN_POINT('Ctrl Pts',(-0.230239453775278,-0.00146793830190954,
0.00189549598038732));
#26356=CARTESIAN_POINT('Ctrl Pts',(-0.230845397068071,-0.00141787620064688,
0.00262486137994144));
#26357=CARTESIAN_POINT('',(-0.230845404648896,0.0164186918782877,-0.00262492054209142));
#26358=CARTESIAN_POINT('Ctrl Pts',(-0.230845406155915,-0.0014188522345682,
-0.00262493217065937));
#26359=CARTESIAN_POINT('Ctrl Pts',(-0.231100299441669,-0.00139413497480491,
-0.00293573599126679));
#26360=CARTESIAN_POINT('Ctrl Pts',(-0.231330251778893,-0.00135629782996439,
-0.00321637052807434));
#26361=CARTESIAN_POINT('Ctrl Pts',(-0.231531679491658,-0.0013145100902101,
-0.0034619443061207));
#26362=CARTESIAN_POINT('Ctrl Pts',(-0.231632394067082,-0.00129361607116236,
-0.00358473207177392));
#26363=CARTESIAN_POINT('Ctrl Pts',(-0.231725977854448,-0.00127179070475759,
-0.00369876011773195));
#26364=CARTESIAN_POINT('Ctrl Pts',(-0.231816013196795,-0.00124889763374325,
-0.00380848713108777));
#26365=CARTESIAN_POINT('Ctrl Pts',(-0.231861030867968,-0.00123745109823607,
-0.00386335063776568));
#26366=CARTESIAN_POINT('Ctrl Pts',(-0.231905161165557,-0.00122569018461765,
-0.00391713013177141));
#26367=CARTESIAN_POINT('Ctrl Pts',(-0.231943478626256,-0.00121513382583439,
-0.00396380513001859));
#26368=CARTESIAN_POINT('Ctrl Pts',(-0.231981796086954,-0.00120457746705113,
-0.00401048012826578));
#26369=CARTESIAN_POINT('Ctrl Pts',(-0.232014301425573,-0.00119538393551268,
-0.00405008474598364));
#26370=CARTESIAN_POINT('Ctrl Pts',(-0.232061143106978,-0.00118152646221356,
-0.00410722013721966));
#26371=CARTESIAN_POINT('Ctrl Pts',(-0.232107984788383,-0.00116766898891443,
-0.00416435552845569));
#26372=CARTESIAN_POINT('Ctrl Pts',(-0.232169161681404,-0.0011488524875137,
-0.00423895187437171));
#26373=CARTESIAN_POINT('Ctrl Pts',(-0.232225617477761,-0.00113056062213835,
-0.00430777422986251));
#26374=CARTESIAN_POINT('Ctrl Pts',(-0.232282073274118,-0.00111226875676299,
-0.00437659658535332));
#26375=CARTESIAN_POINT('Ctrl Pts',(-0.232333808535951,-0.00109470961568399,
-0.00443970151234894));
#26376=CARTESIAN_POINT('Ctrl Pts',(-0.232385378497271,-0.00107654293258796,
-0.00450260476284944));
#26377=CARTESIAN_POINT('Ctrl Pts',(-0.232488518419909,-0.0010402095663959,
-0.00462841126385043));
#26378=CARTESIAN_POINT('Ctrl Pts',(-0.232590997050356,-0.00100125833324369,
-0.00475334688627594));
#26379=CARTESIAN_POINT('Ctrl Pts',(-0.232690760482472,-0.000960596280089447,
-0.00487500141782347));
#26380=CARTESIAN_POINT('Ctrl Pts',(-0.232790523914588,-0.000919934226935205,
-0.004996655949371));
#26381=CARTESIAN_POINT('Ctrl Pts',(-0.232887571737198,-0.000877513589272111,
-0.00511502558860545));
#26382=CARTESIAN_POINT('Ctrl Pts',(-0.232977289062584,-0.000836090591733953,
-0.00522433494448881));
#26383=CARTESIAN_POINT('Ctrl Pts',(-0.23306700638797,-0.000794667594195795,
-0.00533364430037216));
#26384=CARTESIAN_POINT('Ctrl Pts',(-0.233149393276443,-0.000754642065908336,
-0.00543403446638583));
#26385=CARTESIAN_POINT('Ctrl Pts',(-0.233244964237605,-0.000705296829430848,
-0.00555069365387462));
#26386=CARTESIAN_POINT('Ctrl Pts',(-0.233263932311264,-0.000695503226134894,
-0.00557384713098106));
#26387=CARTESIAN_POINT('Ctrl Pts',(-0.233283419765313,-0.000685329050860441,
-0.0055976352729477));
#26388=CARTESIAN_POINT('Ctrl Pts',(-0.233303270183162,-0.000674840562095146,
-0.00562186228754064));
#26389=CARTESIAN_POINT('Ctrl Pts',(-0.233383436432652,-0.000632482622148265,
-0.00571970349728819));
#26390=CARTESIAN_POINT('Ctrl Pts',(-0.233469522483554,-0.000584857161359883,
-0.00582464663831474));
#26391=CARTESIAN_POINT('Ctrl Pts',(-0.233551225695154,-0.000537431472865814,
-0.0059242078377752));
#26392=CARTESIAN_POINT('Ctrl Pts',(-0.233653159900472,-0.000478262441763955,
-0.00604842194819661));
#26393=CARTESIAN_POINT('Ctrl Pts',(-0.233748270154742,-0.000419736430952795,
-0.00616443701620916));
#26394=CARTESIAN_POINT('Ctrl Pts',(-0.233842826257912,-0.000358567629232587,
-0.006279813729117));
#26395=CARTESIAN_POINT('Ctrl Pts',(-0.233937382361082,-0.000297398827512379,
-0.00639519044202484));
#26396=CARTESIAN_POINT('Ctrl Pts',(-0.23403138539862,-0.000233394558382435,
-0.00650982313433746));
#26397=CARTESIAN_POINT('Ctrl Pts',(-0.234119765925877,-0.000170457051937254,
-0.00661747158556569));
#26398=CARTESIAN_POINT('Ctrl Pts',(-0.234208146453135,-0.000107519545492074,
-0.00672512003679392));
#26399=CARTESIAN_POINT('Ctrl Pts',(-0.234290902369359,-4.59714339226739E-5,
-0.00682597114194729));
#26400=CARTESIAN_POINT('Ctrl Pts',(-0.234382044699051,2.52487478127625E-5,
-0.0069372341098404));
#26401=CARTESIAN_POINT('Ctrl Pts',(-0.234473187028743,9.64689295481989E-5,
-0.00704849707773351));
#26402=CARTESIAN_POINT('Ctrl Pts',(-0.234572719802503,0.000177844972312555,
-0.0071698605915413));
#26403=CARTESIAN_POINT('Ctrl Pts',(-0.234666622816077,0.00025855057469694,
-0.00728424768332998));
#26404=CARTESIAN_POINT('Ctrl Pts',(-0.234760525829651,0.000339256177081325,
-0.00739863477511866));
#26405=CARTESIAN_POINT('Ctrl Pts',(-0.234848795572813,0.000418961911282749,
-0.00750628479796341));
#26406=CARTESIAN_POINT('Ctrl Pts',(-0.234936257673823,0.000501597197614576,
-0.00761304043838177));
#26407=CARTESIAN_POINT('Ctrl Pts',(-0.235023719774834,0.000584232483946402,
-0.00771979607880013));
#26408=CARTESIAN_POINT('Ctrl Pts',(-0.235110376404512,0.000669980582370447,
-0.00782551636256507));
#26409=CARTESIAN_POINT('Ctrl Pts',(-0.235190949272289,0.000752957489623783,
-0.00792357768997112));
#26410=CARTESIAN_POINT('Ctrl Pts',(-0.235271522140065,0.000835934396877121,
-0.00802163901737717));
#26411=CARTESIAN_POINT('Ctrl Pts',(-0.235346005838469,0.00091574212505546,
-0.00811237336127969));
#26412=CARTESIAN_POINT('Ctrl Pts',(-0.235430697611473,0.00101127399908969,
-0.00821590594222279));
#26413=CARTESIAN_POINT('Ctrl Pts',(-0.235495103302302,0.00108392327923873,
-0.00829463953301149));
#26414=CARTESIAN_POINT('Ctrl Pts',(-0.23556541824769,0.00116594127053609,
-0.00838051651305141));
#26415=CARTESIAN_POINT('Ctrl Pts',(-0.235634423268975,0.00124968821256174,
-0.00846458116969803));
#26416=CARTESIAN_POINT('Ctrl Pts',(-0.2356561580181,0.0012760662752152,
-0.00849105930401949));
#26417=CARTESIAN_POINT('Ctrl Pts',(-0.23567776281192,0.00130260617834922,
-0.00851736613094175));
#26418=CARTESIAN_POINT('Ctrl Pts',(-0.235699012065757,0.00132904129744443,
-0.00854324751893055));
#26419=CARTESIAN_POINT('Ctrl Pts',(-0.235787724956046,0.00143940450539861,
-0.00865129897103351));
#26420=CARTESIAN_POINT('Ctrl Pts',(-0.235870233267096,0.00154787042356857,
-0.00875206008310034));
#26421=CARTESIAN_POINT('Ctrl Pts',(-0.235950609516249,0.00165880240566226,
-0.00885026655961241));
#26422=CARTESIAN_POINT('Ctrl Pts',(-0.236111362014556,0.00188066636984964,
-0.00904667951263656));
#26423=CARTESIAN_POINT('Ctrl Pts',(-0.236263596251478,0.00211280322822169,
-0.00923236210459433));
#26424=CARTESIAN_POINT('Ctrl Pts',(-0.236403653405857,0.00234841200251143,
-0.00940291221444271));
#26425=CARTESIAN_POINT('Ctrl Pts',(-0.236543710560236,0.00258402077680117,
-0.00957346232429108));
#26426=CARTESIAN_POINT('Ctrl Pts',(-0.236671583724811,0.00282286130642932,
-0.00972922184899156));
#26427=CARTESIAN_POINT('Ctrl Pts',(-0.236789829280297,0.00306884369932654,
-0.00987355935155708));
#26428=CARTESIAN_POINT('Ctrl Pts',(-0.236848952058039,0.00319183489577516,
-0.00994572810283985));
#26429=CARTESIAN_POINT('Ctrl Pts',(-0.236905670597119,0.00331669236566743,
-0.0100149123613222));
#26430=CARTESIAN_POINT('Ctrl Pts',(-0.236957841711828,0.00343737605699863,
-0.0100782450944094));
#26431=CARTESIAN_POINT('Ctrl Pts',(-0.237010012826538,0.00355805974832983,
-0.0101415778274966));
#26432=CARTESIAN_POINT('Ctrl Pts',(-0.237057627129816,0.00367433034474948,
-0.0101995037203407));
#26433=CARTESIAN_POINT('Ctrl Pts',(-0.237109137139568,0.00380985165238374,
-0.0102626509316129));
#26434=CARTESIAN_POINT('Ctrl Pts',(-0.237144687449298,0.0039033834626968,
-0.0103062328088071));
#26435=CARTESIAN_POINT('Ctrl Pts',(-0.237182101443326,0.00400620936376822,
-0.010352031182122));
#26436=CARTESIAN_POINT('Ctrl Pts',(-0.23721831670714,0.00411091512385162,
-0.010396098336241));
#26437=CARTESIAN_POINT('Ctrl Pts',(-0.23723457492686,0.00415792097370976,
-0.0104158815270468));
#26438=CARTESIAN_POINT('Ctrl Pts',(-0.237250591553704,0.00420529857814582,
-0.0104353299151331));
#26439=CARTESIAN_POINT('Ctrl Pts',(-0.237266089505886,0.00425234197839895,
-0.0104541631023438));
#26440=CARTESIAN_POINT('Ctrl Pts',(-0.237316109222227,0.00440417478242368,
-0.0105149473060269));
#26441=CARTESIAN_POINT('Ctrl Pts',(-0.237360714015525,0.00455249920513233,
-0.0105694837750095));
#26442=CARTESIAN_POINT('Ctrl Pts',(-0.237402184731641,0.00470277313262922,
-0.0106202515747131));
#26443=CARTESIAN_POINT('Ctrl Pts',(-0.237485126163871,0.005003320987623,
-0.0107217871741204));
#26444=CARTESIAN_POINT('Ctrl Pts',(-0.237555545013006,0.00531183770396397,
-0.0108076309622602));
#26445=CARTESIAN_POINT('Ctrl Pts',(-0.237611803761463,0.00562137180228855,
-0.0108759573592423));
#26446=CARTESIAN_POINT('Ctrl Pts',(-0.237724321258377,0.0062404399989377,
-0.0110126101532065));
#26447=CARTESIAN_POINT('Ctrl Pts',(-0.23778016147638,0.00686334246713551,
-0.0110808266634648));
#26448=CARTESIAN_POINT('Ctrl Pts',(-0.237780756134355,0.00748828520611799,
-0.0110816774046328));
#26449=CARTESIAN_POINT('Ctrl Pts',(-0.23778075984999,0.00749219007177514,
-0.0110816827203678));
#26450=CARTESIAN_POINT('Ctrl Pts',(-0.237780761409074,0.00749609500352675,
-0.0110816853719659));
#26451=CARTESIAN_POINT('Ctrl Pts',(-0.237780760811121,0.00749999999987464,
-0.0110816853584517));
#26452=CARTESIAN_POINT('Ctrl Pts',(-0.237780665711467,0.0081210586585245,
-0.0110816832091296));
#26453=CARTESIAN_POINT('Ctrl Pts',(-0.237726009720084,0.00874390205312341,
-0.0110147755481997));
#26454=CARTESIAN_POINT('Ctrl Pts',(-0.237614844192197,0.0093617667327187,
-0.0108796617768425));
#26455=CARTESIAN_POINT('Ctrl Pts',(-0.237558911943567,0.00967264152938713,
-0.0108116801174518));
#26456=CARTESIAN_POINT('Ctrl Pts',(-0.237488681296103,0.00998223085392503,
-0.0107261161776055));
#26457=CARTESIAN_POINT('Ctrl Pts',(-0.237405877712267,0.0102838639138477,
-0.0106247544023578));
#26458=CARTESIAN_POINT('Ctrl Pts',(-0.237364475920348,0.0104346804438091,
-0.0105740735147339));
#26459=CARTESIAN_POINT('Ctrl Pts',(-0.237319927437426,0.0105835487558483,
-0.0105195983099089));
#26460=CARTESIAN_POINT('Ctrl Pts',(-0.237269891845089,0.0107360484391602,
-0.0104588008630779));
#26461=CARTESIAN_POINT('Ctrl Pts',(-0.237253187233269,0.0107869611573549,
-0.0104385033568127));
#26462=CARTESIAN_POINT('Ctrl Pts',(-0.237235872411813,0.0108382752930308,
-0.0104174819969918));
#26463=CARTESIAN_POINT('Ctrl Pts',(-0.237218302501169,0.0108890848152787,
-0.0103960980533122));
#26464=CARTESIAN_POINT('Ctrl Pts',(-0.237183244975997,0.0109904658718642,
-0.0103534303267071));
#26465=CARTESIAN_POINT('Ctrl Pts',(-0.237147171867749,0.0110898083390762,
-0.0103092612874042));
#26466=CARTESIAN_POINT('Ctrl Pts',(-0.237112904226435,0.0111802736864231,
-0.0102672450731564));
#26467=CARTESIAN_POINT('Ctrl Pts',(-0.237061462543517,0.0113160778893066,
-0.0102041714361071));
#26468=CARTESIAN_POINT('Ctrl Pts',(-0.237014072093481,0.0114321386325685,
-0.0101465198227962));
#26469=CARTESIAN_POINT('Ctrl Pts',(-0.236962087516987,0.0115527487461073,
-0.0100834191489188));
#26470=CARTESIAN_POINT('Ctrl Pts',(-0.236910102940493,0.0116733588596461,
-0.0100203184750413));
#26471=CARTESIAN_POINT('Ctrl Pts',(-0.236853533870469,0.0117982735066382,
-0.00995131257547577));
#26472=CARTESIAN_POINT('Ctrl Pts',(-0.236794568042232,0.0119213045748546,
-0.00987933188546306));
#26473=CARTESIAN_POINT('Ctrl Pts',(-0.236676636385759,0.0121673667112875,
-0.00973537050543764));
#26474=CARTESIAN_POINT('Ctrl Pts',(-0.236549106830628,0.012406224296211,
-0.00958003617413828));
#26475=CARTESIAN_POINT('Ctrl Pts',(-0.236409420796806,0.0126418686144187,
-0.00940993788674596));
#26476=CARTESIAN_POINT('Ctrl Pts',(-0.236269734762985,0.0128775129326265,
-0.00923983959935364));
#26477=CARTESIAN_POINT('Ctrl Pts',(-0.236117899092723,0.0131097046653902,
-0.0090546383024288));
#26478=CARTESIAN_POINT('Ctrl Pts',(-0.235957462490158,0.013331748912476,
-0.00885861985415937));
#26479=CARTESIAN_POINT('Ctrl Pts',(-0.235877244188876,0.0134427710360188,
-0.00876061063002465));
#26480=CARTESIAN_POINT('Ctrl Pts',(-0.235794873238375,0.0135513550829385,
-0.0086600209302118));
#26481=CARTESIAN_POINT('Ctrl Pts',(-0.235706429188876,0.0136617072842212,
-0.00855229192071309));
#26482=CARTESIAN_POINT('Ctrl Pts',(-0.235682759623755,0.0136912399506845,
-0.00852346127783545));
#26483=CARTESIAN_POINT('Ctrl Pts',(-0.235658655626003,0.013720894062547,
-0.00849411037167573));
#26484=CARTESIAN_POINT('Ctrl Pts',(-0.235634419909639,0.0137503117697787,
-0.008464581126618));
#26485=CARTESIAN_POINT('Ctrl Pts',(-0.235568096087339,0.0138308167054532,
-0.00838377095486792));
#26486=CARTESIAN_POINT('Ctrl Pts',(-0.235500785816309,0.0139094736614859,
-0.00830155764904172));
#26487=CARTESIAN_POINT('Ctrl Pts',(-0.235438693122288,0.0139797160557346,
-0.0082256564292159));
#26488=CARTESIAN_POINT('Ctrl Pts',(-0.235353910829442,0.0140756260711292,
-0.00812201976876574));
#26489=CARTESIAN_POINT('Ctrl Pts',(-0.235278846300897,0.0141562953693376,
-0.00803057258615523));
#26490=CARTESIAN_POINT('Ctrl Pts',(-0.23519776275404,0.0142400036595105,
-0.00793188586844095));
#26491=CARTESIAN_POINT('Ctrl Pts',(-0.235116679207183,0.0143237119496834,
-0.00783319915072666));
#26492=CARTESIAN_POINT('Ctrl Pts',(-0.23502958195438,0.0144100708725911,
-0.00772694763099746));
#26493=CARTESIAN_POINT('Ctrl Pts',(-0.23494168432416,0.0144932752247202,
-0.00761965855480392));
#26494=CARTESIAN_POINT('Ctrl Pts',(-0.23485378669394,0.0145764795768493,
-0.00751236947861039));
#26495=CARTESIAN_POINT('Ctrl Pts',(-0.234765086429372,0.0146567166088885,
-0.00740418831371886));
#26496=CARTESIAN_POINT('Ctrl Pts',(-0.23467045783265,0.0147381470204307,
-0.00728892516558668));
#26497=CARTESIAN_POINT('Ctrl Pts',(-0.234575829235928,0.0148195774319729,
-0.00717366201745451));
#26498=CARTESIAN_POINT('Ctrl Pts',(-0.234475276149762,0.0149018428550239,
-0.00705105563029274));
#26499=CARTESIAN_POINT('Ctrl Pts',(-0.234384083279509,0.014973159658642,
-0.0069397197229418));
#26500=CARTESIAN_POINT('Ctrl Pts',(-0.234292890409256,0.0150444764622601,
-0.00682838381559085));
#26501=CARTESIAN_POINT('Ctrl Pts',(-0.234211053367293,0.0151053712651558,
-0.00672865727439112));
#26502=CARTESIAN_POINT('Ctrl Pts',(-0.234123378056485,0.015167881091967,
-0.00662187470813778));
#26503=CARTESIAN_POINT('Ctrl Pts',(-0.234035702745677,0.0152303909187781,
-0.00651509214188445));
#26504=CARTESIAN_POINT('Ctrl Pts',(-0.233942191406194,0.015294170241559,
-0.006401053727849));
#26505=CARTESIAN_POINT('Ctrl Pts',(-0.233848170620294,0.0153551098348782,
-0.00628632961631849));
#26506=CARTESIAN_POINT('Ctrl Pts',(-0.233754149834394,0.0154160494281974,
-0.00617160550478799));
#26507=CARTESIAN_POINT('Ctrl Pts',(-0.233659618531884,0.0154743434736159,
-0.00605630136650607));
#26508=CARTESIAN_POINT('Ctrl Pts',(-0.233558460970936,0.0155332227250349,
-0.00593303125073153));
#26509=CARTESIAN_POINT('Ctrl Pts',(-0.23347431303379,0.0155822014420113,
-0.00583048898046401));
#26510=CARTESIAN_POINT('Ctrl Pts',(-0.233385581129215,0.0156313533891151,
-0.00572231192292485));
#26511=CARTESIAN_POINT('Ctrl Pts',(-0.233303279293739,0.0156748405665605,
-0.00562186232545755));
#26512=CARTESIAN_POINT('Ctrl Pts',(-0.233286642840047,0.0156836310438269,
-0.00560155749183029));
#26513=CARTESIAN_POINT('Ctrl Pts',(-0.233270269121464,0.0156921965193002,
-0.00558157095462027));
#26514=CARTESIAN_POINT('Ctrl Pts',(-0.233254249108412,0.0157004984529706,
-0.00556201669971721));
#26515=CARTESIAN_POINT('Ctrl Pts',(-0.23315897683986,0.0157498707007693,
-0.00544572601890478));
#26516=CARTESIAN_POINT('Ctrl Pts',(-0.233076213104704,0.0157902460744741,
-0.0053448737747612));
#26517=CARTESIAN_POINT('Ctrl Pts',(-0.232986295777531,0.0158319207926876,
-0.00523531752081867));
#26518=CARTESIAN_POINT('Ctrl Pts',(-0.232896378450358,0.0158735955109011,
-0.00512576126687615));
#26519=CARTESIAN_POINT('Ctrl Pts',(-0.232799307488513,0.0159161860208843,
-0.00500736515900809));
#26520=CARTESIAN_POINT('Ctrl Pts',(-0.232699477083465,0.0159570367517272,
-0.00488562985940448));
#26521=CARTESIAN_POINT('Ctrl Pts',(-0.232599646678417,0.0159978874825702,
-0.00476389455980087));
#26522=CARTESIAN_POINT('Ctrl Pts',(-0.232497057226093,0.0160370420103787,
-0.00463882285759716));
#26523=CARTESIAN_POINT('Ctrl Pts',(-0.232393793026214,0.0160735735624176,
-0.00451286460048705));
#26524=CARTESIAN_POINT('Ctrl Pts',(-0.232342160926274,0.0160918393384371,
-0.00444988547193199));
#26525=CARTESIAN_POINT('Ctrl Pts',(-0.232290360161217,0.0161094961511758,
-0.00438670072149367));
#26526=CARTESIAN_POINT('Ctrl Pts',(-0.232233876486394,0.0161278782621135,
-0.00431784418501812));
#26527=CARTESIAN_POINT('Ctrl Pts',(-0.232177392811571,0.0161462603730512,
-0.00424898764854258));
#26528=CARTESIAN_POINT('Ctrl Pts',(-0.232116225677619,0.0161651614491445,
-0.0041744029891438));
#26529=CARTESIAN_POINT('Ctrl Pts',(-0.232069243605778,0.0161791254692766,
-0.00411709645137768));
#26530=CARTESIAN_POINT('Ctrl Pts',(-0.232022261533936,0.0161930894894088,
-0.00405978991361156));
#26531=CARTESIAN_POINT('Ctrl Pts',(-0.231989465637333,0.0162024097984568,
-0.00401983125579712));
#26532=CARTESIAN_POINT('Ctrl Pts',(-0.231950878188651,0.0162130886498548,
-0.00397282759162673));
#26533=CARTESIAN_POINT('Ctrl Pts',(-0.231912290739969,0.0162237675012527,
-0.00392582392745635));
#26534=CARTESIAN_POINT('Ctrl Pts',(-0.231867911031374,0.0162356469772777,
-0.0038717410533253));
#26535=CARTESIAN_POINT('Ctrl Pts',(-0.231822622786801,0.0162472121451573,
-0.00381654835060898));
#26536=CARTESIAN_POINT('Ctrl Pts',(-0.231732046297657,0.0162703424809165,
-0.00370616294517634));
#26537=CARTESIAN_POINT('Ctrl Pts',(-0.231637836707432,0.0162924051440427,
-0.00359137335257152));
#26538=CARTESIAN_POINT('Ctrl Pts',(-0.231536442028934,0.016313519252232,
-0.00346775641743787));
#26539=CARTESIAN_POINT('Ctrl Pts',(-0.231333654104948,0.0163557471702052,
-0.00322052429424714));
#26540=CARTESIAN_POINT('Ctrl Pts',(-0.231102124372152,0.0163939580101801,
-0.00293796121806425));
#26541=CARTESIAN_POINT('Ctrl Pts',(-0.230845406138858,0.0164188522362164,
-0.00262493214986059));
#26542=CARTESIAN_POINT('',(-0.22989804971791,0.016496143666697,2.94875754215381E-7));
#26543=CARTESIAN_POINT('Ctrl Pts',(-0.22989804971791,0.016496143666697,
2.94875754180074E-7));
#26544=CARTESIAN_POINT('Ctrl Pts',(-0.229898014287119,0.0164961471566313,
-0.000947649746562464));
#26545=CARTESIAN_POINT('Ctrl Pts',(-0.230239453768766,0.0164679382629039,
-0.00189549608053806));
#26546=CARTESIAN_POINT('Ctrl Pts',(-0.230845397069526,0.0164178761451466,
-0.00262486149392285));
#26547=CARTESIAN_POINT('',(-0.22721365317106,0.0165399630933673,2.96878969865867E-7));
#26548=CARTESIAN_POINT('Ctrl Pts',(-0.229898080672427,0.0164981300169968,
2.94888303551387E-7));
#26549=CARTESIAN_POINT('Ctrl Pts',(-0.22721365317106,0.0165399630933672,
2.96878969865846E-7));
#26550=CARTESIAN_POINT('',(-0.234192388872042,0.0132952027870384,-0.00885670411852692));
#26551=CARTESIAN_POINT('Ctrl Pts',(-0.22721365317106,0.0165399630933673,
2.96878969865867E-7));
#26552=CARTESIAN_POINT('Ctrl Pts',(-0.227256908958651,0.0165392899807157,
-0.000116960173666361));
#26553=CARTESIAN_POINT('Ctrl Pts',(-0.227339124107497,0.0165367236578279,
-0.00033776437467711));
#26554=CARTESIAN_POINT('Ctrl Pts',(-0.227420071905186,0.0165329358482603,
-0.000553615272546889));
#26555=CARTESIAN_POINT('Ctrl Pts',(-0.227547101717011,0.0165249913814539,
-0.000878058900339982));
#26556=CARTESIAN_POINT('Ctrl Pts',(-0.22768815065478,0.0165141789319858,
-0.00121703749323916));
#26557=CARTESIAN_POINT('Ctrl Pts',(-0.227909366795336,0.0164944334295571,
-0.00169626548164348));
#26558=CARTESIAN_POINT('Ctrl Pts',(-0.228192601673969,0.0164694168554863,
-0.00221811204306224));
#26559=CARTESIAN_POINT('Ctrl Pts',(-0.228511119230705,0.0164359317145672,
-0.00274316378074596));
#26560=CARTESIAN_POINT('Ctrl Pts',(-0.228965207170631,0.0163483003756339,
-0.00341891990378775));
#26561=CARTESIAN_POINT('Ctrl Pts',(-0.229483054805567,0.0162096171069562,
-0.00406485955552118));
#26562=CARTESIAN_POINT('Ctrl Pts',(-0.229924175135309,0.0160759507361103,
-0.00452880943524848));
#26563=CARTESIAN_POINT('Ctrl Pts',(-0.230206707176665,0.0159866029159255,
-0.00480698677163651));
#26564=CARTESIAN_POINT('Ctrl Pts',(-0.230453694447789,0.015905557072168,
-0.00503765884127183));
#26565=CARTESIAN_POINT('Ctrl Pts',(-0.230627130821605,0.0158469989122931,
-0.00519355104939717));
#26566=CARTESIAN_POINT('Ctrl Pts',(-0.230845400469471,0.0157712591827807,
-0.00538515294067697));
#26567=CARTESIAN_POINT('Ctrl Pts',(-0.231034958715161,0.0157030686492419,
-0.00554683158695247));
#26568=CARTESIAN_POINT('Ctrl Pts',(-0.231182239317623,0.0156484588841278,
-0.00567000124877424));
#26569=CARTESIAN_POINT('Ctrl Pts',(-0.23126064767078,0.0156190133729797,
-0.00573503100777596));
#26570=CARTESIAN_POINT('Ctrl Pts',(-0.231343320990274,0.0155875483379559,
-0.00580304400235552));
#26571=CARTESIAN_POINT('Ctrl Pts',(-0.23134058848968,0.0155885738204978,
-0.00580073392463057));
#26572=CARTESIAN_POINT('Ctrl Pts',(-0.231385286047413,0.0155715171280465,
-0.00583726350714204));
#26573=CARTESIAN_POINT('Ctrl Pts',(-0.231459731254797,0.0155427769176357,
-0.00589778478912086));
#26574=CARTESIAN_POINT('Ctrl Pts',(-0.231588540995542,0.015492298062324,
-0.00600217942498043));
#26575=CARTESIAN_POINT('Ctrl Pts',(-0.231797916190688,0.0154069459195584,
-0.00617020369122395));
#26576=CARTESIAN_POINT('Ctrl Pts',(-0.231913738714637,0.015357925109019,
-0.00626257469253834));
#26577=CARTESIAN_POINT('Ctrl Pts',(-0.232036361551522,0.0153050086703646,
-0.00636048115638375));
#26578=CARTESIAN_POINT('Ctrl Pts',(-0.23214529893423,0.0152564410924344,
-0.00644752873286008));
#26579=CARTESIAN_POINT('Ctrl Pts',(-0.232222140947088,0.0152216138188694,
-0.00650905373166038));
#26580=CARTESIAN_POINT('Ctrl Pts',(-0.232361013019894,0.0151566147032964,
-0.00662098807208995));
#26581=CARTESIAN_POINT('Ctrl Pts',(-0.232511179434643,0.0150830306094505,
-0.00674346122390688));
#26582=CARTESIAN_POINT('Ctrl Pts',(-0.232661263135366,0.0150065039878354,
-0.00686741025236411));
#26583=CARTESIAN_POINT('Ctrl Pts',(-0.232900428682406,0.0148719157351182,
-0.00707399253491582));
#26584=CARTESIAN_POINT('Ctrl Pts',(-0.233081122635965,0.014759363715995,
-0.00723794642342912));
#26585=CARTESIAN_POINT('Ctrl Pts',(-0.233292763592228,0.014610902022631,
-0.0074435244792244));
#26586=CARTESIAN_POINT('Ctrl Pts',(-0.233522503099131,0.014424811635409,
-0.00768695917044636));
#26587=CARTESIAN_POINT('Ctrl Pts',(-0.233917538413758,0.0140205182082748,
-0.00817494331998796));
#26588=CARTESIAN_POINT('Ctrl Pts',(-0.234124037654978,0.0136070371323653,
-0.0085899342809721));
#26589=CARTESIAN_POINT('Ctrl Pts',(-0.234192388872042,0.0132952027870384,
-0.00885670411852691));
#26590=CARTESIAN_POINT('',(-0.230846395327677,0.00748914570500684,-0.0109249562858334));
#26591=CARTESIAN_POINT('Ctrl Pts',(-0.234192388872042,0.0132952027870384,
-0.00885670411852691));
#26592=CARTESIAN_POINT('Ctrl Pts',(-0.234260740089107,0.0129833684417114,
-0.00912347395608173));
#26593=CARTESIAN_POINT('Ctrl Pts',(-0.23425929449908,0.0124613464816401,
-0.00950879250776204));
#26594=CARTESIAN_POINT('Ctrl Pts',(-0.234077282934937,0.0118177007721254,
-0.0098888395261885));
#26595=CARTESIAN_POINT('Ctrl Pts',(-0.233826670793196,0.0112512047590739,
-0.0101709376840775));
#26596=CARTESIAN_POINT('Ctrl Pts',(-0.233610338176317,0.0108796222191891,
-0.0103246296716289));
#26597=CARTESIAN_POINT('Ctrl Pts',(-0.233394114013919,0.0105446557132715,
-0.010448281869205));
#26598=CARTESIAN_POINT('Ctrl Pts',(-0.233195095532645,0.01026174721601,
-0.0105405956701664));
#26599=CARTESIAN_POINT('Ctrl Pts',(-0.233051178813437,0.0100683811397472,
-0.0105975374989383));
#26600=CARTESIAN_POINT('Ctrl Pts',(-0.232868465840991,0.00983137860329251,
-0.0106613388492261));
#26601=CARTESIAN_POINT('Ctrl Pts',(-0.232679944650818,0.00959553063661281,
-0.0107177886081924));
#26602=CARTESIAN_POINT('Ctrl Pts',(-0.232447561116175,0.00931433765584752,
-0.0107753562428179));
#26603=CARTESIAN_POINT('Ctrl Pts',(-0.232290543708524,0.00912877171699688,
-0.0108078703367909));
#26604=CARTESIAN_POINT('Ctrl Pts',(-0.232095278994658,0.00890055703141569,
-0.0108433208555711));
#26605=CARTESIAN_POINT('Ctrl Pts',(-0.231920471854683,0.00869940054062883,
-0.0108683999653081));
#26606=CARTESIAN_POINT('Ctrl Pts',(-0.231782694028032,0.00854205404621492,
-0.0108851588016013));
#26607=CARTESIAN_POINT('Ctrl Pts',(-0.23164586132212,0.00838689206622596,
-0.0108987817482543));
#26608=CARTESIAN_POINT('Ctrl Pts',(-0.231618960279246,0.00835662431924158,
-0.0109009619444762));
#26609=CARTESIAN_POINT('Ctrl Pts',(-0.231521063942898,0.00824631142819562,
-0.0109091055405001));
#26610=CARTESIAN_POINT('Ctrl Pts',(-0.23132077524562,0.00802129497745352,
-0.010922259755925));
#26611=CARTESIAN_POINT('Ctrl Pts',(-0.23105771540997,0.00772600187303795,
-0.0109300225734977));
#26612=CARTESIAN_POINT('Ctrl Pts',(-0.230846362800463,0.00748918187660458,
-0.0109249555950961));
#26613=CARTESIAN_POINT('',(-0.227214261715267,-0.00153995361067246,2.08417333140297E-7));
#26614=CARTESIAN_POINT('Ctrl Pts',(-0.230846395327677,0.00748914570500684,
-0.0109249562858334));
#26615=CARTESIAN_POINT('Ctrl Pts',(-0.231037606532753,0.00727651095947488,
-0.0109290163499947));
#26616=CARTESIAN_POINT('Ctrl Pts',(-0.231284925260294,0.00700085820481965,
-0.0109227670625044));
#26617=CARTESIAN_POINT('Ctrl Pts',(-0.231493557178275,0.00676788077232978,
-0.0109097315243095));
#26618=CARTESIAN_POINT('Ctrl Pts',(-0.231602263022381,0.0066461470035044,
-0.0109008810664884));
#26619=CARTESIAN_POINT('Ctrl Pts',(-0.231644664597747,0.00659866149517143,
-0.0108973277547739));
#26620=CARTESIAN_POINT('Ctrl Pts',(-0.231786496142884,0.00643900367334659,
-0.0108830165106154));
#26621=CARTESIAN_POINT('Ctrl Pts',(-0.231931242135863,0.00627498686834051,
-0.0108651664231131));
#26622=CARTESIAN_POINT('Ctrl Pts',(-0.232108355058939,0.006072781544978,
-0.0108393204957513));
#26623=CARTESIAN_POINT('Ctrl Pts',(-0.232300210417243,0.00584995171828157,
-0.0108039990190336));
#26624=CARTESIAN_POINT('Ctrl Pts',(-0.232440153445732,0.00568521883709722,
-0.0107749745621213));
#26625=CARTESIAN_POINT('Ctrl Pts',(-0.232667681706468,0.00540944023166544,
-0.0107186770907011));
#26626=CARTESIAN_POINT('Ctrl Pts',(-0.232852296030784,0.00517740019893589,
-0.0106633253293673));
#26627=CARTESIAN_POINT('Ctrl Pts',(-0.233034515083928,0.00493973862584453,
-0.0105996345989168));
#26628=CARTESIAN_POINT('Ctrl Pts',(-0.233182763373576,0.0047393646700024,
-0.0105407789701458));
#26629=CARTESIAN_POINT('Ctrl Pts',(-0.233382824203779,0.00445405678985819,
-0.0104474408102256));
#26630=CARTESIAN_POINT('Ctrl Pts',(-0.233543139477693,0.00420824923383913,
-0.0103572130276457));
#26631=CARTESIAN_POINT('Ctrl Pts',(-0.233691663906295,0.00396150500429967,
-0.0102577963056457));
#26632=CARTESIAN_POINT('Ctrl Pts',(-0.233808136742523,0.00375087363724476,
-0.0101661685139463));
#26633=CARTESIAN_POINT('Ctrl Pts',(-0.233945646263649,0.00346795331697028,
-0.0100321308653909));
#26634=CARTESIAN_POINT('Ctrl Pts',(-0.234083992220015,0.00312423902231311,
-0.00985264023662205));
#26635=CARTESIAN_POINT('Ctrl Pts',(-0.234256483655326,0.00254094086020491,
-0.00951179687589967));
#26636=CARTESIAN_POINT('Ctrl Pts',(-0.234262850553755,0.00186094978727132,
-0.00900885554389722));
#26637=CARTESIAN_POINT('Ctrl Pts',(-0.234068396622431,0.00128735914064042,
-0.00848231918710256));
#26638=CARTESIAN_POINT('Ctrl Pts',(-0.233817874309389,0.000881927623917763,
-0.00805541563716329));
#26639=CARTESIAN_POINT('Ctrl Pts',(-0.2335704994029,0.000620516072173728,
-0.00774327437066843));
#26640=CARTESIAN_POINT('Ctrl Pts',(-0.233329249078638,0.000415582269566412,
-0.00747932099276584));
#26641=CARTESIAN_POINT('Ctrl Pts',(-0.233112960961304,0.000260399852082621,
-0.00726601341584551));
#26642=CARTESIAN_POINT('Ctrl Pts',(-0.23293403930091,0.000146997261486484,
-0.00710214095492278));
#26643=CARTESIAN_POINT('Ctrl Pts',(-0.232690819740965,8.6463822485961E-6,
-0.00689139571371004));
#26644=CARTESIAN_POINT('Ctrl Pts',(-0.232534580033651,-7.16401286118548E-5,
-0.00676206118639177));
#26645=CARTESIAN_POINT('Ctrl Pts',(-0.232384733682554,-0.00014564407532251,
-0.00663951871985647));
#26646=CARTESIAN_POINT('Ctrl Pts',(-0.232246570420582,-0.000210741619390237,
-0.00652795918919056));
#26647=CARTESIAN_POINT('Ctrl Pts',(-0.2321756309133,-0.00024311721387142,
-0.00647117665620728));
#26648=CARTESIAN_POINT('Ctrl Pts',(-0.232027018331408,-0.000309581030025878,
-0.00635248279855617));
#26649=CARTESIAN_POINT('Ctrl Pts',(-0.231873513645315,-0.000375942995292352,
-0.00623044356967292));
#26650=CARTESIAN_POINT('Ctrl Pts',(-0.231629252180028,-0.000476033427381937,
-0.00603466477165482));
#26651=CARTESIAN_POINT('Ctrl Pts',(-0.231501652837513,-0.000526562181469526,
-0.00593145040725404));
#26652=CARTESIAN_POINT('Ctrl Pts',(-0.231423161461155,-0.000557113181751774,
-0.00586770399101785));
#26653=CARTESIAN_POINT('Ctrl Pts',(-0.231370959763619,-0.000577174803723653,
-0.00582510216694446));
#26654=CARTESIAN_POINT('Ctrl Pts',(-0.23136223630703,-0.000580549023227225,
-0.00581801997224131));
#26655=CARTESIAN_POINT('Ctrl Pts',(-0.231279110464189,-0.000612251054423109,
-0.00574980208365006));
#26656=CARTESIAN_POINT('Ctrl Pts',(-0.231196728277073,-0.000643235046653219,
-0.0056816723984767));
#26657=CARTESIAN_POINT('Ctrl Pts',(-0.231045192907986,-0.000699432810574991,
-0.00555531580229769));
#26658=CARTESIAN_POINT('Ctrl Pts',(-0.230851532314107,-0.000768988555986341,
-0.00539073770637673));
#26659=CARTESIAN_POINT('Ctrl Pts',(-0.230632644958823,-0.000844755027883067,
-0.00519931949444886));
#26660=CARTESIAN_POINT('Ctrl Pts',(-0.230464821727732,-0.000901324892749503,
-0.00504914540426946));
#26661=CARTESIAN_POINT('Ctrl Pts',(-0.230220831803887,-0.000981615469461095,
-0.00482173766606306));
#26662=CARTESIAN_POINT('Ctrl Pts',(-0.229938496083015,-0.00107153756204175,
-0.00454364289308824));
#26663=CARTESIAN_POINT('Ctrl Pts',(-0.22947806967778,-0.00121182703178667,
-0.00405820411123181));
#26664=CARTESIAN_POINT('Ctrl Pts',(-0.228966516318197,-0.00134816943216903,
-0.0034170007972907));
#26665=CARTESIAN_POINT('Ctrl Pts',(-0.228579626600758,-0.00142248587384968,
-0.00284576218835118));
#26666=CARTESIAN_POINT('Ctrl Pts',(-0.228348114652924,-0.00145443014710487,
-0.00247619241680766));
#26667=CARTESIAN_POINT('Ctrl Pts',(-0.228153271627853,-0.00147191766978348,
-0.00214698541707847));
#26668=CARTESIAN_POINT('Ctrl Pts',(-0.227950831685064,-0.00149080064913227,
-0.00177093667718264));
#26669=CARTESIAN_POINT('Ctrl Pts',(-0.227785980543934,-0.00150568050665454,
-0.0014278840996034));
#26670=CARTESIAN_POINT('Ctrl Pts',(-0.227652169250544,-0.00151706650701674,
-0.0011265269211914));
#26671=CARTESIAN_POINT('Ctrl Pts',(-0.227566987533402,-0.00152351882163508,
-0.000920126530996759));
#26672=CARTESIAN_POINT('Ctrl Pts',(-0.227491225966645,-0.00152867067867476,
-0.000731050631136379));
#26673=CARTESIAN_POINT('Ctrl Pts',(-0.22742256682371,-0.00153264846383891,
-0.000554599488887733));
#26674=CARTESIAN_POINT('Ctrl Pts',(-0.227392474361708,-0.00153416030791209,
-0.000475545942274294));
#26675=CARTESIAN_POINT('Ctrl Pts',(-0.227323585473763,-0.00153729398439594,
-0.000293428211194043));
#26676=CARTESIAN_POINT('Ctrl Pts',(-0.227262110333096,-0.00153920870389092,
-0.00012867603536092));
#26677=CARTESIAN_POINT('Ctrl Pts',(-0.227214261715267,-0.00153995361067246,
2.08417333140297E-7));
#26678=CARTESIAN_POINT('',(-0.228146745678798,-0.00146986864564724,0.00219071825850764));
#26679=CARTESIAN_POINT('Ctrl Pts',(-0.227214261703447,-0.00153995361085648,
2.08449182843721E-7));
#26680=CARTESIAN_POINT('Ctrl Pts',(-0.227260878765733,-0.00153922641144584,
0.000127297385581003));
#26681=CARTESIAN_POINT('Ctrl Pts',(-0.227320680330025,-0.00153736227316047,
0.000289652208553862));
#26682=CARTESIAN_POINT('Ctrl Pts',(-0.227387409157731,-0.00153432194063922,
0.000468825060106595));
#26683=CARTESIAN_POINT('Ctrl Pts',(-0.227416469548984,-0.00153285820742312,
0.000546456828516538));
#26684=CARTESIAN_POINT('Ctrl Pts',(-0.227482475446119,-0.00152901542348585,
0.00071963165722293));
#26685=CARTESIAN_POINT('Ctrl Pts',(-0.22755518908399,-0.00152402406154442,
0.000905839279240665));
#26686=CARTESIAN_POINT('Ctrl Pts',(-0.227636477856155,-0.00151777931669379,
0.00110910239215292));
#26687=CARTESIAN_POINT('Ctrl Pts',(-0.227764726003692,-0.0015065682063797,
0.00141079945586991));
#26688=CARTESIAN_POINT('Ctrl Pts',(-0.227915639874086,-0.00149228529545111,
0.0017430864187612));
#26689=CARTESIAN_POINT('Ctrl Pts',(-0.228055314183631,-0.0014789629619799,
0.00201933604813241));
#26690=CARTESIAN_POINT('Ctrl Pts',(-0.228146745678798,-0.00146986864564724,
0.00219071825850764));
#26691=CARTESIAN_POINT('',(-0.233559158081792,0.00387416783145173,0.0102155391996269));
#26692=CARTESIAN_POINT('Ctrl Pts',(-0.228146745678798,-0.00146986864564724,
0.00219071825850764));
#26693=CARTESIAN_POINT('Ctrl Pts',(-0.228147602077471,-0.00146978346317885,
0.0021923235204298));
#26694=CARTESIAN_POINT('Ctrl Pts',(-0.22824073305991,-0.0014605164879658,
0.00236679973700088));
#26695=CARTESIAN_POINT('Ctrl Pts',(-0.228423001865608,-0.00144158884393021,
0.00268844823641635));
#26696=CARTESIAN_POINT('Ctrl Pts',(-0.228762913960931,-0.00137415185924898,
0.00323117458741793));
#26697=CARTESIAN_POINT('Ctrl Pts',(-0.229113014450919,-0.00128145526964443,
0.00373771571845669));
#26698=CARTESIAN_POINT('Ctrl Pts',(-0.229472512500946,-0.00117031797297195,
0.00420354730297736));
#26699=CARTESIAN_POINT('Ctrl Pts',(-0.229771684855995,-0.00106991162198901,
0.00455062609318909));
#26700=CARTESIAN_POINT('Ctrl Pts',(-0.230037581767111,-0.000975694344253686,
0.00484005819884158));
#26701=CARTESIAN_POINT('Ctrl Pts',(-0.230268198085539,-0.000890512288748131,
0.00507885332770519));
#26702=CARTESIAN_POINT('Ctrl Pts',(-0.230434510419619,-0.000827067762574278,
0.00524460327337801));
#26703=CARTESIAN_POINT('Ctrl Pts',(-0.230638435249322,-0.000747124311760387,
0.00544285167783606));
#26704=CARTESIAN_POINT('Ctrl Pts',(-0.230820428072529,-0.00067292550390027,
0.00561426715448736));
#26705=CARTESIAN_POINT('Ctrl Pts',(-0.230968589245136,-0.00061090734263518,
0.0057512581323597));
#26706=CARTESIAN_POINT('Ctrl Pts',(-0.231102505812003,-0.000553517619805691,
0.00587311727066912));
#26707=CARTESIAN_POINT('Ctrl Pts',(-0.231169109311276,-0.000524526572001451,
0.00593304385290676));
#26708=CARTESIAN_POINT('Ctrl Pts',(-0.231310613527498,-0.000461990851617312,
0.00605961198957369));
#26709=CARTESIAN_POINT('Ctrl Pts',(-0.231447457908593,-0.000400412033682357,
0.00618086667324984));
#26710=CARTESIAN_POINT('Ctrl Pts',(-0.231691440631806,-0.000284675731091188,
0.00639373778767496));
#26711=CARTESIAN_POINT('Ctrl Pts',(-0.231813023978218,-0.00022486405856557,
0.00649884984694274));
#26712=CARTESIAN_POINT('Ctrl Pts',(-0.231884446809911,-0.000189209465118761,
0.00656034920502148));
#26713=CARTESIAN_POINT('Ctrl Pts',(-0.231930078039368,-0.000166097177273578,
0.00659958595864139));
#26714=CARTESIAN_POINT('Ctrl Pts',(-0.231931289957848,-0.000165561101604138,
0.00660060687576811));
#26715=CARTESIAN_POINT('Ctrl Pts',(-0.232013321018402,-0.000123494859710195,
0.00667129148969066));
#26716=CARTESIAN_POINT('Ctrl Pts',(-0.232089020337746,-8.38348221208054E-5,
0.00673658587661242));
#26717=CARTESIAN_POINT('Ctrl Pts',(-0.232184758140682,-3.26941779414291E-5,
0.00681932067970241));
#26718=CARTESIAN_POINT('Ctrl Pts',(-0.232285526066454,2.31781819879938E-5,
0.006907053513387));
#26719=CARTESIAN_POINT('Ctrl Pts',(-0.232387404877587,8.09008443525465E-5,
0.00699635079756444));
#26720=CARTESIAN_POINT('Ctrl Pts',(-0.232596018354059,0.000207336010577208,
0.00718429347931461));
#26721=CARTESIAN_POINT('Ctrl Pts',(-0.232761955293696,0.00031852348252791,
0.00734069697033025));
#26722=CARTESIAN_POINT('Ctrl Pts',(-0.232977684545184,0.000479357868993146,
0.00755646663238428));
#26723=CARTESIAN_POINT('Ctrl Pts',(-0.233216413918051,0.000686789932042174,
0.00781703214787861));
#26724=CARTESIAN_POINT('Ctrl Pts',(-0.233465871951339,0.000950568046321459,
0.0081241062900768));
#26725=CARTESIAN_POINT('Ctrl Pts',(-0.233724009566518,0.00134408173329303,
0.00853029830649302));
#26726=CARTESIAN_POINT('Ctrl Pts',(-0.233947136086876,0.00191722301985356,
0.00904721293907608));
#26727=CARTESIAN_POINT('Ctrl Pts',(-0.233978600563923,0.0025686995100556,
0.00952461220572329));
#26728=CARTESIAN_POINT('Ctrl Pts',(-0.233824605334425,0.00326097954767997,
0.00992663531592156));
#26729=CARTESIAN_POINT('Ctrl Pts',(-0.233668400615857,0.00364781188257956,
0.0101152447960562));
#26730=CARTESIAN_POINT('Ctrl Pts',(-0.23357525881827,0.0038415964420142,
0.0102013285012318));
#26731=CARTESIAN_POINT('Ctrl Pts',(-0.233559158081792,0.00387416783145173,
0.0102155391996269));
#26732=CARTESIAN_POINT('',(-0.230731189036971,0.00749156929015138,0.0109223560943954));
#26733=CARTESIAN_POINT('Ctrl Pts',(-0.233559158081792,0.00387416783145173,
0.0102155391996269));
#26734=CARTESIAN_POINT('Ctrl Pts',(-0.23349648849709,0.00400094684258756,
0.0102708521083235));
#26735=CARTESIAN_POINT('Ctrl Pts',(-0.233387193213595,0.00419960150239789,
0.0103510897124964));
#26736=CARTESIAN_POINT('Ctrl Pts',(-0.233204445962594,0.00449845474264293,
0.0104595791887194));
#26737=CARTESIAN_POINT('Ctrl Pts',(-0.233016552168204,0.00477901086038231,
0.0105498350650121));
#26738=CARTESIAN_POINT('Ctrl Pts',(-0.232874853074723,0.00497762326969598,
0.0106073454722064));
#26739=CARTESIAN_POINT('Ctrl Pts',(-0.232699278541195,0.00521304060449747,
0.0106694214007349));
#26740=CARTESIAN_POINT('Ctrl Pts',(-0.232519935104301,0.00544312585676357,
0.0107234137638662));
#26741=CARTESIAN_POINT('Ctrl Pts',(-0.232296466758271,0.0057176608256759,
0.0107784200472414));
#26742=CARTESIAN_POINT('Ctrl Pts',(-0.2321601909895,0.005879437380212,0.0108063414559013));
#26743=CARTESIAN_POINT('Ctrl Pts',(-0.231972161329767,0.00609921295264491,
0.0108404751193834));
#26744=CARTESIAN_POINT('Ctrl Pts',(-0.231798532022978,0.00629809753013036,
0.0108653480625757));
#26745=CARTESIAN_POINT('Ctrl Pts',(-0.231656082292353,0.00645982495895992,
0.0108825388725517));
#26746=CARTESIAN_POINT('Ctrl Pts',(-0.231517490918546,0.00661596135611126,
0.0108962031604773));
#26747=CARTESIAN_POINT('Ctrl Pts',(-0.23147265186694,0.0066661781042074,
0.0108998770348921));
#26748=CARTESIAN_POINT('Ctrl Pts',(-0.231363974605798,0.00678783230812327,
0.0109084325591462));
#26749=CARTESIAN_POINT('Ctrl Pts',(-0.231157030865224,0.00701863801538526,
0.0109208112149785));
#26750=CARTESIAN_POINT('Ctrl Pts',(-0.230916142610404,0.00728648998098758,
0.0109263403628976));
#26751=CARTESIAN_POINT('Ctrl Pts',(-0.230731189036971,0.00749156929015138,
0.0109223560943954));
#26752=CARTESIAN_POINT('Ctrl Pts',(-0.230731256923034,0.00749164497516978,
0.0109223577006114));
#26753=CARTESIAN_POINT('Ctrl Pts',(-0.230865473404667,0.00764128056035402,
0.0109255326522603));
#26754=CARTESIAN_POINT('Ctrl Pts',(-0.231137213619827,0.007943171205309,
0.0109239758885947));
#26755=CARTESIAN_POINT('Ctrl Pts',(-0.231527434485224,0.00837845914315948,
0.0109008726614748));
#26756=CARTESIAN_POINT('Ctrl Pts',(-0.231887509950401,0.00879119523216391,
0.0108567873229259));
#26757=CARTESIAN_POINT('Ctrl Pts',(-0.232140469910439,0.00909048844268248,
0.010811556341717));
#26758=CARTESIAN_POINT('Ctrl Pts',(-0.232300596136593,0.00928297039316321,
0.0107785093165595));
#26759=CARTESIAN_POINT('Ctrl Pts',(-0.232520666812517,0.00955532757019838,
0.0107237698902202));
#26760=CARTESIAN_POINT('Ctrl Pts',(-0.232703137061035,0.00979022573944132,
0.0106686900691618));
#26761=CARTESIAN_POINT('Ctrl Pts',(-0.232879255800725,0.01002672215703,
0.0106061668367168));
#26762=CARTESIAN_POINT('Ctrl Pts',(-0.233021572234454,0.0102258389513203,
0.0105483766090537));
#26763=CARTESIAN_POINT('Ctrl Pts',(-0.233208640632173,0.0105045789283705,
0.0104586041345504));
#26764=CARTESIAN_POINT('Ctrl Pts',(-0.233412050346818,0.0108382118461368,
0.0103371779477693));
#26765=CARTESIAN_POINT('Ctrl Pts',(-0.233613248968386,0.0112102121412998,
0.0101851544377368));
#26766=CARTESIAN_POINT('Ctrl Pts',(-0.233834860767148,0.0117711747306955,
0.00990917052441051));
#26767=CARTESIAN_POINT('Ctrl Pts',(-0.233983453677809,0.0124159974365663,
0.00953355738971462));
#26768=CARTESIAN_POINT('Ctrl Pts',(-0.233945755044452,0.0131099715084786,
0.00902520045927226));
#26769=CARTESIAN_POINT('Ctrl Pts',(-0.233729334532907,0.0136536630448554,
0.00853186537754338));
#26770=CARTESIAN_POINT('Ctrl Pts',(-0.233466543057227,0.0140565862100828,
0.00811722384353614));
#26771=CARTESIAN_POINT('Ctrl Pts',(-0.233203818000884,0.0143303903479438,
0.00779638666024062));
#26772=CARTESIAN_POINT('Ctrl Pts',(-0.232969475121551,0.0145316536102632,
0.00754200761475823));
#26773=CARTESIAN_POINT('Ctrl Pts',(-0.232762493362533,0.0146856837232449,
0.00733514778261602));
#26774=CARTESIAN_POINT('Ctrl Pts',(-0.232616233535089,0.0147821994045361,
0.00719838339891441));
#26775=CARTESIAN_POINT('Ctrl Pts',(-0.232480708209145,0.0148666127866986,
0.00707499743246925));
#26776=CARTESIAN_POINT('Ctrl Pts',(-0.232356994919711,0.0149394474803228,
0.00696495782458427));
#26777=CARTESIAN_POINT('Ctrl Pts',(-0.232289559739574,0.014977518626712,
0.00690602252937239));
#26778=CARTESIAN_POINT('Ctrl Pts',(-0.23218861866623,0.0150333261724313,
0.00681837562717864));
#26779=CARTESIAN_POINT('Ctrl Pts',(-0.23209277942457,0.0150844247157454,
0.00673569208947289));
#26780=CARTESIAN_POINT('Ctrl Pts',(-0.232015087271052,0.0151250700285569,
0.00666873519572026));
#26781=CARTESIAN_POINT('Ctrl Pts',(-0.23193248413974,0.0151673972827789,
0.00659755450821913));
#26782=CARTESIAN_POINT('Ctrl Pts',(-0.23192477458317,0.0151712366444997,
0.00659092566948877));
#26783=CARTESIAN_POINT('Ctrl Pts',(-0.231874843378034,0.0151964734507034,
0.00654794895099817));
#26784=CARTESIAN_POINT('Ctrl Pts',(-0.231801186064193,0.0152331557486462,
0.00648446076737892));
#26785=CARTESIAN_POINT('Ctrl Pts',(-0.231680565445703,0.0152922140924725,
0.0063800594780042));
#26786=CARTESIAN_POINT('Ctrl Pts',(-0.231456644767689,0.0153983363574462,
0.00618473126690153));
#26787=CARTESIAN_POINT('Ctrl Pts',(-0.231287273794767,0.0154745756686466,
0.00603488776572405));
#26788=CARTESIAN_POINT('Ctrl Pts',(-0.231151897129242,0.0155338645319709,
0.00591370665668096));
#26789=CARTESIAN_POINT('Ctrl Pts',(-0.231105123945984,0.0155541968768278,
0.00587172310084077));
#26790=CARTESIAN_POINT('Ctrl Pts',(-0.230963177640927,0.0156149638966239,
0.00574254549492409));
#26791=CARTESIAN_POINT('Ctrl Pts',(-0.230814830287228,0.0156768473199735,
0.00560537069730955));
#26792=CARTESIAN_POINT('Ctrl Pts',(-0.230630359191633,0.0157517758844927,
0.00543176645051644));
#26793=CARTESIAN_POINT('Ctrl Pts',(-0.230426865261854,0.0158311425106513,
0.00523416260499648));
#26794=CARTESIAN_POINT('Ctrl Pts',(-0.230262165941671,0.0158936258990308,
0.00507035518297227));
#26795=CARTESIAN_POINT('Ctrl Pts',(-0.230036237901951,0.0159768319316395,
0.00483654815190377));
#26796=CARTESIAN_POINT('Ctrl Pts',(-0.229773023242685,0.0160702611120349,
0.00454967053487877));
#26797=CARTESIAN_POINT('Ctrl Pts',(-0.229347345537255,0.0162132627607145,
0.00405272807923008));
#26798=CARTESIAN_POINT('Ctrl Pts',(-0.228795080335764,0.0163782893771517,
0.00329870162389577));
#26799=CARTESIAN_POINT('Ctrl Pts',(-0.228391997949756,0.0164411429389733,
0.00263302315211825));
#26800=CARTESIAN_POINT('Ctrl Pts',(-0.228219847986792,0.016461711610013,
0.00232234304728456));
#26801=CARTESIAN_POINT('Ctrl Pts',(-0.185723055456904,0.00596900147723498,
0.00978267384703966));
#26802=CARTESIAN_POINT('Ctrl Pts',(-0.23232670433304,0.00586421401192308,
0.0108066948117815));
#26803=CARTESIAN_POINT('Ctrl Pts',(-0.185723055456904,0.00647508645933998,
0.00986397141884284));
#26804=CARTESIAN_POINT('Ctrl Pts',(-0.23232670433304,0.00640326228709296,
0.0109072089909106));
#26805=CARTESIAN_POINT('Ctrl Pts',(-0.185723055456904,0.00806363535647837,
0.00999158316816427));
#26806=CARTESIAN_POINT('Ctrl Pts',(-0.23232670433304,0.00810313394959613,
0.011065956770795));
#26807=CARTESIAN_POINT('Ctrl Pts',(-0.185723055456904,0.0107282763804236,
0.00954209216522276));
#26808=CARTESIAN_POINT('Ctrl Pts',(-0.232326704333039,0.010954508418149,
0.0105067943176979));
#26809=CARTESIAN_POINT('Ctrl Pts',(-0.185723055456904,0.0136025641905403,
0.00796594412564821));
#26810=CARTESIAN_POINT('Ctrl Pts',(-0.23232670433304,0.0138912062742137,
0.00858048215857484));
#26811=CARTESIAN_POINT('Ctrl Pts',(-0.185723055456904,0.0158049553585666,
0.0055255423033021));
#26812=CARTESIAN_POINT('Ctrl Pts',(-0.232326704333039,0.0158790519814133,
0.00570322651640249));
#26813=CARTESIAN_POINT('Ctrl Pts',(-0.185723055456903,0.0166573800152265,
0.00349659872621015));
#26814=CARTESIAN_POINT('Ctrl Pts',(-0.232326704333039,0.0163854748419429,
0.00344344619705094));
#26815=CARTESIAN_POINT('Ctrl Pts',(-0.185723055456903,0.0169037490465727,
0.00243669718465325));
#26816=CARTESIAN_POINT('Ctrl Pts',(-0.232326704333039,0.0164203047763951,
0.00231142721965168));
#26817=CARTESIAN_POINT('Ctrl Pts',(-0.185723055456903,0.0169917319681535,
0.0020581868105832));
#26818=CARTESIAN_POINT('Ctrl Pts',(-0.232326704333039,0.0164327431878904,
0.00190716238014556));
#26819=CARTESIAN_POINT('Ctrl Pts',(-0.185723055456904,0.0171348389058692,
0.00126455176521327));
#26820=CARTESIAN_POINT('Ctrl Pts',(-0.232326704333039,0.0164529746481233,
0.00113116956517427));
#26821=CARTESIAN_POINT('Ctrl Pts',(-0.185723055456903,0.0172123852537007,
-4.57104323127425E-14));
#26822=CARTESIAN_POINT('Ctrl Pts',(-0.232326704333039,0.0164639376096499,
-5.12643732643055E-15));
#26823=CARTESIAN_POINT('Ctrl Pts',(-0.185723055456904,0.0171348389058572,
-0.00126455176530287));
#26824=CARTESIAN_POINT('Ctrl Pts',(-0.232326704333039,0.0164529746481216,
-0.00113116956518479));
#26825=CARTESIAN_POINT('Ctrl Pts',(-0.185723055456903,0.0169917319681347,
-0.00205818681066974));
#26826=CARTESIAN_POINT('Ctrl Pts',(-0.232326704333039,0.0164327431878878,
-0.00190716238015681));
#26827=CARTESIAN_POINT('Ctrl Pts',(-0.185723055456903,0.0166573800151943,
-0.00349659872622789));
#26828=CARTESIAN_POINT('Ctrl Pts',(-0.232326704333039,0.0163854748419384,
-0.00344344619644609));
#26829=CARTESIAN_POINT('Ctrl Pts',(-0.185723055456904,0.0158049536659853,
-0.00552554202981291));
#26830=CARTESIAN_POINT('Ctrl Pts',(-0.23232670433304,0.0158790365063827,
-0.00570322401511438));
#26831=CARTESIAN_POINT('Ctrl Pts',(-0.185723055456903,0.0136025708308564,
-0.00796594412460981));
#26832=CARTESIAN_POINT('Ctrl Pts',(-0.232326704333039,0.0138912669883084,
-0.00858048214849728));
#26833=CARTESIAN_POINT('Ctrl Pts',(-0.185723055456904,0.0107282744647946,
-0.00954209114738551));
#26834=CARTESIAN_POINT('Ctrl Pts',(-0.23232670433304,0.0109544909042364,
-0.010506785011137));
#26835=CARTESIAN_POINT('Ctrl Pts',(-0.185723055456903,0.00749999999987153,
-0.0100866616277759));
#26836=CARTESIAN_POINT('Ctrl Pts',(-0.232326704333039,0.00749999999987138,
-0.0111842362468306));
#26837=CARTESIAN_POINT('Ctrl Pts',(-0.185723055456904,0.00427172553496278,
-0.00954209114730134));
#26838=CARTESIAN_POINT('Ctrl Pts',(-0.23232670433304,0.00404550909552549,
-0.0105067850110401));
#26839=CARTESIAN_POINT('Ctrl Pts',(-0.185723055456903,0.00139742916894219,
-0.0079659441244508));
#26840=CARTESIAN_POINT('Ctrl Pts',(-0.232326704333039,0.00110873301150744,
-0.00858048214831799));
#26841=CARTESIAN_POINT('Ctrl Pts',(-0.185723055456904,-0.000804953666122893,
-0.00552554202959671));
#26842=CARTESIAN_POINT('Ctrl Pts',(-0.23232670433304,-0.000879036506486045,
-0.00570322401487933));
#26843=CARTESIAN_POINT('Ctrl Pts',(-0.185723055456903,-0.00165738001527906,
-0.00349659872598971));
#26844=CARTESIAN_POINT('Ctrl Pts',(-0.232326704333039,-0.0013854748419783,
-0.00344344619619682));
#26845=CARTESIAN_POINT('Ctrl Pts',(-0.185723055456903,-0.00199173196817847,
-0.00205818681044279));
#26846=CARTESIAN_POINT('Ctrl Pts',(-0.232326704333039,-0.00143274318789395,
-0.00190716237992731));
#26847=CARTESIAN_POINT('Ctrl Pts',(-0.185723055456903,-0.00213483890587743,
-0.00126455176511326));
#26848=CARTESIAN_POINT('Ctrl Pts',(-0.232326704333039,-0.00145297464812447,
-0.001131169564997));
#26849=CARTESIAN_POINT('Ctrl Pts',(-0.185723055456904,-0.00221238525369828,
8.33588010327838E-14));
#26850=CARTESIAN_POINT('Ctrl Pts',(-0.232326704333039,-0.0014639376096495,
1.20148665217339E-13));
#26851=CARTESIAN_POINT('Ctrl Pts',(-0.185723055456903,-0.00213483890585875,
0.00126455176527974));
#26852=CARTESIAN_POINT('Ctrl Pts',(-0.232326704333039,-0.00145297464812182,
0.00113116956523674));
#26853=CARTESIAN_POINT('Ctrl Pts',(-0.185723055456903,-0.00199173196814768,
0.00205818681060856));
#26854=CARTESIAN_POINT('Ctrl Pts',(-0.232326704333039,-0.0014327431878896,
0.00190716238016579));
#26855=CARTESIAN_POINT('Ctrl Pts',(-0.185723055456903,-0.00165738001522438,
0.00349659872621544));
#26856=CARTESIAN_POINT('Ctrl Pts',(-0.232326704333039,-0.00138547484194287,
0.00344344619705013));
#26857=CARTESIAN_POINT('Ctrl Pts',(-0.185723055456904,-0.000804955358563482,
0.00552554230330677));
#26858=CARTESIAN_POINT('Ctrl Pts',(-0.232326704333039,-0.000879051981413446,
0.0057032265164018));
#26859=CARTESIAN_POINT('Ctrl Pts',(-0.185723055456903,0.00139743580946407,
0.00796594412565152));
#26860=CARTESIAN_POINT('Ctrl Pts',(-0.232326704333039,0.00110879372578601,
0.00858048215857438));
#26861=CARTESIAN_POINT('Ctrl Pts',(-0.185723055456904,0.00381545901438577,
0.00929189433866225));
#26862=CARTESIAN_POINT('Ctrl Pts',(-0.232326704333039,0.00357932000252583,
0.0102010114195229));
#26863=CARTESIAN_POINT('Ctrl Pts',(-0.185723055456904,0.0054123742536131,
0.00969325716154195));
#26864=CARTESIAN_POINT('Ctrl Pts',(-0.232326704333039,0.00527133148148726,
0.0106961423740653));
#26865=CARTESIAN_POINT('Ctrl Pts',(-0.185723055456904,0.00596900147723498,
0.00978267384703966));
#26866=CARTESIAN_POINT('Ctrl Pts',(-0.23232670433304,0.00586421401192308,
0.0108066948117815));
#26867=CARTESIAN_POINT('',(-0.225761332775488,0.0164871798990637,0.00232893089033033));
#26868=CARTESIAN_POINT('',(-0.220090794747946,0.0165472343306677,0.00234431717574848));
#26869=CARTESIAN_POINT('Ctrl Pts',(-0.225761208631098,0.0164884121318173,
0.00232907518148799));
#26870=CARTESIAN_POINT('Ctrl Pts',(-0.220090794747946,0.0165472343306677,
0.00234431717574846));
#26871=CARTESIAN_POINT('',(-0.229322271958198,0.00910280340307597,0.0107454877379686));
#26872=CARTESIAN_POINT('Ctrl Pts',(-0.225761332775488,0.0164871798990637,
0.00232893089033043));
#26873=CARTESIAN_POINT('Ctrl Pts',(-0.225868813295687,0.0164702811459343,
0.00256572214437089));
#26874=CARTESIAN_POINT('Ctrl Pts',(-0.226137029027792,0.0164201503719644,
0.00311230936225717));
#26875=CARTESIAN_POINT('Ctrl Pts',(-0.226622346737041,0.0162529713835771,
0.00396894829373893));
#26876=CARTESIAN_POINT('Ctrl Pts',(-0.227136114083267,0.0160270537581582,
0.00471718824932398));
#26877=CARTESIAN_POINT('Ctrl Pts',(-0.227548052020872,0.015830334783286,
0.00523800076883081));
#26878=CARTESIAN_POINT('Ctrl Pts',(-0.227904933514641,0.0156518603798053,
0.00565166468326421));
#26879=CARTESIAN_POINT('Ctrl Pts',(-0.22824506964293,0.0154746912800295,
0.00601507791742848));
#26880=CARTESIAN_POINT('Ctrl Pts',(-0.228618690523152,0.0152744254805032,
0.0063844617087714));
#26881=CARTESIAN_POINT('Ctrl Pts',(-0.228906681001303,0.0151174744578315,
0.00664687659885061));
#26882=CARTESIAN_POINT('Ctrl Pts',(-0.22916173971917,0.0149769237018957,
0.00686832718740545));
#26883=CARTESIAN_POINT('Ctrl Pts',(-0.229386887100392,0.014851110571812,
0.00705580393505498));
#26884=CARTESIAN_POINT('Ctrl Pts',(-0.229526845406411,0.0147725603957695,
0.00716898590139015));
#26885=CARTESIAN_POINT('Ctrl Pts',(-0.22985665337706,0.0145837017217628,
0.00742915055021459));
#26886=CARTESIAN_POINT('Ctrl Pts',(-0.230067756669372,0.0144588911103182,
0.00758975272001023));
#26887=CARTESIAN_POINT('Ctrl Pts',(-0.230390189204541,0.0142582866306812,
0.00783304005481369));
#26888=CARTESIAN_POINT('Ctrl Pts',(-0.230587131929265,0.0141279794172046,
0.00798292444616597));
#26889=CARTESIAN_POINT('Ctrl Pts',(-0.230774468781011,0.013996606095421,
0.0081276487410968));
#26890=CARTESIAN_POINT('Ctrl Pts',(-0.230911642843167,0.013896223101725,
0.0082349516180805));
#26891=CARTESIAN_POINT('Ctrl Pts',(-0.231125605978502,0.013724550906806,
0.00840987345810032));
#26892=CARTESIAN_POINT('Ctrl Pts',(-0.231269225646072,0.0135968959048821,
0.00853388774673025));
#26893=CARTESIAN_POINT('Ctrl Pts',(-0.231454214398683,0.0134066528799722,
0.00870979256612292));
#26894=CARTESIAN_POINT('Ctrl Pts',(-0.231576826440879,0.0132527642207034,
0.00884432583919974));
#26895=CARTESIAN_POINT('Ctrl Pts',(-0.231699073871839,0.0130506469508559,
0.00901193941612837));
#26896=CARTESIAN_POINT('Ctrl Pts',(-0.231797984546367,0.0127794807589124,
0.00922301260208771));
#26897=CARTESIAN_POINT('Ctrl Pts',(-0.231797546311281,0.0124463550028915,
0.0094545189472133));
#26898=CARTESIAN_POINT('Ctrl Pts',(-0.231726490190532,0.01220148485762,
0.00960823702894843));
#26899=CARTESIAN_POINT('Ctrl Pts',(-0.231639005765325,0.0119843290682612,
0.00973688624094698));
#26900=CARTESIAN_POINT('Ctrl Pts',(-0.231525310404822,0.0117655522917993,
0.00985805531704937));
#26901=CARTESIAN_POINT('Ctrl Pts',(-0.231352361903446,0.0114927855298606,
0.00999609538197112));
#26902=CARTESIAN_POINT('Ctrl Pts',(-0.231244347684152,0.0113413363936371,
0.0100671311393663));
#26903=CARTESIAN_POINT('Ctrl Pts',(-0.231090705799142,0.01113549569015,
0.0101590920502647));
#26904=CARTESIAN_POINT('Ctrl Pts',(-0.230929371790275,0.0109316039033615,
0.0102437095233981));
#26905=CARTESIAN_POINT('Ctrl Pts',(-0.230719165437917,0.0106780079360857,
0.0103396054112657));
#26906=CARTESIAN_POINT('Ctrl Pts',(-0.230586872078737,0.0105231155941536,
0.0103934674402264));
#26907=CARTESIAN_POINT('Ctrl Pts',(-0.230414186940932,0.0103232538972528,
0.0104589357413493));
#26908=CARTESIAN_POINT('Ctrl Pts',(-0.230240646794771,0.0101254517763829,
0.0105184710817764));
#26909=CARTESIAN_POINT('Ctrl Pts',(-0.230026409330978,0.00988432845845099,
0.0105835997465218));
#26910=CARTESIAN_POINT('Ctrl Pts',(-0.229891307016393,0.00973360123118308,
0.0106204354698397));
#26911=CARTESIAN_POINT('Ctrl Pts',(-0.229656258725846,0.00947215625752134,
0.0106797649091995));
#26912=CARTESIAN_POINT('Ctrl Pts',(-0.229463316297648,0.00925865240873361,
0.0107203065532235));
#26913=CARTESIAN_POINT('Ctrl Pts',(-0.229322271958198,0.00910280340307599,
0.0107454877379686));
#26914=CARTESIAN_POINT('',(-0.227992309462812,0.0108760464259574,0.0102016547220559));
#26915=CARTESIAN_POINT('Ctrl Pts',(-0.229322271958198,0.00910280340307614,
0.0107454877379685));
#26916=CARTESIAN_POINT('Ctrl Pts',(-0.229248387424237,0.0091946609993933,
0.0107271294535291));
#26917=CARTESIAN_POINT('Ctrl Pts',(-0.229178401182458,0.00928183676705995,
0.0107081499431178));
#26918=CARTESIAN_POINT('Ctrl Pts',(-0.229120612526884,0.00935384619153853,
0.0106916491124385));
#26919=CARTESIAN_POINT('Ctrl Pts',(-0.22906282387131,0.00942585561601711,
0.0106751482817593));
#26920=CARTESIAN_POINT('Ctrl Pts',(-0.229017225542958,0.00948276183981316,
0.0106614506270637));
#26921=CARTESIAN_POINT('Ctrl Pts',(-0.228958941436709,0.0095562875725616,
0.0106428514999607));
#26922=CARTESIAN_POINT('Ctrl Pts',(-0.22890065733046,0.00962981330531004,
0.0106242523728578));
#26923=CARTESIAN_POINT('Ctrl Pts',(-0.228829699057721,0.0097198395476934,
0.0106002306726335));
#26924=CARTESIAN_POINT('Ctrl Pts',(-0.228770345698383,0.00979561634266397,
0.0105788852380152));
#26925=CARTESIAN_POINT('Ctrl Pts',(-0.228710992339046,0.00987139313763453,
0.0105575398033969));
#26926=CARTESIAN_POINT('Ctrl Pts',(-0.228663232364102,0.00993305883396627,
0.0105393906476383));
#26927=CARTESIAN_POINT('Ctrl Pts',(-0.228604723386985,0.0100100300555052,
0.0105157085654625));
#26928=CARTESIAN_POINT('Ctrl Pts',(-0.228546214409868,0.0100870012770442,
0.0104920264832867));
#26929=CARTESIAN_POINT('Ctrl Pts',(-0.228476966528714,0.0101791433991985,
0.0104623540609925));
#26930=CARTESIAN_POINT('Ctrl Pts',(-0.228414681428224,0.0102636793539038,
0.0104336680888423));
#26931=CARTESIAN_POINT('Ctrl Pts',(-0.228352396327734,0.0103482153086091,
0.0104049821166921));
#26932=CARTESIAN_POINT('Ctrl Pts',(-0.228297067653945,0.0104252427149842,
0.0103775724399405));
#26933=CARTESIAN_POINT('Ctrl Pts',(-0.228243303529506,0.0105019585952468,
0.0103492083290063));
#26934=CARTESIAN_POINT('Ctrl Pts',(-0.228189539405068,0.0105786744755093,
0.010320844218072));
#26935=CARTESIAN_POINT('Ctrl Pts',(-0.228137342432302,0.0106550348405252,
0.0102914062848182));
#26936=CARTESIAN_POINT('Ctrl Pts',(-0.228090589690832,0.0107250747442135,
0.0102634474254206));
#26937=CARTESIAN_POINT('Ctrl Pts',(-0.228062139674782,0.010767695483049,
0.0102464338776888));
#26938=CARTESIAN_POINT('Ctrl Pts',(-0.228035704099044,0.0108079890120059,
0.0102300065388951));
#26939=CARTESIAN_POINT('Ctrl Pts',(-0.228009004449627,0.0108497764912555,
0.0102126270296333));
#26940=CARTESIAN_POINT('Ctrl Pts',(-0.228003457661064,0.0108584577405253,
0.0102090164779849));
#26941=CARTESIAN_POINT('Ctrl Pts',(-0.227997899475325,0.0108672032881771,
0.0102053643805637));
#26942=CARTESIAN_POINT('Ctrl Pts',(-0.227992309462812,0.0108760464259574,
0.0102016547220559));
#26943=CARTESIAN_POINT('',(-0.227099026780033,0.01283031103747,0.00908913013680211));
#26944=CARTESIAN_POINT('Ctrl Pts',(-0.227992309462812,0.0108760464259574,
0.0102016547220559));
#26945=CARTESIAN_POINT('Ctrl Pts',(-0.227980588960823,0.0108945884230957,
0.0101938783175534));
#26946=CARTESIAN_POINT('Ctrl Pts',(-0.227968728545374,0.0109135602167407,
0.0101858506076612));
#26947=CARTESIAN_POINT('Ctrl Pts',(-0.2279565399122,0.0109332710148409,
0.0101774292059006));
#26948=CARTESIAN_POINT('Ctrl Pts',(-0.227910555558433,0.0110076344237606,
0.0101456575780034));
#26949=CARTESIAN_POINT('Ctrl Pts',(-0.227859905396422,0.0110924550180682,
0.0101081303354586));
#26950=CARTESIAN_POINT('Ctrl Pts',(-0.227813773705057,0.0111738765644079,
0.0100706078890561));
#26951=CARTESIAN_POINT('Ctrl Pts',(-0.227767642013693,0.0112552981107476,
0.0100330854426535));
#26952=CARTESIAN_POINT('Ctrl Pts',(-0.22772602561273,0.0113333921774084,
0.00999571733012953));
#26953=CARTESIAN_POINT('Ctrl Pts',(-0.227687001624059,0.0114100817697299,
0.00995776504015784));
#26954=CARTESIAN_POINT('Ctrl Pts',(-0.227647977635389,0.0114867713620514,
0.00991981275018614));
#26955=CARTESIAN_POINT('Ctrl Pts',(-0.227611544765425,0.0115620802269626,
0.00988133589719655));
#26956=CARTESIAN_POINT('Ctrl Pts',(-0.227574056474285,0.0116436347516357,
0.00983810533270652));
#26957=CARTESIAN_POINT('Ctrl Pts',(-0.227536568183146,0.0117251892763089,
0.00979487476821649));
#26958=CARTESIAN_POINT('Ctrl Pts',(-0.227498029236973,0.0118128746272589,
0.009746664582936));
#26959=CARTESIAN_POINT('Ctrl Pts',(-0.227464164954346,0.011892589671401,
0.00970124895034862));
#26960=CARTESIAN_POINT('Ctrl Pts',(-0.22743030067172,0.011972304715543,
0.00965583331776124));
#26961=CARTESIAN_POINT('Ctrl Pts',(-0.227401105512413,0.0120442031594079,
0.00961347988661202));
#26962=CARTESIAN_POINT('Ctrl Pts',(-0.227370538112144,0.0121209395116034,
0.00956682009479379));
#26963=CARTESIAN_POINT('Ctrl Pts',(-0.22735525441201,0.0121593076877011,
0.00954349019888468));
#26964=CARTESIAN_POINT('Ctrl Pts',(-0.227339627918637,0.0121988754292555,
0.00951907014777004));
#26965=CARTESIAN_POINT('Ctrl Pts',(-0.22732271689685,0.0122424277923068,
0.00949166041574463));
#26966=CARTESIAN_POINT('Ctrl Pts',(-0.227305805875064,0.0122859801553581,
0.00946425068371923));
#26967=CARTESIAN_POINT('Ctrl Pts',(-0.22728761252851,0.0123334516519383,
0.00943374365708379));
#26968=CARTESIAN_POINT('Ctrl Pts',(-0.227274223818761,0.012368527112979,
0.00941086715995704));
#26969=CARTESIAN_POINT('Ctrl Pts',(-0.227260835109012,0.0124036025740196,
0.00938799066283029));
#26970=CARTESIAN_POINT('Ctrl Pts',(-0.227252247760813,0.0124263866191674,
0.0093729066453705));
#26971=CARTESIAN_POINT('Ctrl Pts',(-0.227240923007382,0.0124564194502758,
0.0093528274289096));
#26972=CARTESIAN_POINT('Ctrl Pts',(-0.227229598253951,0.0124864522813842,
0.00933274821244871));
#26973=CARTESIAN_POINT('Ctrl Pts',(-0.227215537924042,0.0125236732667803,
0.00930758274915165));
#26974=CARTESIAN_POINT('Ctrl Pts',(-0.227200625928614,0.0125631084337543,
0.00928040810478293));
#26975=CARTESIAN_POINT('Ctrl Pts',(-0.227170806521505,0.0126419666458571,
0.00922606716916939));
#26976=CARTESIAN_POINT('Ctrl Pts',(-0.227137578349285,0.0127297909946739,
0.00916385101444131));
#26977=CARTESIAN_POINT('Ctrl Pts',(-0.227099060731718,0.0128303257879558,
0.00908912033180144));
#26978=CARTESIAN_POINT('',(-0.226399047365308,0.0128166254267281,0.00908546818530889));
#26979=CARTESIAN_POINT('Ctrl Pts',(-0.226399047380228,0.0128166254123418,
0.00908546808718478));
#26980=CARTESIAN_POINT('Ctrl Pts',(-0.226419607262987,0.0128187734864099,
0.00908429865679579));
#26981=CARTESIAN_POINT('Ctrl Pts',(-0.226454462989748,0.0128222624767334,
0.0090824250041845));
#26982=CARTESIAN_POINT('Ctrl Pts',(-0.226486204320344,0.0128250799254038,
0.00908097889269143));
#26983=CARTESIAN_POINT('Ctrl Pts',(-0.226517945651834,0.0128278973741534,
0.00907953278115769));
#26984=CARTESIAN_POINT('Ctrl Pts',(-0.226546572566094,0.0128300440654503,
0.00907851527844382));
#26985=CARTESIAN_POINT('Ctrl Pts',(-0.226573531760671,0.0128318691198156,
0.00907770064679367));
#26986=CARTESIAN_POINT('Ctrl Pts',(-0.226600490955248,0.0128336941741809,
0.00907688601514353));
#26987=CARTESIAN_POINT('Ctrl Pts',(-0.226625782433074,0.0128351974819294,
0.00907627410476947));
#26988=CARTESIAN_POINT('Ctrl Pts',(-0.22665804610537,0.012836295679909,
0.00907609638164778));
#26989=CARTESIAN_POINT('Ctrl Pts',(-0.226690309777666,0.0128373938778886,
0.00907591865852609));
#26990=CARTESIAN_POINT('Ctrl Pts',(-0.226729545644137,0.0128380869755876,
0.00907617513777574));
#26991=CARTESIAN_POINT('Ctrl Pts',(-0.226748701683591,0.0128383575711274,
0.00907635033279388));
#26992=CARTESIAN_POINT('Ctrl Pts',(-0.226758279703318,0.0128384928688973,
0.00907643793030296));
#26993=CARTESIAN_POINT('Ctrl Pts',(-0.226762837766467,0.0128385225347441,
0.00907650519775901));
#26994=CARTESIAN_POINT('Ctrl Pts',(-0.226777364157568,0.0128384660142501,
0.0090768309442104));
#26995=CARTESIAN_POINT('Ctrl Pts',(-0.22679189054867,0.0128384094937561,
0.00907715669066179));
#26996=CARTESIAN_POINT('Ctrl Pts',(-0.226816385267581,0.0128382667923632,
0.0090777409235453));
#26997=CARTESIAN_POINT('Ctrl Pts',(-0.226836329931151,0.0128380537045685,
0.00907828807316758));
#26998=CARTESIAN_POINT('Ctrl Pts',(-0.226876219258291,0.012837627528979,
0.00907938237241213));
#26999=CARTESIAN_POINT('Ctrl Pts',(-0.226897908364983,0.0128369197715561,
0.00908032829070822));
#27000=CARTESIAN_POINT('Ctrl Pts',(-0.22692393469492,0.0128360815957886,
0.0090814550142499));
#27001=CARTESIAN_POINT('Ctrl Pts',(-0.226975767174773,0.0128344123351328,
0.00908369892937038));
#27002=CARTESIAN_POINT('Ctrl Pts',(-0.227044802088362,0.0128322258406691,
0.00908665997123993));
#27003=CARTESIAN_POINT('Ctrl Pts',(-0.227098361224566,0.0128303951409884,
0.009089055605006));
#27004=CARTESIAN_POINT('',(-0.226520627876972,0.0132597435786184,0.00874175742880956));
#27005=CARTESIAN_POINT('Origin',(-0.22782078097521,0.00719470725115772,
0.00186149853466998));
#27006=CARTESIAN_POINT('',(-0.225316581766883,0.0132616346613913,0.00871757524912672));
#27007=CARTESIAN_POINT('',(-0.225316581766768,0.0132616346615032,0.00871757524903155));
#27008=CARTESIAN_POINT('',(-0.225201030506077,0.0128404758197692,0.0090447303940509));
#27009=CARTESIAN_POINT('Ctrl Pts',(-0.225201032785958,0.0128403937127591,
0.00904461617914099));
#27010=CARTESIAN_POINT('Ctrl Pts',(-0.22520217034852,0.0128447365367898,
0.00904144666023971));
#27011=CARTESIAN_POINT('Ctrl Pts',(-0.225206434504416,0.0128611961113402,
0.0090295544399252));
#27012=CARTESIAN_POINT('Ctrl Pts',(-0.22521694138661,0.0129006228490507,
0.00900027455390401));
#27013=CARTESIAN_POINT('Ctrl Pts',(-0.225227448268805,0.0129400495867611,
0.00897099466788282));
#27014=CARTESIAN_POINT('Ctrl Pts',(-0.225244204353462,0.0130022087793867,
0.00892400624483967));
#27015=CARTESIAN_POINT('Ctrl Pts',(-0.225258275192642,0.0130535473699845,
0.00888414630624995));
#27016=CARTESIAN_POINT('Ctrl Pts',(-0.225286416871002,0.01315622455118,
0.00880442642907052));
#27017=CARTESIAN_POINT('Ctrl Pts',(-0.225303791572998,0.0132167305635967,
0.00875462170239737));
#27018=CARTESIAN_POINT('Ctrl Pts',(-0.225316581929261,0.0132616274666869,
0.00871756658863472));
#27019=CARTESIAN_POINT('',(-0.224881672895038,0.0128394796279708,0.00903918282123092));
#27020=CARTESIAN_POINT('Ctrl Pts',(-0.224881672895038,0.0128394796279708,
0.00903918282123092));
#27021=CARTESIAN_POINT('Ctrl Pts',(-0.224944627892334,0.0128441999448473,
0.00903717439391197));
#27022=CARTESIAN_POINT('Ctrl Pts',(-0.225017590937262,0.0128449489007721,
0.00903629354585952));
#27023=CARTESIAN_POINT('Ctrl Pts',(-0.225078012179456,0.0128448149334077,
0.00903805276342249));
#27024=CARTESIAN_POINT('Ctrl Pts',(-0.225141875911401,0.012844673333276,
0.00903991221209972));
#27025=CARTESIAN_POINT('Ctrl Pts',(-0.225191718539843,0.0128427372415438,
0.00904291489718588));
#27026=CARTESIAN_POINT('Ctrl Pts',(-0.225201030475969,0.012840475865135,
0.00904473036080076));
#27027=CARTESIAN_POINT('',(-0.224871009513959,0.0128386119989575,0.00903955781216604));
#27028=CARTESIAN_POINT('Ctrl Pts',(-0.224871010004322,0.0128386125214796,
0.00903955742812217));
#27029=CARTESIAN_POINT('Ctrl Pts',(-0.22487452792311,0.0128389089493161,
0.00903943484621595));
#27030=CARTESIAN_POINT('Ctrl Pts',(-0.224878082488328,0.0128391918532535,
0.00903931570475177));
#27031=CARTESIAN_POINT('Ctrl Pts',(-0.224881672895038,0.0128394796279708,
0.00903918282123092));
#27032=CARTESIAN_POINT('',(-0.225012478343874,0.0119747516700286,0.00960390763878028));
#27033=CARTESIAN_POINT('Ctrl Pts',(-0.225012478352987,0.0119747517006528,
0.00960390762144819));
#27034=CARTESIAN_POINT('Ctrl Pts',(-0.225008710410711,0.012026996045218,
0.00957394039744444));
#27035=CARTESIAN_POINT('Ctrl Pts',(-0.225003438296681,0.0121091891020792,
0.00952597246849311));
#27036=CARTESIAN_POINT('Ctrl Pts',(-0.224994337261927,0.0121985784692992,
0.00947118760888405));
#27037=CARTESIAN_POINT('Ctrl Pts',(-0.22498978674455,0.0122432731529092,
0.00944379517907952));
#27038=CARTESIAN_POINT('Ctrl Pts',(-0.224984279372702,0.0122897558812711,
0.00941468016211316));
#27039=CARTESIAN_POINT('Ctrl Pts',(-0.224979096609221,0.0123276290221422,
0.00939056260385441));
#27040=CARTESIAN_POINT('Ctrl Pts',(-0.22497391384574,0.0123655021630133,
0.00936644504559567));
#27041=CARTESIAN_POINT('Ctrl Pts',(-0.22496905423407,0.0123948120512672,
0.00934739710168434));
#27042=CARTESIAN_POINT('Ctrl Pts',(-0.224965124481069,0.0124175278812019,
0.00933253807523926));
#27043=CARTESIAN_POINT('Ctrl Pts',(-0.224963159604568,0.0124288857961693,
0.00932510856201672));
#27044=CARTESIAN_POINT('Ctrl Pts',(-0.224961426927155,0.0124386035824382,
0.00931873941704309));
#27045=CARTESIAN_POINT('Ctrl Pts',(-0.224958010632985,0.0124564837209923,
0.00930690636953302));
#27046=CARTESIAN_POINT('Ctrl Pts',(-0.224954594338815,0.0124743638595464,
0.00929507332202296));
#27047=CARTESIAN_POINT('Ctrl Pts',(-0.224949495350036,0.012500376081017,
0.00927773042191478));
#27048=CARTESIAN_POINT('Ctrl Pts',(-0.224944426555004,0.0125247400917709,
0.00926128172483698));
#27049=CARTESIAN_POINT('Ctrl Pts',(-0.224939357759971,0.0125491041025248,
0.00924483302775918));
#27050=CARTESIAN_POINT('Ctrl Pts',(-0.224934318807232,0.0125718321678423,
0.00922929625790112));
#27051=CARTESIAN_POINT('Ctrl Pts',(-0.224930551299764,0.0125885920455888,
0.00921776851748214));
#27052=CARTESIAN_POINT('Ctrl Pts',(-0.224926783792295,0.0126053519233354,
0.00920624077706316));
#27053=CARTESIAN_POINT('Ctrl Pts',(-0.224924287175663,0.0126161623503046,
0.0091987498488507));
#27054=CARTESIAN_POINT('Ctrl Pts',(-0.224920930364144,0.0126305427729762,
0.00918873779061256));
#27055=CARTESIAN_POINT('Ctrl Pts',(-0.224914216741104,0.0126593036183194,
0.00916871367413629));
#27056=CARTESIAN_POINT('Ctrl Pts',(-0.224904065469932,0.0127022359337238,
0.00913844733481451));
#27057=CARTESIAN_POINT('Ctrl Pts',(-0.22489519761297,0.0127391097573549,
0.00911196635423408));
#27058=CARTESIAN_POINT('Ctrl Pts',(-0.224886329756008,0.012775983580986,
0.00908548537365366));
#27059=CARTESIAN_POINT('Ctrl Pts',(-0.224878742772621,0.0128068919285356,
0.00906291918311226));
#27060=CARTESIAN_POINT('Ctrl Pts',(-0.224871008983143,0.0128385761256605,
0.00903951085797481));
#27061=CARTESIAN_POINT('',(-0.224873054781352,0.0104158620395419,0.0103054854710163));
#27062=CARTESIAN_POINT('Ctrl Pts',(-0.225012478343874,0.0119747516700286,
0.00960390763878028));
#27063=CARTESIAN_POINT('Ctrl Pts',(-0.224987330133709,0.01182206617983,
0.00969074071080671));
#27064=CARTESIAN_POINT('Ctrl Pts',(-0.224965351168803,0.0116608808019534,
0.0097767691902134));
#27065=CARTESIAN_POINT('Ctrl Pts',(-0.224946345313378,0.0114844605087868,
0.00986337078472748));
#27066=CARTESIAN_POINT('Ctrl Pts',(-0.224927339457954,0.0113080402156202,
0.00994997237924156));
#27067=CARTESIAN_POINT('Ctrl Pts',(-0.224911318282184,0.0111160804773605,
0.0100365919910695));
#27068=CARTESIAN_POINT('Ctrl Pts',(-0.224898835482878,0.0109277687496176,
0.0101137329254911));
#27069=CARTESIAN_POINT('Ctrl Pts',(-0.224896811901168,0.0108972416091349,
0.0101262382121786));
#27070=CARTESIAN_POINT('Ctrl Pts',(-0.224894880873611,0.0108668147692598,
0.0101385061520976));
#27071=CARTESIAN_POINT('Ctrl Pts',(-0.224893040837449,0.0108364759539614,
0.0101505475595201));
#27072=CARTESIAN_POINT('Ctrl Pts',(-0.224884447118257,0.0106947813152176,
0.0102067858423248));
#27073=CARTESIAN_POINT('Ctrl Pts',(-0.22487783816785,0.0105550780358821,
0.0102582455724961));
#27074=CARTESIAN_POINT('Ctrl Pts',(-0.224873054781352,0.0104158620395419,
0.0103054854710163));
#27075=CARTESIAN_POINT('',(-0.224989656143797,0.00749503048378924,0.010792595233899));
#27076=CARTESIAN_POINT('Ctrl Pts',(-0.224873054781352,0.0104158620395419,
0.0103054854710163));
#27077=CARTESIAN_POINT('Ctrl Pts',(-0.224866226582386,0.0102173021707029,
0.0103733294134915));
#27078=CARTESIAN_POINT('Ctrl Pts',(-0.224863118344788,0.0100198072651585,
0.0104327497771305));
#27079=CARTESIAN_POINT('Ctrl Pts',(-0.22486326697531,0.00981927358101678,
0.0104860316796021));
#27080=CARTESIAN_POINT('Ctrl Pts',(-0.224863404497809,0.00963372694671159,
0.0105353315152647));
#27081=CARTESIAN_POINT('Ctrl Pts',(-0.22486633844048,0.00944551647501257,
0.0105790610493068));
#27082=CARTESIAN_POINT('Ctrl Pts',(-0.224872215239344,0.00925595755421325,
0.0106168125946656));
#27083=CARTESIAN_POINT('Ctrl Pts',(-0.224875153638775,0.00916117809381357,
0.010635688367345));
#27084=CARTESIAN_POINT('Ctrl Pts',(-0.224878825962802,0.00906607960841182,
0.0106531498380664));
#27085=CARTESIAN_POINT('Ctrl Pts',(-0.224883681329671,0.00896377930534679,
0.0106701043545088));
#27086=CARTESIAN_POINT('Ctrl Pts',(-0.224888536696539,0.00886147900228176,
0.0106870588709513));
#27087=CARTESIAN_POINT('Ctrl Pts',(-0.224894584175122,0.00875190532334013,
0.0107031016457275));
#27088=CARTESIAN_POINT('Ctrl Pts',(-0.224899808725538,0.00866487696745784,
0.0107145869666058));
#27089=CARTESIAN_POINT('Ctrl Pts',(-0.224905033275954,0.00857784861157555,
0.0107260722874841));
#27090=CARTESIAN_POINT('Ctrl Pts',(-0.224909420529746,0.00851344741040241,
0.010733638861035));
#27091=CARTESIAN_POINT('Ctrl Pts',(-0.224915038388532,0.00843441925484294,
0.0107420341088461));
#27092=CARTESIAN_POINT('Ctrl Pts',(-0.224920656247317,0.00835539109928347,
0.0107504293566573));
#27093=CARTESIAN_POINT('Ctrl Pts',(-0.22492751354538,0.00826169799655761,
0.0107592614034678));
#27094=CARTESIAN_POINT('Ctrl Pts',(-0.224935089512573,0.00816264216894523,
0.0107667780599388));
#27095=CARTESIAN_POINT('Ctrl Pts',(-0.22495024144696,0.00796453051372045,
0.0107818113728808));
#27096=CARTESIAN_POINT('Ctrl Pts',(-0.224968252959357,0.0077449941022938,
0.0107922510362213));
#27097=CARTESIAN_POINT('Ctrl Pts',(-0.224989656143797,0.00749503048378924,
0.010792595233899));
#27098=CARTESIAN_POINT('',(-0.224876132721504,0.00588096715315318,0.010642983684972));
#27099=CARTESIAN_POINT('Ctrl Pts',(-0.224989611770161,0.00749451541494347,
0.0107925939286014));
#27100=CARTESIAN_POINT('Ctrl Pts',(-0.224967889525284,0.00724236729651667,
0.0107919481648337));
#27101=CARTESIAN_POINT('Ctrl Pts',(-0.224949602833122,0.00702085004378462,
0.0107810653131202));
#27102=CARTESIAN_POINT('Ctrl Pts',(-0.224934211963363,0.00682092613373424,
0.0107655246226512));
#27103=CARTESIAN_POINT('Ctrl Pts',(-0.224926511289036,0.00672089611947813,
0.0107577489869667));
#27104=CARTESIAN_POINT('Ctrl Pts',(-0.224919539392079,0.00662627872449041,
0.0107486376236482));
#27105=CARTESIAN_POINT('Ctrl Pts',(-0.224913825599119,0.00654643123053275,
0.0107399825657948));
#27106=CARTESIAN_POINT('Ctrl Pts',(-0.224908111806159,0.0064665837365751,
0.0107313275079415));
#27107=CARTESIAN_POINT('Ctrl Pts',(-0.224903647137783,0.00640146658868505,
0.0107235271217113));
#27108=CARTESIAN_POINT('Ctrl Pts',(-0.224898329718857,0.00631360222420139,
0.0107117163940124));
#27109=CARTESIAN_POINT('Ctrl Pts',(-0.224893012299931,0.00622573785971773,
0.0106999056663135));
#27110=CARTESIAN_POINT('Ctrl Pts',(-0.224886856690796,0.0061152112912604,
0.0106834372017356));
#27111=CARTESIAN_POINT('Ctrl Pts',(-0.224881918316017,0.00601190187579096,
0.0106660263533176));
#27112=CARTESIAN_POINT('Ctrl Pts',(-0.224879775998716,0.00596708519864215,
0.0106584733498581));
#27113=CARTESIAN_POINT('Ctrl Pts',(-0.224877861054523,0.00592361449883146,
0.0106508077009257));
#27114=CARTESIAN_POINT('Ctrl Pts',(-0.224876132721504,0.00588096715315318,
0.010642983684972));
#27115=CARTESIAN_POINT('',(-0.224076522719914,0.00588277614622394,0.010625353510046));
#27116=CARTESIAN_POINT('Ctrl Pts',(-0.224876132721504,0.00588096715315317,
0.010642983684972));
#27117=CARTESIAN_POINT('Ctrl Pts',(-0.224076521518844,0.00588276506383911,
0.0106254138449689));
#27118=CARTESIAN_POINT('',(-0.224190648122848,0.00749528770010443,0.0107745370286281));
#27119=CARTESIAN_POINT('Ctrl Pts',(-0.224076522719914,0.00588277614622425,
0.010625353510046));
#27120=CARTESIAN_POINT('Ctrl Pts',(-0.224077151983702,0.00589828271375071,
0.0106282142999538));
#27121=CARTESIAN_POINT('Ctrl Pts',(-0.224082955020581,0.00603662211173329,
0.0106533554983067));
#27122=CARTESIAN_POINT('Ctrl Pts',(-0.224093480360963,0.0062288683222389,
0.0106833518343927));
#27123=CARTESIAN_POINT('Ctrl Pts',(-0.224110291260917,0.00649044232002643,
0.0107167590851501));
#27124=CARTESIAN_POINT('Ctrl Pts',(-0.224127481546521,0.00672803320751328,
0.0107404347775083));
#27125=CARTESIAN_POINT('Ctrl Pts',(-0.224137535386306,0.00685693381374031,
0.0107505870267272));
#27126=CARTESIAN_POINT('Ctrl Pts',(-0.224157907843775,0.00711079347145578,
0.0107671148153925));
#27127=CARTESIAN_POINT('Ctrl Pts',(-0.224176389710925,0.0073296949891921,
0.0107741272895942));
#27128=CARTESIAN_POINT('Ctrl Pts',(-0.224190649380928,0.00749528605098617,
0.0107745371458377));
#27129=CARTESIAN_POINT('',(-0.224080534199978,0.0105762623394819,0.0102317974583992));
#27130=CARTESIAN_POINT('Ctrl Pts',(-0.224190649231643,0.00749528779516735,
0.010774537143386));
#27131=CARTESIAN_POINT('Ctrl Pts',(-0.224176496049103,0.00766064698633964,
0.0107743046922629));
#27132=CARTESIAN_POINT('Ctrl Pts',(-0.224158158806334,0.00787923373782332,
0.0107675433910972));
#27133=CARTESIAN_POINT('Ctrl Pts',(-0.224137967011069,0.00813268605449651,
0.0107513356813969));
#27134=CARTESIAN_POINT('Ctrl Pts',(-0.224128006599897,0.00826137903423121,
0.0107413516624803));
#27135=CARTESIAN_POINT('Ctrl Pts',(-0.224111011590131,0.00849848535023519,
0.0107180136087507));
#27136=CARTESIAN_POINT('Ctrl Pts',(-0.224094433786784,0.00875959453805924,
0.0106850105184737));
#27137=CARTESIAN_POINT('Ctrl Pts',(-0.224072162870967,0.00917370885433421,
0.0106208996991876));
#27138=CARTESIAN_POINT('Ctrl Pts',(-0.224058304186119,0.00982143528436496,
0.0104791570008723));
#27139=CARTESIAN_POINT('Ctrl Pts',(-0.224068970775361,0.0103174374881225,
0.0103260156650735));
#27140=CARTESIAN_POINT('Ctrl Pts',(-0.224080534199978,0.0105762623394819,
0.0102317974583992));
#27141=CARTESIAN_POINT('',(-0.224520408689827,0.0132627824003338,0.00870166862344196));
#27142=CARTESIAN_POINT('Ctrl Pts',(-0.224080566034144,0.0105769745611062,
0.0102315381587443));
#27143=CARTESIAN_POINT('Ctrl Pts',(-0.224092151509287,0.0108360569066869,
0.0101372010598917));
#27144=CARTESIAN_POINT('Ctrl Pts',(-0.224118896843735,0.0112411393783209,
0.00996911208968928));
#27145=CARTESIAN_POINT('Ctrl Pts',(-0.224170735895982,0.0116930385087458,
0.0097434105075323));
#27146=CARTESIAN_POINT('Ctrl Pts',(-0.224215922342647,0.0119969042554561,
0.00957749590305291));
#27147=CARTESIAN_POINT('Ctrl Pts',(-0.224266689003916,0.0122607174895522,
0.00941974624796191));
#27148=CARTESIAN_POINT('Ctrl Pts',(-0.224313605564443,0.01247477238858,
0.00928306617490918));
#27149=CARTESIAN_POINT('Ctrl Pts',(-0.224360095211767,0.012667384538008,
0.00915273873550236));
#27150=CARTESIAN_POINT('Ctrl Pts',(-0.224383610132216,0.0127587835173505,
0.00908822365193216));
#27151=CARTESIAN_POINT('Ctrl Pts',(-0.224435627652213,0.0129574442013583,
0.00894448849032735));
#27152=CARTESIAN_POINT('Ctrl Pts',(-0.224483462100191,0.013131275288331,
0.00881005173864322));
#27153=CARTESIAN_POINT('Ctrl Pts',(-0.224520870146751,0.0132627197125121,
0.00870173325440467));
#27154=CARTESIAN_POINT('',(-0.22331682546513,0.0132649854369558,0.00867730801686743));
#27155=CARTESIAN_POINT('',(-0.223316825297034,0.0132649928747286,0.00867731700379056));
#27156=CARTESIAN_POINT('',(-0.222880616837559,0.010577337791327,0.0102052819769689));
#27157=CARTESIAN_POINT('Ctrl Pts',(-0.22331682546513,0.0132649854369558,
0.00867730801686743));
#27158=CARTESIAN_POINT('Ctrl Pts',(-0.223279798803615,0.0131348061383841,
0.00878434512588197));
#27159=CARTESIAN_POINT('Ctrl Pts',(-0.223232266045539,0.0129617921433397,
0.00891797582610665));
#27160=CARTESIAN_POINT('Ctrl Pts',(-0.223180368331416,0.0127626377797213,
0.0090618860882604));
#27161=CARTESIAN_POINT('Ctrl Pts',(-0.223156255037636,0.0126681475127752,
0.00912843001754567));
#27162=CARTESIAN_POINT('Ctrl Pts',(-0.223110670361712,0.0124772678792337,
0.00925731159444108));
#27163=CARTESIAN_POINT('Ctrl Pts',(-0.223064300581422,0.0122631114605902,
0.00939386631131441));
#27164=CARTESIAN_POINT('Ctrl Pts',(-0.22301407297073,0.0119976000119375,
0.0095523407640007));
#27165=CARTESIAN_POINT('Ctrl Pts',(-0.222969614485712,0.0116931713173529,
0.0097182094358203));
#27166=CARTESIAN_POINT('Ctrl Pts',(-0.222918481738802,0.0112405948889791,
0.00994374743151154));
#27167=CARTESIAN_POINT('Ctrl Pts',(-0.222892075429266,0.0108362091582251,
0.0101112031578736));
#27168=CARTESIAN_POINT('Ctrl Pts',(-0.222880616837559,0.010577337791327,
0.0102052819769689));
#27169=CARTESIAN_POINT('',(-0.222990244465972,0.0074958307571125,0.0107474072527987));
#27170=CARTESIAN_POINT('Ctrl Pts',(-0.222880616837559,0.010577337791327,
0.0102052819769689));
#27171=CARTESIAN_POINT('Ctrl Pts',(-0.222869158245852,0.010318466424429,
0.0102993607960641));
#27172=CARTESIAN_POINT('Ctrl Pts',(-0.222858532291739,0.0098221619311753,
0.0104524017706292));
#27173=CARTESIAN_POINT('Ctrl Pts',(-0.22287221561341,0.00917417190932849,
0.01059395889742));
#27174=CARTESIAN_POINT('Ctrl Pts',(-0.22289427636194,0.00876014094051484,
0.010657968090584));
#27175=CARTESIAN_POINT('Ctrl Pts',(-0.222910764672285,0.00849894378348925,
0.010690932418882));
#27176=CARTESIAN_POINT('Ctrl Pts',(-0.222927658039428,0.00826210241293319,
0.0107142206595775));
#27177=CARTESIAN_POINT('Ctrl Pts',(-0.222937661815565,0.00813238625044321,
0.0107242728838261));
#27178=CARTESIAN_POINT('Ctrl Pts',(-0.222957828125963,0.00787876829528368,
0.0107404453241587));
#27179=CARTESIAN_POINT('Ctrl Pts',(-0.222976130338379,0.00766059007085584,
0.0107471651883034));
#27180=CARTESIAN_POINT('Ctrl Pts',(-0.222990244465972,0.0074958307571125,
0.0107474072527987));
#27181=CARTESIAN_POINT('',(-0.222876594854072,0.00588547347265839,0.0105989910637735));
#27182=CARTESIAN_POINT('Ctrl Pts',(-0.222990239545162,0.00749577366117287,
0.0107474071147549));
#27183=CARTESIAN_POINT('Ctrl Pts',(-0.22297603597005,0.00733096986388736,
0.0107470081671261));
#27184=CARTESIAN_POINT('Ctrl Pts',(-0.222957600580606,0.00711260011738536,
0.0107400754574236));
#27185=CARTESIAN_POINT('Ctrl Pts',(-0.222937252471541,0.00685858184257114,
0.0107236246276555));
#27186=CARTESIAN_POINT('Ctrl Pts',(-0.22292712606046,0.00672831097961292,
0.0107133900195418));
#27187=CARTESIAN_POINT('Ctrl Pts',(-0.222910059900934,0.00649137236979646,
0.010689833478941));
#27188=CARTESIAN_POINT('Ctrl Pts',(-0.22289333691819,0.00622976706583754,
0.0106565195733224));
#27189=CARTESIAN_POINT('Ctrl Pts',(-0.222882927058416,0.00603800133094661,
0.0106266668100976));
#27190=CARTESIAN_POINT('Ctrl Pts',(-0.222877192716254,0.00590029280163884,
0.0106017151325738));
#27191=CARTESIAN_POINT('Ctrl Pts',(-0.222876594854072,0.00588547347265862,
0.0105989910637735));
#27192=CARTESIAN_POINT('',(-0.222077231673906,0.00588727068028757,0.0105814273450435));
#27193=CARTESIAN_POINT('Ctrl Pts',(-0.222876593582855,0.00588546307913867,
0.0105990478538717));
#27194=CARTESIAN_POINT('Ctrl Pts',(-0.22207723054939,0.00588726043182086,
0.0105814834668851));
#27195=CARTESIAN_POINT('',(-0.222191219837884,0.00749641675969908,0.0107293488757352));
#27196=CARTESIAN_POINT('Ctrl Pts',(-0.222077231673906,0.00588727068028781,
0.0105814273450436));
#27197=CARTESIAN_POINT('Ctrl Pts',(-0.222077817443984,0.00590163889072924,
0.010584062875708));
#27198=CARTESIAN_POINT('Ctrl Pts',(-0.222083585840763,0.00603885906659558,
0.0106088832961562));
#27199=CARTESIAN_POINT('Ctrl Pts',(-0.22209405093591,0.00622999833890161,
0.010638590169762));
#27200=CARTESIAN_POINT('Ctrl Pts',(-0.222110861395534,0.00649158239727542,
0.0106718672026456));
#27201=CARTESIAN_POINT('Ctrl Pts',(-0.22212805244651,0.00672918335429661,
0.0106954431976079));
#27202=CARTESIAN_POINT('Ctrl Pts',(-0.22213810188887,0.00685802378461892,
0.0107055446600767));
#27203=CARTESIAN_POINT('Ctrl Pts',(-0.222158473656955,0.0071118708222244,
0.0107219929296602));
#27204=CARTESIAN_POINT('Ctrl Pts',(-0.222176957436455,0.00733079304772627,
0.0107289601534279));
#27205=CARTESIAN_POINT('Ctrl Pts',(-0.222191219837884,0.00749641675969908,
0.0107293488757352));
#27206=CARTESIAN_POINT('',(-0.222081197665177,0.0105780449623156,0.0101876296223523));
#27207=CARTESIAN_POINT('Ctrl Pts',(-0.222191219671532,0.00749641870290202,
0.0107293488727541));
#27208=CARTESIAN_POINT('Ctrl Pts',(-0.222177058733032,0.00766183514344189,
0.0107290950868428));
#27209=CARTESIAN_POINT('Ctrl Pts',(-0.222158713562285,0.00788046962613566,
0.0107223213320887));
#27210=CARTESIAN_POINT('Ctrl Pts',(-0.22213851683349,0.00813393428353906,
0.0107061245783974));
#27211=CARTESIAN_POINT('Ctrl Pts',(-0.222128559102259,0.00826256686459831,
0.0106961574222194));
#27212=CARTESIAN_POINT('Ctrl Pts',(-0.222111558904582,0.00849971984722734,
0.0106728517706667));
#27213=CARTESIAN_POINT('Ctrl Pts',(-0.222094980050245,0.00876085477560986,
0.0106399064973814));
#27214=CARTESIAN_POINT('Ctrl Pts',(-0.222072711961566,0.00917502974014479,
0.0105759159488009));
#27215=CARTESIAN_POINT('Ctrl Pts',(-0.222058878162029,0.00982287571753665,
0.0104344849162957));
#27216=CARTESIAN_POINT('Ctrl Pts',(-0.222069605421447,0.0103192093797939,
0.0102815997590037));
#27217=CARTESIAN_POINT('Ctrl Pts',(-0.222081197665177,0.0105780449623156,
0.0101876296223523));
#27218=CARTESIAN_POINT('',(-0.222521351578035,0.0132670948112432,0.00866068980045947));
#27219=CARTESIAN_POINT('Ctrl Pts',(-0.222081228766005,0.0105787390845834,
0.0101873775888729));
#27220=CARTESIAN_POINT('Ctrl Pts',(-0.222092842521717,0.0108378253339584,
0.0100932920251452));
#27221=CARTESIAN_POINT('Ctrl Pts',(-0.222119627444957,0.011242674877814,
0.00992576375075805));
#27222=CARTESIAN_POINT('Ctrl Pts',(-0.222171526065299,0.0116950336032214,
0.00970054580926344));
#27223=CARTESIAN_POINT('Ctrl Pts',(-0.222216807058984,0.0119996304538849,
0.00953473789079934));
#27224=CARTESIAN_POINT('Ctrl Pts',(-0.222267519311081,0.0122635513148824,
0.00937741358971341));
#27225=CARTESIAN_POINT('Ctrl Pts',(-0.22231438826496,0.0124778714741315,
0.00924100644392873));
#27226=CARTESIAN_POINT('Ctrl Pts',(-0.222360817077006,0.012670745258053,
0.00911092961363663));
#27227=CARTESIAN_POINT('Ctrl Pts',(-0.222384295531511,0.0127622736095719,
0.0090465381747067));
#27228=CARTESIAN_POINT('Ctrl Pts',(-0.222436236646195,0.0129612471208603,
0.00890306004810599));
#27229=CARTESIAN_POINT('Ctrl Pts',(-0.222483998152326,0.0131353820046699,
0.00876885123967379));
#27230=CARTESIAN_POINT('Ctrl Pts',(-0.222521353943371,0.0132670959637705,
0.00866069202955122));
#27231=CARTESIAN_POINT('',(-0.22131750689037,0.0132679777242635,0.00863749771222783));
#27232=CARTESIAN_POINT('',(-0.221317506737634,0.013267984478113,0.00863750590557259));
#27233=CARTESIAN_POINT('',(-0.22088115156098,0.0105783645468105,0.010161402673548));
#27234=CARTESIAN_POINT('Ctrl Pts',(-0.22131750689037,0.0132679777242635,
0.00863749771222783));
#27235=CARTESIAN_POINT('Ctrl Pts',(-0.221280596683195,0.0131376209513906,
0.00874425583075433));
#27236=CARTESIAN_POINT('Ctrl Pts',(-0.221233204347556,0.0129643814873638,
0.008877547080368));
#27237=CARTESIAN_POINT('Ctrl Pts',(-0.221181438272831,0.0127649663026909,
0.00902110773845264));
#27238=CARTESIAN_POINT('Ctrl Pts',(-0.221157370058087,0.0126703006863166,
0.00908752698191699));
#27239=CARTESIAN_POINT('Ctrl Pts',(-0.221111880231701,0.0124792324471473,
0.00921606458370327));
#27240=CARTESIAN_POINT('Ctrl Pts',(-0.221065554909024,0.0122648142583938,
0.00935229104230504));
#27241=CARTESIAN_POINT('Ctrl Pts',(-0.221015368911087,0.011999454456574,
0.0095101388491494));
#27242=CARTESIAN_POINT('Ctrl Pts',(-0.220970544862955,0.0116933253634984,
0.00967635688216004));
#27243=CARTESIAN_POINT('Ctrl Pts',(-0.220919169872804,0.0112401297049436,
0.00990131927234546));
#27244=CARTESIAN_POINT('Ctrl Pts',(-0.220892657893147,0.0108367113854765,
0.0100677899435825));
#27245=CARTESIAN_POINT('Ctrl Pts',(-0.22088115156098,0.0105783645468105,
0.010161402673548));
#27246=CARTESIAN_POINT('',(-0.220990767119986,0.00749707322251576,0.010702217868989));
#27247=CARTESIAN_POINT('Ctrl Pts',(-0.22088115156098,0.0105783645468105,
0.010161402673548));
#27248=CARTESIAN_POINT('Ctrl Pts',(-0.220869645228813,0.0103200177081445,
0.0102550154035136));
#27249=CARTESIAN_POINT('Ctrl Pts',(-0.220858969206354,0.00982452144610325,
0.0104075054283932));
#27250=CARTESIAN_POINT('Ctrl Pts',(-0.220872745540538,0.00917495312743478,
0.0105490903500837));
#27251=CARTESIAN_POINT('Ctrl Pts',(-0.220894819848736,0.00876114659657297,
0.010612900546867));
#27252=CARTESIAN_POINT('Ctrl Pts',(-0.220911311157844,0.00849998081158383,
0.0106457941366486));
#27253=CARTESIAN_POINT('Ctrl Pts',(-0.220928202324832,0.00826319748824002,
0.0106690348315061));
#27254=CARTESIAN_POINT('Ctrl Pts',(-0.220938201788269,0.00813353165458825,
0.0106790696234058));
#27255=CARTESIAN_POINT('Ctrl Pts',(-0.22095836166011,0.00787996925633426,
0.0106952234487667));
#27256=CARTESIAN_POINT('Ctrl Pts',(-0.220976657670658,0.00766182000071475,
0.0107019528152277));
#27257=CARTESIAN_POINT('Ctrl Pts',(-0.220990767119986,0.00749707322251576,
0.010702217868989));
#27258=CARTESIAN_POINT('',(-0.220877304433504,0.00588996792097283,0.0105550654063144));
#27259=CARTESIAN_POINT('Ctrl Pts',(-0.220990762709943,0.00749702203711106,
0.0107022177524562));
#27260=CARTESIAN_POINT('Ctrl Pts',(-0.220976559819124,0.00733217508802056,
0.0107018420080365));
#27261=CARTESIAN_POINT('Ctrl Pts',(-0.22095812756767,0.00711377483183485,
0.0106949566930038));
#27262=CARTESIAN_POINT('Ctrl Pts',(-0.220937786972359,0.00685976194883156,
0.0106785878913699));
#27263=CARTESIAN_POINT('Ctrl Pts',(-0.220927669297289,0.00672955702063277,
0.0106684068115));
#27264=CARTESIAN_POINT('Ctrl Pts',(-0.220910609290499,0.00649259338853425,
0.0106449511936309));
#27265=CARTESIAN_POINT('Ctrl Pts',(-0.220893896329436,0.00623097711339245,
0.0106117714895317));
#27266=CARTESIAN_POINT('Ctrl Pts',(-0.220883552434346,0.0060402582927849,
0.0105821976385212));
#27267=CARTESIAN_POINT('Ctrl Pts',(-0.220877859202795,0.00590367268940595,
0.0105575697530104));
#27268=CARTESIAN_POINT('Ctrl Pts',(-0.220877304433504,0.005889967920973,
0.0105550654063144));
#27269=CARTESIAN_POINT('',(-0.220077799936617,0.00589176565002758,0.0105374974776579));
#27270=CARTESIAN_POINT('Ctrl Pts',(-0.220877303267762,0.00588995844564909,
0.0105551174901662));
#27271=CARTESIAN_POINT('Ctrl Pts',(-0.220077798878423,0.0058917561161673,
0.0105375499971699));
#27272=CARTESIAN_POINT('',(-0.220191750495462,0.00749752817580766,0.0106841595550818));
#27273=CARTESIAN_POINT('Ctrl Pts',(-0.220077799936617,0.00589176565002776,
0.0105374974776579));
#27274=CARTESIAN_POINT('Ctrl Pts',(-0.220078351608142,0.00590522124109448,
0.0105399511847801));
#27275=CARTESIAN_POINT('Ctrl Pts',(-0.220084100627504,0.00604148651957028,
0.0105644754757549));
#27276=CARTESIAN_POINT('Ctrl Pts',(-0.220094528895997,0.00623167523773941,
0.010593906086857));
#27277=CARTESIAN_POINT('Ctrl Pts',(-0.220111351815037,0.00649315070770517,
0.0106270223766921));
#27278=CARTESIAN_POINT('Ctrl Pts',(-0.220128554181359,0.00673065566572463,
0.0106504779393937));
#27279=CARTESIAN_POINT('Ctrl Pts',(-0.220138604498337,0.00685937820658921,
0.0106605198785713));
#27280=CARTESIAN_POINT('Ctrl Pts',(-0.220158985618377,0.00711309953252186,
0.0106768746775319));
#27281=CARTESIAN_POINT('Ctrl Pts',(-0.220177479403337,0.00733194518244467,
0.0106837913787835));
#27282=CARTESIAN_POINT('Ctrl Pts',(-0.220191750495462,0.00749752817580766,
0.0106841595550818));
#27283=CARTESIAN_POINT('',(-0.220080922141363,0.0105666342787044,0.0101482127006066));
#27284=CARTESIAN_POINT('Ctrl Pts',(-0.220191750367871,0.00749752966457758,
0.0106841595526083));
#27285=CARTESIAN_POINT('Ctrl Pts',(-0.220177627116492,0.00766232360287522,
0.0106838857496589));
#27286=CARTESIAN_POINT('Ctrl Pts',(-0.22015933208859,0.00788007512162449,
0.0106771540698828));
#27287=CARTESIAN_POINT('Ctrl Pts',(-0.220139190917174,0.00813238879895161,
0.0106611110916827));
#27288=CARTESIAN_POINT('Ctrl Pts',(-0.220129266225352,0.00826033660350853,
0.0106512514860819));
#27289=CARTESIAN_POINT('Ctrl Pts',(-0.220112302357682,0.00849632083744043,
0.0106282022977969));
#27290=CARTESIAN_POINT('Ctrl Pts',(-0.220095725865799,0.00875628513266106,
0.010595617319954));
#27291=CARTESIAN_POINT('Ctrl Pts',(-0.220073367500684,0.00916890990113659,
0.0105322979819828));
#27292=CARTESIAN_POINT('Ctrl Pts',(-0.220059171892308,0.00981497694871467,
0.0103921745952535));
#27293=CARTESIAN_POINT('Ctrl Pts',(-0.220069554539533,0.010308881910491,
0.0102410928523781));
#27294=CARTESIAN_POINT('Ctrl Pts',(-0.220080922141363,0.0105666342787044,
0.0101482127006066));
#27295=CARTESIAN_POINT('',(-0.220516756733524,0.0132502006776825,0.00863716366641789));
#27296=CARTESIAN_POINT('Ctrl Pts',(-0.220080948889328,0.0105672405317447,
0.0101479942146856));
#27297=CARTESIAN_POINT('Ctrl Pts',(-0.220092335098988,0.0108252120871597,
0.0100550139845299));
#27298=CARTESIAN_POINT('Ctrl Pts',(-0.220118697300213,0.0112285596160589,
0.00988944046538119));
#27299=CARTESIAN_POINT('Ctrl Pts',(-0.220169906485688,0.0116799609641777,
0.00966654457709283));
#27300=CARTESIAN_POINT('Ctrl Pts',(-0.220214571302728,0.0119840360542289,
0.00950241318882273));
#27301=CARTESIAN_POINT('Ctrl Pts',(-0.220264797648843,0.0122482886171999,
0.00934622564793901));
#27302=CARTESIAN_POINT('Ctrl Pts',(-0.220311203197558,0.0124622454996215,
0.00921119607442466));
#27303=CARTESIAN_POINT('Ctrl Pts',(-0.220356992400339,0.0126538793364392,
0.0090831156431634));
#27304=CARTESIAN_POINT('Ctrl Pts',(-0.220380703772808,0.012746902376668,
0.00901827556250336));
#27305=CARTESIAN_POINT('Ctrl Pts',(-0.220432380283764,0.0129458253658021,
0.00887609019326517));
#27306=CARTESIAN_POINT('Ctrl Pts',(-0.220479785242708,0.0131192947887207,
0.00874360326452844));
#27307=CARTESIAN_POINT('Ctrl Pts',(-0.22051677874237,0.013250196930254,
0.0086371671501659));
#27308=CARTESIAN_POINT('',(-0.219244233672426,0.0130315029362845,0.00878633472257528));
#27309=CARTESIAN_POINT('Ctrl Pts',(-0.220516438237267,0.0132502507262974,
0.00863711659192548));
#27310=CARTESIAN_POINT('Ctrl Pts',(-0.220480268319726,0.013255974430882,
0.00863175603814082));
#27311=CARTESIAN_POINT('Ctrl Pts',(-0.220444069983548,0.0132619562961405,
0.00862616257509982));
#27312=CARTESIAN_POINT('Ctrl Pts',(-0.220413824310793,0.0132667445129213,
0.0086216573058079));
#27313=CARTESIAN_POINT('Ctrl Pts',(-0.220383483725874,0.0132715477553231,
0.00861713789879583));
#27314=CARTESIAN_POINT('Ctrl Pts',(-0.220367610104368,0.0132739986326908,
0.00861482180772873));
#27315=CARTESIAN_POINT('Ctrl Pts',(-0.220344973659625,0.0132771549469773,
0.00861179794256445));
#27316=CARTESIAN_POINT('Ctrl Pts',(-0.220322337214882,0.0132803112612638,
0.00860877407740017));
#27317=CARTESIAN_POINT('Ctrl Pts',(-0.220292924362422,0.0132839471365864,
0.0086052268546576));
#27318=CARTESIAN_POINT('Ctrl Pts',(-0.220265102204071,0.0132865904342554,
0.0086025299413693));
#27319=CARTESIAN_POINT('Ctrl Pts',(-0.220237280045721,0.0132892337319244,
0.00859983302808099));
#27320=CARTESIAN_POINT('Ctrl Pts',(-0.220211364377883,0.0132908098461735,
0.00859805395339447));
#27321=CARTESIAN_POINT('Ctrl Pts',(-0.220185552309859,0.0132914489697062,
0.00859705519961988));
#27322=CARTESIAN_POINT('Ctrl Pts',(-0.220133928173812,0.0132927272167718,
0.0085950576920707));
#27323=CARTESIAN_POINT('Ctrl Pts',(-0.220082288209308,0.013290467608556,
0.00859600043319445));
#27324=CARTESIAN_POINT('Ctrl Pts',(-0.220025068662385,0.0132840223930742,
0.00860026211803082));
#27325=CARTESIAN_POINT('Ctrl Pts',(-0.219967849115462,0.0132775771775925,
0.0086045238028672));
#27326=CARTESIAN_POINT('Ctrl Pts',(-0.219911157066727,0.0132674150573731,
0.00861182319958806));
#27327=CARTESIAN_POINT('Ctrl Pts',(-0.219858169150949,0.0132553285520544,
0.00862069118620989));
#27328=CARTESIAN_POINT('Ctrl Pts',(-0.219805181235171,0.0132432420467357,
0.00862955917283173));
#27329=CARTESIAN_POINT('Ctrl Pts',(-0.219755810159764,0.0132294672326508,
0.00863980980627492));
#27330=CARTESIAN_POINT('Ctrl Pts',(-0.219703713004701,0.0132129558824833,
0.00865213539350521));
#27331=CARTESIAN_POINT('Ctrl Pts',(-0.219651615849639,0.0131964445323158,
0.00866446098073551));
#27332=CARTESIAN_POINT('Ctrl Pts',(-0.219596945811511,0.0131768246090758,
0.0086791425006151));
#27333=CARTESIAN_POINT('Ctrl Pts',(-0.219551385430325,0.0131593781368699,
0.00869216144093205));
#27334=CARTESIAN_POINT('Ctrl Pts',(-0.219505825049139,0.0131419316646639,
0.008705180381249));
#27335=CARTESIAN_POINT('Ctrl Pts',(-0.219469184677475,0.0131270680608145,
0.00871625684184567));
#27336=CARTESIAN_POINT('Ctrl Pts',(-0.21941888662179,0.0131060788644454,
0.00873177776888143));
#27337=CARTESIAN_POINT('Ctrl Pts',(-0.21936858951329,0.0130850900633333,
0.00874729840363565));
#27338=CARTESIAN_POINT('Ctrl Pts',(-0.219313998061988,0.0130616867100786,
0.00876453744485508));
#27339=CARTESIAN_POINT('Ctrl Pts',(-0.21924423382129,0.0130315026592322,
0.00878633481537574));
#27340=CARTESIAN_POINT('',(-0.218875465344166,0.0104240813886614,0.0101716525593504));
#27341=CARTESIAN_POINT('Ctrl Pts',(-0.219244229875535,0.01303150113094,
0.00878633627788661));
#27342=CARTESIAN_POINT('Ctrl Pts',(-0.219212468167501,0.0129041535974503,
0.00888326996627987));
#27343=CARTESIAN_POINT('Ctrl Pts',(-0.219171618151564,0.0127349113020677,
0.00900461726313376));
#27344=CARTESIAN_POINT('Ctrl Pts',(-0.219126905471443,0.0125395266838569,
0.00913592699872258));
#27345=CARTESIAN_POINT('Ctrl Pts',(-0.219105910134124,0.0124456963448853,
0.00919740664822915));
#27346=CARTESIAN_POINT('Ctrl Pts',(-0.21906680529408,0.0122586484724146,
0.00931499746594284));
#27347=CARTESIAN_POINT('Ctrl Pts',(-0.219027129640222,0.0120491216573116,
0.00943952759860135));
#27348=CARTESIAN_POINT('Ctrl Pts',(-0.218984562930208,0.0117904939538435,
0.00958354134450399));
#27349=CARTESIAN_POINT('Ctrl Pts',(-0.218947335080204,0.0114953276327174,
0.00973376831601864));
#27350=CARTESIAN_POINT('Ctrl Pts',(-0.218905067925516,0.011059173820964,
0.00993691740974779));
#27351=CARTESIAN_POINT('Ctrl Pts',(-0.218884139782213,0.010673657181293,
0.0100865682928677));
#27352=CARTESIAN_POINT('Ctrl Pts',(-0.218875511383952,0.0104254101427982,
0.0101711999131546));
#27353=CARTESIAN_POINT('Ctrl Pts',(-0.218875465344166,0.0104240813886614,
0.0101716525593504));
#27354=CARTESIAN_POINT('',(-0.218991322981713,0.00749805982928716,0.0106570290092488));
#27355=CARTESIAN_POINT('Ctrl Pts',(-0.218875465344166,0.0104240813886614,
0.0101716525593504));
#27356=CARTESIAN_POINT('Ctrl Pts',(-0.218866957649238,0.0101785408296986,
0.0102552970778239));
#27357=CARTESIAN_POINT('Ctrl Pts',(-0.218860390040912,0.00970408442057063,
0.010393046425217));
#27358=CARTESIAN_POINT('Ctrl Pts',(-0.21887667134308,0.00908642942615499,
0.0105199428177679));
#27359=CARTESIAN_POINT('Ctrl Pts',(-0.218898757952546,0.00869434427410445,
0.0105770294824024));
#27360=CARTESIAN_POINT('Ctrl Pts',(-0.218914911213311,0.00844740082145461,
0.0106064119739009));
#27361=CARTESIAN_POINT('Ctrl Pts',(-0.218931211986323,0.00822432582340474,
0.0106271363044335));
#27362=CARTESIAN_POINT('Ctrl Pts',(-0.218940889961919,0.00810101478696289,
0.0106361869864059));
#27363=CARTESIAN_POINT('Ctrl Pts',(-0.218960284069682,0.00786083539543083,
0.0106506878405709));
#27364=CARTESIAN_POINT('Ctrl Pts',(-0.2189778221636,0.00765412001126297,
0.0106567575785991));
#27365=CARTESIAN_POINT('Ctrl Pts',(-0.218991322981713,0.00749805982928716,
0.0106570290092488));
#27366=CARTESIAN_POINT('',(-0.218877735683465,0.00589448248302666,0.0105110260225545));
#27367=CARTESIAN_POINT('Ctrl Pts',(-0.21899132312477,0.00749805817564265,
0.0106570290121248));
#27368=CARTESIAN_POINT('Ctrl Pts',(-0.218977743467873,0.00734187731821718,
0.0106566883481389));
#27369=CARTESIAN_POINT('Ctrl Pts',(-0.218960091281344,0.00713491968854588,
0.0106505193076562));
#27370=CARTESIAN_POINT('Ctrl Pts',(-0.218940535583419,0.00689420098152088,
0.0106358601259392));
#27371=CARTESIAN_POINT('Ctrl Pts',(-0.218930767179068,0.00677056161632596,
0.0106267188712399));
#27372=CARTESIAN_POINT('Ctrl Pts',(-0.218914264768996,0.00654649653511506,
0.010605761807423));
#27373=CARTESIAN_POINT('Ctrl Pts',(-0.218897888368177,0.00629855136156268,
0.0105760736711211));
#27374=CARTESIAN_POINT('Ctrl Pts',(-0.218886088918103,0.00609175956828754,
0.0105457931374041));
#27375=CARTESIAN_POINT('Ctrl Pts',(-0.218879322128981,0.00593446536993965,
0.0105182897355673));
#27376=CARTESIAN_POINT('Ctrl Pts',(-0.218877735683465,0.00589448248302666,
0.0105110260225545));
#27377=CARTESIAN_POINT('',(-0.218078126203157,0.00589629686000176,0.0104933642872807));
#27378=CARTESIAN_POINT('Ctrl Pts',(-0.218877732216029,0.00589445444339055,
0.0105111809578404));
#27379=CARTESIAN_POINT('Ctrl Pts',(-0.2180781221123,0.00589625235160557,
0.0104936111419841));
#27380=CARTESIAN_POINT('',(-0.218192328422137,0.00749852093264668,0.0106389711280447));
#27381=CARTESIAN_POINT('Ctrl Pts',(-0.218078126203157,0.00589629686000176,
0.0104933642872807));
#27382=CARTESIAN_POINT('Ctrl Pts',(-0.218080721583118,0.00596266805916596,
0.0105053741575296));
#27383=CARTESIAN_POINT('Ctrl Pts',(-0.218088632405485,0.00614064320404191,
0.0105356256713857));
#27384=CARTESIAN_POINT('Ctrl Pts',(-0.218101925206918,0.0063619630293138,
0.0105662762574105));
#27385=CARTESIAN_POINT('Ctrl Pts',(-0.218117994796678,0.00659663549417377,
0.0105928968047437));
#27386=CARTESIAN_POINT('Ctrl Pts',(-0.21813409507781,0.00680948317083492,
0.0106117489251953));
#27387=CARTESIAN_POINT('Ctrl Pts',(-0.218143411151013,0.00692497699745548,
0.010619841250455));
#27388=CARTESIAN_POINT('Ctrl Pts',(-0.218162246558742,0.00715281682608959,
0.0106330394232576));
#27389=CARTESIAN_POINT('Ctrl Pts',(-0.218179240829485,0.00734956024527172,
0.0106386506502909));
#27390=CARTESIAN_POINT('Ctrl Pts',(-0.218192327995395,0.0074985079816192,
0.010638971132602));
#27391=CARTESIAN_POINT('',(-0.218168590358226,0.00777884796634574,0.0106341206922536));
#27392=CARTESIAN_POINT('Ctrl Pts',(-0.218168590358226,0.00777884796634574,
0.0106341206922536));
#27393=CARTESIAN_POINT('Ctrl Pts',(-0.218176366284116,0.00768367623554517,
0.0106372600686865));
#27394=CARTESIAN_POINT('Ctrl Pts',(-0.218184322411749,0.00759032145937544,
0.0106388051579624));
#27395=CARTESIAN_POINT('Ctrl Pts',(-0.218192385381993,0.00749853455275086,
0.0106389724339549));
#27396=CARTESIAN_POINT('',(-0.218067140731952,0.00994796991712816,0.0103007556072607));
#27397=CARTESIAN_POINT('Ctrl Pts',(-0.218067140731952,0.00994796991712816,
0.0103007556072607));
#27398=CARTESIAN_POINT('Ctrl Pts',(-0.218067114512319,0.00993046860657864,
0.0103056312397923));
#27399=CARTESIAN_POINT('Ctrl Pts',(-0.218067118414372,0.00991224463072161,
0.0103106497977678));
#27400=CARTESIAN_POINT('Ctrl Pts',(-0.218067160950739,0.00989326393083498,
0.0103158106977222));
#27401=CARTESIAN_POINT('Ctrl Pts',(-0.218067298393995,0.00983193360694396,
0.0103324865667715));
#27402=CARTESIAN_POINT('Ctrl Pts',(-0.218067841273241,0.00976267553591436,
0.0103505546203546));
#27403=CARTESIAN_POINT('Ctrl Pts',(-0.218068705378173,0.00969648956991687,
0.0103669952228347));
#27404=CARTESIAN_POINT('Ctrl Pts',(-0.218070433588036,0.00956411763792191,
0.0103998764277948));
#27405=CARTESIAN_POINT('Ctrl Pts',(-0.218073437444364,0.00944413893557428,
0.0104266653780147));
#27406=CARTESIAN_POINT('Ctrl Pts',(-0.218077040466343,0.00933195733859977,
0.0104497653775281));
#27407=CARTESIAN_POINT('Ctrl Pts',(-0.218078841977332,0.0092758665401125,
0.0104613153772848));
#27408=CARTESIAN_POINT('Ctrl Pts',(-0.218080794635338,0.00922171204223149,
0.0104718823298127));
#27409=CARTESIAN_POINT('Ctrl Pts',(-0.218082474141969,0.00917710991001544,
0.0104802748380597));
#27410=CARTESIAN_POINT('Ctrl Pts',(-0.2180841536486,0.00913250777779939,
0.0104886673463067));
#27411=CARTESIAN_POINT('Ctrl Pts',(-0.218085555727444,0.0090974952685411,
0.0104950768614037));
#27412=CARTESIAN_POINT('Ctrl Pts',(-0.218088070100538,0.00904085165419785,
0.0105048607679938));
#27413=CARTESIAN_POINT('Ctrl Pts',(-0.218090584473632,0.00898420803985461,
0.0105146446745839));
#27414=CARTESIAN_POINT('Ctrl Pts',(-0.218094219358009,0.00890586854398972,
0.0105274358597375));
#27415=CARTESIAN_POINT('Ctrl Pts',(-0.218097832002953,0.00883396461653103,
0.0105381790015194));
#27416=CARTESIAN_POINT('Ctrl Pts',(-0.218101444647896,0.00876206068907235,
0.0105489221433012));
#27417=CARTESIAN_POINT('Ctrl Pts',(-0.218105029025212,0.00869663063622081,
0.0105578856505614));
#27418=CARTESIAN_POINT('Ctrl Pts',(-0.218108834948437,0.0086308229479829,
0.0105662276970903));
#27419=CARTESIAN_POINT('Ctrl Pts',(-0.218116446794885,0.00849920757150708,
0.0105829117901482));
#27420=CARTESIAN_POINT('Ctrl Pts',(-0.218124951180851,0.00836605377240373,
0.0105968281293923));
#27421=CARTESIAN_POINT('Ctrl Pts',(-0.218133937516825,0.00823651643260574,
0.0106075978802791));
#27422=CARTESIAN_POINT('Ctrl Pts',(-0.218144870524618,0.00807891796869424,
0.0106207006365895));
#27423=CARTESIAN_POINT('Ctrl Pts',(-0.218156513090154,0.00792668571681208,
0.0106293143666714));
#27424=CARTESIAN_POINT('Ctrl Pts',(-0.218168590358226,0.00777884796634574,
0.0106341206922536));
#27425=CARTESIAN_POINT('',(-0.218240142405069,0.0120825022396936,0.00940257574060758));
#27426=CARTESIAN_POINT('Ctrl Pts',(-0.218240142405069,0.0120825022396936,
0.00940257574060758));
#27427=CARTESIAN_POINT('Ctrl Pts',(-0.218227634732032,0.012011138019393,
0.00944389882041555));
#27428=CARTESIAN_POINT('Ctrl Pts',(-0.218214333283586,0.0119322602189668,
0.00948802720542979));
#27429=CARTESIAN_POINT('Ctrl Pts',(-0.21820394437181,0.0118677561250279,
0.00952309834051516));
#27430=CARTESIAN_POINT('Ctrl Pts',(-0.218193555460033,0.0118032520310891,
0.00955816947560053));
#27431=CARTESIAN_POINT('Ctrl Pts',(-0.21818607359624,0.0117532614381398,
0.00958444739640607));
#27432=CARTESIAN_POINT('Ctrl Pts',(-0.218179879131554,0.0117108626589821,
0.0096064495912512));
#27433=CARTESIAN_POINT('Ctrl Pts',(-0.218173684666869,0.0116684638798244,
0.00962845178609632));
#27434=CARTESIAN_POINT('Ctrl Pts',(-0.218168779249113,0.0116336188534382,
0.0096461000314644));
#27435=CARTESIAN_POINT('Ctrl Pts',(-0.218166009981003,0.0116140367509713,
0.00965596779068263));
#27436=CARTESIAN_POINT('Ctrl Pts',(-0.218163240712894,0.0115944546485044,
0.00966583554990086));
#27437=CARTESIAN_POINT('Ctrl Pts',(-0.218162606670219,0.0115901572125468,
0.00966796681318666));
#27438=CARTESIAN_POINT('Ctrl Pts',(-0.218161139921569,0.0115785731573726,
0.00967374443478997));
#27439=CARTESIAN_POINT('Ctrl Pts',(-0.218158206424268,0.0115554050470242,
0.0096852996779966));
#27440=CARTESIAN_POINT('Ctrl Pts',(-0.218151944072019,0.01150304239737,
0.00971134617996922));
#27441=CARTESIAN_POINT('Ctrl Pts',(-0.218144576693071,0.0114339717952896,
0.0097443075472982));
#27442=CARTESIAN_POINT('Ctrl Pts',(-0.218137209314123,0.0113649011932092,
0.00977726891462718));
#27443=CARTESIAN_POINT('Ctrl Pts',(-0.218128734773963,0.0112791720929526,
0.00981724654533353));
#27444=CARTESIAN_POINT('Ctrl Pts',(-0.218119656687413,0.0111717758059659,
0.0098644073772456));
#27445=CARTESIAN_POINT('Ctrl Pts',(-0.218115117644138,0.0111180776624726,
0.00988798779320165));
#27446=CARTESIAN_POINT('Ctrl Pts',(-0.218110428342051,0.0110589494854822,
0.00991333451127713));
#27447=CARTESIAN_POINT('Ctrl Pts',(-0.218105811430685,0.0109950563350908,
0.00993980046272872));
#27448=CARTESIAN_POINT('Ctrl Pts',(-0.218101615715708,0.0109369920954247,
0.00996385195085639));
#27449=CARTESIAN_POINT('Ctrl Pts',(-0.218097479388685,0.0108750002765632,
0.00998884314078868));
#27450=CARTESIAN_POINT('Ctrl Pts',(-0.218093504352807,0.0108074520307542,
0.0100150801168543));
#27451=CARTESIAN_POINT('Ctrl Pts',(-0.218093105309792,0.0108006710465076,
0.0100177139753542));
#27452=CARTESIAN_POINT('Ctrl Pts',(-0.218092707892206,0.010793834015395,
0.010020360228592));
#27453=CARTESIAN_POINT('Ctrl Pts',(-0.21809231220314,0.0107869392578784,
0.0100230190826078));
#27454=CARTESIAN_POINT('Ctrl Pts',(-0.218087974888293,0.0107113629109957,
0.0100521639035715));
#27455=CARTESIAN_POINT('Ctrl Pts',(-0.218083847156932,0.0106288204023902,
0.0100827571992526));
#27456=CARTESIAN_POINT('Ctrl Pts',(-0.218080324272248,0.0105466504959989,
0.0101118150425837));
#27457=CARTESIAN_POINT('Ctrl Pts',(-0.218078562829906,0.0105055655428032,
0.0101263439642493));
#27458=CARTESIAN_POINT('Ctrl Pts',(-0.218076951141839,0.0104645988975483,
0.0101405562838599));
#27459=CARTESIAN_POINT('Ctrl Pts',(-0.218075307620494,0.0104142110796976,
0.0101575130842937));
#27460=CARTESIAN_POINT('Ctrl Pts',(-0.21807366409915,0.0103638232618468,
0.0101744698847275));
#27461=CARTESIAN_POINT('Ctrl Pts',(-0.218071994487696,0.0103039249942364,
0.0101939079797174));
#27462=CARTESIAN_POINT('Ctrl Pts',(-0.218071182598693,0.0102734617826065,
0.0102036129024837));
#27463=CARTESIAN_POINT('Ctrl Pts',(-0.218070370709691,0.0102429985709766,
0.01021331782525));
#27464=CARTESIAN_POINT('Ctrl Pts',(-0.218070410527697,0.0102420558816815,
0.0102135637764575));
#27465=CARTESIAN_POINT('Ctrl Pts',(-0.218070223423177,0.0102316246750146,
0.0102168335306616));
#27466=CARTESIAN_POINT('Ctrl Pts',(-0.218070036318657,0.0102211934683478,
0.0102201032848658));
#27467=CARTESIAN_POINT('Ctrl Pts',(-0.218069623973603,0.0102012502108673,
0.0102263202343639));
#27468=CARTESIAN_POINT('Ctrl Pts',(-0.218069266473067,0.0101812898039636,
0.0102324502074999));
#27469=CARTESIAN_POINT('Ctrl Pts',(-0.218068551471994,0.0101413689901562,
0.0102447101537719));
#27470=CARTESIAN_POINT('Ctrl Pts',(-0.218068053649516,0.0101014089975905,
0.0102567221360035));
#27471=CARTESIAN_POINT('Ctrl Pts',(-0.218067671539871,0.0100547164560643,
0.0102703336166971));
#27472=CARTESIAN_POINT('Ctrl Pts',(-0.21806740768671,0.0100224744678928,
0.0102797325739003));
#27473=CARTESIAN_POINT('Ctrl Pts',(-0.21806719923304,0.0099870201303414,
0.0102898840623915));
#27474=CARTESIAN_POINT('Ctrl Pts',(-0.218067140731952,0.00994796991712816,
0.0103007556072607));
#27475=CARTESIAN_POINT('',(-0.218374802370667,0.012770849952475,0.00895972547844891));
#27476=CARTESIAN_POINT('Ctrl Pts',(-0.218374815649956,0.0127718879457763,
0.00896105065188488));
#27477=CARTESIAN_POINT('Ctrl Pts',(-0.218353771441862,0.0126721758023642,
0.00903141856439606));
#27478=CARTESIAN_POINT('Ctrl Pts',(-0.218331273836085,0.0125623045273881,
0.00910578154191035));
#27479=CARTESIAN_POINT('Ctrl Pts',(-0.218309124848712,0.0124504844741805,
0.00917776855508357));
#27480=CARTESIAN_POINT('Ctrl Pts',(-0.218286972241046,0.0123386461437777,
0.00924976733466765));
#27481=CARTESIAN_POINT('Ctrl Pts',(-0.218265157751142,0.0122252306802948,
0.00931992958099163));
#27482=CARTESIAN_POINT('Ctrl Pts',(-0.218240142405069,0.0120825022396936,
0.00940257574060758));
#27483=CARTESIAN_POINT('',(-0.217734598291091,0.0127648501815041,0.00895357626288772));
#27484=CARTESIAN_POINT('Ctrl Pts',(-0.218374739957786,0.0127719565711068,
0.00896100046641628));
#27485=CARTESIAN_POINT('Ctrl Pts',(-0.218331429070052,0.0127783087890815,
0.00895564837322821));
#27486=CARTESIAN_POINT('Ctrl Pts',(-0.218256946939598,0.0127887785152065,
0.00894674424652318));
#27487=CARTESIAN_POINT('Ctrl Pts',(-0.21821074281553,0.0127961462225746,
0.00894058692440315));
#27488=CARTESIAN_POINT('Ctrl Pts',(-0.218041570987848,0.0128061304184166,
0.0089301565708801));
#27489=CARTESIAN_POINT('Ctrl Pts',(-0.217906442184221,0.0127950441559907,
0.00893548464298887));
#27490=CARTESIAN_POINT('Ctrl Pts',(-0.217785680204843,0.0127750237429539,
0.00894736337346077));
#27491=CARTESIAN_POINT('Ctrl Pts',(-0.217734598291091,0.0127648501815041,
0.00895357626288772));
#27492=CARTESIAN_POINT('',(-0.217125125910816,0.0125755126764789,0.00907193450211442));
#27493=CARTESIAN_POINT('Ctrl Pts',(-0.217734109130233,0.0127647526978011,
0.00895363580049309));
#27494=CARTESIAN_POINT('Ctrl Pts',(-0.217682923213736,0.0127545455248966,
0.00895987032802755));
#27495=CARTESIAN_POINT('Ctrl Pts',(-0.21759918313078,0.0127337893410419,
0.00897289746848775));
#27496=CARTESIAN_POINT('Ctrl Pts',(-0.217407044851832,0.0126752427904671,
0.00900981145746635));
#27497=CARTESIAN_POINT('Ctrl Pts',(-0.217324996157004,0.0126461555887933,
0.00902814986930927));
#27498=CARTESIAN_POINT('Ctrl Pts',(-0.217195934007024,0.0126008953837128,
0.00905634036820808));
#27499=CARTESIAN_POINT('Ctrl Pts',(-0.217125125910815,0.0125755126764789,
0.00907193450211442));
#27500=CARTESIAN_POINT('',(-0.216865308842943,0.0101529809944104,0.0102146591943612));
#27501=CARTESIAN_POINT('Ctrl Pts',(-0.217125116861616,0.012575509432593,
0.00907193649502888));
#27502=CARTESIAN_POINT('Ctrl Pts',(-0.217103825873541,0.0124556142350541,
0.00915177820299817));
#27503=CARTESIAN_POINT('Ctrl Pts',(-0.21708543586629,0.0123492680897509,
0.00921865902026808));
#27504=CARTESIAN_POINT('Ctrl Pts',(-0.217069076401892,0.0122522130671093,
0.00927757091324666));
#27505=CARTESIAN_POINT('Ctrl Pts',(-0.217060896669693,0.0122036855557885,
0.00930702685973596));
#27506=CARTESIAN_POINT('Ctrl Pts',(-0.217053225625487,0.0121574472103491,
0.00933443792808312));
#27507=CARTESIAN_POINT('Ctrl Pts',(-0.217046930550406,0.0121191622263696,
0.00935679855708027));
#27508=CARTESIAN_POINT('Ctrl Pts',(-0.217040635475325,0.0120808772423901,
0.00937915918607743));
#27509=CARTESIAN_POINT('Ctrl Pts',(-0.217035713759174,0.0120506219046572,
0.00939659786253759));
#27510=CARTESIAN_POINT('Ctrl Pts',(-0.21702870095117,0.0120061367071534,
0.00942173938324392));
#27511=CARTESIAN_POINT('Ctrl Pts',(-0.217021688143166,0.0119616515096496,
0.00944688090395027));
#27512=CARTESIAN_POINT('Ctrl Pts',(-0.217012588916355,0.0119028062528194,
0.00947949707937416));
#27513=CARTESIAN_POINT('Ctrl Pts',(-0.217004505587796,0.0118486712007352,
0.00950870635721085));
#27514=CARTESIAN_POINT('Ctrl Pts',(-0.216996422259236,0.011794536148651,
0.00953791563504754));
#27515=CARTESIAN_POINT('Ctrl Pts',(-0.216989351628543,0.0117451932488908,
0.00956387226315191));
#27516=CARTESIAN_POINT('Ctrl Pts',(-0.216982616444841,0.0116968197156397,
0.00958881655457117));
#27517=CARTESIAN_POINT('Ctrl Pts',(-0.216969146077438,0.0116000726491376,
0.00963870513740967));
#27518=CARTESIAN_POINT('Ctrl Pts',(-0.216957017981496,0.0115071990302703,
0.00968452334188844));
#27519=CARTESIAN_POINT('Ctrl Pts',(-0.21694575682019,0.0114110167413363,
0.00972996806454795));
#27520=CARTESIAN_POINT('Ctrl Pts',(-0.216923234497579,0.0112186521634682,
0.00982085750986698));
#27521=CARTESIAN_POINT('Ctrl Pts',(-0.216904190106109,0.0110128311572041,
0.00990977153176363));
#27522=CARTESIAN_POINT('Ctrl Pts',(-0.216890581505355,0.0107996070424065,
0.00999216578621756));
#27523=CARTESIAN_POINT('Ctrl Pts',(-0.216876972904601,0.0105863829276089,
0.0100745600406715));
#27524=CARTESIAN_POINT('Ctrl Pts',(-0.216868805975623,0.0103656090193981,
0.0101501540238545));
#27525=CARTESIAN_POINT('Ctrl Pts',(-0.21686536061782,0.0101561495392998,
0.010213698561222));
#27526=CARTESIAN_POINT('Ctrl Pts',(-0.216865343240117,0.0101550930670962,
0.0102140190673045));
#27527=CARTESIAN_POINT('Ctrl Pts',(-0.216865325981855,0.0101540368923536,
0.0102143392976063));
#27528=CARTESIAN_POINT('Ctrl Pts',(-0.216865308842943,0.0101529809944104,
0.0102146591943612));
#27529=CARTESIAN_POINT('',(-0.216992039547609,0.00749886050208332,0.0106118434853889));
#27530=CARTESIAN_POINT('Ctrl Pts',(-0.216865308842943,0.0101529809944104,
0.0102146591943612));
#27531=CARTESIAN_POINT('Ctrl Pts',(-0.216861927967694,0.00994469453364889,
0.0102777746867437));
#27532=CARTESIAN_POINT('Ctrl Pts',(-0.21686319133722,0.00974782023658563,
0.0103301991819165));
#27533=CARTESIAN_POINT('Ctrl Pts',(-0.216868396633366,0.00953023558922692,
0.0103799113220085));
#27534=CARTESIAN_POINT('Ctrl Pts',(-0.216871012475229,0.0094208917568765,
0.0104048933966999));
#27535=CARTESIAN_POINT('Ctrl Pts',(-0.216874630000908,0.00930625788422588,
0.0104289129990826));
#27536=CARTESIAN_POINT('Ctrl Pts',(-0.21687910933658,0.0091927203230611,
0.0104504437509994));
#27537=CARTESIAN_POINT('Ctrl Pts',(-0.216881349004416,0.0091359515424787,
0.0104612091269577));
#27538=CARTESIAN_POINT('Ctrl Pts',(-0.216883802899309,0.00907946720242295,
0.0104714071013028));
#27539=CARTESIAN_POINT('Ctrl Pts',(-0.216886764362047,0.00901787666734833,
0.0104818695431398));
#27540=CARTESIAN_POINT('Ctrl Pts',(-0.216889725824785,0.00895628613227371,
0.0104923319849768));
#27541=CARTESIAN_POINT('Ctrl Pts',(-0.216893198774523,0.0088895590569111,
0.0105028838422591));
#27542=CARTESIAN_POINT('Ctrl Pts',(-0.216895951836754,0.00883901354239403,
0.0105104550763784));
#27543=CARTESIAN_POINT('Ctrl Pts',(-0.216898704898984,0.00878846802787697,
0.0105180263104978));
#27544=CARTESIAN_POINT('Ctrl Pts',(-0.216900732586707,0.00875413964732611,
0.0105228613321503));
#27545=CARTESIAN_POINT('Ctrl Pts',(-0.216903232709149,0.0087130859209821,
0.0105284362036829));
#27546=CARTESIAN_POINT('Ctrl Pts',(-0.216905732831591,0.00867203219463808,
0.0105340110752155));
#27547=CARTESIAN_POINT('Ctrl Pts',(-0.216908708333334,0.00862423631372646,
0.010540194832042));
#27548=CARTESIAN_POINT('Ctrl Pts',(-0.216911865038629,0.00857530837293379,
0.0105460897542788));
#27549=CARTESIAN_POINT('Ctrl Pts',(-0.216918178449217,0.00847745249134844,
0.0105578795987525));
#27550=CARTESIAN_POINT('Ctrl Pts',(-0.216925213052354,0.00837508469828663,
0.0105686748320112));
#27551=CARTESIAN_POINT('Ctrl Pts',(-0.21693318406884,0.00826407226117057,
0.0105782317652135));
#27552=CARTESIAN_POINT('Ctrl Pts',(-0.216949126069373,0.00804204783873716,
0.0105973455927233));
#27553=CARTESIAN_POINT('Ctrl Pts',(-0.216968817133433,0.00778544299277556,
0.0106113550316752));
#27554=CARTESIAN_POINT('Ctrl Pts',(-0.216992039472508,0.007498860496276,
0.0106118436486008));
#27555=CARTESIAN_POINT('',(-0.216882060774437,0.00589894167293227,0.0104673301115656));
#27556=CARTESIAN_POINT('Ctrl Pts',(-0.216992039614274,0.00749885874677076,
0.0106118436515835));
#27557=CARTESIAN_POINT('Ctrl Pts',(-0.216968696387162,0.00721250076742298,
0.010611279820427));
#27558=CARTESIAN_POINT('Ctrl Pts',(-0.216948881624643,0.00695603249159739,
0.010597224811972));
#27559=CARTESIAN_POINT('Ctrl Pts',(-0.216932813946421,0.00673401117115549,
0.0105780613240776));
#27560=CARTESIAN_POINT('Ctrl Pts',(-0.216924780107311,0.00662300051093453,
0.0105684795801305));
#27561=CARTESIAN_POINT('Ctrl Pts',(-0.216917682194779,0.00652060110169468,
0.0105576579948596));
#27562=CARTESIAN_POINT('Ctrl Pts',(-0.216911304122608,0.00642272431681689,
0.0105458427496648));
#27563=CARTESIAN_POINT('Ctrl Pts',(-0.216908115086522,0.006373785924378,
0.0105399351270675));
#27564=CARTESIAN_POINT('Ctrl Pts',(-0.216905106906988,0.00632598223781525,
0.0105337393045049));
#27565=CARTESIAN_POINT('Ctrl Pts',(-0.21690257496323,0.00628486308718463,
0.0105281454815176));
#27566=CARTESIAN_POINT('Ctrl Pts',(-0.216900043019471,0.00624374393655401,
0.0105225516585303));
#27567=CARTESIAN_POINT('Ctrl Pts',(-0.216897984395554,0.00620929264573658,
0.0105176895280296));
#27568=CARTESIAN_POINT('Ctrl Pts',(-0.216895196305536,0.00615881306811144,
0.0105101149587025));
#27569=CARTESIAN_POINT('Ctrl Pts',(-0.216892408215518,0.0061083334904863,
0.0105025403893753));
#27570=CARTESIAN_POINT('Ctrl Pts',(-0.216888896080399,0.00604186083493618,
0.0104920119045022));
#27571=CARTESIAN_POINT('Ctrl Pts',(-0.216885892590301,0.00598048099048582,
0.0104815726477788));
#27572=CARTESIAN_POINT('Ctrl Pts',(-0.216884519120359,0.00595241252061771,
0.0104767988663297));
#27573=CARTESIAN_POINT('Ctrl Pts',(-0.216883251207378,0.00592540375787019,
0.0104720739912376));
#27574=CARTESIAN_POINT('Ctrl Pts',(-0.216882060774437,0.00589894167293226,
0.0104673301115656));
#27575=CARTESIAN_POINT('',(-0.216081273279547,0.00590074222848907,0.0104497344249182));
#27576=CARTESIAN_POINT('Ctrl Pts',(-0.216882060774437,0.00589894167293227,
0.0104673301115656));
#27577=CARTESIAN_POINT('Ctrl Pts',(-0.216081273279547,0.00590074222848907,
0.0104497344249183));
#27578=CARTESIAN_POINT('',(-0.216192972388059,0.00749913681337735,0.0105937841926617));
#27579=CARTESIAN_POINT('Ctrl Pts',(-0.216081273279547,0.00590074222848906,
0.0104497344249182));
#27580=CARTESIAN_POINT('Ctrl Pts',(-0.216082791066702,0.00593458609584699,
0.0104557868301711));
#27581=CARTESIAN_POINT('Ctrl Pts',(-0.21608442756336,0.00596908492338023,
0.0104617673197763));
#27582=CARTESIAN_POINT('Ctrl Pts',(-0.216086248348797,0.00600539180340494,
0.0104678328343025));
#27583=CARTESIAN_POINT('Ctrl Pts',(-0.216089278806263,0.00606581982170094,
0.0104779280840874));
#27584=CARTESIAN_POINT('Ctrl Pts',(-0.216092823551175,0.00613128149711444,
0.0104881115930235));
#27585=CARTESIAN_POINT('Ctrl Pts',(-0.216095619523186,0.00618069805460236,
0.0104953971611742));
#27586=CARTESIAN_POINT('Ctrl Pts',(-0.216098415495197,0.00623011461209028,
0.0105026827293249));
#27587=CARTESIAN_POINT('Ctrl Pts',(-0.216100457387313,0.00626345219645691,
0.0105073067142719));
#27588=CARTESIAN_POINT('Ctrl Pts',(-0.21610298377209,0.00630350339604497,
0.0105126662070077));
#27589=CARTESIAN_POINT('Ctrl Pts',(-0.216105510156868,0.00634355459563303,
0.0105180256997435));
#27590=CARTESIAN_POINT('Ctrl Pts',(-0.216108523881857,0.00639033543187153,
0.0105239940636935));
#27591=CARTESIAN_POINT('Ctrl Pts',(-0.216111720854193,0.00643827294491396,
0.0105296922193121));
#27592=CARTESIAN_POINT('Ctrl Pts',(-0.216118114798864,0.00653414797099881,
0.0105410885305492));
#27593=CARTESIAN_POINT('Ctrl Pts',(-0.216125238212349,0.00663463402037178,
0.0105515602441198));
#27594=CARTESIAN_POINT('Ctrl Pts',(-0.216133313517992,0.00674383793891926,
0.0105608594503349));
#27595=CARTESIAN_POINT('Ctrl Pts',(-0.216149464114079,0.00696224557046546,
0.0105794578452618));
#27596=CARTESIAN_POINT('Ctrl Pts',(-0.216169425475875,0.00721552619151367,
0.0105932247838232));
#27597=CARTESIAN_POINT('Ctrl Pts',(-0.216192972777483,0.00749913678123476,
0.0105937840962717));
#27598=CARTESIAN_POINT('',(-0.216064560542751,0.0101118708899842,0.0102094226853462));
#27599=CARTESIAN_POINT('Ctrl Pts',(-0.216192972843966,0.00749913758197346,
0.0105937840978508));
#27600=CARTESIAN_POINT('Ctrl Pts',(-0.216169511009818,0.0077829711165385,
0.010593280960363));
#27601=CARTESIAN_POINT('Ctrl Pts',(-0.21614963981566,0.00803639489599444,
0.0105795447869103));
#27602=CARTESIAN_POINT('Ctrl Pts',(-0.216133579485032,0.00825490153361357,
0.0105609705977376));
#27603=CARTESIAN_POINT('Ctrl Pts',(-0.216125549319719,0.00836415485242313,
0.0105516835031512));
#27604=CARTESIAN_POINT('Ctrl Pts',(-0.216118471086411,0.00846467923742192,
0.0105412215031039));
#27605=CARTESIAN_POINT('Ctrl Pts',(-0.216112126913198,0.00856054432573829,
0.0105298400899683));
#27606=CARTESIAN_POINT('Ctrl Pts',(-0.216108954826591,0.00860847686989648,
0.0105241493834004));
#27607=CARTESIAN_POINT('Ctrl Pts',(-0.216105967127652,0.00865524070694128,
0.0105181900976421));
#27608=CARTESIAN_POINT('Ctrl Pts',(-0.216103461654188,0.00869531413130442,
0.0105128334261085));
#27609=CARTESIAN_POINT('Ctrl Pts',(-0.216100956180724,0.00873538755566756,
0.010507476754575));
#27610=CARTESIAN_POINT('Ctrl Pts',(-0.216098930112014,0.00876878642481055,
0.0105028481395904));
#27611=CARTESIAN_POINT('Ctrl Pts',(-0.216096170413117,0.00881809405563216,
0.0104955859918311));
#27612=CARTESIAN_POINT('Ctrl Pts',(-0.21609341071422,0.00886740168645377,
0.0104883238440719));
#27613=CARTESIAN_POINT('Ctrl Pts',(-0.216089922626847,0.00893258466305817,
0.0104781947154111));
#27614=CARTESIAN_POINT('Ctrl Pts',(-0.216086943126735,0.00899279416913099,
0.0104681492303132));
#27615=CARTESIAN_POINT('Ctrl Pts',(-0.216083963626623,0.00905300367520381,
0.0104581037452152));
#27616=CARTESIAN_POINT('Ctrl Pts',(-0.216081488978781,0.00910826813489991,
0.0104483086920604));
#27617=CARTESIAN_POINT('Ctrl Pts',(-0.21607922328395,0.00916383245088221,
0.0104379673721727));
#27618=CARTESIAN_POINT('Ctrl Pts',(-0.216074691894287,0.0092749610828468,
0.0104172847323973));
#27619=CARTESIAN_POINT('Ctrl Pts',(-0.216071000885213,0.00938725056091497,
0.010394212662589));
#27620=CARTESIAN_POINT('Ctrl Pts',(-0.216068305929166,0.00949480823549394,
0.0103701146189438));
#27621=CARTESIAN_POINT('Ctrl Pts',(-0.216062916017071,0.00970992358465189,
0.0103219185316535));
#27622=CARTESIAN_POINT('Ctrl Pts',(-0.216061489104538,0.00990631862573795,
0.0102705706903127));
#27623=CARTESIAN_POINT('Ctrl Pts',(-0.216064560542751,0.0101118708899842,
0.0102094226853462));
#27624=CARTESIAN_POINT('',(-0.216308818597444,0.0125017236340575,0.00910474588717665));
#27625=CARTESIAN_POINT('Ctrl Pts',(-0.216064560542751,0.0101118708899842,
0.0102094226853462));
#27626=CARTESIAN_POINT('Ctrl Pts',(-0.216067631980963,0.0103174231542305,
0.0101482746803796));
#27627=CARTESIAN_POINT('Ctrl Pts',(-0.216075221767079,0.0105318422526481,
0.0100764137690631));
#27628=CARTESIAN_POINT('Ctrl Pts',(-0.216088333546939,0.010742801430779,
0.00999663280107556));
#27629=CARTESIAN_POINT('Ctrl Pts',(-0.216089497788197,0.0107615332415328,
0.00998954876705846));
#27630=CARTESIAN_POINT('Ctrl Pts',(-0.216090705584094,0.0107802390027244,
0.00998240422592453));
#27631=CARTESIAN_POINT('Ctrl Pts',(-0.216091955010119,0.0107989083874413,
0.00997520316767751));
#27632=CARTESIAN_POINT('Ctrl Pts',(-0.216104776721723,0.0109904951337436,
0.0099013053215298));
#27633=CARTESIAN_POINT('Ctrl Pts',(-0.216121982515131,0.011178144367165,
0.00982123433870025));
#27634=CARTESIAN_POINT('Ctrl Pts',(-0.216141492564637,0.0113514549451286,
0.0097409837926396));
#27635=CARTESIAN_POINT('Ctrl Pts',(-0.216152198178685,0.0114465544556392,
0.00969694846751261));
#27636=CARTESIAN_POINT('Ctrl Pts',(-0.216163593829438,0.0115374139528911,
0.00965302332847526));
#27637=CARTESIAN_POINT('Ctrl Pts',(-0.216176229165743,0.0116325830866664,
0.00960496228856018));
#27638=CARTESIAN_POINT('Ctrl Pts',(-0.216182546833896,0.0116801676535541,
0.00958093176860265));
#27639=CARTESIAN_POINT('Ctrl Pts',(-0.216189174365757,0.011728828677417,
0.00955586940376413));
#27640=CARTESIAN_POINT('Ctrl Pts',(-0.216196770953834,0.011782465366349,
0.00952753419512687));
#27641=CARTESIAN_POINT('Ctrl Pts',(-0.216204367541912,0.011836102055281,
0.0094991989864896));
#27642=CARTESIAN_POINT('Ctrl Pts',(-0.216212936459505,0.0118946326686426,
0.00946743362499819));
#27643=CARTESIAN_POINT('Ctrl Pts',(-0.216219428400284,0.0119382154723126,
0.00944332261912472));
#27644=CARTESIAN_POINT('Ctrl Pts',(-0.216225920341063,0.0119817982759826,
0.00941921161325124));
#27645=CARTESIAN_POINT('Ctrl Pts',(-0.216230330548599,0.0120105625630745,
0.00940298648815025));
#27646=CARTESIAN_POINT('Ctrl Pts',(-0.216236085834532,0.0120477886518902,
0.00938172145544078));
#27647=CARTESIAN_POINT('Ctrl Pts',(-0.216241841120465,0.012085014740706,
0.0093604564227313));
#27648=CARTESIAN_POINT('Ctrl Pts',(-0.21624894412124,0.0121306276008068,
0.00933402218323825));
#27649=CARTESIAN_POINT('Ctrl Pts',(-0.216256536977254,0.0121787064133767,
0.00930549209652678));
#27650=CARTESIAN_POINT('Ctrl Pts',(-0.216271722689283,0.0122748640385166,
0.00924843192310387));
#27651=CARTESIAN_POINT('Ctrl Pts',(-0.216288863445513,0.0123810212896488,
0.00918320633356622));
#27652=CARTESIAN_POINT('Ctrl Pts',(-0.216308820388115,0.0125016658513436,
0.00910465761837708));
#27653=CARTESIAN_POINT('',(-0.215098009459442,0.0124568456463798,0.0091097211321646));
#27654=CARTESIAN_POINT('',(-0.215098005579294,0.0124567804451349,0.00910961844171237));
#27655=CARTESIAN_POINT('',(-0.214992631591026,0.00749947366491129,0.0105666553962969));
#27656=CARTESIAN_POINT('Ctrl Pts',(-0.215098003539502,0.0124568465122051,
0.00910972101494852));
#27657=CARTESIAN_POINT('Ctrl Pts',(-0.215078872046694,0.0123380764007811,
0.00918586969150996));
#27658=CARTESIAN_POINT('Ctrl Pts',(-0.215054131147941,0.0121807387915435,
0.00928132552116643));
#27659=CARTESIAN_POINT('Ctrl Pts',(-0.215026675832497,0.0119991748863345,
0.00938495086713676));
#27660=CARTESIAN_POINT('Ctrl Pts',(-0.215013610883414,0.0119113355207368,
0.00943387856890056));
#27661=CARTESIAN_POINT('Ctrl Pts',(-0.214989031420947,0.0117378895077981,
0.00952674741057423));
#27662=CARTESIAN_POINT('Ctrl Pts',(-0.214963576161329,0.0115442929638235,
0.00962484494645074));
#27663=CARTESIAN_POINT('Ctrl Pts',(-0.214925227292808,0.0112265332226401,
0.00977661166210876));
#27664=CARTESIAN_POINT('Ctrl Pts',(-0.214881441558165,0.0107160404592738,
0.00998992422239802));
#27665=CARTESIAN_POINT('Ctrl Pts',(-0.214860205463023,0.0100784557054517,
0.0102002397837531));
#27666=CARTESIAN_POINT('Ctrl Pts',(-0.214864228119364,0.00959024177348553,
0.0103262146705758));
#27667=CARTESIAN_POINT('Ctrl Pts',(-0.21487723133723,0.00920082508041648,
0.0104053314978383));
#27668=CARTESIAN_POINT('Ctrl Pts',(-0.214887103785318,0.00898179083587286,
0.0104437555890133));
#27669=CARTESIAN_POINT('Ctrl Pts',(-0.214897482284705,0.00878838978616738,
0.010473386966028));
#27670=CARTESIAN_POINT('Ctrl Pts',(-0.214903550412397,0.00868845669247843,
0.0104869713617598));
#27671=CARTESIAN_POINT('Ctrl Pts',(-0.21491541624627,0.00850295185423011,
0.010510401431549));
#27672=CARTESIAN_POINT('Ctrl Pts',(-0.214939980745825,0.00815449444337298,
0.0105460278742306));
#27673=CARTESIAN_POINT('Ctrl Pts',(-0.214969453551002,0.00777926145812896,
0.0105661478361195));
#27674=CARTESIAN_POINT('Ctrl Pts',(-0.214992631591026,0.00749947366491129,
0.0105666553962969));
#27675=CARTESIAN_POINT('',(-0.214881405086202,0.00590343232515273,0.010423413516648));
#27676=CARTESIAN_POINT('Ctrl Pts',(-0.214992631712683,0.00749947219635508,
0.0105666553989609));
#27677=CARTESIAN_POINT('Ctrl Pts',(-0.214969345086721,0.00721945056383405,
0.0105661127593133));
#27678=CARTESIAN_POINT('Ctrl Pts',(-0.214939718136512,0.00684386172483547,
0.0105459149352619));
#27679=CARTESIAN_POINT('Ctrl Pts',(-0.214914989990807,0.00649491171184848,
0.0105101571201946));
#27680=CARTESIAN_POINT('Ctrl Pts',(-0.214903034202549,0.00630918418157328,
0.010486651391931));
#27681=CARTESIAN_POINT('Ctrl Pts',(-0.214896903335095,0.00620889075875752,
0.0104729859984906));
#27682=CARTESIAN_POINT('Ctrl Pts',(-0.214887550141049,0.00603608466518826,
0.0104464571131324));
#27683=CARTESIAN_POINT('Ctrl Pts',(-0.214883083515895,0.00594134340781319,
0.0104301910449969));
#27684=CARTESIAN_POINT('Ctrl Pts',(-0.214881405086202,0.00590343232515273,
0.010423413516648));
#27685=CARTESIAN_POINT('',(-0.214076623138809,0.00590524964646623,0.0104056862898775));
#27686=CARTESIAN_POINT('Ctrl Pts',(-0.214881405971139,0.00590344010746865,
0.0104233697659896));
#27687=CARTESIAN_POINT('Ctrl Pts',(-0.214076623138809,0.00590524964646622,
0.0104056862898775));
#27688=CARTESIAN_POINT('',(-0.214193732109028,0.0074996355091127,0.0105485995725959));
#27689=CARTESIAN_POINT('Ctrl Pts',(-0.214076623138809,0.00590524964646623,
0.0104056862898775));
#27690=CARTESIAN_POINT('Ctrl Pts',(-0.214081030343595,0.0060102586589984,
0.0104243439605997));
#27691=CARTESIAN_POINT('Ctrl Pts',(-0.214086490632834,0.00611852560763557,
0.0104415773943015));
#27692=CARTESIAN_POINT('Ctrl Pts',(-0.214092160447561,0.00621752004041992,
0.0104557189458005));
#27693=CARTESIAN_POINT('Ctrl Pts',(-0.214098162696277,0.00632231873944863,
0.01047068964827));
#27694=CARTESIAN_POINT('Ctrl Pts',(-0.214104391052137,0.00641667668968166,
0.0104825643640814));
#27695=CARTESIAN_POINT('Ctrl Pts',(-0.214111719185919,0.00651975718570092,
0.010493857431119));
#27696=CARTESIAN_POINT('Ctrl Pts',(-0.21411538325281,0.00657129743371054,
0.0104995039646378));
#27697=CARTESIAN_POINT('Ctrl Pts',(-0.214119323016901,0.00662501987917694,
0.0105049718007339));
#27698=CARTESIAN_POINT('Ctrl Pts',(-0.214123856766003,0.00668403817010079,
0.0105103742411977));
#27699=CARTESIAN_POINT('Ctrl Pts',(-0.214128390515105,0.00674305646102463,
0.0105157766816615));
#27700=CARTESIAN_POINT('Ctrl Pts',(-0.214133521551491,0.00680738547514745,
0.0105209671307191));
#27701=CARTESIAN_POINT('Ctrl Pts',(-0.21413756648669,0.00685708916630594,
0.0105245747996913));
#27702=CARTESIAN_POINT('Ctrl Pts',(-0.214141611421888,0.00690679285746443,
0.0105281824686634));
#27703=CARTESIAN_POINT('Ctrl Pts',(-0.214144565043588,0.00694185507893422,
0.010530438346143));
#27704=CARTESIAN_POINT('Ctrl Pts',(-0.214148272384198,0.00698531422333201,
0.0105329838694676));
#27705=CARTESIAN_POINT('Ctrl Pts',(-0.214151979724807,0.00702877336772981,
0.0105355293927922));
#27706=CARTESIAN_POINT('Ctrl Pts',(-0.214156443777976,0.00708063634940085,
0.0105382319945326));
#27707=CARTESIAN_POINT('Ctrl Pts',(-0.214161201957962,0.0071351444945118,
0.0105405294888697));
#27708=CARTESIAN_POINT('Ctrl Pts',(-0.214170718317934,0.0072441607847337,
0.010545124477544));
#27709=CARTESIAN_POINT('Ctrl Pts',(-0.214181406291325,0.00736375332914952,
0.0105483155487178));
#27710=CARTESIAN_POINT('Ctrl Pts',(-0.214193732134263,0.00749963493590358,
0.0105485996009061));
#27711=CARTESIAN_POINT('',(-0.214298616704839,0.0123842992752686,0.00914002570287846));
#27712=CARTESIAN_POINT('Ctrl Pts',(-0.214193732082292,0.00749963550673335,
0.0105485995997545));
#27713=CARTESIAN_POINT('Ctrl Pts',(-0.21418135470816,0.00763558496278679,
0.0105483253328312));
#27714=CARTESIAN_POINT('Ctrl Pts',(-0.214170627765918,0.00775519907777331,
0.0105451404750745));
#27715=CARTESIAN_POINT('Ctrl Pts',(-0.214161082456179,0.00786421691816746,
0.0105405524240497));
#27716=CARTESIAN_POINT('Ctrl Pts',(-0.21415630979463,0.00791872591465589,
0.0105382583953265));
#27717=CARTESIAN_POINT('Ctrl Pts',(-0.214151833770909,0.00797058473444226,
0.0105355591998067));
#27718=CARTESIAN_POINT('Ctrl Pts',(-0.214148119499745,0.00801400838918349,
0.0105330187644806));
#27719=CARTESIAN_POINT('Ctrl Pts',(-0.214144405228581,0.00805743204392473,
0.0105304783291545));
#27720=CARTESIAN_POINT('Ctrl Pts',(-0.214141449705021,0.00809242746166554,
0.0105282297214948));
#27721=CARTESIAN_POINT('Ctrl Pts',(-0.214137397798384,0.0081421383557626,
0.0105246256114229));
#27722=CARTESIAN_POINT('Ctrl Pts',(-0.214133345891746,0.00819184924985966,
0.010521021501351));
#27723=CARTESIAN_POINT('Ctrl Pts',(-0.214128202838708,0.0082562594338092,
0.0105158298221815));
#27724=CARTESIAN_POINT('Ctrl Pts',(-0.214123663791741,0.00831534124163444,
0.010510425603309));
#27725=CARTESIAN_POINT('Ctrl Pts',(-0.214119124744774,0.00837442304945969,
0.0105050213844365));
#27726=CARTESIAN_POINT('Ctrl Pts',(-0.214115186372202,0.00842819143853195,
0.0104995525234799));
#27727=CARTESIAN_POINT('Ctrl Pts',(-0.214111522655542,0.00847986203160938,
0.0104938941059396));
#27728=CARTESIAN_POINT('Ctrl Pts',(-0.214104195222222,0.00858320321776425,
0.0104825772708589));
#27729=CARTESIAN_POINT('Ctrl Pts',(-0.214097963705752,0.00867815821440496,
0.0104706218623882));
#27730=CARTESIAN_POINT('Ctrl Pts',(-0.214092018994477,0.00878283988616916,
0.0104556648092747));
#27731=CARTESIAN_POINT('Ctrl Pts',(-0.214086074283202,0.00888752155793336,
0.0104407077561611));
#27732=CARTESIAN_POINT('Ctrl Pts',(-0.21408042455788,0.00900188078205631,
0.0104223849419874));
#27733=CARTESIAN_POINT('Ctrl Pts',(-0.214075995668272,0.00911209226776831,
0.0104025901996249));
#27734=CARTESIAN_POINT('Ctrl Pts',(-0.214071566778664,0.00922230375348032,
0.0103827954572624));
#27735=CARTESIAN_POINT('Ctrl Pts',(-0.214068354575988,0.00932840606684898,
0.0103617148722127));
#27736=CARTESIAN_POINT('Ctrl Pts',(-0.21406606092194,0.00943215845042625,
0.0103393090665216));
#27737=CARTESIAN_POINT('Ctrl Pts',(-0.214061473613844,0.0096396632175808,
0.0102944974551394));
#27738=CARTESIAN_POINT('Ctrl Pts',(-0.214060553047391,0.00983780282009029,
0.010244714261598));
#27739=CARTESIAN_POINT('Ctrl Pts',(-0.214064457168896,0.0100437599210286,
0.0101854017246378));
#27740=CARTESIAN_POINT('Ctrl Pts',(-0.214068361290401,0.0102497170219669,
0.0101260891876776));
#27741=CARTESIAN_POINT('Ctrl Pts',(-0.214077112891257,0.0104632184510982,
0.0100562165635347));
#27742=CARTESIAN_POINT('Ctrl Pts',(-0.214089778662037,0.0106579611285809,
0.00998505527974717));
#27743=CARTESIAN_POINT('Ctrl Pts',(-0.214092686874479,0.0107026763762739,
0.0099687157979662));
#27744=CARTESIAN_POINT('Ctrl Pts',(-0.214095800114063,0.0107464159991479,
0.00995234655654839));
#27745=CARTESIAN_POINT('Ctrl Pts',(-0.214099201263413,0.0107904022882614,
0.0099355014535182));
#27746=CARTESIAN_POINT('Ctrl Pts',(-0.214103206412418,0.0108421999672176,
0.00991566488043311));
#27747=CARTESIAN_POINT('Ctrl Pts',(-0.214107610809052,0.0108943415937377,
0.00989517215769459));
#27748=CARTESIAN_POINT('Ctrl Pts',(-0.214112549798375,0.0109487698960818,
0.00987316106416006));
#27749=CARTESIAN_POINT('Ctrl Pts',(-0.214121682948841,0.0110494183976918,
0.00983245827741794));
#27750=CARTESIAN_POINT('Ctrl Pts',(-0.214132652227213,0.0111577726619784,
0.00978628689672306));
#27751=CARTESIAN_POINT('Ctrl Pts',(-0.214143344904991,0.0112548181255048,
0.00974288121974354));
#27752=CARTESIAN_POINT('Ctrl Pts',(-0.214154037582768,0.0113518635890311,
0.00969947554276402));
#27753=CARTESIAN_POINT('Ctrl Pts',(-0.214164444648207,0.011437799618632,
0.00965926249227631));
#27754=CARTESIAN_POINT('Ctrl Pts',(-0.214176207369434,0.0115304860340288,
0.00961406849670311));
#27755=CARTESIAN_POINT('Ctrl Pts',(-0.214182088730047,0.0115768292417272,
0.00959147149891651));
#27756=CARTESIAN_POINT('Ctrl Pts',(-0.214188309585668,0.0116248432647129,
0.00956760069860009));
#27757=CARTESIAN_POINT('Ctrl Pts',(-0.21419536162867,0.0116774425761363,
0.00954078007922124));
#27758=CARTESIAN_POINT('Ctrl Pts',(-0.214202413671673,0.0117300418875597,
0.00951395945984239));
#27759=CARTESIAN_POINT('Ctrl Pts',(-0.214210299808724,0.0117871572668679,
0.00948405000663253));
#27760=CARTESIAN_POINT('Ctrl Pts',(-0.21421633123925,0.0118301674283987,
0.00946109345410688));
#27761=CARTESIAN_POINT('Ctrl Pts',(-0.214222362669776,0.0118731775899295,
0.00943813690158122));
#27762=CARTESIAN_POINT('Ctrl Pts',(-0.214226535000872,0.0119021970009535,
0.00942234608511879));
#27763=CARTESIAN_POINT('Ctrl Pts',(-0.214231897691757,0.0119391914736748,
0.0094019549473163));
#27764=CARTESIAN_POINT('Ctrl Pts',(-0.214237260382641,0.0119761859463962,
0.00938156380951382));
#27765=CARTESIAN_POINT('Ctrl Pts',(-0.214243815897177,0.012021088180201,
0.00935645208833323));
#27766=CARTESIAN_POINT('Ctrl Pts',(-0.214250800777236,0.0120683176568899,
0.00932941698431488));
#27767=CARTESIAN_POINT('Ctrl Pts',(-0.214264770500878,0.0121627763636332,
0.00927534691745677));
#27768=CARTESIAN_POINT('Ctrl Pts',(-0.214280453653274,0.0122666637658923,
0.0092137826947823));
#27769=CARTESIAN_POINT('Ctrl Pts',(-0.214298616704839,0.0123842992752686,
0.00914002570287846));
#27770=CARTESIAN_POINT('',(-0.213096469059738,0.0123844644794285,0.0091159443654941));
#27771=CARTESIAN_POINT('',(-0.214298616958418,0.0123842966787186,0.00914001954130824));
#27772=CARTESIAN_POINT('',(-0.212993233607984,0.00749979378001809,0.0105214673239713));
#27773=CARTESIAN_POINT('Ctrl Pts',(-0.213096467719112,0.0123844633545295,
0.00911594223570887));
#27774=CARTESIAN_POINT('Ctrl Pts',(-0.213078420142776,0.0122675494764246,
0.00918905359400996));
#27775=CARTESIAN_POINT('Ctrl Pts',(-0.213054987849986,0.0121122935736829,
0.00928101043997303));
#27776=CARTESIAN_POINT('Ctrl Pts',(-0.213028799864989,0.0119324471038202,
0.00938126321650623));
#27777=CARTESIAN_POINT('Ctrl Pts',(-0.213016132724809,0.0118440752678231,
0.00942931729501684));
#27778=CARTESIAN_POINT('Ctrl Pts',(-0.21299265415091,0.0116732229327397,
0.00951867247851693));
#27779=CARTESIAN_POINT('Ctrl Pts',(-0.212967912547534,0.0114808221189265,
0.00961383183775737));
#27780=CARTESIAN_POINT('Ctrl Pts',(-0.212941941715022,0.0112643974489121,
0.00971525592341462));
#27781=CARTESIAN_POINT('Ctrl Pts',(-0.212909723910377,0.0109415762419991,
0.00985240537371464));
#27782=CARTESIAN_POINT('Ctrl Pts',(-0.212881010751181,0.0105690751444958,
0.00999510672893007));
#27783=CARTESIAN_POINT('Ctrl Pts',(-0.212859850312569,0.0100382998289195,
0.0101685314876836));
#27784=CARTESIAN_POINT('Ctrl Pts',(-0.212862264629342,0.00954044254449958,
0.0102927030439336));
#27785=CARTESIAN_POINT('Ctrl Pts',(-0.212875146130418,0.00911578320726967,
0.0103772945146413));
#27786=CARTESIAN_POINT('Ctrl Pts',(-0.212892087627978,0.00877197251470777,
0.0104321046170394));
#27787=CARTESIAN_POINT('Ctrl Pts',(-0.21290752809911,0.00853543064909932,
0.0104615284810289));
#27788=CARTESIAN_POINT('Ctrl Pts',(-0.212923142391528,0.00832054440866613,
0.0104835679646797));
#27789=CARTESIAN_POINT('Ctrl Pts',(-0.21293837109707,0.00812810624263752,
0.0104989675440877));
#27790=CARTESIAN_POINT('Ctrl Pts',(-0.212947295077721,0.00802145374136446,
0.0105057380077258));
#27791=CARTESIAN_POINT('Ctrl Pts',(-0.212965075598067,0.00781377237991675,
0.0105165932490521));
#27792=CARTESIAN_POINT('Ctrl Pts',(-0.212981009563412,0.00763489019592171,
0.0105211941227256));
#27793=CARTESIAN_POINT('Ctrl Pts',(-0.212993233607984,0.00749979378001809,
0.0105214673239713));
#27794=CARTESIAN_POINT('',(-0.212877121847906,0.00590794924227077,0.0103793151952651));
#27795=CARTESIAN_POINT('Ctrl Pts',(-0.212993233832586,0.00749979129778757,
0.0105214673289907));
#27796=CARTESIAN_POINT('Ctrl Pts',(-0.212981064276903,0.00736479612297992,
0.0105211891819061));
#27797=CARTESIAN_POINT('Ctrl Pts',(-0.212965188112315,0.00718593222917332,
0.0105165874876166));
#27798=CARTESIAN_POINT('Ctrl Pts',(-0.212947440678806,0.00697802927922566,
0.0105057127229899));
#27799=CARTESIAN_POINT('Ctrl Pts',(-0.212938511600499,0.00687104507816289,
0.0104989140613425));
#27800=CARTESIAN_POINT('Ctrl Pts',(-0.212923279603605,0.00667828233926936,
0.010483467255871));
#27801=CARTESIAN_POINT('Ctrl Pts',(-0.212907633153483,0.00646298952442557,
0.0104613557234546));
#27802=CARTESIAN_POINT('Ctrl Pts',(-0.212892518991003,0.00623200226523625,
0.0104325693249221));
#27803=CARTESIAN_POINT('Ctrl Pts',(-0.212881462846515,0.00601154310194284,
0.0103975761963385));
#27804=CARTESIAN_POINT('Ctrl Pts',(-0.212877121847906,0.00590794924227077,
0.0103793151952651));
#27805=CARTESIAN_POINT('',(-0.212077933064703,0.00590974366334612,0.0103617691152544));
#27806=CARTESIAN_POINT('Ctrl Pts',(-0.212877121524224,0.00590794670319015,
0.0103793296663314));
#27807=CARTESIAN_POINT('Ctrl Pts',(-0.212077933064703,0.00590974366334613,
0.0103617691152544));
#27808=CARTESIAN_POINT('',(-0.212194330076657,0.00749995162518921,0.0105034114101302));
#27809=CARTESIAN_POINT('Ctrl Pts',(-0.212077933064703,0.00590974366334612,
0.0103617691152544));
#27810=CARTESIAN_POINT('Ctrl Pts',(-0.212082368745612,0.00601342674098364,
0.010380079592749));
#27811=CARTESIAN_POINT('Ctrl Pts',(-0.212087815760883,0.00612012877535262,
0.010396980289355));
#27812=CARTESIAN_POINT('Ctrl Pts',(-0.212093440442612,0.00621771619664684,
0.0104108738576259));
#27813=CARTESIAN_POINT('Ctrl Pts',(-0.212099476969926,0.00632244907977018,
0.0104257847287463));
#27814=CARTESIAN_POINT('Ctrl Pts',(-0.212105709360604,0.00641663519518074,
0.0104375997296922));
#27815=CARTESIAN_POINT('Ctrl Pts',(-0.212113022792179,0.0065197130300263,
0.0104488559154187));
#27816=CARTESIAN_POINT('Ctrl Pts',(-0.212116679507966,0.00657125194744908,
0.010454484008282));
#27817=CARTESIAN_POINT('Ctrl Pts',(-0.212120607255694,0.0066250154413234,
0.0104599382687491));
#27818=CARTESIAN_POINT('Ctrl Pts',(-0.212125117953049,0.00668407316279022,
0.0104653259590911));
#27819=CARTESIAN_POINT('Ctrl Pts',(-0.212129628650405,0.00674313088425705,
0.0104707136494332));
#27820=CARTESIAN_POINT('Ctrl Pts',(-0.212134725573122,0.0068074975565799,
0.0104758893432661));
#27821=CARTESIAN_POINT('Ctrl Pts',(-0.212138749104645,0.00685733713676164,
0.0104794930978266));
#27822=CARTESIAN_POINT('Ctrl Pts',(-0.212142772636168,0.00690717671694339,
0.0104830968523871));
#27823=CARTESIAN_POINT('Ctrl Pts',(-0.212145717600668,0.00694247322496747,
0.0104853580454887));
#27824=CARTESIAN_POINT('Ctrl Pts',(-0.212149400129846,0.00698607185520561,
0.0104878990841841));
#27825=CARTESIAN_POINT('Ctrl Pts',(-0.212153082659023,0.00702967048544376,
0.0104904401228795));
#27826=CARTESIAN_POINT('Ctrl Pts',(-0.212157505724507,0.0070815780620546,
0.0104931294137848));
#27827=CARTESIAN_POINT('Ctrl Pts',(-0.212162213970043,0.00713608398057281,
0.0104954127786815));
#27828=CARTESIAN_POINT('Ctrl Pts',(-0.212171630461117,0.00724509581760926,
0.0104999795084749));
#27829=CARTESIAN_POINT('Ctrl Pts',(-0.212182182843636,0.00736449674603688,
0.0105031361654474));
#27830=CARTESIAN_POINT('Ctrl Pts',(-0.212194330095429,0.0074999511942267,
0.0105034114311707));
#27831=CARTESIAN_POINT('',(-0.212297175950961,0.0123849010587109,0.00909973979562649));
#27832=CARTESIAN_POINT('Ctrl Pts',(-0.212194330056779,0.00749995162344025,
0.0105034114302995));
#27833=CARTESIAN_POINT('Ctrl Pts',(-0.212182132380261,0.00763540882905098,
0.0105031364739071));
#27834=CARTESIAN_POINT('Ctrl Pts',(-0.212171540637664,0.00775478092759007,
0.0104999805125386));
#27835=CARTESIAN_POINT('Ctrl Pts',(-0.212162092907394,0.00786375793232145,
0.0104954163568162));
#27836=CARTESIAN_POINT('Ctrl Pts',(-0.21215736903727,0.00791824649223841,
0.0104931342765446));
#27837=CARTESIAN_POINT('Ctrl Pts',(-0.212152932382641,0.00797013520137814,
0.0104904465348834));
#27838=CARTESIAN_POINT('Ctrl Pts',(-0.212149241231138,0.00801368798592748,
0.0104879090327744));
#27839=CARTESIAN_POINT('Ctrl Pts',(-0.212145550079636,0.0080572407704768,
0.0104853715306654));
#27840=CARTESIAN_POINT('Ctrl Pts',(-0.212142601449191,0.00809246447236669,
0.0104831163236127));
#27841=CARTESIAN_POINT('Ctrl Pts',(-0.212138567500056,0.0081423062165424,
0.0104795141318218));
#27842=CARTESIAN_POINT('Ctrl Pts',(-0.212134533550921,0.00819214796071812,
0.010475911940031));
#27843=CARTESIAN_POINT('Ctrl Pts',(-0.212129419483177,0.00825659171681023,
0.0104707323120953));
#27844=CARTESIAN_POINT('Ctrl Pts',(-0.212124898353902,0.00831570414042495,
0.0104653409394229));
#27845=CARTESIAN_POINT('Ctrl Pts',(-0.212120377224626,0.00837481656403967,
0.0104599495667504));
#27846=CARTESIAN_POINT('Ctrl Pts',(-0.212116445728773,0.00842861246583197,
0.0104544931741294));
#27847=CARTESIAN_POINT('Ctrl Pts',(-0.21211278424837,0.00848025913524566,
0.0104488535403145));
#27848=CARTESIAN_POINT('Ctrl Pts',(-0.212105461287565,0.00858355247407304,
0.0104375742726846));
#27849=CARTESIAN_POINT('Ctrl Pts',(-0.212099215586247,0.00867825431068825,
0.0104256859327208));
#27850=CARTESIAN_POINT('Ctrl Pts',(-0.212093221159177,0.00878282659072353,
0.0104107923438481));
#27851=CARTESIAN_POINT('Ctrl Pts',(-0.212087226732106,0.0088873988707588,
0.0103958987549755));
#27852=CARTESIAN_POINT('Ctrl Pts',(-0.212081491858564,0.00900179202119997,
0.0103776313788772));
#27853=CARTESIAN_POINT('Ctrl Pts',(-0.212076978987956,0.00911199897354088,
0.0103579020720291));
#27854=CARTESIAN_POINT('Ctrl Pts',(-0.212072466117349,0.00922220592588179,
0.0103381727651811));
#27855=CARTESIAN_POINT('Ctrl Pts',(-0.212069171050528,0.00932826550458844,
0.0103171699030088));
#27856=CARTESIAN_POINT('Ctrl Pts',(-0.212066791644702,0.00943199934212568,
0.0102948428129182));
#27857=CARTESIAN_POINT('Ctrl Pts',(-0.212062032833051,0.00963946701720017,
0.0102501886327371));
#27858=CARTESIAN_POINT('Ctrl Pts',(-0.212060929441922,0.00983766460797513,
0.0102005566356354));
#27859=CARTESIAN_POINT('Ctrl Pts',(-0.212064581442097,0.0100435201415751,
0.0101414775852836));
#27860=CARTESIAN_POINT('Ctrl Pts',(-0.212068233442271,0.0102493756751751,
0.0100823985349317));
#27861=CARTESIAN_POINT('Ctrl Pts',(-0.212076662975467,0.010462624545103,
0.0100128706935483));
#27862=CARTESIAN_POINT('Ctrl Pts',(-0.212089094170597,0.0106577554360329,
0.00994182361406666));
#27863=CARTESIAN_POINT('Ctrl Pts',(-0.212091761677008,0.0106996269453244,
0.0099265782142508));
#27864=CARTESIAN_POINT('Ctrl Pts',(-0.212094612320762,0.0107406751960078,
0.00991129437080939));
#27865=CARTESIAN_POINT('Ctrl Pts',(-0.212097710996392,0.0107818588971139,
0.00989562568130839));
#27866=CARTESIAN_POINT('Ctrl Pts',(-0.212101832592334,0.0108366379690795,
0.00987478451728645));
#27867=CARTESIAN_POINT('Ctrl Pts',(-0.212106393007951,0.0108916597408158,
0.00985326912746405));
#27868=CARTESIAN_POINT('Ctrl Pts',(-0.212111544956238,0.0109491208093745,
0.00983011378293056));
#27869=CARTESIAN_POINT('Ctrl Pts',(-0.212120570213998,0.0110497819429915,
0.0097895499144105));
#27870=CARTESIAN_POINT('Ctrl Pts',(-0.212131418571356,0.0111578178242854,
0.00974368193973834));
#27871=CARTESIAN_POINT('Ctrl Pts',(-0.212142039045027,0.0112547719580293,
0.00970048378486729));
#27872=CARTESIAN_POINT('Ctrl Pts',(-0.212152659518698,0.0113517260917732,
0.00965728562999623));
#27873=CARTESIAN_POINT('Ctrl Pts',(-0.212163043358788,0.0114377915105051,
0.00961717228658461));
#27874=CARTESIAN_POINT('Ctrl Pts',(-0.212174781369626,0.0115305319976495,
0.00957213117622237));
#27875=CARTESIAN_POINT('Ctrl Pts',(-0.212180650375044,0.0115769022412217,
0.00954961062104125));
#27876=CARTESIAN_POINT('Ctrl Pts',(-0.212186858479183,0.0116249251490129,
0.00952583071720044));
#27877=CARTESIAN_POINT('Ctrl Pts',(-0.212193904618974,0.0116775623276343,
0.00949909874670926));
#27878=CARTESIAN_POINT('Ctrl Pts',(-0.212200950758764,0.0117301995062557,
0.00947236677621809));
#27879=CARTESIAN_POINT('Ctrl Pts',(-0.212208837846504,0.0117873817604858,
0.00944254326647152));
#27880=CARTESIAN_POINT('Ctrl Pts',(-0.212214862593021,0.0118303815249037,
0.00941968588074516));
#27881=CARTESIAN_POINT('Ctrl Pts',(-0.212220887339537,0.0118733812893216,
0.0093968284950188));
#27882=CARTESIAN_POINT('Ctrl Pts',(-0.212225045352742,0.0119023127283524,
0.00938115035527493));
#27883=CARTESIAN_POINT('Ctrl Pts',(-0.212230400693812,0.0119392716659875,
0.00936086398329727));
#27884=CARTESIAN_POINT('Ctrl Pts',(-0.212235756034883,0.0119762306036225,
0.00934057761131961));
#27885=CARTESIAN_POINT('Ctrl Pts',(-0.212242311164843,0.0120211499898962,
0.00931556268835316));
#27886=CARTESIAN_POINT('Ctrl Pts',(-0.212249298978313,0.0120684169725973,
0.00928862110546898));
#27887=CARTESIAN_POINT('Ctrl Pts',(-0.2122632745675,0.0121629506826447,
0.00923473808524962));
#27888=CARTESIAN_POINT('Ctrl Pts',(-0.212278976851095,0.0122669943691938,
0.0091733484633276));
#27889=CARTESIAN_POINT('Ctrl Pts',(-0.212297175950961,0.0123849010587109,
0.00909973979562649));
#27890=CARTESIAN_POINT('',(-0.211094963303624,0.0123855555142644,0.00907540141503557));
#27891=CARTESIAN_POINT('',(-0.212297176216748,0.0123848982829031,0.00909973325119912));
#27892=CARTESIAN_POINT('',(-0.210993898514632,0.00749995658642614,0.010476280662273));
#27893=CARTESIAN_POINT('Ctrl Pts',(-0.211094961783628,0.0123855543264941,
0.00907539913122092));
#27894=CARTESIAN_POINT('Ctrl Pts',(-0.211076890136153,0.012268357395815,
0.00914837879912795));
#27895=CARTESIAN_POINT('Ctrl Pts',(-0.211053444315123,0.0121128461295332,
0.00924009652403312));
#27896=CARTESIAN_POINT('Ctrl Pts',(-0.211027274789818,0.0119329009254192,
0.0093399877574131));
#27897=CARTESIAN_POINT('Ctrl Pts',(-0.211014657068081,0.0118447643381785,
0.00938772124358589));
#27898=CARTESIAN_POINT('Ctrl Pts',(-0.21099119418584,0.0116736959797512,
0.00947683380478672));
#27899=CARTESIAN_POINT('Ctrl Pts',(-0.210966522628683,0.0114812428550573,
0.00957164908266));
#27900=CARTESIAN_POINT('Ctrl Pts',(-0.210940620910424,0.0112643612015598,
0.00967287560159098));
#27901=CARTESIAN_POINT('Ctrl Pts',(-0.210908819689275,0.0109427780958805,
0.00980901902062219));
#27902=CARTESIAN_POINT('Ctrl Pts',(-0.210880462883198,0.0105684325415033,
0.00995195000100696));
#27903=CARTESIAN_POINT('Ctrl Pts',(-0.210860078776075,0.0100383092010752,
0.0101244849284952));
#27904=CARTESIAN_POINT('Ctrl Pts',(-0.210862935637832,0.00954053436561135,
0.01024825280501));
#27905=CARTESIAN_POINT('Ctrl Pts',(-0.210876137375512,0.00911593919119299,
0.0103325648865413));
#27906=CARTESIAN_POINT('Ctrl Pts',(-0.210893328842,0.00877175418342708,
0.0103872508672743));
#27907=CARTESIAN_POINT('Ctrl Pts',(-0.210908796910629,0.00853585371980837,
0.0104165008407334));
#27908=CARTESIAN_POINT('Ctrl Pts',(-0.210924389683485,0.00832083102382324,
0.0104384918762313));
#27909=CARTESIAN_POINT('Ctrl Pts',(-0.210939545249769,0.00812824961765805,
0.0104538562101529));
#27910=CARTESIAN_POINT('Ctrl Pts',(-0.210948448409464,0.00802099004519663,
0.0104606402662976));
#27911=CARTESIAN_POINT('Ctrl Pts',(-0.21096608665718,0.00781318629174079,
0.0104714488432744));
#27912=CARTESIAN_POINT('Ctrl Pts',(-0.210981836917698,0.00763462031690367,
0.0104760087040924));
#27913=CARTESIAN_POINT('Ctrl Pts',(-0.210993898514632,0.00749995658642614,
0.010476280662273));
#27914=CARTESIAN_POINT('',(-0.210878462469796,0.00591244389125894,0.0103353945802353));
#27915=CARTESIAN_POINT('Ctrl Pts',(-0.210993898714441,0.00749995435564087,
0.0104762806667779));
#27916=CARTESIAN_POINT('Ctrl Pts',(-0.210981892668771,0.00736532351394722,
0.0104760086450893));
#27917=CARTESIAN_POINT('Ctrl Pts',(-0.210966203249496,0.00718669232467104,
0.0104714501353086));
#27918=CARTESIAN_POINT('Ctrl Pts',(-0.210948605953594,0.00697858674150669,
0.0104606209082496));
#27919=CARTESIAN_POINT('Ctrl Pts',(-0.210939703683893,0.00687096559900909,
0.0104538079458758));
#27920=CARTESIAN_POINT('Ctrl Pts',(-0.21092455816711,0.00667800085658727,
0.010438393086424));
#27921=CARTESIAN_POINT('Ctrl Pts',(-0.210908952138233,0.00646249488114474,
0.0104163222518967));
#27922=CARTESIAN_POINT('Ctrl Pts',(-0.210893929543052,0.00623342510638356,
0.0103878647232971));
#27923=CARTESIAN_POINT('Ctrl Pts',(-0.210882826575908,0.00601460089362695,
0.0103532881465335));
#27924=CARTESIAN_POINT('Ctrl Pts',(-0.210878462469796,0.00591244389125894,
0.0103353945802353));
#27925=CARTESIAN_POINT('',(-0.21007929998055,0.00591424122749678,0.0103178320466886));
#27926=CARTESIAN_POINT('Ctrl Pts',(-0.210878462054166,0.00591244065125743,
0.0103354131641705));
#27927=CARTESIAN_POINT('Ctrl Pts',(-0.210079299576428,0.00591423755299386,
0.0103178531839906));
#27928=CARTESIAN_POINT('',(-0.210194951358703,0.00750007523249054,0.0104582237667519));
#27929=CARTESIAN_POINT('Ctrl Pts',(-0.21007929998055,0.00591424122749678,
0.0103178320466886));
#27930=CARTESIAN_POINT('Ctrl Pts',(-0.210083751067343,0.00601645214670358,
0.0103356854655352));
#27931=CARTESIAN_POINT('Ctrl Pts',(-0.210095071594484,0.00623600174548137,
0.0103702841806485));
#27932=CARTESIAN_POINT('Ctrl Pts',(-0.210110128003962,0.00646332524691155,
0.010398431828706));
#27933=CARTESIAN_POINT('Ctrl Pts',(-0.210125776896694,0.00667853050594156,
0.0104204386569121));
#27934=CARTESIAN_POINT('Ctrl Pts',(-0.21014095902768,0.00687163015652102,
0.0104358281073399));
#27935=CARTESIAN_POINT('Ctrl Pts',(-0.21014977367735,0.00697823725658171,
0.010442563363362));
#27936=CARTESIAN_POINT('Ctrl Pts',(-0.21016731346144,0.0071860660981192,
0.0104533779643737));
#27937=CARTESIAN_POINT('Ctrl Pts',(-0.210182963205961,0.00736496853713723,
0.0104579539494083));
#27938=CARTESIAN_POINT('Ctrl Pts',(-0.210194951369192,0.00750007498543175,
0.0104582237809153));
#27939=CARTESIAN_POINT('',(-0.210295577942689,0.0123859825112166,0.00905923576391993));
#27940=CARTESIAN_POINT('Ctrl Pts',(-0.210194951347265,0.00750007523149893,
0.0104582237804177));
#27941=CARTESIAN_POINT('Ctrl Pts',(-0.210182907666862,0.00763523111115919,
0.010457950468014));
#27942=CARTESIAN_POINT('Ctrl Pts',(-0.210172431709479,0.00775451113746308,
0.0104548172251436));
#27943=CARTESIAN_POINT('Ctrl Pts',(-0.210163068965682,0.00786355077921227,
0.0104502697590671));
#27944=CARTESIAN_POINT('Ctrl Pts',(-0.210158387590943,0.00791807063317346,
0.010447996024649));
#27945=CARTESIAN_POINT('Ctrl Pts',(-0.210153985715518,0.00797002934151878,
0.0104453158402741));
#27946=CARTESIAN_POINT('Ctrl Pts',(-0.21015031426293,0.00801374514118166,
0.0104427776730748));
#27947=CARTESIAN_POINT('Ctrl Pts',(-0.210146642810342,0.00805746094084455,
0.0104402395058756));
#27948=CARTESIAN_POINT('Ctrl Pts',(-0.210143698823214,0.00809294059101559,
0.0104379743195514));
#27949=CARTESIAN_POINT('Ctrl Pts',(-0.210139683892845,0.0081429132131209,
0.0104343719254984));
#27950=CARTESIAN_POINT('Ctrl Pts',(-0.210135668962475,0.00819288583522622,
0.0104307695314454));
#27951=CARTESIAN_POINT('Ctrl Pts',(-0.210130588242887,0.00825733556983972,
0.0104256015122868));
#27952=CARTESIAN_POINT('Ctrl Pts',(-0.210126088751837,0.00831647279630859,
0.0104202212801215));
#27953=CARTESIAN_POINT('Ctrl Pts',(-0.210121589260786,0.00837561002277747,
0.0104148410479561));
#27954=CARTESIAN_POINT('Ctrl Pts',(-0.210117667730163,0.00842944937139556,
0.0104093936980803));
#27955=CARTESIAN_POINT('Ctrl Pts',(-0.210114012308968,0.00848109369784154,
0.0104037684374952));
#27956=CARTESIAN_POINT('Ctrl Pts',(-0.210106701466579,0.00858438235073352,
0.010392517916325));
#27957=CARTESIAN_POINT('Ctrl Pts',(-0.210100452137536,0.00867889688402659,
0.0103806850618465));
#27958=CARTESIAN_POINT('Ctrl Pts',(-0.210094415517649,0.00878350791480637,
0.0103658268947457));
#27959=CARTESIAN_POINT('Ctrl Pts',(-0.210088378897761,0.00888811894558615,
0.0103509687276449));
#27960=CARTESIAN_POINT('Ctrl Pts',(-0.210082563432376,0.00900277600701533,
0.0103327092752339));
#27961=CARTESIAN_POINT('Ctrl Pts',(-0.21007797133636,0.00911312815624517,
0.0103130047596318));
#27962=CARTESIAN_POINT('Ctrl Pts',(-0.210073379240344,0.00922348030547501,
0.0102933002440297));
#27963=CARTESIAN_POINT('Ctrl Pts',(-0.21007000621618,0.00932956712989777,
0.0102723434943911));
#27964=CARTESIAN_POINT('Ctrl Pts',(-0.210067544254891,0.00943326599643501,
0.0102500828349819));
#27965=CARTESIAN_POINT('Ctrl Pts',(-0.210062620332315,0.00964066372950947,
0.0102055615161635));
#27966=CARTESIAN_POINT('Ctrl Pts',(-0.210061333369762,0.00983854323490633,
0.0101561467361826));
#27967=CARTESIAN_POINT('Ctrl Pts',(-0.210064741391414,0.0100441652705734,
0.0100973199897705));
#27968=CARTESIAN_POINT('Ctrl Pts',(-0.210068149413066,0.0102497873062405,
0.0100384932433585));
#27969=CARTESIAN_POINT('Ctrl Pts',(-0.210076274349181,0.0104628899608491,
0.00996926186745797));
#27970=CARTESIAN_POINT('Ctrl Pts',(-0.210088469406629,0.0106584516234858,
0.00989829532363724));
#27971=CARTESIAN_POINT('Ctrl Pts',(-0.210090884318977,0.0106971774987838,
0.0098842422547009));
#27972=CARTESIAN_POINT('Ctrl Pts',(-0.210093457913029,0.0107352244438639,
0.00987014672261548));
#27973=CARTESIAN_POINT('Ctrl Pts',(-0.210096239220074,0.0107733155848942,
0.00985575027748959));
#27974=CARTESIAN_POINT('Ctrl Pts',(-0.210100480569403,0.0108314026039995,
0.00983379644359394));
#27975=CARTESIAN_POINT('Ctrl Pts',(-0.210105204948483,0.0108895968858756,
0.00981115310644442));
#27976=CARTESIAN_POINT('Ctrl Pts',(-0.210110586232912,0.010950395982138,
0.00978673331551824));
#27977=CARTESIAN_POINT('Ctrl Pts',(-0.210119496348177,0.0110510646910251,
0.00974630000359497));
#27978=CARTESIAN_POINT('Ctrl Pts',(-0.210130214863807,0.0111587657784774,
0.00970073002795545));
#27979=CARTESIAN_POINT('Ctrl Pts',(-0.210140752998032,0.0112556061415998,
0.00965773926679269));
#27980=CARTESIAN_POINT('Ctrl Pts',(-0.210151291132256,0.0113524465047223,
0.00961474850562993));
#27981=CARTESIAN_POINT('Ctrl Pts',(-0.210161640396964,0.011438612936933,
0.0095747400194307));
#27982=CARTESIAN_POINT('Ctrl Pts',(-0.210173341134653,0.0115313791441276,
0.00952985714870897));
#27983=CARTESIAN_POINT('Ctrl Pts',(-0.210179191503498,0.0115777622477249,
0.00950741571334811));
#27984=CARTESIAN_POINT('Ctrl Pts',(-0.210185380272374,0.0116257798470562,
0.00948372939897313));
#27985=CARTESIAN_POINT('Ctrl Pts',(-0.210192412741908,0.0116784375103859,
0.00945709044010566));
#27986=CARTESIAN_POINT('Ctrl Pts',(-0.210199445211442,0.0117310951737156,
0.00943045148123819));
#27987=CARTESIAN_POINT('Ctrl Pts',(-0.21020732429623,0.0117883237967492,
0.00940072009878417));
#27988=CARTESIAN_POINT('Ctrl Pts',(-0.210213336041793,0.0118313014592588,
0.00937796454941558));
#27989=CARTESIAN_POINT('Ctrl Pts',(-0.210219347787355,0.0118742791217684,
0.009355209000047));
#27990=CARTESIAN_POINT('Ctrl Pts',(-0.210223487807067,0.0119031195863775,
0.00933964247891056));
#27991=CARTESIAN_POINT('Ctrl Pts',(-0.210228830139808,0.01194003302514,
0.00931946325008595));
#27992=CARTESIAN_POINT('Ctrl Pts',(-0.210234172472549,0.0119769464639024,
0.00929928402126134));
#27993=CARTESIAN_POINT('Ctrl Pts',(-0.210240719573932,0.0120218661345205,
0.00927437182809841));
#27994=CARTESIAN_POINT('Ctrl Pts',(-0.210247701848314,0.0120691509098138,
0.00924753170250139));
#27995=CARTESIAN_POINT('Ctrl Pts',(-0.210261666357686,0.0121637201936272,
0.00919385160273513));
#27996=CARTESIAN_POINT('Ctrl Pts',(-0.210277367518394,0.0122678692136601,
0.00913266022226723));
#27997=CARTESIAN_POINT('Ctrl Pts',(-0.210295577942689,0.0123859825112166,
0.00905923576391993));
#27998=CARTESIAN_POINT('',(-0.209093386669321,0.0123867890340704,0.00903485594096656));
#27999=CARTESIAN_POINT('',(-0.210295578218103,0.0123859796930808,0.009059229030905));
#28000=CARTESIAN_POINT('',(-0.208994544866511,0.00750001217157779,0.0104310935790768));
#28001=CARTESIAN_POINT('Ctrl Pts',(-0.209093384956975,0.0123867878335644,
0.00903485357938685));
#28002=CARTESIAN_POINT('Ctrl Pts',(-0.209075271471196,0.0122692180496618,
0.00910775390628676));
#28003=CARTESIAN_POINT('Ctrl Pts',(-0.209051790486463,0.0121133375619839,
0.00919929174406344));
#28004=CARTESIAN_POINT('Ctrl Pts',(-0.209025620677105,0.0119331891109362,
0.00929886865408172));
#28005=CARTESIAN_POINT('Ctrl Pts',(-0.209013043216911,0.0118452328040021,
0.00934630625189574));
#28006=CARTESIAN_POINT('Ctrl Pts',(-0.20898959237479,0.0116739217040356,
0.00943517733250513));
#28007=CARTESIAN_POINT('Ctrl Pts',(-0.20896498827012,0.0114813739337843,
0.00952965577098411));
#28008=CARTESIAN_POINT('Ctrl Pts',(-0.20893915704693,0.0112639714210063,
0.00963069685261997));
#28009=CARTESIAN_POINT('Ctrl Pts',(-0.208907791001968,0.0109436242567375,
0.00976581223976034));
#28010=CARTESIAN_POINT('Ctrl Pts',(-0.208879845713628,0.0105675636138655,
0.00990890057783304));
#28011=CARTESIAN_POINT('Ctrl Pts',(-0.208860241917163,0.0100378203115335,
0.0100805840213093));
#28012=CARTESIAN_POINT('Ctrl Pts',(-0.20886359193908,0.00954120967817297,
0.0102036756318696));
#28013=CARTESIAN_POINT('Ctrl Pts',(-0.208877126664812,0.00911647469127787,
0.0102877839561455));
#28014=CARTESIAN_POINT('Ctrl Pts',(-0.208894583352245,0.00877121788909045,
0.0103424510565681));
#28015=CARTESIAN_POINT('Ctrl Pts',(-0.208910056796663,0.00853595851793098,
0.0103715120818308));
#28016=CARTESIAN_POINT('Ctrl Pts',(-0.208925617543613,0.00832081882800243,
0.0103934437827441));
#28017=CARTESIAN_POINT('Ctrl Pts',(-0.208940687467563,0.00812822373671741,
0.0104087564496012));
#28018=CARTESIAN_POINT('Ctrl Pts',(-0.208949569648136,0.00802036799570133,
0.0104155514242314));
#28019=CARTESIAN_POINT('Ctrl Pts',(-0.208967066582641,0.00781248286347796,
0.0104263073185167));
#28020=CARTESIAN_POINT('Ctrl Pts',(-0.208982639473909,0.0076342416541042,
0.0104308243299841));
#28021=CARTESIAN_POINT('Ctrl Pts',(-0.208994544866511,0.00750001217157779,
0.0104310935790768));
#28022=CARTESIAN_POINT('',(-0.208879854976475,0.00591693841052602,0.0102914751265115));
#28023=CARTESIAN_POINT('Ctrl Pts',(-0.208994545029769,0.00750001033091269,
0.0104310935827688));
#28024=CARTESIAN_POINT('Ctrl Pts',(-0.208982707573584,0.0073658755916226,
0.0104308261979098));
#28025=CARTESIAN_POINT('Ctrl Pts',(-0.20896721346356,0.00718766232772565,
0.0104263173020414));
#28026=CARTESIAN_POINT('Ctrl Pts',(-0.208949780090682,0.00697958258322114,
0.0104155541122085));
#28027=CARTESIAN_POINT('Ctrl Pts',(-0.20894091519731,0.00687147249956225,
0.0104087427206195));
#28028=CARTESIAN_POINT('Ctrl Pts',(-0.208925870776048,0.00667848686935303,
0.0103933897413847));
#28029=CARTESIAN_POINT('Ctrl Pts',(-0.208910320714726,0.0064628834835101,
0.0103713923556962));
#28030=CARTESIAN_POINT('Ctrl Pts',(-0.20889540134221,0.00623562335293567,
0.0103432779976701));
#28031=CARTESIAN_POINT('Ctrl Pts',(-0.208884244471473,0.00601792720410426,
0.0103090504550555));
#28032=CARTESIAN_POINT('Ctrl Pts',(-0.208879854976475,0.00591693841052602,
0.0102914751265115));
#28033=CARTESIAN_POINT('',(-0.208080872472194,0.00591873554374485,0.0102739153516223));
#28034=CARTESIAN_POINT('Ctrl Pts',(-0.208879854469394,0.00591693448266163,
0.0102914978020838));
#28035=CARTESIAN_POINT('Ctrl Pts',(-0.208080871978074,0.005918730979702,
0.0102739417767417));
#28036=CARTESIAN_POINT('',(-0.208195607365079,0.0075000238688742,0.0104130369087551));
#28037=CARTESIAN_POINT('Ctrl Pts',(-0.208080872472194,0.00591873554374485,
0.0102739153516223));
#28038=CARTESIAN_POINT('Ctrl Pts',(-0.208085329775637,0.00601949218603198,
0.0102914009897838));
#28039=CARTESIAN_POINT('Ctrl Pts',(-0.208096663114823,0.00623761016686182,
0.0103256168419561));
#28040=CARTESIAN_POINT('Ctrl Pts',(-0.208111573860928,0.00646304574628812,
0.010353430237953));
#28041=CARTESIAN_POINT('Ctrl Pts',(-0.20812714033341,0.00667838970390981,
0.0103753803244538));
#28042=CARTESIAN_POINT('Ctrl Pts',(-0.208142186770862,0.00687138867708767,
0.0103907122427205));
#28043=CARTESIAN_POINT('Ctrl Pts',(-0.208150968215157,0.00697867959623386,
0.0103974668961326));
#28044=CARTESIAN_POINT('Ctrl Pts',(-0.20816833676301,0.00718664995486033,
0.0104082341148987));
#28045=CARTESIAN_POINT('Ctrl Pts',(-0.208183789388884,0.00736530067962771,
0.0104127701685665));
#28046=CARTESIAN_POINT('Ctrl Pts',(-0.208195607372227,0.00750002370009737,
0.0104130369160257));
#28047=CARTESIAN_POINT('',(-0.208294260069062,0.0123873539202809,0.00901864499536075));
#28048=CARTESIAN_POINT('Ctrl Pts',(-0.208195607357402,0.00750002386821102,
0.0104130369156901));
#28049=CARTESIAN_POINT('Ctrl Pts',(-0.208183725521012,0.00763476041676933,
0.0104127680247592));
#28050=CARTESIAN_POINT('Ctrl Pts',(-0.208173372346303,0.00775385061720008,
0.0104096649778735));
#28051=CARTESIAN_POINT('Ctrl Pts',(-0.208164101441032,0.00786286797816972,
0.0104051436089863));
#28052=CARTESIAN_POINT('Ctrl Pts',(-0.208159465986469,0.00791737668132509,
0.0104028829236024));
#28053=CARTESIAN_POINT('Ctrl Pts',(-0.208155102276373,0.00796936615530415,
0.0104002155912398));
#28054=CARTESIAN_POINT('Ctrl Pts',(-0.208151453172895,0.00801321643662261,
0.0103976814114876));
#28055=CARTESIAN_POINT('Ctrl Pts',(-0.208147804069418,0.00805706671794107,
0.0103951472317354));
#28056=CARTESIAN_POINT('Ctrl Pts',(-0.208144866645942,0.00809278446206585,
0.0103928758074853));
#28057=CARTESIAN_POINT('Ctrl Pts',(-0.208140874703066,0.00814285080404548,
0.0103892798192253));
#28058=CARTESIAN_POINT('Ctrl Pts',(-0.20813688276019,0.00819291714602511,
0.0103856838309653));
#28059=CARTESIAN_POINT('Ctrl Pts',(-0.20813184139307,0.00825731645169599,
0.0103805374635568));
#28060=CARTESIAN_POINT('Ctrl Pts',(-0.20812736863174,0.00831644241587525,
0.0103751771930394));
#28061=CARTESIAN_POINT('Ctrl Pts',(-0.208122895870409,0.00837556838005451,
0.010369816922522));
#28062=CARTESIAN_POINT('Ctrl Pts',(-0.208118988493735,0.00842943539830661,
0.0103643857681925));
#28063=CARTESIAN_POINT('Ctrl Pts',(-0.208115343387974,0.0084810693505092,
0.010358781032824));
#28064=CARTESIAN_POINT('Ctrl Pts',(-0.208108053176452,0.00858433725491439,
0.0103475715620869));
#28065=CARTESIAN_POINT('Ctrl Pts',(-0.208101808983563,0.00867867946861084,
0.010335803318858));
#28066=CARTESIAN_POINT('Ctrl Pts',(-0.208095735383128,0.00878341828696095,
0.0103209780293898));
#28067=CARTESIAN_POINT('Ctrl Pts',(-0.208089661782693,0.00888815710531106,
0.0103061527399216));
#28068=CARTESIAN_POINT('Ctrl Pts',(-0.208083767437249,0.00900324089728844,
0.0102878847212649));
#28069=CARTESIAN_POINT('Ctrl Pts',(-0.20807909837359,0.00911384130045568,
0.0102681932846837));
#28070=CARTESIAN_POINT('Ctrl Pts',(-0.208074429309932,0.00922444170362292,
0.0102485018481024));
#28071=CARTESIAN_POINT('Ctrl Pts',(-0.208070981091356,0.00933059943503606,
0.0102275861108202));
#28072=CARTESIAN_POINT('Ctrl Pts',(-0.208068438597206,0.00943425036157439,
0.0102053993543059));
#28073=CARTESIAN_POINT('Ctrl Pts',(-0.208063353608906,0.00964155221465106,
0.0101610258412775));
#28074=CARTESIAN_POINT('Ctrl Pts',(-0.208061883982439,0.00983886264689967,
0.0101119014126196));
#28075=CARTESIAN_POINT('Ctrl Pts',(-0.208065050743897,0.0100441495251014,
0.010053375551578));
#28076=CARTESIAN_POINT('Ctrl Pts',(-0.208068217505355,0.0102494364033031,
0.00999484969053644));
#28077=CARTESIAN_POINT('Ctrl Pts',(-0.208076042548387,0.0104624381000747,
0.00992593082114766));
#28078=CARTESIAN_POINT('Ctrl Pts',(-0.208088010578668,0.0106586113426422,
0.00985499861608774));
#28079=CARTESIAN_POINT('Ctrl Pts',(-0.208090192295864,0.0106943728277592,
0.00984206799944312));
#28080=CARTESIAN_POINT('Ctrl Pts',(-0.208092510941534,0.0107295822993813,
0.00982909116751217));
#28081=CARTESIAN_POINT('Ctrl Pts',(-0.208095002750416,0.0107647732770846,
0.00981587956169499));
#28082=CARTESIAN_POINT('Ctrl Pts',(-0.208099345476324,0.0108261041326129,
0.00979285436772329));
#28083=CARTESIAN_POINT('Ctrl Pts',(-0.208104214160172,0.0108873846775921,
0.00976912991166498));
#28084=CARTESIAN_POINT('Ctrl Pts',(-0.208109800610626,0.0109513663728325,
0.00974352101739119));
#28085=CARTESIAN_POINT('Ctrl Pts',(-0.208118592505577,0.0110520600687654,
0.00970321801817414));
#28086=CARTESIAN_POINT('Ctrl Pts',(-0.208129169253644,0.0111593388284774,
0.00965798950224713));
#28087=CARTESIAN_POINT('Ctrl Pts',(-0.208139623820843,0.0112560665917109,
0.00961521305913846));
#28088=CARTESIAN_POINT('Ctrl Pts',(-0.208150078388041,0.0113527943549444,
0.00957243661602978));
#28089=CARTESIAN_POINT('Ctrl Pts',(-0.208160402620197,0.0114391501065935,
0.00953249992055839));
#28090=CARTESIAN_POINT('Ctrl Pts',(-0.208172074236449,0.0115320013768258,
0.00948775271911064));
#28091=CARTESIAN_POINT('Ctrl Pts',(-0.208177910044575,0.0115784270119419,
0.00946537911838677));
#28092=CARTESIAN_POINT('Ctrl Pts',(-0.20818408319898,0.0116264619118133,
0.0094417780872376));
#28093=CARTESIAN_POINT('Ctrl Pts',(-0.208191106905069,0.0116791675793703,
0.00941522122005211));
#28094=CARTESIAN_POINT('Ctrl Pts',(-0.208198130611159,0.0117318732469273,
0.00938866435286662));
#28095=CARTESIAN_POINT('Ctrl Pts',(-0.208206007790269,0.011789180565019,
0.00935901134666794));
#28096=CARTESIAN_POINT('Ctrl Pts',(-0.208212011214235,0.0118321593655242,
0.00933634716649299));
#28097=CARTESIAN_POINT('Ctrl Pts',(-0.208218014638201,0.0118751381660294,
0.00931368298631804));
#28098=CARTESIAN_POINT('Ctrl Pts',(-0.208222139920884,0.0119039019332434,
0.00929822114678945));
#28099=CARTESIAN_POINT('Ctrl Pts',(-0.208227473863976,0.0119407908460249,
0.00927813875387184));
#28100=CARTESIAN_POINT('Ctrl Pts',(-0.208232807807067,0.0119776797588065,
0.00925805636095424));
#28101=CARTESIAN_POINT('Ctrl Pts',(-0.208239352863477,0.0120226273113437,
0.00923323308531815));
#28102=CARTESIAN_POINT('Ctrl Pts',(-0.208246336249947,0.0120699600589816,
0.00920647857997257));
#28103=CARTESIAN_POINT('Ctrl Pts',(-0.208260302981663,0.0121646252748504,
0.00915296972721423));
#28104=CARTESIAN_POINT('Ctrl Pts',(-0.208276018986776,0.0122689504658964,
0.0090919370770759));
#28105=CARTESIAN_POINT('Ctrl Pts',(-0.208294260069062,0.0123873539202809,
0.00901864499536075));
#28106=CARTESIAN_POINT('',(-0.207092313768591,0.0123882174867341,0.00899428887323861));
#28107=CARTESIAN_POINT('',(-0.208294260353821,0.0123873510979057,0.00901863812336346));
#28108=CARTESIAN_POINT('',(-0.206995158242226,0.00749997779533629,0.0103859057504772));
#28109=CARTESIAN_POINT('Ctrl Pts',(-0.20709231184162,0.012388216289393,
0.00899428645318913));
#28110=CARTESIAN_POINT('Ctrl Pts',(-0.207074169755397,0.0122704302801191,
0.0090670078806541));
#28111=CARTESIAN_POINT('Ctrl Pts',(-0.207050668983289,0.0121143816651057,
0.00915825300058597));
#28112=CARTESIAN_POINT('Ctrl Pts',(-0.207024508217981,0.0119342143511166,
0.00925742631421442));
#28113=CARTESIAN_POINT('Ctrl Pts',(-0.207011976852465,0.0118465431096515,
0.0093045210258247));
#28114=CARTESIAN_POINT('Ctrl Pts',(-0.206988525025257,0.0116750185140633,
0.00939315137049461));
#28115=CARTESIAN_POINT('Ctrl Pts',(-0.206963979310437,0.0114824390834477,
0.00948728155437886));
#28116=CARTESIAN_POINT('Ctrl Pts',(-0.206938206287943,0.0112645547797643,
0.00958813968390749));
#28117=CARTESIAN_POINT('Ctrl Pts',(-0.206907269851096,0.0109455825524754,
0.00972221310561395));
#28118=CARTESIAN_POINT('Ctrl Pts',(-0.206879687420821,0.0105673434823094,
0.00986567451972152));
#28119=CARTESIAN_POINT('Ctrl Pts',(-0.206860821301113,0.0100376767561021,
0.0100366007334439));
#28120=CARTESIAN_POINT('Ctrl Pts',(-0.206864629141656,0.00954303962447637,
0.0101588564587864));
#28121=CARTESIAN_POINT('Ctrl Pts',(-0.206878437662789,0.00911790159733215,
0.0102428688551869));
#28122=CARTESIAN_POINT('Ctrl Pts',(-0.206896112137639,0.00877089042089746,
0.0102976375929108));
#28123=CARTESIAN_POINT('Ctrl Pts',(-0.206911523653191,0.00853624604372451,
0.0103265108082205));
#28124=CARTESIAN_POINT('Ctrl Pts',(-0.206926997316845,0.00832094260799099,
0.0103483888826665));
#28125=CARTESIAN_POINT('Ctrl Pts',(-0.20694192568622,0.00812840320520952,
0.0103636459186607));
#28126=CARTESIAN_POINT('Ctrl Pts',(-0.206950766774903,0.00801985265443885,
0.010370459281196));
#28127=CARTESIAN_POINT('Ctrl Pts',(-0.206968077025284,0.0078118100493795,
0.0103811661821285));
#28128=CARTESIAN_POINT('Ctrl Pts',(-0.206983436288678,0.00763382030278916,
0.010385641149766));
#28129=CARTESIAN_POINT('Ctrl Pts',(-0.206995158242226,0.00749997779533629,
0.0103859057504772));
#28130=CARTESIAN_POINT('',(-0.206881571004172,0.00592143254235674,0.0102475607510614));
#28131=CARTESIAN_POINT('Ctrl Pts',(-0.206995158364972,0.00749997639380803,
0.0103859057532479));
#28132=CARTESIAN_POINT('Ctrl Pts',(-0.206983492947492,0.00736607084721818,
0.0103856417602202));
#28133=CARTESIAN_POINT('Ctrl Pts',(-0.206968200812035,0.00718792179638615,
0.0103811634468022));
#28134=CARTESIAN_POINT('Ctrl Pts',(-0.20695095010466,0.00697952724386687,
0.0103704294756607));
#28135=CARTESIAN_POINT('Ctrl Pts',(-0.206942127827325,0.00687066431350494,
0.0103635889922793));
#28136=CARTESIAN_POINT('Ctrl Pts',(-0.20692723590354,0.00667768022036194,
0.0103482739306657));
#28137=CARTESIAN_POINT('Ctrl Pts',(-0.206911792379283,0.00646186189337934,
0.0103263096445771));
#28138=CARTESIAN_POINT('Ctrl Pts',(-0.20689707330291,0.00623681443106316,
0.0102985550840657));
#28139=CARTESIAN_POINT('Ctrl Pts',(-0.206885945076055,0.00602074128867715,
0.0102647305309386));
#28140=CARTESIAN_POINT('Ctrl Pts',(-0.206881571004172,0.00592143254235674,
0.0102475607510614));
#28141=CARTESIAN_POINT('',(-0.206082602390132,0.00592322960732982,0.0102300014544386));
#28142=CARTESIAN_POINT('Ctrl Pts',(-0.206881570360281,0.00592142758673692,
0.0102475895477209));
#28143=CARTESIAN_POINT('Ctrl Pts',(-0.206082601797357,0.00592322405245955,
0.0102300338284272));
#28144=CARTESIAN_POINT('',(-0.206196245004281,0.00749992072476384,0.0103678496348724));
#28145=CARTESIAN_POINT('Ctrl Pts',(-0.206082602390132,0.00592322960732983,
0.0102300014544386));
#28146=CARTESIAN_POINT('Ctrl Pts',(-0.206087053038459,0.00602255130965301,
0.0102471249980864));
#28147=CARTESIAN_POINT('Ctrl Pts',(-0.206098374242025,0.00623937330301455,
0.0102809786338258));
#28148=CARTESIAN_POINT('Ctrl Pts',(-0.206113102929825,0.00646287265370996,
0.0103084456160293));
#28149=CARTESIAN_POINT('Ctrl Pts',(-0.206128560594177,0.00667833597196627,
0.0103303329190581));
#28150=CARTESIAN_POINT('Ctrl Pts',(-0.206143447710207,0.00687116699017132,
0.0103455994805507));
#28151=CARTESIAN_POINT('Ctrl Pts',(-0.206152184530551,0.00697912187521234,
0.010352371501617));
#28152=CARTESIAN_POINT('Ctrl Pts',(-0.206169362913561,0.00718720041427173,
0.0103630888895013));
#28153=CARTESIAN_POINT('Ctrl Pts',(-0.206184605677713,0.00736558647702679,
0.010367585415964));
#28154=CARTESIAN_POINT('Ctrl Pts',(-0.206196245007266,0.00749992065302299,
0.010367849635414));
#28155=CARTESIAN_POINT('',(-0.206293181463369,0.0123888250109843,0.00897808768959864));
#28156=CARTESIAN_POINT('Ctrl Pts',(-0.206196245001035,0.0074999207244816,
0.0103678496352738));
#28157=CARTESIAN_POINT('Ctrl Pts',(-0.206184542529965,0.00763412632884294,
0.0103675863081985));
#28158=CARTESIAN_POINT('Ctrl Pts',(-0.2061692179339,0.00781233643911382,
0.0103630995604675));
#28159=CARTESIAN_POINT('Ctrl Pts',(-0.206151946738275,0.00802024236853892,
0.0103524012407256));
#28160=CARTESIAN_POINT('Ctrl Pts',(-0.206143167389231,0.00812804320649983,
0.0103456471072809));
#28161=CARTESIAN_POINT('Ctrl Pts',(-0.206128189094492,0.00832091762604645,
0.0103303904006423));
#28162=CARTESIAN_POINT('Ctrl Pts',(-0.206112648998793,0.008536396951546,
0.0103085230622252));
#28163=CARTESIAN_POINT('Ctrl Pts',(-0.206097072443987,0.00877190099198238,
0.0102795657449935));
#28164=CARTESIAN_POINT('Ctrl Pts',(-0.206079161137434,0.00911884914045566,
0.0102248371881941));
#28165=CARTESIAN_POINT('Ctrl Pts',(-0.206065089571356,0.00954381660755296,
0.0101409002075465));
#28166=CARTESIAN_POINT('Ctrl Pts',(-0.206060937605528,0.010035297153322,
0.010019686043107));
#28167=CARTESIAN_POINT('Ctrl Pts',(-0.206079738162382,0.0105675848158489,
0.00984827657715455));
#28168=CARTESIAN_POINT('Ctrl Pts',(-0.206107422248231,0.0109458329710147,
0.00970501723280112));
#28169=CARTESIAN_POINT('Ctrl Pts',(-0.206138686284396,0.011266165094612,
0.00957054361039449));
#28170=CARTESIAN_POINT('Ctrl Pts',(-0.206164458349906,0.0114825743096787,
0.00947049134904797));
#28171=CARTESIAN_POINT('Ctrl Pts',(-0.206189095067363,0.0116749698665059,
0.00937663021818898));
#28172=CARTESIAN_POINT('Ctrl Pts',(-0.206212738063899,0.0118471644912719,
0.0092877970955207));
#28173=CARTESIAN_POINT('Ctrl Pts',(-0.206225078944011,0.0119332236759434,
0.00924164612878725));
#28174=CARTESIAN_POINT('Ctrl Pts',(-0.206251270428428,0.0121132674835715,
0.00914276021107132));
#28175=CARTESIAN_POINT('Ctrl Pts',(-0.206274891330583,0.0122700535809347,
0.00905129095501176));
#28176=CARTESIAN_POINT('Ctrl Pts',(-0.206293181463369,0.0123888250109843,
0.00897808768959864));
#28177=CARTESIAN_POINT('',(-0.205091194491485,0.0123896885085703,0.00895378586049373));
#28178=CARTESIAN_POINT('',(-0.206293181757635,0.0123888222119803,0.00897808071050165));
#28179=CARTESIAN_POINT('',(-0.204995827543056,0.00749981733645938,0.0103407191840654));
#28180=CARTESIAN_POINT('Ctrl Pts',(-0.205091192354661,0.012389687321618,
0.00895378339447929));
#28181=CARTESIAN_POINT('Ctrl Pts',(-0.205073014821144,0.01227160358044,
0.00902637100980068));
#28182=CARTESIAN_POINT('Ctrl Pts',(-0.205049485910908,0.0121152792329455,
0.00911737677581394));
#28183=CARTESIAN_POINT('Ctrl Pts',(-0.205023328523559,0.0119349871360469,
0.00921619202382797));
#28184=CARTESIAN_POINT('Ctrl Pts',(-0.205010838477898,0.0118475323830429,
0.00926297457286685));
#28185=CARTESIAN_POINT('Ctrl Pts',(-0.204987393403255,0.0116757713626103,
0.00935136047384095));
#28186=CARTESIAN_POINT('Ctrl Pts',(-0.204962913930657,0.0114831266914915,
0.00944514341353462));
#28187=CARTESIAN_POINT('Ctrl Pts',(-0.20493720267966,0.0112646364096667,
0.0095458509373571));
#28188=CARTESIAN_POINT('Ctrl Pts',(-0.204906741670358,0.0109473007740114,
0.00967875276225383));
#28189=CARTESIAN_POINT('Ctrl Pts',(-0.204879520873365,0.0105666748706983,
0.00982263833066586));
#28190=CARTESIAN_POINT('Ctrl Pts',(-0.204861373406722,0.0100372093631709,
0.00999271941458411));
#28191=CARTESIAN_POINT('Ctrl Pts',(-0.204865624696935,0.00954478680686117,
0.0101140694872304));
#28192=CARTESIAN_POINT('Ctrl Pts',(-0.204879700592637,0.00911920611846394,
0.0101979851582911));
#28193=CARTESIAN_POINT('Ctrl Pts',(-0.204897588310666,0.00877029818710369,
0.0102528656904525));
#28194=CARTESIAN_POINT('Ctrl Pts',(-0.204912941251136,0.00853620075514094,
0.0102815493069361));
#28195=CARTESIAN_POINT('Ctrl Pts',(-0.204928337381059,0.00832076733418454,
0.0103033614244297));
#28196=CARTESIAN_POINT('Ctrl Pts',(-0.204943136754122,0.00812836001515498,
0.0103185508067787));
#28197=CARTESIAN_POINT('Ctrl Pts',(-0.204951944478282,0.00801917500798704,
0.0103253762389851));
#28198=CARTESIAN_POINT('Ctrl Pts',(-0.204969092080602,0.00781102280142051,
0.0103360285986065));
#28199=CARTESIAN_POINT('Ctrl Pts',(-0.204984265519491,0.00763328673646041,
0.0103404605227132));
#28200=CARTESIAN_POINT('Ctrl Pts',(-0.204995827543056,0.00749981733645938,
0.0103407191840654));
#28201=CARTESIAN_POINT('',(-0.204883316991064,0.00592592657070326,0.0102036471645642));
#28202=CARTESIAN_POINT('Ctrl Pts',(-0.204995827641741,0.0074998161972604,
0.0103407191862731));
#28203=CARTESIAN_POINT('Ctrl Pts',(-0.204984332499912,0.00736625211880565,
0.0103404567187726));
#28204=CARTESIAN_POINT('Ctrl Pts',(-0.20496924147999,0.00718832573187981,
0.0103360137909475));
#28205=CARTESIAN_POINT('Ctrl Pts',(-0.204952174630355,0.00697980517123724,
0.0103253251092728));
#28206=CARTESIAN_POINT('Ctrl Pts',(-0.204943399499021,0.00687032365940605,
0.0103184693400497));
#28207=CARTESIAN_POINT('Ctrl Pts',(-0.204928658370534,0.00667745245189651,
0.0103032129340482));
#28208=CARTESIAN_POINT('Ctrl Pts',(-0.204913320512947,0.00646149678877712,
0.0102813055099391));
#28209=CARTESIAN_POINT('Ctrl Pts',(-0.20489879336288,0.00623853473943785,
0.0102539134026724));
#28210=CARTESIAN_POINT('Ctrl Pts',(-0.204887680136377,0.00602375668886092,
0.0102204500366935));
#28211=CARTESIAN_POINT('Ctrl Pts',(-0.204883316991064,0.00592592657070326,
0.0102036471645642));
#28212=CARTESIAN_POINT('',(-0.204084593180221,0.00592771653709633,0.0101861316274437));
#28213=CARTESIAN_POINT('Ctrl Pts',(-0.204883316213314,0.00592592062344288,
0.0102036819517157));
#28214=CARTESIAN_POINT('Ctrl Pts',(-0.204084593180221,0.00592771653709633,
0.0101861316274437));
#28215=CARTESIAN_POINT('',(-0.204196825282865,0.00749983108742957,0.0103226610633396));
#28216=CARTESIAN_POINT('Ctrl Pts',(-0.204084593180221,0.00592771653709633,
0.0101861316274437));
#28217=CARTESIAN_POINT('Ctrl Pts',(-0.204088954952523,0.00602549703428869,
0.0102029698422185));
#28218=CARTESIAN_POINT('Ctrl Pts',(-0.204093930289245,0.00612296943935068,
0.0102181387928113));
#28219=CARTESIAN_POINT('Ctrl Pts',(-0.204099344857712,0.00621696792384513,
0.0102313459157465));
#28220=CARTESIAN_POINT('Ctrl Pts',(-0.204105493253929,0.00632370587167922,
0.0102463429788));
#28221=CARTESIAN_POINT('Ctrl Pts',(-0.204112201386035,0.00642595904684314,
0.0102589347405499));
#28222=CARTESIAN_POINT('Ctrl Pts',(-0.204119539651985,0.00653093717501485,
0.0102701117909915));
#28223=CARTESIAN_POINT('Ctrl Pts',(-0.204123208784961,0.0065834262391007,
0.0102757003162123));
#28224=CARTESIAN_POINT('Ctrl Pts',(-0.204127036788764,0.00663660201222637,
0.0102808758285888));
#28225=CARTESIAN_POINT('Ctrl Pts',(-0.204130483044463,0.00668325954882323,
0.0102850760016559));
#28226=CARTESIAN_POINT('Ctrl Pts',(-0.204133929300162,0.00672991708542009,
0.0102892761747229));
#28227=CARTESIAN_POINT('Ctrl Pts',(-0.204136991852014,0.00677004892262425,
0.0102925877734305));
#28228=CARTESIAN_POINT('Ctrl Pts',(-0.204140414174299,0.00681404637568421,
0.0102959292212381));
#28229=CARTESIAN_POINT('Ctrl Pts',(-0.204154103461852,0.00699003616755132,
0.0103092950109213));
#28230=CARTESIAN_POINT('Ctrl Pts',(-0.204173571820494,0.00722794042724961,
0.0103221305265275));
#28231=CARTESIAN_POINT('Ctrl Pts',(-0.204196825280084,0.00749983108767882,
0.0103226610574747));
#28232=CARTESIAN_POINT('',(-0.204292038138456,0.0123902600478229,0.00893764321216362));
#28233=CARTESIAN_POINT('Ctrl Pts',(-0.20419682528816,0.00749983118210175,
0.010322661057659));
#28234=CARTESIAN_POINT('Ctrl Pts',(-0.204185287994438,0.00763376309286183,
0.0103224027582973));
#28235=CARTESIAN_POINT('Ctrl Pts',(-0.204170161862589,0.00781178846879767,
0.0103179525824367));
#28236=CARTESIAN_POINT('Ctrl Pts',(-0.204153078342857,0.00801977906802176,
0.010307304969565));
#28237=CARTESIAN_POINT('Ctrl Pts',(-0.204144357953895,0.00812805074055648,
0.0103005481704218));
#28238=CARTESIAN_POINT('Ctrl Pts',(-0.204129530124552,0.00832083172535136,
0.0102853561683061));
#28239=CARTESIAN_POINT('Ctrl Pts',(-0.204114093058388,0.00853643222207643,
0.0102635538200186));
#28240=CARTESIAN_POINT('Ctrl Pts',(-0.2040986064084,0.0087713093979552,
0.0102347984868405));
#28241=CARTESIAN_POINT('Ctrl Pts',(-0.204080485546677,0.00912046100820518,
0.0101799103396762));
#28242=CARTESIAN_POINT('Ctrl Pts',(-0.204066152296679,0.00954600523903629,
0.0100960102926049));
#28243=CARTESIAN_POINT('Ctrl Pts',(-0.204061486979092,0.0100343873479205,
0.00997597456805669));
#28244=CARTESIAN_POINT('Ctrl Pts',(-0.204079650090975,0.0105680873423369,
0.00980479049483992));
#28245=CARTESIAN_POINT('Ctrl Pts',(-0.204106639710054,0.010945641344127,
0.00966233015414049));
#28246=CARTESIAN_POINT('Ctrl Pts',(-0.204137681642606,0.0112667974884081,
0.00952805592914953));
#28247=CARTESIAN_POINT('Ctrl Pts',(-0.20416333123174,0.0114831919246611,
0.00942840223806717));
#28248=CARTESIAN_POINT('Ctrl Pts',(-0.204187914714008,0.0116757242786425,
0.00933486309581412));
#28249=CARTESIAN_POINT('Ctrl Pts',(-0.204211557237231,0.0118481462689717,
0.00924628149172132));
#28250=CARTESIAN_POINT('Ctrl Pts',(-0.204223858296622,0.0119339725206118,
0.00920044954244206));
#28251=CARTESIAN_POINT('Ctrl Pts',(-0.204250052390331,0.0121141295177386,
0.00910193095114931));
#28252=CARTESIAN_POINT('Ctrl Pts',(-0.204273707494313,0.0122711889090159,
0.00901070810291783));
#28253=CARTESIAN_POINT('Ctrl Pts',(-0.204292038138456,0.0123902600478229,
0.00893764321216362));
#28254=CARTESIAN_POINT('',(-0.203101390374644,0.0123905784886725,0.00891395760438764));
#28255=CARTESIAN_POINT('',(-0.204292038444341,0.0123902572194587,0.00893763603478656));
#28256=CARTESIAN_POINT('',(-0.203011370131853,0.00751797523340815,0.0102940321261883));
#28257=CARTESIAN_POINT('Ctrl Pts',(-0.203013533411654,0.00751781230923161,
0.0102959004892027));
#28258=CARTESIAN_POINT('Ctrl Pts',(-0.202890705906049,0.00853201876615493,
0.0102911689991259));
#28259=CARTESIAN_POINT('Ctrl Pts',(-0.20286207477571,0.00939893234967562,
0.010121503230433));
#28260=CARTESIAN_POINT('Ctrl Pts',(-0.202882497840241,0.0109708227094279,
0.00967762743988251));
#28261=CARTESIAN_POINT('Ctrl Pts',(-0.202987079475644,0.0117485829910666,
0.00930640625159674));
#28262=CARTESIAN_POINT('Ctrl Pts',(-0.203101360711969,0.0123898923172725,
0.00891437384716674));
#28263=CARTESIAN_POINT('',(-0.202885099445385,0.00593040690138148,0.0101598141695237));
#28264=CARTESIAN_POINT('Ctrl Pts',(-0.202996526590838,0.0074995785670763,
0.0102955332839449));
#28265=CARTESIAN_POINT('Ctrl Pts',(-0.202973024640025,0.00722307829876791,
0.0102949895048917));
#28266=CARTESIAN_POINT('Ctrl Pts',(-0.202943193857677,0.00685288796118912,
0.010275686682386));
#28267=CARTESIAN_POINT('Ctrl Pts',(-0.202918430663541,0.0065100870074686,
0.0102417504832254));
#28268=CARTESIAN_POINT('Ctrl Pts',(-0.202906519367261,0.00632809932186647,
0.0102195321989363));
#28269=CARTESIAN_POINT('Ctrl Pts',(-0.202900436007646,0.0062299981588559,
0.0102066417983168));
#28270=CARTESIAN_POINT('Ctrl Pts',(-0.20289118428028,0.0060609044627119,
0.0101816418860839));
#28271=CARTESIAN_POINT('Ctrl Pts',(-0.202886766832153,0.00596786024350971,
0.0101662602137973));
#28272=CARTESIAN_POINT('Ctrl Pts',(-0.202885099445385,0.00593040690138148,
0.0101598141695237));
#28273=CARTESIAN_POINT('',(-0.202086848594906,0.00593220842806255,0.0101422352280257));
#28274=CARTESIAN_POINT('Ctrl Pts',(-0.202885100231941,0.00593041357433423,
0.0101597751943222));
#28275=CARTESIAN_POINT('Ctrl Pts',(-0.202086848594906,0.00593220842806255,
0.0101422352280257));
#28276=CARTESIAN_POINT('',(-0.20219754174379,0.00749953411020732,0.0102774755667304));
#28277=CARTESIAN_POINT('Ctrl Pts',(-0.202086848594906,0.00593220842806255,
0.0101422352280257));
#28278=CARTESIAN_POINT('Ctrl Pts',(-0.202088519117636,0.00596903688538452,
0.0101485364647982));
#28279=CARTESIAN_POINT('Ctrl Pts',(-0.202090324455866,0.00600648645140127,
0.0101547274732126));
#28280=CARTESIAN_POINT('Ctrl Pts',(-0.202092356858527,0.00604614439339113,
0.0101610181868496));
#28281=CARTESIAN_POINT('Ctrl Pts',(-0.202095367721964,0.00610489488108823,
0.0101703374423528));
#28282=CARTESIAN_POINT('Ctrl Pts',(-0.202098880399795,0.00616851443157102,
0.0101797365089284));
#28283=CARTESIAN_POINT('Ctrl Pts',(-0.202101645600268,0.00621650288703459,
0.0101864571866253));
#28284=CARTESIAN_POINT('Ctrl Pts',(-0.20210441080074,0.00626449134249817,
0.0101931778643221));
#28285=CARTESIAN_POINT('Ctrl Pts',(-0.202106423626697,0.00629681902919462,
0.0101974383451088));
#28286=CARTESIAN_POINT('Ctrl Pts',(-0.202108915349507,0.00633570339411839,
0.0102023833567655));
#28287=CARTESIAN_POINT('Ctrl Pts',(-0.202111407072318,0.00637458775904215,
0.0102073283684222));
#28288=CARTESIAN_POINT('Ctrl Pts',(-0.202114380321182,0.00642004285894188,
0.0102128409478528));
#28289=CARTESIAN_POINT('Ctrl Pts',(-0.202117532890599,0.00646663661792655,
0.0102181065813405));
#28290=CARTESIAN_POINT('Ctrl Pts',(-0.202123838029432,0.00655982413589589,
0.0102286378483159));
#28291=CARTESIAN_POINT('Ctrl Pts',(-0.202130857195231,0.00665755250225107,
0.0102383258202183));
#28292=CARTESIAN_POINT('Ctrl Pts',(-0.202138811348339,0.00676382059618203,
0.010246936229931));
#28293=CARTESIAN_POINT('Ctrl Pts',(-0.202154719654555,0.00697635678404395,
0.0102641570493565));
#28294=CARTESIAN_POINT('Ctrl Pts',(-0.202174370848536,0.00722305320371844,
0.0102769379360553));
#28295=CARTESIAN_POINT('Ctrl Pts',(-0.202197541766043,0.00749953388485717,
0.0102774755490777));
#28296=CARTESIAN_POINT('',(-0.202290696343322,0.0123919560860567,0.00889712716492088));
#28297=CARTESIAN_POINT('Ctrl Pts',(-0.20219754174698,0.0074995341104433,
0.0102774755486583));
#28298=CARTESIAN_POINT('Ctrl Pts',(-0.202174197410107,0.00777578331222019,
0.0102769618592336));
#28299=CARTESIAN_POINT('Ctrl Pts',(-0.202154396477338,0.00802226572456519,
0.0102642230991678));
#28300=CARTESIAN_POINT('Ctrl Pts',(-0.202138363651234,0.00823461651089539,
0.010247050000429));
#28301=CARTESIAN_POINT('Ctrl Pts',(-0.202130347236,0.00834079193296164,
0.0102384634487223));
#28302=CARTESIAN_POINT('Ctrl Pts',(-0.20212327211763,0.00843843476446932,
0.0102288005419976));
#28303=CARTESIAN_POINT('Ctrl Pts',(-0.202116915784324,0.00853153325630933,
0.0102182965579286));
#28304=CARTESIAN_POINT('Ctrl Pts',(-0.20211373761767,0.00857808250222934,
0.0102130445658941));
#28305=CARTESIAN_POINT('Ctrl Pts',(-0.20211073995827,0.00862349223463621,
0.0102075463081249));
#28306=CARTESIAN_POINT('Ctrl Pts',(-0.202108227148492,0.00866234475445357,
0.0102026130993859));
#28307=CARTESIAN_POINT('Ctrl Pts',(-0.202105714338715,0.00870119727427093,
0.0101976798906468));
#28308=CARTESIAN_POINT('Ctrl Pts',(-0.20210368375886,0.0087335065640619,
0.0101934282692858));
#28309=CARTESIAN_POINT('Ctrl Pts',(-0.202100895377743,0.00878143132743709,
0.0101867267582064));
#28310=CARTESIAN_POINT('Ctrl Pts',(-0.202098106996625,0.00882935609081229,
0.0101800252471269));
#28311=CARTESIAN_POINT('Ctrl Pts',(-0.202094565690218,0.0088928668284534,
0.0101706566026742));
#28312=CARTESIAN_POINT('Ctrl Pts',(-0.202091528815688,0.00895153035166877,
0.0101613655220642));
#28313=CARTESIAN_POINT('Ctrl Pts',(-0.202088491941158,0.00901019387488415,
0.0101520744414542));
#28314=CARTESIAN_POINT('Ctrl Pts',(-0.20208595602052,0.00906403531818589,
0.0101430163228177));
#28315=CARTESIAN_POINT('Ctrl Pts',(-0.202083619010167,0.00911818415598467,
0.0101334511154132));
#28316=CARTESIAN_POINT('Ctrl Pts',(-0.202078944989461,0.00922648183158223,
0.0101143207006041));
#28317=CARTESIAN_POINT('Ctrl Pts',(-0.202075070817907,0.00933597511595025,
0.0100929735403107));
#28318=CARTESIAN_POINT('Ctrl Pts',(-0.202072169668726,0.00944105319838383,
0.0100706352896346));
#28319=CARTESIAN_POINT('Ctrl Pts',(-0.202066367370365,0.009651209363251,
0.0100259587882825));
#28320=CARTESIAN_POINT('Ctrl Pts',(-0.202064438475617,0.00984387915731189,
0.00997815759471386));
#28321=CARTESIAN_POINT('Ctrl Pts',(-0.202066752064248,0.0100445919900524,
0.00992154314919459));
#28322=CARTESIAN_POINT('Ctrl Pts',(-0.202069065652879,0.0102453048227928,
0.00986492870367532));
#28323=CARTESIAN_POINT('Ctrl Pts',(-0.202075638665163,0.0104538251381158,
0.00979872593742554));
#28324=CARTESIAN_POINT('Ctrl Pts',(-0.202087420101427,0.0106597907467386,
0.00972506974541213));
#28325=CARTESIAN_POINT('Ctrl Pts',(-0.202088936142116,0.0106862944968907,
0.00971559163242359));
#28326=CARTESIAN_POINT('Ctrl Pts',(-0.202090538475574,0.0107127579251253,
0.0097059932895129));
#28327=CARTESIAN_POINT('Ctrl Pts',(-0.20209222178385,0.0107391503167258,
0.00969628591170712));
#28328=CARTESIAN_POINT('Ctrl Pts',(-0.202103619779601,0.0109178581455779,
0.0096305554376458));
#28329=CARTESIAN_POINT('Ctrl Pts',(-0.202118730388031,0.011093231614691,
0.00955965491820764));
#28330=CARTESIAN_POINT('Ctrl Pts',(-0.202135902640255,0.0112563083096395,
0.00948841915018892));
#28331=CARTESIAN_POINT('Ctrl Pts',(-0.202145756804842,0.0113498886141496,
0.00944754105374905));
#28332=CARTESIAN_POINT('Ctrl Pts',(-0.202156286377539,0.0114394851745847,
0.00940669911095104));
#28333=CARTESIAN_POINT('Ctrl Pts',(-0.202167967182874,0.0115333353934138,
0.00936203130577747));
#28334=CARTESIAN_POINT('Ctrl Pts',(-0.202173807585541,0.0115802605028284,
0.00933969740319068));
#28335=CARTESIAN_POINT('Ctrl Pts',(-0.202179935730716,0.011628248451796,
0.00931640956649808));
#28336=CARTESIAN_POINT('Ctrl Pts',(-0.202186965540118,0.011681172702445,
0.00929007516233768));
#28337=CARTESIAN_POINT('Ctrl Pts',(-0.202193995349519,0.0117340969530941,
0.00926374075817729));
#28338=CARTESIAN_POINT('Ctrl Pts',(-0.202201929887158,0.0117918850794239,
0.00923421185299353));
#28339=CARTESIAN_POINT('Ctrl Pts',(-0.202207941287984,0.0118349233812734,
0.00921180059453036));
#28340=CARTESIAN_POINT('Ctrl Pts',(-0.202213952688811,0.0118779616831228,
0.00918938933606718));
#28341=CARTESIAN_POINT('Ctrl Pts',(-0.202218036500617,0.0119063646643708,
0.00917431357946753));
#28342=CARTESIAN_POINT('Ctrl Pts',(-0.20222336517733,0.0119431275555664,
0.00915455707647552));
#28343=CARTESIAN_POINT('Ctrl Pts',(-0.202228693854044,0.0119798904467619,
0.00913480057348351));
#28344=CARTESIAN_POINT('Ctrl Pts',(-0.202235269863326,0.0120249468234503,
0.00911024162445137));
#28345=CARTESIAN_POINT('Ctrl Pts',(-0.202242299009262,0.0120724598365375,
0.00908373556252275));
#28346=CARTESIAN_POINT('Ctrl Pts',(-0.202256357261165,0.0121674855925353,
0.0090307235893888));
#28347=CARTESIAN_POINT('Ctrl Pts',(-0.202272223951729,0.0122724580287967,
0.0089701285643458));
#28348=CARTESIAN_POINT('Ctrl Pts',(-0.202290696343322,0.0123919560860567,
0.00889712716492088));
#28349=CARTESIAN_POINT('',(-0.20108848344321,0.0123927133101065,0.00887232988670267));
#28350=CARTESIAN_POINT('',(-0.202290696630135,0.0123919530714235,0.0088971199712788));
#28351=CARTESIAN_POINT('',(-0.200997245792689,0.00749926539693365,0.0102503478276375));
#28352=CARTESIAN_POINT('Ctrl Pts',(-0.201088482311616,0.0123930036514002,
0.00887281699432422));
#28353=CARTESIAN_POINT('Ctrl Pts',(-0.201070199293268,0.0122742486992986,
0.00894517069201058));
#28354=CARTESIAN_POINT('Ctrl Pts',(-0.201054452846893,0.0121695861583328,
0.00900546027918073));
#28355=CARTESIAN_POINT('Ctrl Pts',(-0.201040476460977,0.0120745671878803,
0.0090583506901546));
#28356=CARTESIAN_POINT('Ctrl Pts',(-0.201033488268019,0.012027057702654,
0.00908479589564153));
#28357=CARTESIAN_POINT('Ctrl Pts',(-0.201026943578741,0.0119819301252515,
0.00910934169276158));
#28358=CARTESIAN_POINT('Ctrl Pts',(-0.201021605938962,0.0119448472291696,
0.0091292248705987));
#28359=CARTESIAN_POINT('Ctrl Pts',(-0.201016268299182,0.0119077643330876,
0.00914910804843582));
#28360=CARTESIAN_POINT('Ctrl Pts',(-0.201012135299618,0.0118787909044927,
0.0091644475674369));
#28361=CARTESIAN_POINT('Ctrl Pts',(-0.201006157019148,0.0118356171761458,
0.00918687265224561));
#28362=CARTESIAN_POINT('Ctrl Pts',(-0.201000178738679,0.0117924434477989,
0.00920929773705432));
#28363=CARTESIAN_POINT('Ctrl Pts',(-0.200992359495022,0.0117349585664124,
0.00923859690537065));
#28364=CARTESIAN_POINT('Ctrl Pts',(-0.200985418410638,0.0116821788340252,
0.00926479726236227));
#28365=CARTESIAN_POINT('Ctrl Pts',(-0.200978477326255,0.011629399101638,
0.00929099761935389));
#28366=CARTESIAN_POINT('Ctrl Pts',(-0.200972411446029,0.0115813942784893,
0.00931424197335796));
#28367=CARTESIAN_POINT('Ctrl Pts',(-0.200966628185391,0.0115343884230262,
0.00933656306557079));
#28368=CARTESIAN_POINT('Ctrl Pts',(-0.200955061664114,0.0114403767121,0.00938120524999644));
#28369=CARTESIAN_POINT('Ctrl Pts',(-0.200944625932499,0.0113503615239781,
0.00942214177493506));
#28370=CARTESIAN_POINT('Ctrl Pts',(-0.200934892884681,0.011256626007776,
0.00946298870578385));
#28371=CARTESIAN_POINT('Ctrl Pts',(-0.200917744065162,0.0110914718361288,
0.00953495759550671));
#28372=CARTESIAN_POINT('Ctrl Pts',(-0.200902786406862,0.0109145834168858,
0.00960623035823801));
#28373=CARTESIAN_POINT('Ctrl Pts',(-0.200891567611251,0.010734025306428,
0.00967236522966423));
#28374=CARTESIAN_POINT('Ctrl Pts',(-0.200890051644097,0.0107096269508223,
0.0096813018656697));
#28375=CARTESIAN_POINT('Ctrl Pts',(-0.200888603946429,0.0106851628805553,
0.00969014751367443));
#28376=CARTESIAN_POINT('Ctrl Pts',(-0.200887228336966,0.0106606542815155,
0.00969889424409479));
#28377=CARTESIAN_POINT('Ctrl Pts',(-0.200875672637934,0.0104547717241602,
0.00977237046460479));
#28378=CARTESIAN_POINT('Ctrl Pts',(-0.200869202538282,0.0102456202057633,
0.00983864844216689));
#28379=CARTESIAN_POINT('Ctrl Pts',(-0.200866946989291,0.0100445494558891,
0.00989523320289807));
#28380=CARTESIAN_POINT('Ctrl Pts',(-0.2008646914403,0.00984347870601498,
0.00995181796362925));
#28381=CARTESIAN_POINT('Ctrl Pts',(-0.200866632893402,0.00965072981297347,
0.00999951216075563));
#28382=CARTESIAN_POINT('Ctrl Pts',(-0.200872404140185,0.00944057932809876,
0.0100440752795689));
#28383=CARTESIAN_POINT('Ctrl Pts',(-0.200875289763577,0.0093355040856614,
0.0100663568389755));
#28384=CARTESIAN_POINT('Ctrl Pts',(-0.200879137516127,0.00922603513339181,
0.0100876453128725));
#28385=CARTESIAN_POINT('Ctrl Pts',(-0.200883778490859,0.00911775499283436,
0.0101067242803535));
#28386=CARTESIAN_POINT('Ctrl Pts',(-0.200886098978226,0.00906361492255562,
0.0101162637640941));
#28387=CARTESIAN_POINT('Ctrl Pts',(-0.200888616732779,0.00900978039076347,
0.0101252973592866));
#28388=CARTESIAN_POINT('Ctrl Pts',(-0.200891627110003,0.00895118991645648,
0.0101345536484139));
#28389=CARTESIAN_POINT('Ctrl Pts',(-0.200894637487227,0.00889259944214949,
0.0101438099375413));
#28390=CARTESIAN_POINT('Ctrl Pts',(-0.200898143906586,0.00882922837542473,
0.0101531361237415));
#28391=CARTESIAN_POINT('Ctrl Pts',(-0.200900916691685,0.00878122412212321,
0.0101598324166721));
#28392=CARTESIAN_POINT('Ctrl Pts',(-0.200903689476784,0.00873321986882169,
0.0101665287096026));
#28393=CARTESIAN_POINT('Ctrl Pts',(-0.20090572382208,0.00870061144149407,
0.0101708092296612));
#28394=CARTESIAN_POINT('Ctrl Pts',(-0.20090823384213,0.00866155148029748,
0.010175754140507));
#28395=CARTESIAN_POINT('Ctrl Pts',(-0.20091074386218,0.00862249151910088,
0.0101806990513527));
#28396=CARTESIAN_POINT('Ctrl Pts',(-0.200913732147395,0.00857696623911426,
0.0101861931125867));
#28397=CARTESIAN_POINT('Ctrl Pts',(-0.200916900703198,0.00853031734238165,
0.0101914382865752));
#28398=CARTESIAN_POINT('Ctrl Pts',(-0.200923237814804,0.00843701954891641,
0.0102019286345521));
#28399=CARTESIAN_POINT('Ctrl Pts',(-0.200930292809032,0.00833924075920457,
0.0102115654584951));
#28400=CARTESIAN_POINT('Ctrl Pts',(-0.200938283557203,0.00823304991383771,
0.010220115993609));
#28401=CARTESIAN_POINT('Ctrl Pts',(-0.200954265053545,0.00802066822310398,
0.0102372170638366));
#28402=CARTESIAN_POINT('Ctrl Pts',(-0.200973992485866,0.00777463695403748,
0.0102498441003304));
#28403=CARTESIAN_POINT('Ctrl Pts',(-0.200997245792689,0.00749926539693342,
0.0102503478276375));
#28404=CARTESIAN_POINT('',(-0.200887345683122,0.0059348980442802,0.0101159223609127));
#28405=CARTESIAN_POINT('Ctrl Pts',(-0.200997245792689,0.00749926539693344,
0.0102503478276375));
#28406=CARTESIAN_POINT('Ctrl Pts',(-0.200974220810078,0.00722377349386874,
0.0102498056169339));
#28407=CARTESIAN_POINT('Ctrl Pts',(-0.20094492337546,0.00685451096840348,
0.0102306958255404));
#28408=CARTESIAN_POINT('Ctrl Pts',(-0.200920472411397,0.0065119382581388,
0.0101969879151918));
#28409=CARTESIAN_POINT('Ctrl Pts',(-0.200908641045106,0.00632963709598595,
0.0101748447830745));
#28410=CARTESIAN_POINT('Ctrl Pts',(-0.200902595650718,0.0062316418888999,
0.0101620407673395));
#28411=CARTESIAN_POINT('Ctrl Pts',(-0.20089337088145,0.0060629478196754,
0.010137205831809));
#28412=CARTESIAN_POINT('Ctrl Pts',(-0.200888966074273,0.00597085304664883,
0.010122068388625));
#28413=CARTESIAN_POINT('Ctrl Pts',(-0.200887345683122,0.0059348980442802,
0.0101159223609127));
#28414=CARTESIAN_POINT('',(-0.200088157086456,0.00593670244816755,0.0100983180218859));
#28415=CARTESIAN_POINT('Ctrl Pts',(-0.200887346564016,0.00593490548572253,
0.0101158785953323));
#28416=CARTESIAN_POINT('Ctrl Pts',(-0.200088157086456,0.00593670244816755,
0.0100983180218859));
#28417=CARTESIAN_POINT('',(-0.200198400286692,0.00749894756480746,0.0102322932334285));
#28418=CARTESIAN_POINT('Ctrl Pts',(-0.200088157086456,0.00593670244816755,
0.0100983180218859));
#28419=CARTESIAN_POINT('Ctrl Pts',(-0.20008976368105,0.00597187626689402,
0.0101042966301346));
#28420=CARTESIAN_POINT('Ctrl Pts',(-0.200091496143024,0.0060076832085402,
0.0101101856171118));
#28421=CARTESIAN_POINT('Ctrl Pts',(-0.200093434362444,0.00604550028339444,
0.0101161648357467));
#28422=CARTESIAN_POINT('Ctrl Pts',(-0.200096446784859,0.00610427639652141,
0.0101254578662693));
#28423=CARTESIAN_POINT('Ctrl Pts',(-0.200099959719856,0.00616793036557959,
0.0101348314515784));
#28424=CARTESIAN_POINT('Ctrl Pts',(-0.200102723819808,0.00621593654063874,
0.0101415327659766));
#28425=CARTESIAN_POINT('Ctrl Pts',(-0.200105487919759,0.00626394271569789,
0.0101482340803749));
#28426=CARTESIAN_POINT('Ctrl Pts',(-0.200107498298591,0.00629627158481284,
0.0101524808478668));
#28427=CARTESIAN_POINT('Ctrl Pts',(-0.200109986693639,0.00633516002956199,
0.010157410421101));
#28428=CARTESIAN_POINT('Ctrl Pts',(-0.200112475088687,0.00637404847431113,
0.0101623399943352));
#28429=CARTESIAN_POINT('Ctrl Pts',(-0.200115444122225,0.00641951046982536,
0.0101678357074836));
#28430=CARTESIAN_POINT('Ctrl Pts',(-0.200118591478095,0.00646610918157705,
0.0101730851224447));
#28431=CARTESIAN_POINT('Ctrl Pts',(-0.200124886189833,0.00655930660508041,
0.0101835839523668));
#28432=CARTESIAN_POINT('Ctrl Pts',(-0.200131890944902,0.00665703718747477,
0.0101932416757067));
#28433=CARTESIAN_POINT('Ctrl Pts',(-0.200139826778877,0.0067633028814333,
0.0102018259719556));
#28434=CARTESIAN_POINT('Ctrl Pts',(-0.200155698446825,0.00697583426935033,
0.0102189945644533));
#28435=CARTESIAN_POINT('Ctrl Pts',(-0.200175297369914,0.00722250745150977,
0.0102317397242931));
#28436=CARTESIAN_POINT('Ctrl Pts',(-0.200198400307928,0.00749894710515932,
0.0102322932135127));
#28437=CARTESIAN_POINT('',(-0.200288451010882,0.0123939123990367,0.00885652921296301));
#28438=CARTESIAN_POINT('Ctrl Pts',(-0.200198400269183,0.00749894756328928,
0.0102322932126889));
#28439=CARTESIAN_POINT('Ctrl Pts',(-0.200175034204682,0.00777522439535255,
0.0102317964311445));
#28440=CARTESIAN_POINT('Ctrl Pts',(-0.200155209703933,0.00802173299218074,
0.0102191166516208));
#28441=CARTESIAN_POINT('Ctrl Pts',(-0.200139151983605,0.00823411531667132,
0.0102020146145068));
#28442=CARTESIAN_POINT('Ctrl Pts',(-0.200131123119003,0.008340306537613,
0.0101934635912232));
#28443=CARTESIAN_POINT('Ctrl Pts',(-0.200124035223245,0.00843796649754914,
0.0101838390983458));
#28444=CARTESIAN_POINT('Ctrl Pts',(-0.200117665261195,0.00853107942461829,
0.01017337629834));
#28445=CARTESIAN_POINT('Ctrl Pts',(-0.200114480280169,0.00857763588815286,
0.0101681448983371));
#28446=CARTESIAN_POINT('Ctrl Pts',(-0.200111475589978,0.00862305219430565,
0.0101626680823682));
#28447=CARTESIAN_POINT('Ctrl Pts',(-0.200108956259927,0.0086619155983258,
0.0101577533046134));
#28448=CARTESIAN_POINT('Ctrl Pts',(-0.200106436929877,0.00870077900234596,
0.0101528385268586));
#28449=CARTESIAN_POINT('Ctrl Pts',(-0.200104400351822,0.00873310336940028,
0.0101486018214236));
#28450=CARTESIAN_POINT('Ctrl Pts',(-0.200101603498619,0.00878102716460599,
0.0101419270521032));
#28451=CARTESIAN_POINT('Ctrl Pts',(-0.200098806645416,0.00882895095981169,
0.0101352522827829));
#28452=CARTESIAN_POINT('Ctrl Pts',(-0.200095254369762,0.00889244493919518,
0.0101259232194401));
#28453=CARTESIAN_POINT('Ctrl Pts',(-0.200092205971828,0.00895109935058674,
0.010116670426863));
#28454=CARTESIAN_POINT('Ctrl Pts',(-0.200089157573894,0.0090097537619783,
0.0101074176342858));
#28455=CARTESIAN_POINT('Ctrl Pts',(-0.200086609593287,0.00906359351686766,
0.0100983957483952));
#28456=CARTESIAN_POINT('Ctrl Pts',(-0.200084259375412,0.00911774172770745,
0.010088868514949));
#28457=CARTESIAN_POINT('Ctrl Pts',(-0.200079558939661,0.00922603814938702,
0.0100698140480564));
#28458=CARTESIAN_POINT('Ctrl Pts',(-0.200075653739693,0.0093355347325092,
0.0100485508013927));
#28459=CARTESIAN_POINT('Ctrl Pts',(-0.200072718973702,0.00944063469604749,
0.010026295922952));
#28460=CARTESIAN_POINT('Ctrl Pts',(-0.200066849441721,0.00965083462312407,
0.00998178616607069));
#28461=CARTESIAN_POINT('Ctrl Pts',(-0.200064843100723,0.00984362058227625,
0.00993414342631784));
#28462=CARTESIAN_POINT('Ctrl Pts',(-0.200067049334776,0.0100444089630219,
0.00987772837450729));
#28463=CARTESIAN_POINT('Ctrl Pts',(-0.200069255568829,0.0102451973437676,
0.00982131332269675));
#28464=CARTESIAN_POINT('Ctrl Pts',(-0.200075691166784,0.010453755471825,
0.00975535739903431));
#28465=CARTESIAN_POINT('Ctrl Pts',(-0.200087297015736,0.0106597933730671,
0.00968196917157241));
#28466=CARTESIAN_POINT('Ctrl Pts',(-0.200088628878771,0.0106834378531548,
0.00967354729155693));
#28467=CARTESIAN_POINT('Ctrl Pts',(-0.200090028868672,0.0107070506993985,
0.00966503005969394));
#28468=CARTESIAN_POINT('Ctrl Pts',(-0.200091493264414,0.0107306101771093,
0.00965642531582548));
#28469=CARTESIAN_POINT('Ctrl Pts',(-0.20010278960708,0.0109123478902808,
0.0095900483573769));
#28470=CARTESIAN_POINT('Ctrl Pts',(-0.200117918466425,0.0110908281621165,
0.0095182815256283));
#28471=CARTESIAN_POINT('Ctrl Pts',(-0.200135171791351,0.011256666011491,
0.00944614031450078));
#28472=CARTESIAN_POINT('Ctrl Pts',(-0.200144916766895,0.0113503340895811,
0.00940539371399374));
#28473=CARTESIAN_POINT('Ctrl Pts',(-0.200155336031474,0.0114400347331477,
0.00936467528287738));
#28474=CARTESIAN_POINT('Ctrl Pts',(-0.200166896763449,0.0115339917398713,
0.00932014468728363));
#28475=CARTESIAN_POINT('Ctrl Pts',(-0.200172677129437,0.0115809702432331,
0.00929787938948676));
#28476=CARTESIAN_POINT('Ctrl Pts',(-0.200178742796055,0.0116290122849527,
0.00927466360579343));
#28477=CARTESIAN_POINT('Ctrl Pts',(-0.200185701217565,0.0116819926846841,
0.00924841301065489));
#28478=CARTESIAN_POINT('Ctrl Pts',(-0.200192659639076,0.0117349730844156,
0.00922216241551634));
#28479=CARTESIAN_POINT('Ctrl Pts',(-0.200200513864588,0.0117928199715147,
0.00919272958044644));
#28480=CARTESIAN_POINT('Ctrl Pts',(-0.200206466983726,0.0118359189361975,
0.00917038274469422));
#28481=CARTESIAN_POINT('Ctrl Pts',(-0.200212420102864,0.0118790179008803,
0.00914803590894199));
#28482=CARTESIAN_POINT('Ctrl Pts',(-0.200216467684153,0.0119074826106276,
0.00913299227818158));
#28483=CARTESIAN_POINT('Ctrl Pts',(-0.200221747414023,0.0119443129647354,
0.00911328442399996));
#28484=CARTESIAN_POINT('Ctrl Pts',(-0.200227027143894,0.0119811433188431,
0.00909357656981834));
#28485=CARTESIAN_POINT('Ctrl Pts',(-0.200233541479317,0.0120262733482081,
0.00906908309913212));
#28486=CARTESIAN_POINT('Ctrl Pts',(-0.200240504920934,0.012073865662999,
0.00904264723468476));
#28487=CARTESIAN_POINT('Ctrl Pts',(-0.200254431765176,0.0121690500260711,
0.00898977565382692));
#28488=CARTESIAN_POINT('Ctrl Pts',(-0.200270150944277,0.0122742028687716,
0.00892933943482924));
#28489=CARTESIAN_POINT('Ctrl Pts',(-0.200288451010882,0.0123939123990367,
0.00885652921296301));
#28490=CARTESIAN_POINT('',(-0.19908556181331,0.0123952967315942,0.00883206936057618));
#28491=CARTESIAN_POINT('',(-0.20028845129905,0.0123939092169457,0.00885652174964775));
#28492=CARTESIAN_POINT('',(-0.198998259704992,0.0074982742183944,0.0102051689206332));
#28493=CARTESIAN_POINT('Ctrl Pts',(-0.199085562115416,0.0123952939201688,
0.00883206023608842));
#28494=CARTESIAN_POINT('Ctrl Pts',(-0.199067470452782,0.0122762676185759,
0.00890426489238289));
#28495=CARTESIAN_POINT('Ctrl Pts',(-0.199051890543392,0.0121713830788781,
0.00896442147583353));
#28496=CARTESIAN_POINT('Ctrl Pts',(-0.199038064980175,0.0120761788114213,
0.0090171873028811));
#28497=CARTESIAN_POINT('Ctrl Pts',(-0.199031152179298,0.012028576545002,
0.00904357028994718));
#28498=CARTESIAN_POINT('Ctrl Pts',(-0.199024678952974,0.0119833655290427,
0.00906805600834903));
#28499=CARTESIAN_POINT('Ctrl Pts',(-0.199019399757912,0.0119462147288482,
0.00908789030800503));
#28500=CARTESIAN_POINT('Ctrl Pts',(-0.19901412056285,0.0119090639286538,
0.00910772460766103));
#28501=CARTESIAN_POINT('Ctrl Pts',(-0.19901003299821,0.0118800377414823,
0.00912302625132981));
#28502=CARTESIAN_POINT('Ctrl Pts',(-0.199004123482984,0.0118367997345112,
0.00914538891032673));
#28503=CARTESIAN_POINT('Ctrl Pts',(-0.198998213967757,0.0117935617275401,
0.00916775156932366));
#28504=CARTESIAN_POINT('Ctrl Pts',(-0.198990486803648,0.0117360017473575,
0.00919696418540885));
#28505=CARTESIAN_POINT('Ctrl Pts',(-0.198983628961391,0.0116831543854901,
0.00922308703443275));
#28506=CARTESIAN_POINT('Ctrl Pts',(-0.198976771119134,0.0116303070236227,
0.00924920988345665));
#28507=CARTESIAN_POINT('Ctrl Pts',(-0.198970779654378,0.0115822415967694,
0.00927238546542428));
#28508=CARTESIAN_POINT('Ctrl Pts',(-0.198965068227769,0.0115351728563396,
0.00929464241602615));
#28509=CARTESIAN_POINT('Ctrl Pts',(-0.198953645374551,0.01144103537548,
0.00933915631722987));
#28510=CARTESIAN_POINT('Ctrl Pts',(-0.198943343001692,0.0113508848199434,
0.00937998227748156));
#28511=CARTESIAN_POINT('Ctrl Pts',(-0.198933748124436,0.011257069527313,
0.00942069391882997));
#28512=CARTESIAN_POINT('Ctrl Pts',(-0.198916567779573,0.0110890862339493,
0.00949359115551921));
#28513=CARTESIAN_POINT('Ctrl Pts',(-0.198901665630765,0.0109091651201766,
0.00956569424943081));
#28514=CARTESIAN_POINT('Ctrl Pts',(-0.198890623754789,0.0107254842476422,
0.00963250034361427));
#28515=CARTESIAN_POINT('Ctrl Pts',(-0.198889332299217,0.0107040009700714,
0.00964031397083064));
#28516=CARTESIAN_POINT('Ctrl Pts',(-0.198888093650609,0.0106824672530659,
0.00964805732130372));
#28517=CARTESIAN_POINT('Ctrl Pts',(-0.198886910340231,0.0106608970216631,
0.00965572517693894));
#28518=CARTESIAN_POINT('Ctrl Pts',(-0.198875609789499,0.0104549024671198,
0.00972895278754657));
#28519=CARTESIAN_POINT('Ctrl Pts',(-0.198869355171845,0.0102454484024135,
0.00979506721264478));
#28520=CARTESIAN_POINT('Ctrl Pts',(-0.198867277759337,0.0100442901244564,
0.0098514531584819));
#28521=CARTESIAN_POINT('Ctrl Pts',(-0.198865200346828,0.00984313184649926,
0.00990783910431903));
#28522=CARTESIAN_POINT('Ctrl Pts',(-0.198867282268461,0.00965051324536303,
0.00995531424483447));
#28523=CARTESIAN_POINT('Ctrl Pts',(-0.198873165980298,0.00944032859203435,
0.00999971204990802));
#28524=CARTESIAN_POINT('Ctrl Pts',(-0.198876107836217,0.00933523626537001,
0.0100219109524448));
#28525=CARTESIAN_POINT('Ctrl Pts',(-0.19888000485948,0.0092257090094105,
0.0100431284145762));
#28526=CARTESIAN_POINT('Ctrl Pts',(-0.19888468657262,0.00911736588760557,
0.0100621429764505));
#28527=CARTESIAN_POINT('Ctrl Pts',(-0.198887027429189,0.0090631943267031,
0.0100716502573876));
#28528=CARTESIAN_POINT('Ctrl Pts',(-0.198889563419655,0.00900932709267297,
0.0100806533178575));
#28529=CARTESIAN_POINT('Ctrl Pts',(-0.19889259098924,0.00895069447560245,
0.0100898787764111));
#28530=CARTESIAN_POINT('Ctrl Pts',(-0.198895618558826,0.00889206185853193,
0.0100991042349646));
#28531=CARTESIAN_POINT('Ctrl Pts',(-0.198899141120948,0.00882863935187035,
0.0101083995418997));
#28532=CARTESIAN_POINT('Ctrl Pts',(-0.198901924819502,0.00878059702204565,
0.0101150730859184));
#28533=CARTESIAN_POINT('Ctrl Pts',(-0.198904708518055,0.00873255469222094,
0.0101217466299372));
#28534=CARTESIAN_POINT('Ctrl Pts',(-0.198906748557306,0.00869992137052802,
0.0101260121169608));
#28535=CARTESIAN_POINT('Ctrl Pts',(-0.198909264339861,0.00866083550968477,
0.010130938969545));
#28536=CARTESIAN_POINT('Ctrl Pts',(-0.198911780122415,0.00862174964884151,
0.0101358658221292));
#28537=CARTESIAN_POINT('Ctrl Pts',(-0.198914774232609,0.00857619755678408,
0.0101413390608318));
#28538=CARTESIAN_POINT('Ctrl Pts',(-0.198917947386027,0.00852952442602086,
0.0101465635597709));
#28539=CARTESIAN_POINT('Ctrl Pts',(-0.198924293692863,0.00843617816449441,
0.010157012557649));
#28540=CARTESIAN_POINT('Ctrl Pts',(-0.198931352981443,0.00833836111898063,
0.0101666082468319));
#28541=CARTESIAN_POINT('Ctrl Pts',(-0.198939344055784,0.00823214024472807,
0.0101751192122635));
#28542=CARTESIAN_POINT('Ctrl Pts',(-0.198955326204467,0.00801969849622294,
0.0101921411431267));
#28543=CARTESIAN_POINT('Ctrl Pts',(-0.198975038419768,0.00777364006771175,
0.010204695155617));
#28544=CARTESIAN_POINT('Ctrl Pts',(-0.198998259704992,0.00749827421839462,
0.0102051689206332));
#28545=CARTESIAN_POINT('',(-0.198888606651639,0.00593939180859995,0.0100720065732061));
#28546=CARTESIAN_POINT('Ctrl Pts',(-0.198998259704992,0.00749827421839462,
0.0102051689206332));
#28547=CARTESIAN_POINT('Ctrl Pts',(-0.198975256733037,0.00722282626960612,
0.0102045979631378));
#28548=CARTESIAN_POINT('Ctrl Pts',(-0.198945979827808,0.00685361694055798,
0.0101855256812312));
#28549=CARTESIAN_POINT('Ctrl Pts',(-0.198921532147383,0.00651107764630125,
0.0101519141152692));
#28550=CARTESIAN_POINT('Ctrl Pts',(-0.198909695399112,0.00632878155323742,
0.0101298367493766));
#28551=CARTESIAN_POINT('Ctrl Pts',(-0.198903646060906,0.0062308013688519,
0.0101170734658568));
#28552=CARTESIAN_POINT('Ctrl Pts',(-0.198894518754158,0.00606415358536155,
0.010092615312019));
#28553=CARTESIAN_POINT('Ctrl Pts',(-0.198890163386274,0.00597361763698084,
0.0100778157362859));
#28554=CARTESIAN_POINT('Ctrl Pts',(-0.198888606651639,0.00593939180859995,
0.0100720065732061));
#28555=CARTESIAN_POINT('',(-0.198089410867419,0.00594119659128827,0.0100543996135915));
#28556=CARTESIAN_POINT('Ctrl Pts',(-0.198888607579108,0.00593939961257745,
0.0100719603459932));
#28557=CARTESIAN_POINT('Ctrl Pts',(-0.198089410867419,0.00594119659128827,
0.0100543996135915));
#28558=CARTESIAN_POINT('',(-0.198199413892123,0.00749784490164266,0.0101871142630232));
#28559=CARTESIAN_POINT('Ctrl Pts',(-0.198089410867419,0.00594119659128827,
0.0100543996135915));
#28560=CARTESIAN_POINT('Ctrl Pts',(-0.198090952098397,0.0059746271363879,
0.0100600442196936));
#28561=CARTESIAN_POINT('Ctrl Pts',(-0.198092609970194,0.0060086916375095,
0.0100656179332038));
#28562=CARTESIAN_POINT('Ctrl Pts',(-0.198094452783454,0.00604456647828324,
0.0100712724478378));
#28563=CARTESIAN_POINT('Ctrl Pts',(-0.198097472408025,0.00610335081255558,
0.0100805379071742));
#28564=CARTESIAN_POINT('Ctrl Pts',(-0.198100992073415,0.00616701774472966,
0.0100898846297762));
#28565=CARTESIAN_POINT('Ctrl Pts',(-0.198103760284483,0.00621502726683673,
0.0100965660669984));
#28566=CARTESIAN_POINT('Ctrl Pts',(-0.19810652849555,0.00626303678894381,
0.0101032475042207));
#28567=CARTESIAN_POINT('Ctrl Pts',(-0.198108540381426,0.00629535956821877,
0.0101074807298124));
#28568=CARTESIAN_POINT('Ctrl Pts',(-0.198111030365065,0.00633424346512967,
0.0101123951528504));
#28569=CARTESIAN_POINT('Ctrl Pts',(-0.198113520348705,0.00637312736204057,
0.0101173095758883));
#28570=CARTESIAN_POINT('Ctrl Pts',(-0.198116491043605,0.0064185862647321,
0.0101227889096156));
#28571=CARTESIAN_POINT('Ctrl Pts',(-0.198119639481253,0.00646518065693026,
0.0101280228980885));
#28572=CARTESIAN_POINT('Ctrl Pts',(-0.198125936356551,0.00655836944132657,
0.0101384908750344));
#28573=CARTESIAN_POINT('Ctrl Pts',(-0.198132940968095,0.00665608656171364,
0.010148121066479));
#28574=CARTESIAN_POINT('Ctrl Pts',(-0.198140874820444,0.00676233559324092,
0.010156683054696));
#28575=CARTESIAN_POINT('Ctrl Pts',(-0.198156742525141,0.00697483365629548,
0.0101738070311301));
#28576=CARTESIAN_POINT('Ctrl Pts',(-0.198176330129256,0.0072214607371163,
0.0101865286206563));
#28577=CARTESIAN_POINT('Ctrl Pts',(-0.198199413926082,0.00749784439333545,
0.010187114241221));
#28578=CARTESIAN_POINT('',(-0.198286007594511,0.0123960164106601,0.00881593489558765));
#28579=CARTESIAN_POINT('Ctrl Pts',(-0.198199413883263,0.00749784490085718,
0.0101871142403706));
#28580=CARTESIAN_POINT('Ctrl Pts',(-0.198176103477868,0.00777413486843259,
0.0101866512761317));
#28581=CARTESIAN_POINT('Ctrl Pts',(-0.198156318254055,0.00802067698994559,
0.0101740470863644));
#28582=CARTESIAN_POINT('Ctrl Pts',(-0.19814028359857,0.00823311616486342,
0.0101570274772293));
#28583=CARTESIAN_POINT('Ctrl Pts',(-0.198132266265918,0.00833933581736117,
0.0101485176674511));
#28584=CARTESIAN_POINT('Ctrl Pts',(-0.198125185849937,0.00843703003828308,
0.0101389360636091));
#28585=CARTESIAN_POINT('Ctrl Pts',(-0.198118819143145,0.00853018215640962,
0.0101285171408901));
#28586=CARTESIAN_POINT('Ctrl Pts',(-0.198115635789749,0.00857675821547287,
0.0101233076795306));
#28587=CARTESIAN_POINT('Ctrl Pts',(-0.198112631668245,0.00862219537792419,
0.0101178531725202));
#28588=CARTESIAN_POINT('Ctrl Pts',(-0.198110112092516,0.00866108138839014,
0.0101129574980669));
#28589=CARTESIAN_POINT('Ctrl Pts',(-0.198107592516787,0.00869996739885609,
0.0101080618236135));
#28590=CARTESIAN_POINT('Ctrl Pts',(-0.198105554887214,0.00873231601502186,
0.0101038406457708));
#28591=CARTESIAN_POINT('Ctrl Pts',(-0.198102755159942,0.0087802636455589,
0.0100971915835399));
#28592=CARTESIAN_POINT('Ctrl Pts',(-0.19809995543267,0.00882821127609593,
0.010090542521309));
#28593=CARTESIAN_POINT('Ctrl Pts',(-0.19809639844434,0.00889172889943068,
0.0100812500372814));
#28594=CARTESIAN_POINT('Ctrl Pts',(-0.198093343481625,0.00895040621919025,
0.0100720328458692));
#28595=CARTESIAN_POINT('Ctrl Pts',(-0.198090288518909,0.00900908353894982,
0.0100628156544569));
#28596=CARTESIAN_POINT('Ctrl Pts',(-0.198087732132926,0.00906294528084993,
0.0100538279006226));
#28597=CARTESIAN_POINT('Ctrl Pts',(-0.198085371573665,0.00911711565823163,
0.0100443363717712));
#28598=CARTESIAN_POINT('Ctrl Pts',(-0.198080650455144,0.00922545641299502,
0.0100253533140684));
#28599=CARTESIAN_POINT('Ctrl Pts',(-0.198076716817448,0.0093349982870547,
0.0100041682240223));
#28600=CARTESIAN_POINT('Ctrl Pts',(-0.198073747068821,0.00944013375262981,
0.0099819961171781));
#28601=CARTESIAN_POINT('Ctrl Pts',(-0.198067807571566,0.00965040468378001,
0.00993765190348967));
#28602=CARTESIAN_POINT('Ctrl Pts',(-0.198065705080381,0.00984322172765309,
0.00989019358358982));
#28603=CARTESIAN_POINT('Ctrl Pts',(-0.198067775303428,0.0100441274792667,
0.00983397148392325));
#28604=CARTESIAN_POINT('Ctrl Pts',(-0.198069845526475,0.0102450332308803,
0.00977774938425667));
#28605=CARTESIAN_POINT('Ctrl Pts',(-0.198076105322089,0.0104537951798029,
0.00971199140777644));
#28606=CARTESIAN_POINT('Ctrl Pts',(-0.198087491404007,0.0106599840281665,
0.00963884205248109));
#28607=CARTESIAN_POINT('Ctrl Pts',(-0.198088635894388,0.0106807094326789,
0.00963148932710166));
#28608=CARTESIAN_POINT('Ctrl Pts',(-0.198089832205802,0.0107014100382362,
0.00962406390124972));
#28609=CARTESIAN_POINT('Ctrl Pts',(-0.198091077878136,0.0107220713741063,
0.00961657095850853));
#28610=CARTESIAN_POINT('Ctrl Pts',(-0.198102224906933,0.0109069614930296,
0.00954951957890682));
#28611=CARTESIAN_POINT('Ctrl Pts',(-0.198117324635717,0.0110886212795307,
0.00947686846080482));
#28612=CARTESIAN_POINT('Ctrl Pts',(-0.198134614191499,0.0112572894281296,
0.00940379951023843));
#28613=CARTESIAN_POINT('Ctrl Pts',(-0.198144225017011,0.011351047773691,
0.00936318233400258));
#28614=CARTESIAN_POINT('Ctrl Pts',(-0.198154509073741,0.0114408574485988,
0.00932258431859022));
#28615=CARTESIAN_POINT('Ctrl Pts',(-0.19816592275737,0.0115349254228497,
0.00927818801413299));
#28616=CARTESIAN_POINT('Ctrl Pts',(-0.198171629599184,0.0115819594099751,
0.00925598986190438));
#28617=CARTESIAN_POINT('Ctrl Pts',(-0.198177618780531,0.0116300574555616,
0.00923284473727326));
#28618=CARTESIAN_POINT('Ctrl Pts',(-0.198184490318301,0.0116830979811874,
0.00920667541869562));
#28619=CARTESIAN_POINT('Ctrl Pts',(-0.198191361856072,0.0117361385068132,
0.00918050610011798));
#28620=CARTESIAN_POINT('Ctrl Pts',(-0.198199118785794,0.0117940501595618,
0.00915116559653516));
#28621=CARTESIAN_POINT('Ctrl Pts',(-0.198205000064564,0.0118372091942293,
0.00912888306599363));
#28622=CARTESIAN_POINT('Ctrl Pts',(-0.198210881343333,0.0118803682288967,
0.00910660053545211));
#28623=CARTESIAN_POINT('Ctrl Pts',(-0.198214882559401,0.0119088875112645,
0.00909159258929125));
#28624=CARTESIAN_POINT('Ctrl Pts',(-0.198220100259032,0.0119457768970234,
0.00907193770317756));
#28625=CARTESIAN_POINT('Ctrl Pts',(-0.198225317958663,0.0119826662827822,
0.00905228281706388));
#28626=CARTESIAN_POINT('Ctrl Pts',(-0.198231754588115,0.0120278602541438,
0.00902785990193314));
#28627=CARTESIAN_POINT('Ctrl Pts',(-0.198238634937554,0.0120755196795865,
0.0090015009955941));
#28628=CARTESIAN_POINT('Ctrl Pts',(-0.198252395597808,0.0121708382629281,
0.00894878333088588));
#28629=CARTESIAN_POINT('Ctrl Pts',(-0.198267927067132,0.0122761371757607,
0.00888852612430001));
#28630=CARTESIAN_POINT('Ctrl Pts',(-0.198286007594511,0.0123960164106601,
0.00881593489558765));
#28631=CARTESIAN_POINT('',(-0.197086979519691,0.0123971201193948,0.00879177325798805));
#28632=CARTESIAN_POINT('',(-0.198286007879611,0.0123960132910725,0.00881592749813436));
#28633=CARTESIAN_POINT('',(-0.196999270591198,0.00749728421803852,0.010159989841476));
#28634=CARTESIAN_POINT('Ctrl Pts',(-0.197086976737809,0.0123971189185158,
0.00879177056663458));
#28635=CARTESIAN_POINT('Ctrl Pts',(-0.197068794899013,0.0122778890515698,
0.00886376427758092));
#28636=CARTESIAN_POINT('Ctrl Pts',(-0.197045310518113,0.0121203981355003,
0.00895382276837131));
#28637=CARTESIAN_POINT('Ctrl Pts',(-0.19701930346749,0.0119393127272318,
0.00905133624140467));
#28638=CARTESIAN_POINT('Ctrl Pts',(-0.197006993671684,0.0118522429931005,
0.0090971191097409));
#28639=CARTESIAN_POINT('Ctrl Pts',(-0.19698370828621,0.0116794024840158,
0.00918453494617847));
#28640=CARTESIAN_POINT('Ctrl Pts',(-0.196959653037427,0.011486887794521,
0.00927674502930554));
#28641=CARTESIAN_POINT('Ctrl Pts',(-0.196923454455795,0.0111710535502845,
0.00941943933573583));
#28642=CARTESIAN_POINT('Ctrl Pts',(-0.196882607614813,0.0106654311014493,
0.00961961998668078));
#28643=CARTESIAN_POINT('Ctrl Pts',(-0.196864002095244,0.0100351435763335,
0.0098170164219494));
#28644=CARTESIAN_POINT('Ctrl Pts',(-0.196869375982058,0.00955457285278419,
0.00993489875212199));
#28645=CARTESIAN_POINT('Ctrl Pts',(-0.196883083155349,0.00917085742961943,
0.0100090632638723));
#28646=CARTESIAN_POINT('Ctrl Pts',(-0.196893255927463,0.00895513606961216,
0.010045064644907));
#28647=CARTESIAN_POINT('Ctrl Pts',(-0.196903850141088,0.00876446023912426,
0.0100728505475419));
#28648=CARTESIAN_POINT('Ctrl Pts',(-0.196909966763981,0.00866656949678343,
0.010085504284038));
#28649=CARTESIAN_POINT('Ctrl Pts',(-0.196921934611565,0.00848426778298676,
0.0101074108318155));
#28650=CARTESIAN_POINT('Ctrl Pts',(-0.19694660867882,0.00814179776041215,
0.0101407229405312));
#28651=CARTESIAN_POINT('Ctrl Pts',(-0.196976109231857,0.00777266281110438,
0.0101595464069006));
#28652=CARTESIAN_POINT('Ctrl Pts',(-0.196999270591198,0.00749728421803852,
0.010159989841476));
#28653=CARTESIAN_POINT('',(-0.196889861047832,0.00594388566779889,0.0100280902017948));
#28654=CARTESIAN_POINT('Ctrl Pts',(-0.196999270581664,0.00749728410378425,
0.0101599898412273));
#28655=CARTESIAN_POINT('Ctrl Pts',(-0.196976289970089,0.00722188673154521,
0.0101593904194489));
#28656=CARTESIAN_POINT('Ctrl Pts',(-0.196947033468888,0.00685273767299148,
0.0101403579352097));
#28657=CARTESIAN_POINT('Ctrl Pts',(-0.196922587915481,0.00651023541354164,
0.0101068459602804));
#28658=CARTESIAN_POINT('Ctrl Pts',(-0.196910744693017,0.00632794452775094,
0.0100848361630135));
#28659=CARTESIAN_POINT('Ctrl Pts',(-0.196904690767546,0.00622998027451274,
0.0100721147663665));
#28660=CARTESIAN_POINT('Ctrl Pts',(-0.196895659032348,0.00606536557185553,
0.0100480314473845));
#28661=CARTESIAN_POINT('Ctrl Pts',(-0.19689135334592,0.00597639027351646,
0.010033567696482));
#28662=CARTESIAN_POINT('Ctrl Pts',(-0.196889861047832,0.00594388566779889,
0.0100280902017948));
#28663=CARTESIAN_POINT('',(-0.196090558152439,0.0059456909738631,0.0100104788652639));
#28664=CARTESIAN_POINT('Ctrl Pts',(-0.196889862013759,0.00594389375422837,
0.0100280419520622));
#28665=CARTESIAN_POINT('Ctrl Pts',(-0.196090558152439,0.00594569097386311,
0.0100104788652639));
#28666=CARTESIAN_POINT('',(-0.196200534255837,0.00749682943752911,0.0101419375996538));
#28667=CARTESIAN_POINT('Ctrl Pts',(-0.196090558152439,0.0059456909738631,
0.0100104788652639));
#28668=CARTESIAN_POINT('Ctrl Pts',(-0.196092036966744,0.00597743019073511,
0.0100158019567583));
#28669=CARTESIAN_POINT('Ctrl Pts',(-0.196093623627043,0.00600979364775697,
0.0100210696180627));
#28670=CARTESIAN_POINT('Ctrl Pts',(-0.19609537642288,0.00604378231372989,
0.0100264093026737));
#28671=CARTESIAN_POINT('Ctrl Pts',(-0.196098407576924,0.00610255977097751,
0.0100356433539364));
#28672=CARTESIAN_POINT('Ctrl Pts',(-0.196101939030964,0.00616621904611668,
0.0100449588622492));
#28673=CARTESIAN_POINT('Ctrl Pts',(-0.196104715665148,0.00621422025408268,
0.0100516179388472));
#28674=CARTESIAN_POINT('Ctrl Pts',(-0.196107492299332,0.00626222146204868,
0.0100582770154452));
#28675=CARTESIAN_POINT('Ctrl Pts',(-0.196109509262426,0.00629453547881922,
0.0100624958862634));
#28676=CARTESIAN_POINT('Ctrl Pts',(-0.196112005272899,0.0063334107959747,
0.0100673940802161));
#28677=CARTESIAN_POINT('Ctrl Pts',(-0.196114501283371,0.00637228611313019,
0.0100722922741689));
#28678=CARTESIAN_POINT('Ctrl Pts',(-0.196117478944139,0.00641773652099083,
0.0100777539636736));
#28679=CARTESIAN_POINT('Ctrl Pts',(-0.196120634241672,0.00646432235999981,
0.0100829714859763));
#28680=CARTESIAN_POINT('Ctrl Pts',(-0.196126944836739,0.00655749403801779,
0.0100934065305818));
#28681=CARTESIAN_POINT('Ctrl Pts',(-0.196133962757214,0.00665519391160338,
0.010103007929413));
#28682=CARTESIAN_POINT('Ctrl Pts',(-0.196141910262291,0.00676142536250142,
0.0101115466471449));
#28683=CARTESIAN_POINT('Ctrl Pts',(-0.196157805269417,0.00697388822379259,
0.010128624079353));
#28684=CARTESIAN_POINT('Ctrl Pts',(-0.196177421541099,0.00722047876700838,
0.0101413216007707));
#28685=CARTESIAN_POINT('Ctrl Pts',(-0.196200534622597,0.00749682940687443,
0.0101419375907076));
#28686=CARTESIAN_POINT('',(-0.196289694237227,0.0123980179824918,0.00877562173246871));
#28687=CARTESIAN_POINT('Ctrl Pts',(-0.196200534635816,0.00749682956492873,
0.0101419375910599));
#28688=CARTESIAN_POINT('Ctrl Pts',(-0.196177276589334,0.00777317637202428,
0.0101415055483995));
#28689=CARTESIAN_POINT('Ctrl Pts',(-0.196157531423872,0.00801978727065713,
0.0101289709947919));
#28690=CARTESIAN_POINT('Ctrl Pts',(-0.196141525528564,0.00823228920837771,
0.0101120304784238));
#28691=CARTESIAN_POINT('Ctrl Pts',(-0.196133522580911,0.008338540177238,
0.0101035602202398));
#28692=CARTESIAN_POINT('Ctrl Pts',(-0.196126453718094,0.00843626423202327,
0.0100940208040487));
#28693=CARTESIAN_POINT('Ctrl Pts',(-0.196120094749083,0.00852946486601058,
0.0100836436364289));
#28694=CARTESIAN_POINT('Ctrl Pts',(-0.196116915264578,0.00857606518300422,
0.0100784550526191));
#28695=CARTESIAN_POINT('Ctrl Pts',(-0.196113914059311,0.00862153128516846,
0.0100730212605219));
#28696=CARTESIAN_POINT('Ctrl Pts',(-0.196111397802879,0.00866042255792442,
0.0100681464772229));
#28697=CARTESIAN_POINT('Ctrl Pts',(-0.196108881546448,0.00869931383068038,
0.010063271693924));
#28698=CARTESIAN_POINT('Ctrl Pts',(-0.196106847634349,0.00873164399457394,
0.0100590718101258));
#28699=CARTESIAN_POINT('Ctrl Pts',(-0.196104046485699,0.00877966529198083,
0.0100524412147516));
#28700=CARTESIAN_POINT('Ctrl Pts',(-0.196101245337049,0.00882768658938773,
0.0100458106193774));
#28701=CARTESIAN_POINT('Ctrl Pts',(-0.196097681806366,0.0088913700220046,
0.0100365329555621));
#28702=CARTESIAN_POINT('Ctrl Pts',(-0.196094621587336,0.00895016935677664,
0.0100273336378995));
#28703=CARTESIAN_POINT('Ctrl Pts',(-0.196091561368305,0.00900896869154867,
0.0100181343202368));
#28704=CARTESIAN_POINT('Ctrl Pts',(-0.196089000994026,0.00906290867838897,
0.0100091683225499));
#28705=CARTESIAN_POINT('Ctrl Pts',(-0.196086636460145,0.00911715513908172,
0.00999969989365157));
#28706=CARTESIAN_POINT('Ctrl Pts',(-0.196081907392384,0.00922564806046722,
0.00998076303585484));
#28707=CARTESIAN_POINT('Ctrl Pts',(-0.196077965906811,0.00933533335161433,
0.00995962741549134));
#28708=CARTESIAN_POINT('Ctrl Pts',(-0.196074985519283,0.00944047383056635,
0.0099375364402495));
#28709=CARTESIAN_POINT('Ctrl Pts',(-0.196069024744227,0.0096507547884704,
0.0098933544897658));
#28710=CARTESIAN_POINT('Ctrl Pts',(-0.196066889138433,0.00984303266291651,
0.00984621534378884));
#28711=CARTESIAN_POINT('Ctrl Pts',(-0.196068960891635,0.0100440889418934,
0.00979017784857315));
#28712=CARTESIAN_POINT('Ctrl Pts',(-0.196071032644837,0.0102451452208703,
0.00973414035335747));
#28713=CARTESIAN_POINT('Ctrl Pts',(-0.196077329814913,0.0104547341212989,
0.00966837753257755));
#28714=CARTESIAN_POINT('Ctrl Pts',(-0.196088794234009,0.0106610878249387,
0.00959544953614604));
#28715=CARTESIAN_POINT('Ctrl Pts',(-0.196089766942066,0.0106785960744598,
0.00958926190037273));
#28716=CARTESIAN_POINT('Ctrl Pts',(-0.196090776858213,0.0106960819662541,
0.00958302432059695));
#28717=CARTESIAN_POINT('Ctrl Pts',(-0.19609182253648,0.0107135375227711,
0.00957673971280791));
#28718=CARTESIAN_POINT('Ctrl Pts',(-0.196103101310356,0.0109018146257095,
0.00950895340381963));
#28719=CARTESIAN_POINT('Ctrl Pts',(-0.196118540635543,0.0110864784082488,
0.00943550685500762));
#28720=CARTESIAN_POINT('Ctrl Pts',(-0.196136326039856,0.0112581063636262,
0.00936147409591625));
#28721=CARTESIAN_POINT('Ctrl Pts',(-0.196146043202675,0.011351876331258,
0.00932102585187333));
#28722=CARTESIAN_POINT('Ctrl Pts',(-0.196156457446536,0.0114418177297387,
0.00928054563720497));
#28723=CARTESIAN_POINT('Ctrl Pts',(-0.196168015734873,0.0115359797763114,
0.00923629917301674));
#28724=CARTESIAN_POINT('Ctrl Pts',(-0.196173794879042,0.0115830607995978,
0.00921417594092263));
#28725=CARTESIAN_POINT('Ctrl Pts',(-0.196179859956068,0.0116311967773508,
0.00919111429181154));
#28726=CARTESIAN_POINT('Ctrl Pts',(-0.196186821829453,0.0116842943055095,
0.00916503255320362));
#28727=CARTESIAN_POINT('Ctrl Pts',(-0.196193783702839,0.0117373918336683,
0.00913895081459569));
#28728=CARTESIAN_POINT('Ctrl Pts',(-0.196201645404458,0.0117953798276383,
0.00910970194449075));
#28729=CARTESIAN_POINT('Ctrl Pts',(-0.196207602088749,0.011838565397306,
0.00908750520708496));
#28730=CARTESIAN_POINT('Ctrl Pts',(-0.196213558773039,0.0118817509669737,
0.00906530846967916));
#28731=CARTESIAN_POINT('Ctrl Pts',(-0.196217606038112,0.0119102464348559,
0.00905038037191789));
#28732=CARTESIAN_POINT('Ctrl Pts',(-0.196222889321542,0.0119471453490749,
0.00903080940373713));
#28733=CARTESIAN_POINT('Ctrl Pts',(-0.196228172604971,0.0119840442632939,
0.00901123843555637));
#28734=CARTESIAN_POINT('Ctrl Pts',(-0.196234694346225,0.0120292814575428,
0.00898690361769893));
#28735=CARTESIAN_POINT('Ctrl Pts',(-0.196241667116672,0.0120769974006122,
0.00896063422923547));
#28736=CARTESIAN_POINT('Ctrl Pts',(-0.196255612617835,0.0121724290148659,
0.00890809560199133));
#28737=CARTESIAN_POINT('Ctrl Pts',(-0.196271358170245,0.012277893677688,
0.00884802326661943));
#28738=CARTESIAN_POINT('Ctrl Pts',(-0.196289694237227,0.0123980179824918,
0.00877562173246871));
#28739=CARTESIAN_POINT('',(-0.195088692557014,0.012399858493754,0.00875103165054581));
#28740=CARTESIAN_POINT('',(-0.196289694536967,0.0123980145734612,0.00877561378979003));
#28741=CARTESIAN_POINT('',(-0.195000270973505,0.00749643710195729,0.0101148104777022));
#28742=CARTESIAN_POINT('Ctrl Pts',(-0.195088686761518,0.0123998593307978,
0.0087510315654015));
#28743=CARTESIAN_POINT('Ctrl Pts',(-0.195070524157984,0.012280426500865,
0.00882282829312997));
#28744=CARTESIAN_POINT('Ctrl Pts',(-0.195047066286106,0.0121226970251309,
0.00891262811377333));
#28745=CARTESIAN_POINT('Ctrl Pts',(-0.195021091927219,0.011941375725594,
0.00900984723560098));
#28746=CARTESIAN_POINT('Ctrl Pts',(-0.195008801086326,0.0118542212625203,
0.00905547838632326));
#28747=CARTESIAN_POINT('Ctrl Pts',(-0.19498554606785,0.011681164348149,
0.00914263187491693));
#28748=CARTESIAN_POINT('Ctrl Pts',(-0.194961527649185,0.0114884416080279,
0.00923455510442664));
#28749=CARTESIAN_POINT('Ctrl Pts',(-0.194925387021228,0.0111721758540357,
0.00937684361623232));
#28750=CARTESIAN_POINT('Ctrl Pts',(-0.19488468173109,0.0106667894376668,
0.00957614827161772));
#28751=CARTESIAN_POINT('Ctrl Pts',(-0.194866009785313,0.0100353625144586,
0.00977316795720429));
#28752=CARTESIAN_POINT('Ctrl Pts',(-0.194871255332421,0.00955436493404818,
0.0098906602441633));
#28753=CARTESIAN_POINT('Ctrl Pts',(-0.194884823298476,0.00917052629843446,
0.00996454232337369));
#28754=CARTESIAN_POINT('Ctrl Pts',(-0.194894908669353,0.00895478347064921,
0.010000396236686));
#28755=CARTESIAN_POINT('Ctrl Pts',(-0.194905417808874,0.00876415090922611,
0.0100280594449763));
#28756=CARTESIAN_POINT('Ctrl Pts',(-0.194911493249848,0.00866621227369239,
0.0100406662862808));
#28757=CARTESIAN_POINT('Ctrl Pts',(-0.194923381164897,0.0084838614482423,
0.010062484755121));
#28758=CARTESIAN_POINT('Ctrl Pts',(-0.194947903272857,0.00814125774315901,
0.0100956622885852));
#28759=CARTESIAN_POINT('Ctrl Pts',(-0.194977236161783,0.00777195597507231,
0.0101143944992188));
#28760=CARTESIAN_POINT('Ctrl Pts',(-0.195000270973505,0.00749643710195729,
0.0101148104777022));
#28761=CARTESIAN_POINT('',(-0.194890827700361,0.00594838029502342,0.00998416681136753));
#28762=CARTESIAN_POINT('Ctrl Pts',(-0.195000270970932,0.00749643707118917,
0.0101148104776324));
#28763=CARTESIAN_POINT('Ctrl Pts',(-0.194977245972861,0.00722106026275752,
0.0101141855185706));
#28764=CARTESIAN_POINT('Ctrl Pts',(-0.194947928951926,0.0068519599252208,
0.0100951947060793));
#28765=CARTESIAN_POINT('Ctrl Pts',(-0.194923425325342,0.00650953030717665,
0.0100617907603107));
#28766=CARTESIAN_POINT('Ctrl Pts',(-0.194911550293609,0.00632728904432808,
0.010039858086659));
#28767=CARTESIAN_POINT('Ctrl Pts',(-0.194905479264634,0.00622935798919421,
0.0100271829557886));
#28768=CARTESIAN_POINT('Ctrl Pts',(-0.194896524007881,0.00606673866737475,
0.010003472786475));
#28769=CARTESIAN_POINT('Ctrl Pts',(-0.194892260299988,0.00597926531552397,
0.00998933372937761));
#28770=CARTESIAN_POINT('Ctrl Pts',(-0.194890827700361,0.00594838029502342,
0.00998416681136753));
#28771=CARTESIAN_POINT('',(-0.194091473879223,0.00595018587709226,0.00996655302891216));
#28772=CARTESIAN_POINT('Ctrl Pts',(-0.194890828691577,0.00594838854289509,
0.00998411723525648));
#28773=CARTESIAN_POINT('Ctrl Pts',(-0.194091473879223,0.00595018587709227,
0.00996655302891217));
#28774=CARTESIAN_POINT('',(-0.194201348312574,0.00749635098887472,0.0100967541335085));
#28775=CARTESIAN_POINT('Ctrl Pts',(-0.194091473879223,0.00595018587709226,
0.00996655302891216));
#28776=CARTESIAN_POINT('Ctrl Pts',(-0.194092893260719,0.00598038565548873,
0.00997158348733984));
#28777=CARTESIAN_POINT('Ctrl Pts',(-0.1940944124127,0.0060111935220733,
0.00997657056587733));
#28778=CARTESIAN_POINT('Ctrl Pts',(-0.194096081351887,0.00604346677041894,
0.00998162208136269));
#28779=CARTESIAN_POINT('Ctrl Pts',(-0.194099120690989,0.00610224023943114,
0.00999082149896281));
#28780=CARTESIAN_POINT('Ctrl Pts',(-0.194102660243686,0.00616589483843443,
0.0100001022695497));
#28781=CARTESIAN_POINT('Ctrl Pts',(-0.194105442536318,0.00621389063753854,
0.0100067364108301));
#28782=CARTESIAN_POINT('Ctrl Pts',(-0.194108224828951,0.00626188643664265,
0.0100133705521104));
#28783=CARTESIAN_POINT('Ctrl Pts',(-0.194110245029893,0.00629419453290709,
0.0100175734425098));
#28784=CARTESIAN_POINT('Ctrl Pts',(-0.19411274481096,0.00633306407823682,
0.0100224533522769));
#28785=CARTESIAN_POINT('Ctrl Pts',(-0.194115244592027,0.00637193362356654,
0.010027333262044));
#28786=CARTESIAN_POINT('Ctrl Pts',(-0.19411822654559,0.0064173783039094,
0.0100327748217541));
#28787=CARTESIAN_POINT('Ctrl Pts',(-0.194121385941165,0.00646395830510856,
0.0100379733009625));
#28788=CARTESIAN_POINT('Ctrl Pts',(-0.194127704732313,0.00655711830750687,
0.0100483702593794));
#28789=CARTESIAN_POINT('Ctrl Pts',(-0.194134730082943,0.00665480616567737,
0.0100579373457575));
#28790=CARTESIAN_POINT('Ctrl Pts',(-0.194142684768261,0.00676102501734502,
0.0100664466792698));
#28791=CARTESIAN_POINT('Ctrl Pts',(-0.194158594136303,0.00697346268606376,
0.0100834653435213));
#28792=CARTESIAN_POINT('Ctrl Pts',(-0.194178223760992,0.00722002570874856,
0.0100961241872306));
#28793=CARTESIAN_POINT('Ctrl Pts',(-0.194201348677899,0.00749635095831825,
0.0100967541262211));
#28794=CARTESIAN_POINT('',(-0.194290135517151,0.0124010358448944,0.00873473146705155));
#28795=CARTESIAN_POINT('Ctrl Pts',(-0.194201348689204,0.00749635109339938,
0.010096754126529));
#28796=CARTESIAN_POINT('Ctrl Pts',(-0.19417839809719,0.00777274162232543,
0.0100963427415159));
#28797=CARTESIAN_POINT('Ctrl Pts',(-0.194158914654811,0.00801941390229902,
0.0100838710831682));
#28798=CARTESIAN_POINT('Ctrl Pts',(-0.194143121423411,0.00823199987814832,
0.0100670009474999));
#28799=CARTESIAN_POINT('Ctrl Pts',(-0.194135224807711,0.00833829286607297,
0.0100585658796657));
#28800=CARTESIAN_POINT('Ctrl Pts',(-0.194128250013288,0.00843606460448117,
0.0100490634695762));
#28801=CARTESIAN_POINT('Ctrl Pts',(-0.194121976173201,0.00852931596995155,
0.0100387245100895));
#28802=CARTESIAN_POINT('Ctrl Pts',(-0.194118839253157,0.00857594165268673,
0.0100335550303461));
#28803=CARTESIAN_POINT('Ctrl Pts',(-0.194115878374334,0.00862143390960432,
0.0100281407808191));
#28804=CARTESIAN_POINT('Ctrl Pts',(-0.194113395643768,0.00866035501257453,
0.0100232823451317));
#28805=CARTESIAN_POINT('Ctrl Pts',(-0.194110912913201,0.00869927611554473,
0.0100184239094444));
#28806=CARTESIAN_POINT('Ctrl Pts',(-0.194108905736036,0.00873163968044151,
0.0100142367594833));
#28807=CARTESIAN_POINT('Ctrl Pts',(-0.194106143178116,0.00877968609643283,
0.010007629394791));
#28808=CARTESIAN_POINT('Ctrl Pts',(-0.194103380620196,0.00882773251242415,
0.0100010220300988));
#28809=CARTESIAN_POINT('Ctrl Pts',(-0.194099867516978,0.00889143300494494,
0.00999177891797512));
#28810=CARTESIAN_POINT('Ctrl Pts',(-0.194096850970845,0.0089502520280375,
0.0099826130467189));
#28811=CARTESIAN_POINT('Ctrl Pts',(-0.194093834424713,0.00900907105113006,
0.00997344717546269));
#28812=CARTESIAN_POINT('Ctrl Pts',(-0.194091310982932,0.00906303316147349,
0.00996451291131835));
#28813=CARTESIAN_POINT('Ctrl Pts',(-0.194088981155853,0.00911730215254522,
0.00995507773633089));
#28814=CARTESIAN_POINT('Ctrl Pts',(-0.194084321501694,0.00922584013468866,
0.00993620738635599));
#28815=CARTESIAN_POINT('Ctrl Pts',(-0.19408044051176,0.00933557236943365,
0.00991514499932196));
#28816=CARTESIAN_POINT('Ctrl Pts',(-0.194077508702697,0.00944075777199428,
0.00989313016091075));
#28817=CARTESIAN_POINT('Ctrl Pts',(-0.194071645084572,0.00965112857711557,
0.00984910048408833));
#28818=CARTESIAN_POINT('Ctrl Pts',(-0.194069559001171,0.00984348716114984,
0.00980212389481556));
#28819=CARTESIAN_POINT('Ctrl Pts',(-0.194071632503713,0.0100446831425687,
0.00974626273392905));
#28820=CARTESIAN_POINT('Ctrl Pts',(-0.194073706006256,0.0102458791239875,
0.00969040157304254));
#28821=CARTESIAN_POINT('Ctrl Pts',(-0.194079957172833,0.0104556674988114,
0.0096248275184175));
#28822=CARTESIAN_POINT('Ctrl Pts',(-0.194091310588948,0.0106621736514585,
0.00955212697861027));
#28823=CARTESIAN_POINT('Ctrl Pts',(-0.194092096501302,0.0106764685328405,
0.00954709446224389));
#28824=CARTESIAN_POINT('Ctrl Pts',(-0.194092906868285,0.0106907483068779,
0.00954202890043225));
#28825=CARTESIAN_POINT('Ctrl Pts',(-0.194093740917631,0.0107050086814893,
0.00953693185123461));
#28826=CARTESIAN_POINT('Ctrl Pts',(-0.194104955679111,0.0108967559691738,
0.00946839610897852));
#28827=CARTESIAN_POINT('Ctrl Pts',(-0.194120452193851,0.0110849074006952,
0.00939396682608216));
#28828=CARTESIAN_POINT('Ctrl Pts',(-0.194138353045008,0.0112596343946404,
0.00931890116882885));
#28829=CARTESIAN_POINT('Ctrl Pts',(-0.19414796911975,0.0113534951735784,
0.00927857699852063));
#28830=CARTESIAN_POINT('Ctrl Pts',(-0.19415827580787,0.011443544814752,
0.00923821296413418));
#28831=CARTESIAN_POINT('Ctrl Pts',(-0.194169714563209,0.0115378191763271,
0.00919409524759436));
#28832=CARTESIAN_POINT('Ctrl Pts',(-0.194175433940879,0.0115849563571147,
0.00917203638932445));
#28833=CARTESIAN_POINT('Ctrl Pts',(-0.194181436256656,0.0116331495330089,
0.00914904227575429));
#28834=CARTESIAN_POINT('Ctrl Pts',(-0.19418832529866,0.0116863066725952,
0.00912303927144579));
#28835=CARTESIAN_POINT('Ctrl Pts',(-0.194195214340665,0.0117394638121814,
0.0090970362671373));
#28836=CARTESIAN_POINT('Ctrl Pts',(-0.194202993125362,0.0117975143746339,
0.0090678778462092));
#28837=CARTESIAN_POINT('Ctrl Pts',(-0.194208889351679,0.0118407646400332,
0.00904574078869874));
#28838=CARTESIAN_POINT('Ctrl Pts',(-0.194214785577995,0.0118840149054326,
0.00902360373118828));
#28839=CARTESIAN_POINT('Ctrl Pts',(-0.194218794866063,0.0119125763632006,
0.00900870385309618));
#28840=CARTESIAN_POINT('Ctrl Pts',(-0.194224025749138,0.0119495408514585,
0.00898918035970167));
#28841=CARTESIAN_POINT('Ctrl Pts',(-0.194229256632214,0.0119865053397165,
0.00896965686630715));
#28842=CARTESIAN_POINT('Ctrl Pts',(-0.194235711537924,0.0120318081568371,
0.00894538912837073));
#28843=CARTESIAN_POINT('Ctrl Pts',(-0.194242612268476,0.0120795910204617,
0.00891919414592734));
#28844=CARTESIAN_POINT('Ctrl Pts',(-0.194256413690112,0.012175156474426,
0.00886680433085772));
#28845=CARTESIAN_POINT('Ctrl Pts',(-0.194271994367652,0.0122807592863758,
0.00880690946492122));
#28846=CARTESIAN_POINT('Ctrl Pts',(-0.194290135517151,0.0124010358448944,
0.00873473146705154));
#28847=CARTESIAN_POINT('',(-0.193089361378644,0.0124020596755973,0.00871070447764098));
#28848=CARTESIAN_POINT('',(-0.194290135807019,0.0124010327218338,0.00873472395739432));
#28849=CARTESIAN_POINT('',(-0.193001273707137,0.00749669443297029,0.0100696315455101));
#28850=CARTESIAN_POINT('Ctrl Pts',(-0.193089358767972,0.0124020584333727,
0.00871070174821093));
#28851=CARTESIAN_POINT('Ctrl Pts',(-0.193071463321464,0.0122825687629352,
0.00878220102527336));
#28852=CARTESIAN_POINT('Ctrl Pts',(-0.193048338632269,0.0121247155490339,
0.00887166876060142));
#28853=CARTESIAN_POINT('Ctrl Pts',(-0.193022710464114,0.0119431553320592,
0.00896858691283708));
#28854=CARTESIAN_POINT('Ctrl Pts',(-0.193010556294765,0.0118556966153157,
0.00901417351058592));
#28855=CARTESIAN_POINT('Ctrl Pts',(-0.192987610729991,0.0116825316742599,
0.00910099721599476));
#28856=CARTESIAN_POINT('Ctrl Pts',(-0.192963877510663,0.0114895941408424,
0.00919262043208103));
#28857=CARTESIAN_POINT('Ctrl Pts',(-0.192928147068825,0.0111733485297158,
0.00933431543839347));
#28858=CARTESIAN_POINT('Ctrl Pts',(-0.192887506351826,0.010665479443791,
0.00953365685024814));
#28859=CARTESIAN_POINT('Ctrl Pts',(-0.192868616421275,0.0100366274996396,
0.00972901949957174));
#28860=CARTESIAN_POINT('Ctrl Pts',(-0.192873471399313,0.00955372558207172,
0.00984654890078579));
#28861=CARTESIAN_POINT('Ctrl Pts',(-0.192886770773999,0.00917022211560873,
0.00992002607284564));
#28862=CARTESIAN_POINT('Ctrl Pts',(-0.192896701545223,0.00895471565908591,
0.00995569170294781));
#28863=CARTESIAN_POINT('Ctrl Pts',(-0.192907068941763,0.00876450992109302,
0.00998318410436103));
#28864=CARTESIAN_POINT('Ctrl Pts',(-0.19291308785454,0.00866655446820109,
0.00999574754872156));
#28865=CARTESIAN_POINT('Ctrl Pts',(-0.192924866870832,0.00848429967818722,
0.0100174729609137));
#28866=CARTESIAN_POINT('Ctrl Pts',(-0.192949204804265,0.00814172016512548,
0.0100505317675662));
#28867=CARTESIAN_POINT('Ctrl Pts',(-0.192978361376715,0.00777233514591411,
0.0100692104249619));
#28868=CARTESIAN_POINT('Ctrl Pts',(-0.193001273707137,0.00749669443297029,
0.0100696315455101));
#28869=CARTESIAN_POINT('',(-0.192891760060441,0.00595287508888906,0.00994024214377629));
#28870=CARTESIAN_POINT('Ctrl Pts',(-0.193001273760643,0.00749669378927915,
0.0100696315464935));
#28871=CARTESIAN_POINT('Ctrl Pts',(-0.192978205734294,0.00722129220356709,
0.0100690135372334));
#28872=CARTESIAN_POINT('Ctrl Pts',(-0.192948829052146,0.00685217164030578,
0.0100501026422024));
#28873=CARTESIAN_POINT('Ctrl Pts',(-0.192924266441674,0.00650973865669913,
0.0100168357684943));
#28874=CARTESIAN_POINT('Ctrl Pts',(-0.192912358362987,0.00632750117293093,
0.00999499336760895));
#28875=CARTESIAN_POINT('Ctrl Pts',(-0.192906269413198,0.00622957857896456,
0.00998237122778532));
#28876=CARTESIAN_POINT('Ctrl Pts',(-0.192897372796077,0.00606860775490319,
0.0099589975389574));
#28877=CARTESIAN_POINT('Ctrl Pts',(-0.192893142125076,0.00598239332744973,
0.00994514452605578));
#28878=CARTESIAN_POINT('Ctrl Pts',(-0.192891760060441,0.00595287508888906,
0.00994024214377629));
#28879=CARTESIAN_POINT('',(-0.192094713079881,0.0059546755560343,0.0099226782462026));
#28880=CARTESIAN_POINT('Ctrl Pts',(-0.192891761067258,0.00595288340868952,
0.00994019176473061));
#28881=CARTESIAN_POINT('Ctrl Pts',(-0.192094713079881,0.00595467555603431,
0.00992267824620261));
#28882=CARTESIAN_POINT('',(-0.192177628746443,0.00719873229308102,0.0100462148679757));
#28883=CARTESIAN_POINT('Ctrl Pts',(-0.192177628746443,0.00719873229308102,
0.0100462148679757));
#28884=CARTESIAN_POINT('Ctrl Pts',(-0.192167980406568,0.00707953718124289,
0.01004222928847));
#28885=CARTESIAN_POINT('Ctrl Pts',(-0.192158471548071,0.00695723555078092,
0.0100358498652635));
#28886=CARTESIAN_POINT('Ctrl Pts',(-0.192149223388019,0.00683104810276648,
0.0100267199468337));
#28887=CARTESIAN_POINT('Ctrl Pts',(-0.192140662013969,0.0067142315752879,
0.0100182680335577));
#28888=CARTESIAN_POINT('Ctrl Pts',(-0.192132326398386,0.00659409211459482,
0.01000735549836));
#28889=CARTESIAN_POINT('Ctrl Pts',(-0.19212465062001,0.00647606086168701,
0.00999439458421457));
#28890=CARTESIAN_POINT('Ctrl Pts',(-0.192120812730822,0.0064170452352331,
0.00998791412714188));
#28891=CARTESIAN_POINT('Ctrl Pts',(-0.192117138346337,0.00635855104574488,
0.00998098610549107));
#28892=CARTESIAN_POINT('Ctrl Pts',(-0.192113265796624,0.00629325645586128,
0.00997255046049252));
#28893=CARTESIAN_POINT('Ctrl Pts',(-0.192109393246911,0.00622796186597769,
0.00996411481549397));
#28894=CARTESIAN_POINT('Ctrl Pts',(-0.192105328079181,0.00615589765055839,
0.00995392449603349));
#28895=CARTESIAN_POINT('Ctrl Pts',(-0.192102653944682,0.00610736421817033,
0.00994668951150614));
#28896=CARTESIAN_POINT('Ctrl Pts',(-0.192099979810182,0.00605883078578226,
0.0099394545269788));
#28897=CARTESIAN_POINT('Ctrl Pts',(-0.19209868952615,0.00603377873850918,
0.00993549588664673));
#28898=CARTESIAN_POINT('Ctrl Pts',(-0.192096922039073,0.00599881098332664,
0.00992987630703842));
#28899=CARTESIAN_POINT('Ctrl Pts',(-0.192096246446119,0.00598544513227643,
0.00992772831487772));
#28900=CARTESIAN_POINT('Ctrl Pts',(-0.19209550159305,0.00597063393719339,
0.00992531890744154));
#28901=CARTESIAN_POINT('Ctrl Pts',(-0.192094713079881,0.00595467555603429,
0.0099226782462026));
#28902=CARTESIAN_POINT('',(-0.192202394110733,0.00749688548776383,0.0100515763031989));
#28903=CARTESIAN_POINT('Ctrl Pts',(-0.19220250029781,0.00749685985592344,
0.0100515786483995));
#28904=CARTESIAN_POINT('Ctrl Pts',(-0.192194158548644,0.0073994198253338,
0.0100513576997749));
#28905=CARTESIAN_POINT('Ctrl Pts',(-0.192185843096806,0.00730020111470772,
0.010049657533291));
#28906=CARTESIAN_POINT('Ctrl Pts',(-0.192177628746443,0.00719873229308102,
0.0100462148679757));
#28907=CARTESIAN_POINT('',(-0.192248245628462,0.0121622160293808,0.00883352570391155));
#28908=CARTESIAN_POINT('Ctrl Pts',(-0.192202393318722,0.00749691043568044,
0.0100515762472776));
#28909=CARTESIAN_POINT('Ctrl Pts',(-0.192180228518616,0.0077593291150696,
0.0100511612228246));
#28910=CARTESIAN_POINT('Ctrl Pts',(-0.192161385886692,0.00799320657152351,
0.0100399281001668));
#28911=CARTESIAN_POINT('Ctrl Pts',(-0.19214608376665,0.00819447813377408,
0.01002481001183));
#28912=CARTESIAN_POINT('Ctrl Pts',(-0.19213843270663,0.00829511391489936,
0.0100172509676615));
#28913=CARTESIAN_POINT('Ctrl Pts',(-0.19213166614736,0.00838759844388116,
0.010008748362129));
#28914=CARTESIAN_POINT('Ctrl Pts',(-0.192125567626799,0.00847569269532253,
0.00999951868732737));
#28915=CARTESIAN_POINT('Ctrl Pts',(-0.192122518366519,0.00851973982104321,
0.00999490384992657));
#28916=CARTESIAN_POINT('Ctrl Pts',(-0.192119636826805,0.00856268658865227,
0.0099900756945606));
#28917=CARTESIAN_POINT('Ctrl Pts',(-0.19211721921592,0.00859941695979594,
0.00998574630260704));
#28918=CARTESIAN_POINT('Ctrl Pts',(-0.192114801605036,0.00863614733093961,
0.00998141691065349));
#28919=CARTESIAN_POINT('Ctrl Pts',(-0.192112845631441,0.00866667265043585,
0.00997768820603295));
#28920=CARTESIAN_POINT('Ctrl Pts',(-0.192110143911072,0.00871191896280949,
0.009971817222549));
#28921=CARTESIAN_POINT('Ctrl Pts',(-0.192107442190704,0.00875716527518314,
0.00996594623906505));
#28922=CARTESIAN_POINT('Ctrl Pts',(-0.192103998979885,0.00881710870440329,
0.00995774338022245));
#28923=CARTESIAN_POINT('Ctrl Pts',(-0.192101021701336,0.00887251825317918,
0.00994960527259644));
#28924=CARTESIAN_POINT('Ctrl Pts',(-0.192098044422788,0.00892792780195507,
0.00994146716497044));
#28925=CARTESIAN_POINT('Ctrl Pts',(-0.192095530045259,0.00897882377973813,
0.00993352920721947));
#28926=CARTESIAN_POINT('Ctrl Pts',(-0.192093186612127,0.00903002074062252,
0.00992514684629181));
#28927=CARTESIAN_POINT('Ctrl Pts',(-0.192088499745864,0.00913241466239132,
0.00990838212443648));
#28928=CARTESIAN_POINT('Ctrl Pts',(-0.192084500273023,0.00923598513733071,
0.0098896779208332));
#28929=CARTESIAN_POINT('Ctrl Pts',(-0.192081377795291,0.00933565028455126,
0.00987005703892966));
#28930=CARTESIAN_POINT('Ctrl Pts',(-0.192075132839828,0.00953498057899234,
0.00983081527512258));
#28931=CARTESIAN_POINT('Ctrl Pts',(-0.19207238078893,0.00971882360254878,
0.00978858457889742));
#28932=CARTESIAN_POINT('Ctrl Pts',(-0.192073205607948,0.00990902730152387,
0.00973897536808205));
#28933=CARTESIAN_POINT('Ctrl Pts',(-0.192074030426965,0.010099231000499,
0.00968936615726668));
#28934=CARTESIAN_POINT('Ctrl Pts',(-0.192078443750876,0.0102956373022703,
0.00963184480374686));
#28935=CARTESIAN_POINT('Ctrl Pts',(-0.19208744368846,0.010493041239175,
0.00956677871270986));
#28936=CARTESIAN_POINT('Ctrl Pts',(-0.192090542834519,0.0105610176698445,
0.00954437307736307));
#28937=CARTESIAN_POINT('Ctrl Pts',(-0.192094186834636,0.0106291184315858,
0.00952107554338757));
#28938=CARTESIAN_POINT('Ctrl Pts',(-0.192098268361286,0.0106964909770299,
0.00949717597011999));
#28939=CARTESIAN_POINT('Ctrl Pts',(-0.192106039610979,0.0108247686824003,
0.00945167104822796));
#28940=CARTESIAN_POINT('Ctrl Pts',(-0.192115396998233,0.0109503823502024,
0.00940393032371728));
#28941=CARTESIAN_POINT('Ctrl Pts',(-0.192125599697784,0.0110677442694379,
0.00935672263646901));
#28942=CARTESIAN_POINT('Ctrl Pts',(-0.192133380319991,0.0111572449697668,
0.00932072185276375));
#28943=CARTESIAN_POINT('Ctrl Pts',(-0.192141648232579,0.0112420070490703,
0.00928517282558984));
#28944=CARTESIAN_POINT('Ctrl Pts',(-0.192150895106228,0.0113318344768315,
0.00924587766023839));
#28945=CARTESIAN_POINT('Ctrl Pts',(-0.192155518543052,0.0113767481907121,
0.00922623007756266));
#28946=CARTESIAN_POINT('Ctrl Pts',(-0.192160386727942,0.0114229260324994,
0.00920564494416717));
#28947=CARTESIAN_POINT('Ctrl Pts',(-0.192166015780157,0.0114742829902484,
0.00918217302365252));
#28948=CARTESIAN_POINT('Ctrl Pts',(-0.192171644832372,0.0115256399479974,
0.00915870110313788));
#28949=CARTESIAN_POINT('Ctrl Pts',(-0.1921780377212,0.0115821118763141,
0.00913219959862655));
#28950=CARTESIAN_POINT('Ctrl Pts',(-0.192182785100559,0.0116233971300319,
0.00911246411289596));
#28951=CARTESIAN_POINT('Ctrl Pts',(-0.192187532479917,0.0116646823837497,
0.00909272862716538));
#28952=CARTESIAN_POINT('Ctrl Pts',(-0.192190630073563,0.0116908814352336,
0.00907996747514309));
#28953=CARTESIAN_POINT('Ctrl Pts',(-0.192194774678747,0.0117257245369188,
0.00906279949863401));
#28954=CARTESIAN_POINT('Ctrl Pts',(-0.192198919283931,0.0117605676386041,
0.00904563152212493));
#28955=CARTESIAN_POINT('Ctrl Pts',(-0.192204113235252,0.0118039975259787,
0.00902394217457035));
#28956=CARTESIAN_POINT('Ctrl Pts',(-0.192209681331023,0.0118500055934258,
0.00900043329314138));
#28957=CARTESIAN_POINT('Ctrl Pts',(-0.192220817465032,0.011942021252934,
0.00895341577319288));
#28958=CARTESIAN_POINT('Ctrl Pts',(-0.19223344616902,0.0120444558358653,
0.00889931899870446));
#28959=CARTESIAN_POINT('Ctrl Pts',(-0.192248245628462,0.0121622160293808,
0.00883352570391155));
#28960=CARTESIAN_POINT('',(-0.191554125307806,0.0118883026303221,0.00896741436455696));
#28961=CARTESIAN_POINT('Ctrl Pts',(-0.19224824585784,0.0121622178545567,
0.00883352468417506));
#28962=CARTESIAN_POINT('Ctrl Pts',(-0.192159518863803,0.0121296845027705,
0.00885002244467388));
#28963=CARTESIAN_POINT('Ctrl Pts',(-0.192051956961713,0.0120900338487957,
0.00886978569799122));
#28964=CARTESIAN_POINT('Ctrl Pts',(-0.191942470283334,0.0120490970867389,
0.00888990055962757));
#28965=CARTESIAN_POINT('Ctrl Pts',(-0.191911575843803,0.0120376351952446,
0.00889551572980783));
#28966=CARTESIAN_POINT('Ctrl Pts',(-0.191794878078659,0.0119925045909905,
0.00891747933582714));
#28967=CARTESIAN_POINT('Ctrl Pts',(-0.191680025579849,0.0119451674942562,
0.00894028684644732));
#28968=CARTESIAN_POINT('Ctrl Pts',(-0.191608665025318,0.0119142953286677,
0.0089550645765395));
#28969=CARTESIAN_POINT('Ctrl Pts',(-0.191554125307806,0.011888302630322,
0.00896741436455696));
#28970=CARTESIAN_POINT('',(-0.190961084118303,0.0114685865085303,0.00915978503157149));
#28971=CARTESIAN_POINT('Ctrl Pts',(-0.191554125307806,0.011888302630322,
0.00896741436455696));
#28972=CARTESIAN_POINT('Ctrl Pts',(-0.191553768718147,0.0118881326857775,
0.00896749510950585));
#28973=CARTESIAN_POINT('Ctrl Pts',(-0.191498468995547,0.0118617639595744,
0.00898002307501838));
#28974=CARTESIAN_POINT('Ctrl Pts',(-0.191373580637263,0.0117979333855556,
0.00901020026221204));
#28975=CARTESIAN_POINT('Ctrl Pts',(-0.191231902181779,0.0117097408939042,
0.00905123150723658));
#28976=CARTESIAN_POINT('Ctrl Pts',(-0.191109961893247,0.0116176746087238,
0.009093426564697));
#28977=CARTESIAN_POINT('Ctrl Pts',(-0.19101676606608,0.0115308722382138,
0.00913229805935754));
#28978=CARTESIAN_POINT('Ctrl Pts',(-0.19098601401332,0.0114982365429277,
0.0091467926911297));
#28979=CARTESIAN_POINT('Ctrl Pts',(-0.190959787032258,0.0114700741135794,
0.00915912665052349));
#28980=CARTESIAN_POINT('',(-0.191002065707968,0.00749708279836952,0.0100253807384898));
#28981=CARTESIAN_POINT('Ctrl Pts',(-0.19100206665356,0.0074971335629277,
0.0100244479210457));
#28982=CARTESIAN_POINT('Ctrl Pts',(-0.190986683760753,0.00767397789806786,
0.0100241538388789));
#28983=CARTESIAN_POINT('Ctrl Pts',(-0.190971218918847,0.00785819622901983,
0.0100189885523563));
#28984=CARTESIAN_POINT('Ctrl Pts',(-0.190956182171111,0.00805343011906291,
0.0100072581408944));
#28985=CARTESIAN_POINT('Ctrl Pts',(-0.190948663797244,0.00815104706408445,
0.0100013929351634));
#28986=CARTESIAN_POINT('Ctrl Pts',(-0.190941253875676,0.00825141510217649,
0.00999382328925438));
#28987=CARTESIAN_POINT('Ctrl Pts',(-0.190934286441721,0.00835059160622239,
0.00998476935492619));
#28988=CARTESIAN_POINT('Ctrl Pts',(-0.190930802724744,0.00840017985824532,
0.0099802423877621));
#28989=CARTESIAN_POINT('Ctrl Pts',(-0.190927428745033,0.00844947295853139,
0.00997538355317677));
#28990=CARTESIAN_POINT('Ctrl Pts',(-0.190923860389269,0.00850380681690841,
0.00996954702725766));
#28991=CARTESIAN_POINT('Ctrl Pts',(-0.190920292033504,0.00855814067528543,
0.00996371050133854));
#28992=CARTESIAN_POINT('Ctrl Pts',(-0.190916532851425,0.00861749920453185,
0.00995673852077294));
#28993=CARTESIAN_POINT('Ctrl Pts',(-0.190914005462433,0.0086580952751689,
0.00995171459185508));
#28994=CARTESIAN_POINT('Ctrl Pts',(-0.190911478073442,0.00869869134580596,
0.00994669066293722));
#28995=CARTESIAN_POINT('Ctrl Pts',(-0.190910177721542,0.00872055166708246,
0.00994382666834577));
#28996=CARTESIAN_POINT('Ctrl Pts',(-0.190908423243387,0.00875052923422294,
0.00993982342290933));
#28997=CARTESIAN_POINT('Ctrl Pts',(-0.190906668765231,0.00878050680136342,
0.00993582017747289));
#28998=CARTESIAN_POINT('Ctrl Pts',(-0.190904462326314,0.00881858795112804,
0.00993058103832489));
#28999=CARTESIAN_POINT('Ctrl Pts',(-0.190902180272689,0.00886036900673494,
0.00992451324510244));
#29000=CARTESIAN_POINT('Ctrl Pts',(-0.190897616165437,0.00894393111794873,
0.00991237765865754));
#29001=CARTESIAN_POINT('Ctrl Pts',(-0.190892753455369,0.00904227178739623,
0.00989675575918558));
#29002=CARTESIAN_POINT('Ctrl Pts',(-0.190888956462199,0.00913131048889955,
0.00988124033834146));
#29003=CARTESIAN_POINT('Ctrl Pts',(-0.19088515946903,0.00922034919040288,
0.00986572491749735));
#29004=CARTESIAN_POINT('Ctrl Pts',(-0.190882423438742,0.00930012282878565,
0.00985052905346753));
#29005=CARTESIAN_POINT('Ctrl Pts',(-0.190880507454492,0.00936698017388253,
0.00983717231909918));
#29006=CARTESIAN_POINT('Ctrl Pts',(-0.190878591470243,0.00943383751897941,
0.00982381558473084));
#29007=CARTESIAN_POINT('Ctrl Pts',(-0.190877495133955,0.00948778150108325,
0.00981231581913288));
#29008=CARTESIAN_POINT('Ctrl Pts',(-0.190876883399623,0.00952450165897181,
0.00980434732239747));
#29009=CARTESIAN_POINT('Ctrl Pts',(-0.190876271665291,0.00956122181686037,
0.00979637882566207));
#29010=CARTESIAN_POINT('Ctrl Pts',(-0.190876141741644,0.00958074470783384,
0.00979206747310957));
#29011=CARTESIAN_POINT('Ctrl Pts',(-0.190876061499207,0.00962245794566154,
0.00978257098913304));
#29012=CARTESIAN_POINT('Ctrl Pts',(-0.19087598125677,0.00966417118348925,
0.0097730745051565));
#29013=CARTESIAN_POINT('Ctrl Pts',(-0.190875954631328,0.00972803631233191,
0.00975821523746728));
#29014=CARTESIAN_POINT('Ctrl Pts',(-0.190876427965958,0.00980145036407707,
0.00974002553962839));
#29015=CARTESIAN_POINT('Ctrl Pts',(-0.190876901300588,0.00987486441582223,
0.00972183584178949));
#29016=CARTESIAN_POINT('Ctrl Pts',(-0.190877870777047,0.00995786507123561,
0.0097004880049227));
#29017=CARTESIAN_POINT('Ctrl Pts',(-0.190880285373099,0.0100602485747828,
0.00967209531717562));
#29018=CARTESIAN_POINT('Ctrl Pts',(-0.190882699969151,0.0101626320783299,
0.00964370262942855));
#29019=CARTESIAN_POINT('Ctrl Pts',(-0.190886570246384,0.0102842736444069,
0.00960778445427251));
#29020=CARTESIAN_POINT('Ctrl Pts',(-0.19089094525052,0.0103959644833041,
0.00957237684338193));
#29021=CARTESIAN_POINT('Ctrl Pts',(-0.19089510761836,0.0105022268642017,
0.00953869013216839));
#29022=CARTESIAN_POINT('Ctrl Pts',(-0.190899716336516,0.0105996034892998,
0.00950582546699569));
#29023=CARTESIAN_POINT('Ctrl Pts',(-0.190904641056022,0.0106913959610204,
0.00947339528464159));
#29024=CARTESIAN_POINT('Ctrl Pts',(-0.190910068938224,0.0107925669460626,
0.00943765168353396));
#29025=CARTESIAN_POINT('Ctrl Pts',(-0.190915880692719,0.0108869575165467,
0.00940243567738127));
#29026=CARTESIAN_POINT('Ctrl Pts',(-0.190921901795841,0.0109788179154417,
0.00936661769722615));
#29027=CARTESIAN_POINT('Ctrl Pts',(-0.190933385848026,0.0111540232878415,
0.00929830205057994));
#29028=CARTESIAN_POINT('Ctrl Pts',(-0.190945647941777,0.0113198121677733,
0.00922750758659213));
#29029=CARTESIAN_POINT('Ctrl Pts',(-0.190957452801276,0.0114675275550143,
0.00916024243452467));
#29030=CARTESIAN_POINT('',(-0.190890340272952,0.00595738356554221,0.00989621458805049));
#29031=CARTESIAN_POINT('Ctrl Pts',(-0.190890340272952,0.00595738356554221,
0.00989621458805049));
#29032=CARTESIAN_POINT('Ctrl Pts',(-0.190894915404536,0.00606113469594346,
0.0099132975649711));
#29033=CARTESIAN_POINT('Ctrl Pts',(-0.190900653165076,0.00616984093714869,
0.00992921711480411));
#29034=CARTESIAN_POINT('Ctrl Pts',(-0.190905948052378,0.00626017147666541,
0.00994117671185138));
#29035=CARTESIAN_POINT('Ctrl Pts',(-0.190908643320577,0.00630615263107193,
0.0099472645319996));
#29036=CARTESIAN_POINT('Ctrl Pts',(-0.190911222687648,0.00634736641256037,
0.00995237514057524));
#29037=CARTESIAN_POINT('Ctrl Pts',(-0.190913290364573,0.00637989510476361,
0.00995626995284936));
#29038=CARTESIAN_POINT('Ctrl Pts',(-0.190915358041499,0.00641242379696684,
0.00996016476512347));
#29039=CARTESIAN_POINT('Ctrl Pts',(-0.190916911969626,0.0064362557549028,
0.0099629355045932));
#29040=CARTESIAN_POINT('Ctrl Pts',(-0.190919652594268,0.0064763503677113,
0.00996732930590072));
#29041=CARTESIAN_POINT('Ctrl Pts',(-0.19092239321891,0.00651644498051981,
0.00997172310720824));
#29042=CARTESIAN_POINT('Ctrl Pts',(-0.190926324857418,0.00657282358380945,
0.00997754791989819));
#29043=CARTESIAN_POINT('Ctrl Pts',(-0.190930015220125,0.00662397847503081,
0.00998235767785981));
#29044=CARTESIAN_POINT('Ctrl Pts',(-0.190933705582833,0.00667513336625216,
0.00998716743582143));
#29045=CARTESIAN_POINT('Ctrl Pts',(-0.190937151568628,0.00672105240954706,
0.00999109980941678));
#29046=CARTESIAN_POINT('Ctrl Pts',(-0.190940660503065,0.00676673498668278,
0.0099947106672863));
#29047=CARTESIAN_POINT('Ctrl Pts',(-0.19094767837194,0.00685810014095424,
0.0100019323830254));
#29048=CARTESIAN_POINT('Ctrl Pts',(-0.19095495110437,0.0069485273983888,
0.0100077320996249));
#29049=CARTESIAN_POINT('Ctrl Pts',(-0.190962073245139,0.00703432837724492,
0.0100121057353759));
#29050=CARTESIAN_POINT('Ctrl Pts',(-0.190976316751223,0.00720592099300054,
0.0100208525306791));
#29051=CARTESIAN_POINT('Ctrl Pts',(-0.190989952613009,0.00735900406038744,
0.0100241318856088));
#29052=CARTESIAN_POINT('Ctrl Pts',(-0.191002105392592,0.00749710580794768,
0.01002444878813));
#29053=CARTESIAN_POINT('',(-0.186240951883218,0.00596786139892776,0.00979390672266723));
#29054=CARTESIAN_POINT('Ctrl Pts',(-0.190890340272952,0.00595738356554221,
0.00989621458805049));
#29055=CARTESIAN_POINT('Ctrl Pts',(-0.186240948602376,0.00596783763489472,
0.00979405360344712));
#29056=CARTESIAN_POINT('',(-0.186116972251352,0.00692238523863633,0.0098966261734716));
#29057=CARTESIAN_POINT('Ctrl Pts',(-0.186240951883218,0.00596786139892777,
0.00979390672266723));
#29058=CARTESIAN_POINT('Ctrl Pts',(-0.18618127827554,0.00628331776306349,
0.00984332128605338));
#29059=CARTESIAN_POINT('Ctrl Pts',(-0.186139877348579,0.00660240075550953,
0.00987785878236367));
#29060=CARTESIAN_POINT('Ctrl Pts',(-0.186117379209483,0.00692241345077483,
0.00989663789032303));
#29061=CARTESIAN_POINT('',(-0.186100495909817,0.00706118611434217,0.00990361595894344));
#29062=CARTESIAN_POINT('Ctrl Pts',(-0.186100495909817,0.00706118611434217,
0.00990361595894344));
#29063=CARTESIAN_POINT('Ctrl Pts',(-0.18610727117329,0.00701742533621366,
0.0099017649716299));
#29064=CARTESIAN_POINT('Ctrl Pts',(-0.186113922382522,0.00696643159218044,
0.00989921281268404));
#29065=CARTESIAN_POINT('Ctrl Pts',(-0.186116958514757,0.00692241191146765,
0.00989662830553491));
#29066=CARTESIAN_POINT('',(-0.185999364351488,0.00750000000238413,0.00991138348459431));
#29067=CARTESIAN_POINT('Ctrl Pts',(-0.18599946985063,0.00750001264944467,
0.00991138543689015));
#29068=CARTESIAN_POINT('Ctrl Pts',(-0.186001386963565,0.0074922177442551,
0.00991142880243267));
#29069=CARTESIAN_POINT('Ctrl Pts',(-0.186009183053014,0.00746314578508971,
0.00991164535693259));
#29070=CARTESIAN_POINT('Ctrl Pts',(-0.186021064239623,0.00741696715879665,
0.00991151314847068));
#29071=CARTESIAN_POINT('Ctrl Pts',(-0.18602700643212,0.00739387163006314,
0.00991144702644463));
#29072=CARTESIAN_POINT('Ctrl Pts',(-0.186033970262415,0.00736649702883345,
0.00991130192321211));
#29073=CARTESIAN_POINT('Ctrl Pts',(-0.186042754012062,0.00733038060627387,
0.0099108605130772));
#29074=CARTESIAN_POINT('Ctrl Pts',(-0.186051537761709,0.00729426418371429,
0.00991041910294229));
#29075=CARTESIAN_POINT('Ctrl Pts',(-0.186062143508568,0.00724940808696103,
0.00990958946141067));
#29076=CARTESIAN_POINT('Ctrl Pts',(-0.186070367192256,0.00721342297553624,
0.00990869861220074));
#29077=CARTESIAN_POINT('Ctrl Pts',(-0.186086814559632,0.00714145275268665,
0.00990691691378087));
#29078=CARTESIAN_POINT('Ctrl Pts',(-0.186093720646345,0.00710494689247067,
0.00990546694625697));
#29079=CARTESIAN_POINT('Ctrl Pts',(-0.186100495909817,0.00706118611434217,
0.00990361595894344));
#29080=CARTESIAN_POINT('',(-0.186096189557052,0.00791857507561077,0.00990442417341608));
#29081=CARTESIAN_POINT('Ctrl Pts',(-0.186096189557052,0.00791857507561077,
0.00990442417341608));
#29082=CARTESIAN_POINT('Ctrl Pts',(-0.18607770875607,0.00781175464853721,
0.00990892132930148));
#29083=CARTESIAN_POINT('Ctrl Pts',(-0.186046718548287,0.00767179620115901,
0.00991245356955209));
#29084=CARTESIAN_POINT('Ctrl Pts',(-0.185999469365137,0.00749998520788652,
0.00991138542591451));
#29085=CARTESIAN_POINT('',(-0.186116972833414,0.0080776147210469,0.0098966261914198));
#29086=CARTESIAN_POINT('Ctrl Pts',(-0.18611695911767,0.00807758801254939,
0.00989662832371766));
#29087=CARTESIAN_POINT('Ctrl Pts',(-0.186114180673599,0.00803730371254755,
0.0098989935180196));
#29088=CARTESIAN_POINT('Ctrl Pts',(-0.18610754762937,0.00798419117485202,
0.00990194617345709));
#29089=CARTESIAN_POINT('Ctrl Pts',(-0.186096189557052,0.00791857507561077,
0.00990442417341608));
#29090=CARTESIAN_POINT('',(-0.192768467995089,0.0155311216351573,0.0056536625113424));
#29091=CARTESIAN_POINT('Ctrl Pts',(-0.186117379209481,0.00807758654919004,
0.0098966378903251));
#29092=CARTESIAN_POINT('Ctrl Pts',(-0.186150545225195,0.00854933872546041,
0.00986895434783201));
#29093=CARTESIAN_POINT('Ctrl Pts',(-0.186261919503042,0.0092539535920186,
0.0097760582598693));
#29094=CARTESIAN_POINT('Ctrl Pts',(-0.186527601389658,0.0101614599702767,
0.00955792650929634));
#29095=CARTESIAN_POINT('Ctrl Pts',(-0.18679758954749,0.0108464676001627,
0.00933806715709752));
#29096=CARTESIAN_POINT('Ctrl Pts',(-0.187089763175687,0.011436922039813,
0.00910207381557108));
#29097=CARTESIAN_POINT('Ctrl Pts',(-0.187448533491602,0.0120332237854272,
0.00881682178178802));
#29098=CARTESIAN_POINT('Ctrl Pts',(-0.187826342609042,0.012557792726591,
0.00852178580869477));
#29099=CARTESIAN_POINT('Ctrl Pts',(-0.18840556546863,0.0132382397543376,
0.00808059549680021));
#29100=CARTESIAN_POINT('Ctrl Pts',(-0.189013583658982,0.0138007773072184,
0.00763500415641499));
#29101=CARTESIAN_POINT('Ctrl Pts',(-0.18972487030737,0.0143170911390719,
0.00715050345499707));
#29102=CARTESIAN_POINT('Ctrl Pts',(-0.190247984426023,0.0146379596486388,
0.0068153101803706));
#29103=CARTESIAN_POINT('Ctrl Pts',(-0.190863684275869,0.0149488034885615,
0.00645469056019629));
#29104=CARTESIAN_POINT('Ctrl Pts',(-0.191418393853279,0.0151762816431142,
0.0061643508478786));
#29105=CARTESIAN_POINT('Ctrl Pts',(-0.192123222073703,0.0153998088983173,
0.00585357929219802));
#29106=CARTESIAN_POINT('Ctrl Pts',(-0.19255235159128,0.015492619926808,
0.00571282248164196));
#29107=CARTESIAN_POINT('Ctrl Pts',(-0.192768462908894,0.0155311208402429,
0.00565366372878435));
#29108=CARTESIAN_POINT('',(-0.214999728175217,0.0156143085563526,0.00564621407322209));
#29109=CARTESIAN_POINT('Ctrl Pts',(-0.214999727535667,0.0156143027716101,
0.00564622516979127));
#29110=CARTESIAN_POINT('Ctrl Pts',(-0.20758929868895,0.0155894973834204,
0.00565023637807664));
#29111=CARTESIAN_POINT('Ctrl Pts',(-0.200178876390433,0.0155616813952821,
0.00565299213563701));
#29112=CARTESIAN_POINT('Ctrl Pts',(-0.192768468030038,0.015531113584314,
0.00565367517106059));
#29113=CARTESIAN_POINT('Ctrl Pts',(-0.214999728175217,0.0156143085563526,
0.00564621407322209));
#29114=CARTESIAN_POINT('Ctrl Pts',(-0.215340072574214,0.0156154113571772,
0.00564609976598468));
#29115=CARTESIAN_POINT('Ctrl Pts',(-0.215681165557661,0.0156337701167024,
0.00561327712279368));
#29116=CARTESIAN_POINT('Ctrl Pts',(-0.216016169200434,0.0156661766377763,
0.00555035271376907));
#29117=CARTESIAN_POINT('Ctrl Pts',(-0.216408346438714,0.0157041138370015,
0.00547668927313487));
#29118=CARTESIAN_POINT('Ctrl Pts',(-0.21679217849177,0.0157612870617016,
0.00536172046298686));
#29119=CARTESIAN_POINT('Ctrl Pts',(-0.217156694948461,0.0158297441906165,
0.00520865424064648));
#29120=CARTESIAN_POINT('Ctrl Pts',(-0.21783258679598,0.0159566784194797,
0.00492483656956197));
#29121=CARTESIAN_POINT('Ctrl Pts',(-0.21844207919684,0.0161219310071257,
0.00450934047096636));
#29122=CARTESIAN_POINT('Ctrl Pts',(-0.218954689895408,0.0162629602056725,
0.00399196702471092));
#29123=CARTESIAN_POINT('Ctrl Pts',(-0.219210995244691,0.0163334748049458,
0.00373328030158321));
#29124=CARTESIAN_POINT('Ctrl Pts',(-0.219443075431225,0.0163979734266596,
0.00344928409231887));
#29125=CARTESIAN_POINT('Ctrl Pts',(-0.219646842623798,0.01644956204799,
0.0031433958631618));
#29126=CARTESIAN_POINT('Ctrl Pts',(-0.219815132048998,0.0164921686095318,
0.00289076562563261));
#29127=CARTESIAN_POINT('Ctrl Pts',(-0.219964093926562,0.0165258943750711,
0.00262368966702913));
#29128=CARTESIAN_POINT('Ctrl Pts',(-0.220090794747946,0.0165472343306677,
0.00234431717574848));
#29129=CARTESIAN_POINT('Ctrl Pts',(-0.224903047769934,0.0163974953490442,
0.00232527569536224));
#29130=CARTESIAN_POINT('Ctrl Pts',(-0.228003678801843,0.0163652528946496,
0.00231821622721085));
#29131=CARTESIAN_POINT('Ctrl Pts',(-0.23110431006382,0.0163330357098684,
0.00231114482972889));
#29132=CARTESIAN_POINT('Ctrl Pts',(-0.234204941533998,0.0163008422866106,
0.00230405918705812));
#29133=CARTESIAN_POINT('Ctrl Pts',(-0.224902923051373,0.016421905903896,
0.001999690061282));
#29134=CARTESIAN_POINT('Ctrl Pts',(-0.228003554472057,0.0163857948128496,
0.00199154431614981));
#29135=CARTESIAN_POINT('Ctrl Pts',(-0.231104186130884,0.0163497065102629,
0.00198339075959686));
#29136=CARTESIAN_POINT('Ctrl Pts',(-0.23420481801057,0.0163136399270852,
0.00197522735965944));
#29137=CARTESIAN_POINT('Ctrl Pts',(-0.224902686634519,0.0164496060066283,
0.00134999605462854));
#29138=CARTESIAN_POINT('Ctrl Pts',(-0.228003316903349,0.0164061218898441,
0.00134119319572166));
#29139=CARTESIAN_POINT('Ctrl Pts',(-0.231103947348719,0.0163626446434222,
0.00133240817680761));
#29140=CARTESIAN_POINT('Ctrl Pts',(-0.234204577993315,0.0163191760221561,
0.00132364096404516));
#29141=CARTESIAN_POINT('Ctrl Pts',(-0.22490247733934,0.0164891827557564,
8.48946422705292E-5));
#29142=CARTESIAN_POINT('Ctrl Pts',(-0.2280031047451,0.0164387037966636,
8.36968421714054E-5));
#29143=CARTESIAN_POINT('Ctrl Pts',(-0.231103732057188,0.01638822192355,
8.25020821930779E-5));
#29144=CARTESIAN_POINT('Ctrl Pts',(-0.234204359262361,0.016337735996471,
8.13110569434896E-5));
#29145=CARTESIAN_POINT('Ctrl Pts',(-0.224902601832635,0.0164577305274795,
-0.00116946331798178));
#29146=CARTESIAN_POINT('Ctrl Pts',(-0.22800323228218,0.0164115731563456,
-0.00115947279336496));
#29147=CARTESIAN_POINT('Ctrl Pts',(-0.231103862912676,0.016365419418937,
-0.00114950763219157));
#29148=CARTESIAN_POINT('Ctrl Pts',(-0.234204493754791,0.0163192718567599,
-0.00113956819841304));
#29149=CARTESIAN_POINT('Ctrl Pts',(-0.2249031047193,0.016401050271707,-0.00247428944274167));
#29150=CARTESIAN_POINT('Ctrl Pts',(-0.228003735976318,0.016370691448232,
-0.00246735407024901));
#29151=CARTESIAN_POINT('Ctrl Pts',(-0.231104367476673,0.0163403620163895,
-0.00246039974613875));
#29152=CARTESIAN_POINT('Ctrl Pts',(-0.234204999188339,0.0163100597051565,
-0.00245342363871553));
#29153=CARTESIAN_POINT('Ctrl Pts',(-0.224903620482978,0.0162331344936927,
-0.00377581649114323));
#29154=CARTESIAN_POINT('Ctrl Pts',(-0.228004247053984,0.0162183248288798,
-0.00377611183675602));
#29155=CARTESIAN_POINT('Ctrl Pts',(-0.231104873706723,0.0162035348039987,
-0.00377640360674382));
#29156=CARTESIAN_POINT('Ctrl Pts',(-0.23420550044494,0.0161887639228305,
-0.00377669038870648));
#29157=CARTESIAN_POINT('Ctrl Pts',(-0.224904244439412,0.0157454055087051,
-0.00535508843351867));
#29158=CARTESIAN_POINT('Ctrl Pts',(-0.228004869356698,0.015745877431058,
-0.00536654194974573));
#29159=CARTESIAN_POINT('Ctrl Pts',(-0.231105494288016,0.0157463686608469,
-0.00537798949180189));
#29160=CARTESIAN_POINT('Ctrl Pts',(-0.234206119236561,0.0157468784277487,
-0.00538942975580705));
#29161=CARTESIAN_POINT('Ctrl Pts',(-0.224904927056323,0.014756116525245,
-0.0070809462510311));
#29162=CARTESIAN_POINT('Ctrl Pts',(-0.228005551277712,0.0147682738612367,
-0.00710847555851588));
#29163=CARTESIAN_POINT('Ctrl Pts',(-0.231106175457583,0.0147804448844733,
-0.00713600323790223));
#29164=CARTESIAN_POINT('Ctrl Pts',(-0.234206799604821,0.014792629252247,
-0.00716352865861212));
#29165=CARTESIAN_POINT('Ctrl Pts',(-0.224905705935764,0.0129587456084716,
-0.00904270204015799));
#29166=CARTESIAN_POINT('Ctrl Pts',(-0.228006331471737,0.0129775263446935,
-0.00909152831654588));
#29167=CARTESIAN_POINT('Ctrl Pts',(-0.231106956961612,0.0129963155259409,
-0.00914035417356039));
#29168=CARTESIAN_POINT('Ctrl Pts',(-0.234207582410669,0.0130151128918419,
-0.00918917939755658));
#29169=CARTESIAN_POINT('Ctrl Pts',(-0.224906344901157,0.00996717482975785,
-0.0106558172504251));
#29170=CARTESIAN_POINT('Ctrl Pts',(-0.228006973196984,0.00997888641244874,
-0.0107253416344494));
#29171=CARTESIAN_POINT('Ctrl Pts',(-0.23110760149003,0.00999060093234777,
-0.0107948661290257));
#29172=CARTESIAN_POINT('Ctrl Pts',(-0.234208229780548,0.0100023182636535,
-0.010864390745125));
#29173=CARTESIAN_POINT('Ctrl Pts',(-0.224906421473904,0.00588448586822914,
-0.0108495989887083));
#29174=CARTESIAN_POINT('Ctrl Pts',(-0.228007050197119,0.00587660352368733,
-0.0109217704181749));
#29175=CARTESIAN_POINT('Ctrl Pts',(-0.231107678925808,0.00586871925150363,
-0.0109939418074081));
#29176=CARTESIAN_POINT('Ctrl Pts',(-0.23420830765933,0.00586083314294305,
-0.0110661131658069));
#29177=CARTESIAN_POINT('Ctrl Pts',(-0.224905896797368,0.00275206275993148,
-0.00952499259309634));
#29178=CARTESIAN_POINT('Ctrl Pts',(-0.22800652301585,0.00273399542249794,
-0.00957977151548));
#29179=CARTESIAN_POINT('Ctrl Pts',(-0.231107149196805,0.00271592133715538,
-0.00963455045765119));
#29180=CARTESIAN_POINT('Ctrl Pts',(-0.234207775344483,0.00269784071003669,
-0.00968932931015458));
#29181=CARTESIAN_POINT('Ctrl Pts',(-0.224905188461513,0.000775386387695849,
-0.00774097724716007));
#29182=CARTESIAN_POINT('Ctrl Pts',(-0.228005812987761,0.000760338332521188,
-0.0077754138708565));
#29183=CARTESIAN_POINT('Ctrl Pts',(-0.231106437467874,0.000745278047377309,
-0.00780984908461508));
#29184=CARTESIAN_POINT('Ctrl Pts',(-0.234207061909447,0.000730205873823641,
-0.00784428237662763));
#29185=CARTESIAN_POINT('Ctrl Pts',(-0.224904545212544,-0.00037433699893992,
-0.00611286595312136));
#29186=CARTESIAN_POINT('Ctrl Pts',(-0.228005169500613,-0.000380655003703386,
-0.00613103039787742));
#29187=CARTESIAN_POINT('Ctrl Pts',(-0.231105793767721,-0.000386989095479687,
-0.00614919200572512));
#29188=CARTESIAN_POINT('Ctrl Pts',(-0.234206418022201,-0.000393338834079428,
-0.00616734988680402));
#29189=CARTESIAN_POINT('Ctrl Pts',(-0.224903937950997,-0.00100476933014151,
-0.00458381173225385));
#29190=CARTESIAN_POINT('Ctrl Pts',(-0.228004563842973,-0.000997949740617374,
-0.00458943898701532));
#29191=CARTESIAN_POINT('Ctrl Pts',(-0.231105189790958,-0.000991151361328939,
-0.00459505880592969));
#29192=CARTESIAN_POINT('Ctrl Pts',(-0.234205815794275,-0.000984373265027772,
-0.00460066961067425));
#29193=CARTESIAN_POINT('Ctrl Pts',(-0.224903434943426,-0.00130314167877163,
-0.00330350941820122));
#29194=CARTESIAN_POINT('Ctrl Pts',(-0.228004062879574,-0.00128286930948369,
-0.00330122419140405));
#29195=CARTESIAN_POINT('Ctrl Pts',(-0.231104690943801,-0.00126261869681616,
-0.0032989320974583));
#29196=CARTESIAN_POINT('Ctrl Pts',(-0.234205319131308,-0.00124238896138437,
-0.00329663139924215));
#29197=CARTESIAN_POINT('Ctrl Pts',(-0.224903041260456,-0.00140805611840559,
-0.00232453718253355));
#29198=CARTESIAN_POINT('Ctrl Pts',(-0.228003673257076,-0.0013756315595115,
-0.00231672000225054));
#29199=CARTESIAN_POINT('Ctrl Pts',(-0.231104305522642,-0.00134323774830377,
-0.00230888218475535));
#29200=CARTESIAN_POINT('Ctrl Pts',(-0.234204938019884,-0.00131087220379368,
-0.00230102069899992));
#29201=CARTESIAN_POINT('Ctrl Pts',(-0.224902686634356,-0.00144960594189391,
-0.00134999602285112));
#29202=CARTESIAN_POINT('Ctrl Pts',(-0.228003316903184,-0.00140612182039602,
-0.00134119316178982));
#29203=CARTESIAN_POINT('Ctrl Pts',(-0.23110394734855,-0.00136264456921374,
-0.00133240814074275));
#29204=CARTESIAN_POINT('Ctrl Pts',(-0.234204577993143,-0.00131917594314456,
-0.00132364092587474));
#29205=CARTESIAN_POINT('Ctrl Pts',(-0.22490247733939,-0.0014891827680679,
-8.48946648711828E-5));
#29206=CARTESIAN_POINT('Ctrl Pts',(-0.228003104745152,-0.00143870380997731,
-8.36968663193096E-5));
#29207=CARTESIAN_POINT('Ctrl Pts',(-0.231103732057244,-0.00138822193789455,
-8.25021078797203E-5));
#29208=CARTESIAN_POINT('Ctrl Pts',(-0.23420435926242,-0.00133773601187166,
-8.1311084157012E-5));
#29209=CARTESIAN_POINT('Ctrl Pts',(-0.22490260183294,-0.0014577307002292,
0.00116946334942344));
#29210=CARTESIAN_POINT('Ctrl Pts',(-0.228003232282475,-0.00141157334093523,
0.00115947282708936));
#29211=CARTESIAN_POINT('Ctrl Pts',(-0.231103862912961,-0.00136541961535455,
0.00114950766822477));
#29212=CARTESIAN_POINT('Ctrl Pts',(-0.234204493755065,-0.001319272064998,
0.00113956823678177));
#29213=CARTESIAN_POINT('Ctrl Pts',(-0.224903104718753,-0.00140104996632292,
0.00247428939345485));
#29214=CARTESIAN_POINT('Ctrl Pts',(-0.228003735975788,-0.00137069112187628,
0.00246735401736931));
#29215=CARTESIAN_POINT('Ctrl Pts',(-0.231104367476161,-0.0013403616690761,
0.00246039968961847));
#29216=CARTESIAN_POINT('Ctrl Pts',(-0.234204999187845,-0.00131005933689176,
0.00245342357850486));
#29217=CARTESIAN_POINT('Ctrl Pts',(-0.224903620487317,-0.00123313642614889,
0.00377581720335721));
#29218=CARTESIAN_POINT('Ctrl Pts',(-0.228004247058324,-0.00121832689931329,
0.00377611259775251));
#29219=CARTESIAN_POINT('Ctrl Pts',(-0.231104873711069,-0.00120353701330459,
0.00377640441621043));
#29220=CARTESIAN_POINT('Ctrl Pts',(-0.234205500449294,-0.00118876627184354,
0.00377669124621538));
#29221=CARTESIAN_POINT('Ctrl Pts',(-0.224904244452509,-0.000745411287960432,
0.00535508951527424));
#29222=CARTESIAN_POINT('Ctrl Pts',(-0.228004869369835,-0.000745883603517816,
0.00536654310520161));
#29223=CARTESIAN_POINT('Ctrl Pts',(-0.231105494301186,-0.000746375225293753,
0.00537799072107391));
#29224=CARTESIAN_POINT('Ctrl Pts',(-0.234206119249757,-0.000746885383007411,
0.00538943105918803));
#29225=CARTESIAN_POINT('Ctrl Pts',(-0.224904927022406,0.000243903830950042,
0.00708094602779947));
#29226=CARTESIAN_POINT('Ctrl Pts',(-0.22800555124417,0.000231747907332828,
0.00710847531073915));
#29227=CARTESIAN_POINT('Ctrl Pts',(-0.231106175424446,0.00021957829815924,
0.00713600296412369));
#29228=CARTESIAN_POINT('Ctrl Pts',(-0.234206799572117,0.000207395346249357,
0.0071635283576419));
#29229=CARTESIAN_POINT('Ctrl Pts',(-0.224905705882564,0.00204129536417242,
0.00904270545084878));
#29230=CARTESIAN_POINT('Ctrl Pts',(-0.228006331417495,0.00202251745037019,
0.00909153197079319));
#29231=CARTESIAN_POINT('Ctrl Pts',(-0.231106956906316,0.00200373108991613,
0.00914035807264341));
#29232=CARTESIAN_POINT('Ctrl Pts',(-0.234207582354303,0.00198493654309014,
0.00918918354252649));
#29233=CARTESIAN_POINT('Ctrl Pts',(-0.224906344934492,0.00503279669879239,
0.0106558220281949));
#29234=CARTESIAN_POINT('Ctrl Pts',(-0.228006973230644,0.00502108315461209,
0.0107253467403358));
#29235=CARTESIAN_POINT('Ctrl Pts',(-0.231107601524016,0.00500936667421796,
0.0107948715627757));
#29236=CARTESIAN_POINT('Ctrl Pts',(-0.234208229814862,0.00499764738343722,
0.0108643965065502));
#29237=CARTESIAN_POINT('Ctrl Pts',(-0.22490642148267,0.00911553811978304,
0.0108495997280891));
#29238=CARTESIAN_POINT('Ctrl Pts',(-0.22800705020616,0.00912342211753167,
0.0109217712057851));
#29239=CARTESIAN_POINT('Ctrl Pts',(-0.231107678935135,0.0091313080421625,
0.0109939426427322));
#29240=CARTESIAN_POINT('Ctrl Pts',(-0.234208307668951,0.00913919580236395,
0.0110661140483708));
#29241=CARTESIAN_POINT('Ctrl Pts',(-0.224905896781363,0.0122479140000228,
0.00952499840433065));
#29242=CARTESIAN_POINT('Ctrl Pts',(-0.228006522998932,0.0122659797356893,
0.00957977773742142));
#29243=CARTESIAN_POINT('Ctrl Pts',(-0.231107149178945,0.012284052220171,
0.00963455709198015));
#29244=CARTESIAN_POINT('Ctrl Pts',(-0.234207775325653,0.0123021312474762,
0.00968933635838273));
#29245=CARTESIAN_POINT('Ctrl Pts',(-0.224905188406661,0.0142245802852993,
0.00774097735435126));
#29246=CARTESIAN_POINT('Ctrl Pts',(-0.228005812932864,0.014239626038719,
0.0077754139801973));
#29247=CARTESIAN_POINT('Ctrl Pts',(-0.231106437412959,0.0142546840218181,
0.00780984919513146));
#29248=CARTESIAN_POINT('Ctrl Pts',(-0.234207061854539,0.014269753892948,
0.00784428248742507));
#29249=CARTESIAN_POINT('Ctrl Pts',(-0.224904545213284,0.0153743354777482,
0.00611286639462737));
#29250=CARTESIAN_POINT('Ctrl Pts',(-0.228005169501712,0.0153806533667306,
0.00613103086359291));
#29251=CARTESIAN_POINT('Ctrl Pts',(-0.231105793769188,0.0153869873403304,
0.0061491924949429));
#29252=CARTESIAN_POINT('Ctrl Pts',(-0.234206418024041,0.0153933369583363,
0.00616735039916125));
#29253=CARTESIAN_POINT('Ctrl Pts',(-0.224903937959543,0.0160047733300576,
0.00458381273421664));
#29254=CARTESIAN_POINT('Ctrl Pts',(-0.228004563851456,0.015997954017428,
0.00458944005855562));
#29255=CARTESIAN_POINT('Ctrl Pts',(-0.231105189799372,0.0159911559151915,
0.00459505994710943));
#29256=CARTESIAN_POINT('Ctrl Pts',(-0.234205815802617,0.0159843780961064,
0.00460067082154373));
#29257=CARTESIAN_POINT('Ctrl Pts',(-0.224903434945887,0.0163031426775171,
0.00330350985910996));
#29258=CARTESIAN_POINT('Ctrl Pts',(-0.228004062882068,0.0162828703806443,
0.0033012246620879));
#29259=CARTESIAN_POINT('Ctrl Pts',(-0.231104690946332,0.0162626198410551,
0.00329893259759974));
#29260=CARTESIAN_POINT('Ctrl Pts',(-0.23420531913388,0.0162423901793082,
0.00329663192843727));
#29261=CARTESIAN_POINT('Ctrl Pts',(-0.224903172488496,0.0163730847941923,
0.00265086132944247));
#29262=CARTESIAN_POINT('Ctrl Pts',(-0.22800380313163,0.0163447109764496,
0.00264488813827189));
#29263=CARTESIAN_POINT('Ctrl Pts',(-0.231104433996755,0.0163163649094739,
0.00263889889986091));
#29264=CARTESIAN_POINT('Ctrl Pts',(-0.234205065057425,0.0162880446461359,
0.00263289101445681));
#29265=CARTESIAN_POINT('Ctrl Pts',(-0.224903047769934,0.0163974953490442,
0.00232527569536224));
#29266=CARTESIAN_POINT('Ctrl Pts',(-0.228003678801843,0.0163652528946496,
0.00231821622721085));
#29267=CARTESIAN_POINT('Ctrl Pts',(-0.23110431006382,0.0163330357098684,
0.00231114482972889));
#29268=CARTESIAN_POINT('Ctrl Pts',(-0.234204941533998,0.0163008422866106,
0.00230405918705812));
#29269=CARTESIAN_POINT('',(-0.228104649974285,0.0163642118483275,0.00231798200374012));
#29270=CARTESIAN_POINT('',(-0.225870784240265,0.0163857105469993,0.002322957879709));
#29271=CARTESIAN_POINT('Ctrl Pts',(-0.228104649974285,0.0163642118483275,
0.00231798200374011));
#29272=CARTESIAN_POINT('Ctrl Pts',(-0.227360035832473,0.0163719507139063,
0.00231967936742506));
#29273=CARTESIAN_POINT('Ctrl Pts',(-0.226615421703495,0.0163796910068899,
0.00232137599715635));
#29274=CARTESIAN_POINT('Ctrl Pts',(-0.225870807587654,0.0163874327481649,
0.00232307192500813));
#29275=CARTESIAN_POINT('',(-0.230598290824789,0.00749145062540444,0.0108193267850442));
#29276=CARTESIAN_POINT('Ctrl Pts',(-0.230598338270789,0.00749148676553765,
0.0108179004527726));
#29277=CARTESIAN_POINT('Ctrl Pts',(-0.231075709301529,0.0080180520759082,
0.0108293962485369));
#29278=CARTESIAN_POINT('Ctrl Pts',(-0.231557645328989,0.00854079758906138,
0.0107959726164992));
#29279=CARTESIAN_POINT('Ctrl Pts',(-0.232015464789001,0.00907681658494018,
0.010708872070951));
#29280=CARTESIAN_POINT('Ctrl Pts',(-0.232075029452916,0.00914655541024208,
0.0106975398424733));
#29281=CARTESIAN_POINT('Ctrl Pts',(-0.232134185876658,0.00921651233077271,
0.0106852715763912));
#29282=CARTESIAN_POINT('Ctrl Pts',(-0.232192870888001,0.00928671955653243,
0.0106720330949619));
#29283=CARTESIAN_POINT('Ctrl Pts',(-0.232447746520514,0.00959163746764531,
0.0106145368748788));
#29284=CARTESIAN_POINT('Ctrl Pts',(-0.232693736801378,0.00990130138696256,
0.0105389619391001));
#29285=CARTESIAN_POINT('Ctrl Pts',(-0.232918888539751,0.0102190020370645,
0.0104406042903564));
#29286=CARTESIAN_POINT('Ctrl Pts',(-0.233144040278124,0.0105367026871664,
0.0103422466416127));
#29287=CARTESIAN_POINT('Ctrl Pts',(-0.233348352430801,0.0108624519973364,
0.0102211499069169));
#29288=CARTESIAN_POINT('Ctrl Pts',(-0.233508739760675,0.0111978248649097,
0.0100695900518698));
#29289=CARTESIAN_POINT('Ctrl Pts',(-0.23366912709055,0.011533197732483,
0.00991803019682276));
#29290=CARTESIAN_POINT('Ctrl Pts',(-0.233785605808925,0.0118778624208235,
0.00973525367538941));
#29291=CARTESIAN_POINT('Ctrl Pts',(-0.233833346895058,0.0122149827284696,
0.00952313657254382));
#29292=CARTESIAN_POINT('Ctrl Pts',(-0.233858854995816,0.0123951063802632,
0.00940980223371623));
#29293=CARTESIAN_POINT('Ctrl Pts',(-0.233864744317832,0.0125731343241547,
0.00928811633672739));
#29294=CARTESIAN_POINT('Ctrl Pts',(-0.233851336158348,0.0127452593029888,
0.00916045586438089));
#29295=CARTESIAN_POINT('Ctrl Pts',(-0.233839649540966,0.01289528427637,
0.00904918637232152));
#29296=CARTESIAN_POINT('Ctrl Pts',(-0.233813302729673,0.0130408301132514,
0.00893339848908481));
#29297=CARTESIAN_POINT('Ctrl Pts',(-0.233772508743751,0.0131799182240714,
0.00881533220150123));
#29298=CARTESIAN_POINT('Ctrl Pts',(-0.233684911456983,0.0134785833545798,
0.00856180741795297));
#29299=CARTESIAN_POINT('Ctrl Pts',(-0.233530684540018,0.0137474510773739,
0.00829768449632733));
#29300=CARTESIAN_POINT('Ctrl Pts',(-0.233333723716297,0.0139829954115555,
0.00803862781489455));
#29301=CARTESIAN_POINT('Ctrl Pts',(-0.233268591230206,0.0140608869829865,
0.00795296100369058));
#29302=CARTESIAN_POINT('Ctrl Pts',(-0.233198784817145,0.0141351725004418,
0.00786786509877418));
#29303=CARTESIAN_POINT('Ctrl Pts',(-0.233125029661844,0.0142061824254741,
0.00778346848116448));
#29304=CARTESIAN_POINT('Ctrl Pts',(-0.232975749017138,0.014349906716285,
0.00761264948639352));
#29305=CARTESIAN_POINT('Ctrl Pts',(-0.232810292019128,0.0144802373306716,
0.00744474134059401));
#29306=CARTESIAN_POINT('Ctrl Pts',(-0.232634671293171,0.0145996931398721,
0.00728027181219894));
#29307=CARTESIAN_POINT('Ctrl Pts',(-0.232372281556117,0.0147781685344756,
0.00703454274990358));
#29308=CARTESIAN_POINT('Ctrl Pts',(-0.232087200057163,0.0149326947045112,
0.00679688383923861));
#29309=CARTESIAN_POINT('Ctrl Pts',(-0.231801872342179,0.0150754733334955,
0.00655540940052881));
#29310=CARTESIAN_POINT('Ctrl Pts',(-0.231631035659178,0.0151609603931055,
0.00641082936160338));
#29311=CARTESIAN_POINT('Ctrl Pts',(-0.23146011161664,0.0152420740677067,
0.00626478376969512));
#29312=CARTESIAN_POINT('Ctrl Pts',(-0.231289702355054,0.0153194156731576,
0.00611622994638233));
#29313=CARTESIAN_POINT('Ctrl Pts',(-0.231175497771615,0.0153712483361878,
0.00601667240266783));
#29314=CARTESIAN_POINT('Ctrl Pts',(-0.231061524394753,0.0154213809749297,
0.00591598467855481));
#29315=CARTESIAN_POINT('Ctrl Pts',(-0.230947963472988,0.015469955354092,
0.00581382564276621));
#29316=CARTESIAN_POINT('Ctrl Pts',(-0.230417408077528,0.0156968943269831,
0.00533653973498424));
#29317=CARTESIAN_POINT('Ctrl Pts',(-0.229895853940728,0.0158913130140226,
0.00482791912667798));
#29318=CARTESIAN_POINT('Ctrl Pts',(-0.229425773391357,0.0160470074394846,
0.00426455622278852));
#29319=CARTESIAN_POINT('Ctrl Pts',(-0.229394351628951,0.0160574145776897,
0.00422689915457296));
#29320=CARTESIAN_POINT('Ctrl Pts',(-0.229363159852714,0.0160676398558769,
0.00418899687521678));
#29321=CARTESIAN_POINT('Ctrl Pts',(-0.229332210744518,0.01607767331279,
0.00415084139727865));
#29322=CARTESIAN_POINT('Ctrl Pts',(-0.229110485079378,0.0161495550256201,
0.00387748784308456));
#29323=CARTESIAN_POINT('Ctrl Pts',(-0.228901208712299,0.0162114615840728,
0.00359107867848368));
#29324=CARTESIAN_POINT('Ctrl Pts',(-0.228703844969547,0.0162580746565335,
0.00329766208763771));
#29325=CARTESIAN_POINT('Ctrl Pts',(-0.228681366063252,0.0162633836908746,
0.00326424316297096));
#29326=CARTESIAN_POINT('Ctrl Pts',(-0.228659041690429,0.0162684961078405,
0.00323073414136287));
#29327=CARTESIAN_POINT('Ctrl Pts',(-0.22863687106733,0.0162734193664932,
0.00319714803077916));
#29328=CARTESIAN_POINT('Ctrl Pts',(-0.228447731836008,0.0163154200514998,
0.00291062242838303));
#29329=CARTESIAN_POINT('Ctrl Pts',(-0.228269796174735,0.0163437143844762,
0.00261818156401676));
#29330=CARTESIAN_POINT('Ctrl Pts',(-0.228104649974285,0.0163642118483275,
0.00231798200374011));
#29331=CARTESIAN_POINT('',(-0.227106092853892,-0.00144162713113215,-4.25945305502357E-13));
#29332=CARTESIAN_POINT('Ctrl Pts',(-0.230598290824789,0.00749145062540444,
0.0108193267850442));
#29333=CARTESIAN_POINT('Ctrl Pts',(-0.231137836558405,0.00690031499117376,
0.0108309420867985));
#29334=CARTESIAN_POINT('Ctrl Pts',(-0.231682656491661,0.00631350273122054,
0.0107850743940513));
#29335=CARTESIAN_POINT('Ctrl Pts',(-0.232703657130117,0.00510282767464983,
0.0105570407887783));
#29336=CARTESIAN_POINT('Ctrl Pts',(-0.233184403552031,0.00447117767383195,
0.0103741673526736));
#29337=CARTESIAN_POINT('Ctrl Pts',(-0.233827791930478,0.0031373542154347,
0.0097711747197396));
#29338=CARTESIAN_POINT('Ctrl Pts',(-0.233942287932662,0.0024255222673528,
0.00932750132739732));
#29339=CARTESIAN_POINT('Ctrl Pts',(-0.233597340137198,0.0012312754121852,
0.00831720595736921));
#29340=CARTESIAN_POINT('Ctrl Pts',(-0.233162895208997,0.000765896829771336,
0.00778165408574167));
#29341=CARTESIAN_POINT('Ctrl Pts',(-0.232120497057948,5.30358000006855E-5,
0.00680295301175275));
#29342=CARTESIAN_POINT('Ctrl Pts',(-0.231523946961238,-0.000221033348423707,
0.0063348547730625));
#29343=CARTESIAN_POINT('Ctrl Pts',(-0.2303894174303,-0.000708453126336253,
0.00531619348403926));
#29344=CARTESIAN_POINT('Ctrl Pts',(-0.229838118249783,-0.000912401449299848,
0.00477583518142244));
#29345=CARTESIAN_POINT('Ctrl Pts',(-0.228861523205001,-0.00122893765634945,
0.00357768912857529));
#29346=CARTESIAN_POINT('Ctrl Pts',(-0.228422516777517,-0.00133275751547238,
0.00291658072635947));
#29347=CARTESIAN_POINT('Ctrl Pts',(-0.22766666238982,-0.00140726267608253,
0.00150192904840282));
#29348=CARTESIAN_POINT('Ctrl Pts',(-0.227382852307235,-0.00143731421920346,
0.000752971789795249));
#29349=CARTESIAN_POINT('Ctrl Pts',(-0.227106092853892,-0.00144162713113215,
-4.25945305518629E-13));
#29350=CARTESIAN_POINT('',(-0.230713724481977,0.00748904929732134,-0.0108219320073967));
#29351=CARTESIAN_POINT('Ctrl Pts',(-0.227106121514272,-0.00144104810369251,
-1.02597508904584E-7));
#29352=CARTESIAN_POINT('Ctrl Pts',(-0.227155693329604,-0.00144058004175401,
-0.000133357544037));
#29353=CARTESIAN_POINT('Ctrl Pts',(-0.227205192185135,-0.00143930885807063,
-0.000266817081085626));
#29354=CARTESIAN_POINT('Ctrl Pts',(-0.227255433548676,-0.00143710688843238,
-0.000399941268947333));
#29355=CARTESIAN_POINT('Ctrl Pts',(-0.227349644824292,-0.00143297781322698,
-0.000649572223793228));
#29356=CARTESIAN_POINT('Ctrl Pts',(-0.227446467189041,-0.00142558282116148,
-0.000898063096286006));
#29357=CARTESIAN_POINT('Ctrl Pts',(-0.227551278208355,-0.00141727302005574,
-0.00114210175313649));
#29358=CARTESIAN_POINT('Ctrl Pts',(-0.227580845424984,-0.00141492882293749,
-0.00121094512361562));
#29359=CARTESIAN_POINT('Ctrl Pts',(-0.227611049598159,-0.00141251265768409,
-0.00127939207005976));
#29360=CARTESIAN_POINT('Ctrl Pts',(-0.227641897465485,-0.0014100715425958,
-0.00134749262536686));
#29361=CARTESIAN_POINT('Ctrl Pts',(-0.227778730077697,-0.00139924343085938,
-0.00164956786373419));
#29362=CARTESIAN_POINT('Ctrl Pts',(-0.227928226950739,-0.00138769770517313,
-0.00194470860115159));
#29363=CARTESIAN_POINT('Ctrl Pts',(-0.228090954362009,-0.00136955019749903,
-0.00223115768111268));
#29364=CARTESIAN_POINT('Ctrl Pts',(-0.228107429541393,-0.00136771287063466,
-0.00226015894119409));
#29365=CARTESIAN_POINT('Ctrl Pts',(-0.228124040407681,-0.00136580989150037,
-0.00228907248515574));
#29366=CARTESIAN_POINT('Ctrl Pts',(-0.228140785043584,-0.00136383629327108,
-0.00231789963233035));
#29367=CARTESIAN_POINT('Ctrl Pts',(-0.228326714931641,-0.00134192175897111,
-0.00263799188624149));
#29368=CARTESIAN_POINT('Ctrl Pts',(-0.228529137687204,-0.00131121851168663,
-0.00294734231443703));
#29369=CARTESIAN_POINT('Ctrl Pts',(-0.228745449586204,-0.00126531502200679,
-0.00324782568531596));
#29370=CARTESIAN_POINT('Ctrl Pts',(-0.228757414188977,-0.00126277601688286,
-0.00326444596459402));
#29371=CARTESIAN_POINT('Ctrl Pts',(-0.2287694212518,-0.00126019050384389,
-0.00328103996521208));
#29372=CARTESIAN_POINT('Ctrl Pts',(-0.228781470464013,-0.00125755773271125,
-0.00329760590338844));
#29373=CARTESIAN_POINT('Ctrl Pts',(-0.229006881398939,-0.00120830510175236,
-0.00360751360078454));
#29374=CARTESIAN_POINT('Ctrl Pts',(-0.229247043436343,-0.00114232304878351,
-0.00390750717283466));
#29375=CARTESIAN_POINT('Ctrl Pts',(-0.229499929863164,-0.00106702408187035,
-0.00418927640242565));
#29376=CARTESIAN_POINT('Ctrl Pts',(-0.229522633013788,-0.00106026403622785,
-0.0042145725376951));
#29377=CARTESIAN_POINT('Ctrl Pts',(-0.229545438774004,-0.00105343027253221,
-0.00423972250785708));
#29378=CARTESIAN_POINT('Ctrl Pts',(-0.229568343811177,-0.00104652599570539,
-0.00426473093900274));
#29379=CARTESIAN_POINT('Ctrl Pts',(-0.230082985397726,-0.000891397324517587,
-0.00482663261088408));
#29380=CARTESIAN_POINT('Ctrl Pts',(-0.230647745298193,-0.000704074407847329,
-0.00531755702186263));
#29381=CARTESIAN_POINT('Ctrl Pts',(-0.231224812138477,-0.000484699658335017,
-0.00578481572901948));
#29382=CARTESIAN_POINT('Ctrl Pts',(-0.231363643146476,-0.000431922379381618,
-0.00589722904543737));
#29383=CARTESIAN_POINT('Ctrl Pts',(-0.231503186860206,-0.000377137686368691,
-0.00600819219499035));
#29384=CARTESIAN_POINT('Ctrl Pts',(-0.231642644775951,-0.000320010544310574,
-0.00611831970598614));
#29385=CARTESIAN_POINT('Ctrl Pts',(-0.231805922867053,-0.000253125773693158,
-0.00624725759866292));
#29386=CARTESIAN_POINT('Ctrl Pts',(-0.231969083349277,-0.000183034363518878,
-0.0063750542300276));
#29387=CARTESIAN_POINT('Ctrl Pts',(-0.232130844677489,-0.000109068387591157,
-0.00650260226534622));
#29388=CARTESIAN_POINT('Ctrl Pts',(-0.232430768434771,2.80728788441698E-5,
-0.00673909071663125));
#29389=CARTESIAN_POINT('Ctrl Pts',(-0.232725879386454,0.000178054062844723,
-0.00697503327306245));
#29390=CARTESIAN_POINT('Ctrl Pts',(-0.232995079390541,0.000354507597007201,
-0.00722285002535608));
#29391=CARTESIAN_POINT('Ctrl Pts',(-0.233193492774877,0.000484562360601881,
-0.00740550292198027));
#29392=CARTESIAN_POINT('Ctrl Pts',(-0.23337783274223,0.000629180229882582,
-0.00759438076149401));
#29393=CARTESIAN_POINT('Ctrl Pts',(-0.233537670556691,0.000791923770424381,
-0.00778802745486344));
#29394=CARTESIAN_POINT('Ctrl Pts',(-0.23359469482767,0.00084998469791584,
-0.00785711349407122));
#29395=CARTESIAN_POINT('Ctrl Pts',(-0.233648600459144,0.00091035749609578,
-0.00792679521495199));
#29396=CARTESIAN_POINT('Ctrl Pts',(-0.233698913878109,0.000973215124293755,
-0.00799697080557788));
#29397=CARTESIAN_POINT('Ctrl Pts',(-0.233890254736577,0.00121226134273606,
-0.00826384707894346));
#29398=CARTESIAN_POINT('Ctrl Pts',(-0.234029653034362,0.00148782950287383,
-0.00853756246098401));
#29399=CARTESIAN_POINT('Ctrl Pts',(-0.234097409173442,0.001791730240335,
-0.00879751626456002));
#29400=CARTESIAN_POINT('Ctrl Pts',(-0.234130392260149,0.00193966642014468,
-0.0089240594672824));
#29401=CARTESIAN_POINT('Ctrl Pts',(-0.234146401069839,0.00209427982761353,
-0.00904742046654428));
#29402=CARTESIAN_POINT('Ctrl Pts',(-0.234145973735161,0.00225315437049859,
-0.00916512267717759));
#29403=CARTESIAN_POINT('Ctrl Pts',(-0.234145523209371,0.00242065090741761,
-0.00928921249239144));
#29404=CARTESIAN_POINT('Ctrl Pts',(-0.234126804174283,0.00259287994874721,
-0.00940699897382431));
#29405=CARTESIAN_POINT('Ctrl Pts',(-0.234090447596687,0.00276628068025388,
-0.00951652399136892));
#29406=CARTESIAN_POINT('Ctrl Pts',(-0.234019605920159,0.00310415622694662,
-0.00972993615438505));
#29407=CARTESIAN_POINT('Ctrl Pts',(-0.233881780562192,0.00344657603079677,
-0.00991199840598362));
#29408=CARTESIAN_POINT('Ctrl Pts',(-0.233704476049298,0.00377932616870677,
-0.0100631762672343));
#29409=CARTESIAN_POINT('Ctrl Pts',(-0.233527171536405,0.00411207630661675,
-0.010214354128485));
#29410=CARTESIAN_POINT('Ctrl Pts',(-0.233310373291621,0.0044348431974112,
-0.0103353281859855));
#29411=CARTESIAN_POINT('Ctrl Pts',(-0.233075995771984,0.00475136497202466,
-0.010434359257892));
#29412=CARTESIAN_POINT('Ctrl Pts',(-0.232841618252347,0.00506788674663812,
-0.0105333903297984));
#29413=CARTESIAN_POINT('Ctrl Pts',(-0.232589665495774,0.00537823114335763,
-0.0106102967675239));
#29414=CARTESIAN_POINT('Ctrl Pts',(-0.232329965345587,0.00568405166373154,
-0.0106689815317353));
#29415=CARTESIAN_POINT('Ctrl Pts',(-0.232262092790211,0.00576397776384801,
-0.0106843187770383));
#29416=CARTESIAN_POINT('Ctrl Pts',(-0.232193690473423,0.0058435951715305,
-0.0106984007232942));
#29417=CARTESIAN_POINT('Ctrl Pts',(-0.232124836546004,0.00592295531648019,
-0.0107112767769113));
#29418=CARTESIAN_POINT('Ctrl Pts',(-0.231666783618184,0.00645090118840314,
-0.0107969351304606));
#29419=CARTESIAN_POINT('Ctrl Pts',(-0.231188744745006,0.0069671170222193,
-0.0108308057086929));
#29420=CARTESIAN_POINT('Ctrl Pts',(-0.230713726037419,0.00748903819150086,
-0.0108205087422449));
#29421=CARTESIAN_POINT('',(-0.234023415843097,0.0119530144195835,-0.00968754222491457));
#29422=CARTESIAN_POINT('Ctrl Pts',(-0.234023415843097,0.0119530144195835,
-0.00968754222491458));
#29423=CARTESIAN_POINT('Ctrl Pts',(-0.233998683723066,0.0118727846179345,
-0.00973406438791556));
#29424=CARTESIAN_POINT('Ctrl Pts',(-0.23397056860494,0.0117925041061299,
-0.00977883091294268));
#29425=CARTESIAN_POINT('Ctrl Pts',(-0.233939459378908,0.011712360700619,
-0.00982184594259534));
#29426=CARTESIAN_POINT('Ctrl Pts',(-0.233906531720292,0.0116275326597581,
-0.00986737533668266));
#29427=CARTESIAN_POINT('Ctrl Pts',(-0.233870251248877,0.0115428629938598,
-0.00991093971570111));
#29428=CARTESIAN_POINT('Ctrl Pts',(-0.233831092791455,0.0114585911001557,
-0.0099525457345314));
#29429=CARTESIAN_POINT('Ctrl Pts',(-0.233791934334034,0.0113743192064516,
-0.0099941517533617));
#29430=CARTESIAN_POINT('Ctrl Pts',(-0.233749898049093,0.0112904464442962,
-0.0100337987227811));
#29431=CARTESIAN_POINT('Ctrl Pts',(-0.233705465063116,0.0112072604761169,
-0.0100716075304163));
#29432=CARTESIAN_POINT('Ctrl Pts',(-0.233699173834174,0.0111954822451664,
-0.0100769608475446));
#29433=CARTESIAN_POINT('Ctrl Pts',(-0.233692834401958,0.0111837168196184,
-0.0100822762601016));
#29434=CARTESIAN_POINT('Ctrl Pts',(-0.233686447950412,0.0111719644848117,
-0.0100875538720711));
#29435=CARTESIAN_POINT('Ctrl Pts',(-0.233602623374971,0.0110177106760192,
-0.0101568245115666));
#29436=CARTESIAN_POINT('Ctrl Pts',(-0.233510718268797,0.0108657049951045,
-0.0102195982119736));
#29437=CARTESIAN_POINT('Ctrl Pts',(-0.233412688278746,0.0107154377630033,
-0.0102766354386831));
#29438=CARTESIAN_POINT('Ctrl Pts',(-0.233333564232802,0.0105941508856854,
-0.0103226725355387));
#29439=CARTESIAN_POINT('Ctrl Pts',(-0.233250441725231,0.0104739963145191,
-0.0103649693346423));
#29440=CARTESIAN_POINT('Ctrl Pts',(-0.233164241243107,0.0103547247161384,
-0.0104038910053084));
#29441=CARTESIAN_POINT('Ctrl Pts',(-0.233148078652709,0.010332361291442,
-0.0104111888185583));
#29442=CARTESIAN_POINT('Ctrl Pts',(-0.233131807676021,0.0103100289856585,
-0.0104183679101736));
#29443=CARTESIAN_POINT('Ctrl Pts',(-0.233115434172931,0.0102877262655216,
-0.0104254306152962));
#29444=CARTESIAN_POINT('Ctrl Pts',(-0.233100084013784,0.0102668174653932,
-0.0104320519013487));
#29445=CARTESIAN_POINT('Ctrl Pts',(-0.233084643742608,0.0102459346686751,
-0.0104385708941842));
#29446=CARTESIAN_POINT('Ctrl Pts',(-0.233069118157046,0.0102250766398245,
-0.0104449895109426));
#29447=CARTESIAN_POINT('Ctrl Pts',(-0.233060689266457,0.0102137527485372,
-0.0104484741987291));
#29448=CARTESIAN_POINT('Ctrl Pts',(-0.23305223484736,0.0102024356442983,
-0.0104519294538125));
#29449=CARTESIAN_POINT('Ctrl Pts',(-0.233043755972735,0.0101911255930563,
-0.0104553555826644));
#29450=CARTESIAN_POINT('Ctrl Pts',(-0.232817970043332,0.00988994760137852,
-0.0105465907667275));
#29451=CARTESIAN_POINT('Ctrl Pts',(-0.232574738474408,0.00959387094466128,
-0.0106170019038402));
#29452=CARTESIAN_POINT('Ctrl Pts',(-0.232325841945328,0.00930178982792201,
-0.0106719485881545));
#29453=CARTESIAN_POINT('Ctrl Pts',(-0.232311113206488,0.00928450559135841,
-0.010675200121498));
#29454=CARTESIAN_POINT('Ctrl Pts',(-0.232296365216068,0.00926723529665681,
-0.0106783970891451));
#29455=CARTESIAN_POINT('Ctrl Pts',(-0.232281599593838,0.00924997750557925,
-0.0106815404822746));
#29456=CARTESIAN_POINT('Ctrl Pts',(-0.232165449998461,0.00911422396810377,
-0.0107062670961898));
#29457=CARTESIAN_POINT('Ctrl Pts',(-0.232048211199567,0.00897924268871302,
-0.0107276812960103));
#29458=CARTESIAN_POINT('Ctrl Pts',(-0.231930153270517,0.00884477586957425,
-0.0107458524092826));
#29459=CARTESIAN_POINT('Ctrl Pts',(-0.231530959771025,0.008390098402932,
-0.0108072950447345));
#29460=CARTESIAN_POINT('Ctrl Pts',(-0.231122467023115,0.00794125511677842,
-0.010831736494172));
#29461=CARTESIAN_POINT('Ctrl Pts',(-0.230713724481977,0.00748904929732134,
-0.0108219320073967));
#29462=CARTESIAN_POINT('',(-0.231901468479132,0.0119424667401788,-0.00964990277379924));
#29463=CARTESIAN_POINT('Ctrl Pts',(-0.234023433762422,0.0119524819221575,
-0.00968663343302877));
#29464=CARTESIAN_POINT('Ctrl Pts',(-0.233316123319583,0.0119489346689107,
-0.00967403592336861));
#29465=CARTESIAN_POINT('Ctrl Pts',(-0.232608812875373,0.0119453877511959,
-0.00966143839039684));
#29466=CARTESIAN_POINT('Ctrl Pts',(-0.231901502429748,0.0119418411715371,
-0.00964884083595424));
#29467=CARTESIAN_POINT('',(-0.229385993393222,0.00897975235454292,-0.0106669748894047));
#29468=CARTESIAN_POINT('Ctrl Pts',(-0.229385993393222,0.00897975235454292,
-0.0106669748894047));
#29469=CARTESIAN_POINT('Ctrl Pts',(-0.229637801997236,0.00925253156900348,
-0.0106263784371995));
#29470=CARTESIAN_POINT('Ctrl Pts',(-0.230143566989202,0.00979324393307198,
-0.0105200797848502));
#29471=CARTESIAN_POINT('Ctrl Pts',(-0.230877045355225,0.0106009051517507,
-0.0102792296753082));
#29472=CARTESIAN_POINT('Ctrl Pts',(-0.231476239279836,0.0113059241165943,
-0.00998938196234091));
#29473=CARTESIAN_POINT('Ctrl Pts',(-0.231800050197011,0.0117639008386206,
-0.00975185034792822));
#29474=CARTESIAN_POINT('Ctrl Pts',(-0.231901468479132,0.0119424667401788,
-0.00964990277379923));
#29475=CARTESIAN_POINT('',(-0.227310930575325,0.0119192283365604,-0.00956777733553798));
#29476=CARTESIAN_POINT('Ctrl Pts',(-0.229385995664121,0.00897975213139759,
-0.0106669749755967));
#29477=CARTESIAN_POINT('Ctrl Pts',(-0.229355006960483,0.0090179060614615,
-0.0106598121462576));
#29478=CARTESIAN_POINT('Ctrl Pts',(-0.2293240394562,0.00905602083052721,
-0.0106524155099456));
#29479=CARTESIAN_POINT('Ctrl Pts',(-0.229293106141903,0.0090941017672963,
-0.0106447797757962));
#29480=CARTESIAN_POINT('Ctrl Pts',(-0.229177106213288,0.00923690528018039,
-0.010616145772736));
#29481=CARTESIAN_POINT('Ctrl Pts',(-0.229061589290613,0.00937923436170777,
-0.0105841480216996));
#29482=CARTESIAN_POINT('Ctrl Pts',(-0.228947224677079,0.00952135862731606,
-0.0105485174003977));
#29483=CARTESIAN_POINT('Ctrl Pts',(-0.228861451216929,0.00962795182652228,
-0.0105217944344212));
#29484=CARTESIAN_POINT('Ctrl Pts',(-0.228776325494406,0.00973442928749065,
-0.0104930283924105));
#29485=CARTESIAN_POINT('Ctrl Pts',(-0.22869211714611,0.00984090006277285,
-0.0104621132231097));
#29486=CARTESIAN_POINT('Ctrl Pts',(-0.228679702108351,0.00985659730327293,
-0.0104575553259184));
#29487=CARTESIAN_POINT('Ctrl Pts',(-0.228667307031986,0.00987229430785859,
-0.0104529506167934));
#29488=CARTESIAN_POINT('Ctrl Pts',(-0.228654932681678,0.00988799157762058,
-0.0104482989585942));
#29489=CARTESIAN_POINT('Ctrl Pts',(-0.228635832391485,0.00991222092301825,
-0.0104411189435412));
#29490=CARTESIAN_POINT('Ctrl Pts',(-0.228616781482349,0.00993645090019369,
-0.010433827071427));
#29491=CARTESIAN_POINT('Ctrl Pts',(-0.228597784506831,0.00996068343972998,
-0.0104264214928838));
#29492=CARTESIAN_POINT('Ctrl Pts',(-0.228378653761545,0.0102402065903429,
-0.010340997897746));
#29493=CARTESIAN_POINT('Ctrl Pts',(-0.228166673055731,0.0105201209803018,
-0.0102404785070309));
#29494=CARTESIAN_POINT('Ctrl Pts',(-0.227968690415889,0.0108036788995433,
-0.0101224755697179));
#29495=CARTESIAN_POINT('Ctrl Pts',(-0.22796299351652,0.0108118382054919,
-0.0101190800656497));
#29496=CARTESIAN_POINT('Ctrl Pts',(-0.227957308339109,0.0108200003027273,
-0.0101156700705878));
#29497=CARTESIAN_POINT('Ctrl Pts',(-0.227951635015369,0.0108281652984639,
-0.0101122454794729));
#29498=CARTESIAN_POINT('Ctrl Pts',(-0.227850485459292,0.0109737388161945,
-0.0100511885247029));
#29499=CARTESIAN_POINT('Ctrl Pts',(-0.227753100523097,0.011120233530301,
-0.0099854970956529));
#29500=CARTESIAN_POINT('Ctrl Pts',(-0.227661892781027,0.011267846672996,
-0.00991438783483416));
#29501=CARTESIAN_POINT('Ctrl Pts',(-0.227565569336343,0.0114237392108692,
-0.00983929016444434));
#29502=CARTESIAN_POINT('Ctrl Pts',(-0.227476121499233,0.0115808747436384,
-0.00975815798534802));
#29503=CARTESIAN_POINT('Ctrl Pts',(-0.227396458999089,0.0117396983195354,
-0.00967000980079083));
#29504=CARTESIAN_POINT('Ctrl Pts',(-0.227386884764274,0.0117587865254929,
-0.00965941571428886));
#29505=CARTESIAN_POINT('Ctrl Pts',(-0.227377452040833,0.0117778998428984,
-0.00964872059403839));
#29506=CARTESIAN_POINT('Ctrl Pts',(-0.227368166621285,0.0117970380862449,
-0.00963792287468519));
#29507=CARTESIAN_POINT('Ctrl Pts',(-0.227348451517957,0.0118376730239714,
-0.00961499680746148));
#29508=CARTESIAN_POINT('Ctrl Pts',(-0.227329400560137,0.0118784203858247,
-0.00959160817866039));
#29509=CARTESIAN_POINT('Ctrl Pts',(-0.227310930575325,0.0119192283365604,
-0.00956777733553797));
#29510=CARTESIAN_POINT('',(-0.225106030640403,0.0119077779586431,-0.00952780946947742));
#29511=CARTESIAN_POINT('Ctrl Pts',(-0.227310944993972,0.0119188280769467,
-0.00956708041891526));
#29512=CARTESIAN_POINT('Ctrl Pts',(-0.226575973544427,0.0119151443323247,
-0.00955399012063065));
#29513=CARTESIAN_POINT('Ctrl Pts',(-0.225841002093253,0.0119114609586129,
-0.00954089980346294));
#29514=CARTESIAN_POINT('Ctrl Pts',(-0.225106030640403,0.0119077779586431,
-0.00952780946947742));
#29515=CARTESIAN_POINT('',(-0.22509230219787,0.00750490891545138,-0.0106935438270112));
#29516=CARTESIAN_POINT('Ctrl Pts',(-0.225106030640403,0.0119077779586431,
-0.00952780946947742));
#29517=CARTESIAN_POINT('Ctrl Pts',(-0.225003294965764,0.0112735761688805,
-0.00988629126619056));
#29518=CARTESIAN_POINT('Ctrl Pts',(-0.224964958507158,0.0105924278097438,
-0.0101704206208673));
#29519=CARTESIAN_POINT('Ctrl Pts',(-0.224967573052356,0.0098852358922856,
-0.0103667934727557));
#29520=CARTESIAN_POINT('Ctrl Pts',(-0.224967640189741,0.00986707632239798,
-0.0103718360169928));
#29521=CARTESIAN_POINT('Ctrl Pts',(-0.224967734329484,0.00984889964653936,
-0.0103768207544314));
#29522=CARTESIAN_POINT('Ctrl Pts',(-0.224967855074635,0.00983070628477451,
-0.010381747639153));
#29523=CARTESIAN_POINT('Ctrl Pts',(-0.224972881642603,0.00907332457073518,
-0.0105868517009247));
#29524=CARTESIAN_POINT('Ctrl Pts',(-0.225024020919892,0.00828816777677607,
-0.0106912747006324));
#29525=CARTESIAN_POINT('Ctrl Pts',(-0.22509230219787,0.00750490891545138,
-0.0106935438270112));
#29526=CARTESIAN_POINT('',(-0.22512339082026,0.00302752783129386,-0.00949179287466226));
#29527=CARTESIAN_POINT('Ctrl Pts',(-0.225092302193471,0.00750490886465332,
-0.010693543826959));
#29528=CARTESIAN_POINT('Ctrl Pts',(-0.225046870204233,0.00698064601573159,
-0.0106930042825971));
#29529=CARTESIAN_POINT('Ctrl Pts',(-0.225008961521983,0.00645533295426021,
-0.0106467019987212));
#29530=CARTESIAN_POINT('Ctrl Pts',(-0.224987521850832,0.0059382751191565,
-0.0105541685444992));
#29531=CARTESIAN_POINT('Ctrl Pts',(-0.224976996951193,0.00568444744690854,
-0.0105087431593767));
#29532=CARTESIAN_POINT('Ctrl Pts',(-0.224970440928504,0.00543260917693936,
-0.0104521853841945));
#29533=CARTESIAN_POINT('Ctrl Pts',(-0.224968912294139,0.00518375239436985,
-0.010384946549299));
#29534=CARTESIAN_POINT('Ctrl Pts',(-0.224964269823687,0.00442797306195466,
-0.0101807418608635));
#29535=CARTESIAN_POINT('Ctrl Pts',(-0.225005941234088,0.00370066390407666,
-0.00987820272963985));
#29536=CARTESIAN_POINT('Ctrl Pts',(-0.22512331575626,0.00302780787790367,
-0.00949128794938887));
#29537=CARTESIAN_POINT('',(-0.225017273462258,0.00228350670705836,-0.00900753387751742));
#29538=CARTESIAN_POINT('Ctrl Pts',(-0.225016552084744,0.00228362488138197,
-0.00900760247763402));
#29539=CARTESIAN_POINT('Ctrl Pts',(-0.22504874328166,0.00240252866617142,
-0.00909390486499722));
#29540=CARTESIAN_POINT('Ctrl Pts',(-0.225073793197746,0.00252475423756348,
-0.00917795515386039));
#29541=CARTESIAN_POINT('Ctrl Pts',(-0.225101157805034,0.00271695196711039,
-0.00930284738549845));
#29542=CARTESIAN_POINT('Ctrl Pts',(-0.225108617894573,0.00278472801619829,
-0.00934556621454342));
#29543=CARTESIAN_POINT('Ctrl Pts',(-0.225118522059823,0.00291094688437005,
-0.00942268118093157));
#29544=CARTESIAN_POINT('Ctrl Pts',(-0.225121568541063,0.00296915254795865,
-0.00945731247850366));
#29545=CARTESIAN_POINT('Ctrl Pts',(-0.22512312969261,0.00302779944139895,
-0.00949127923732032));
#29546=CARTESIAN_POINT('',(-0.225277037624834,0.00232818316358624,-0.00904462761620701));
#29547=CARTESIAN_POINT('Ctrl Pts',(-0.225276566204441,0.00232796030677252,
-0.00904445642067167));
#29548=CARTESIAN_POINT('Ctrl Pts',(-0.22523775196089,0.00230950230683335,
-0.00903055888584819));
#29549=CARTESIAN_POINT('Ctrl Pts',(-0.225195493315447,0.00229628530974549,
-0.00902022639715284));
#29550=CARTESIAN_POINT('Ctrl Pts',(-0.225107254455047,0.00228121212563282,
-0.00900764771093501));
#29551=CARTESIAN_POINT('Ctrl Pts',(-0.225061856391577,0.00227945979119184,
-0.00900548999868191));
#29552=CARTESIAN_POINT('Ctrl Pts',(-0.225016908981005,0.00228354087081739,
-0.00900754894665053));
#29553=CARTESIAN_POINT('',(-0.225398032236364,0.00187965741570819,-0.00870574455337625));
#29554=CARTESIAN_POINT('Ctrl Pts',(-0.225398012644317,0.00187968458752203,
-0.00870571095552509));
#29555=CARTESIAN_POINT('Ctrl Pts',(-0.225377108190577,0.00195288094167168,
-0.00876479409570467));
#29556=CARTESIAN_POINT('Ctrl Pts',(-0.225356430217593,0.00202706411817278,
-0.00882273457646027));
#29557=CARTESIAN_POINT('Ctrl Pts',(-0.225315794003022,0.00217643669042039,
-0.00893557398364217));
#29558=CARTESIAN_POINT('Ctrl Pts',(-0.225295825541299,0.00225161976744987,
-0.00899051371721635));
#29559=CARTESIAN_POINT('Ctrl Pts',(-0.225276087777197,0.0023277455613394,
-0.00904429419962185));
#29560=CARTESIAN_POINT('',(-0.226396396172104,0.00188100664625559,-0.00872574966728709));
#29561=CARTESIAN_POINT('Ctrl Pts',(-0.225398022753316,0.00187968462648945,
-0.00870571117852498));
#29562=CARTESIAN_POINT('Ctrl Pts',(-0.225564669450736,0.00187995036891675,
-0.00870908127754952));
#29563=CARTESIAN_POINT('Ctrl Pts',(-0.225731316227715,0.00188021543557644,
-0.00871245219588737));
#29564=CARTESIAN_POINT('Ctrl Pts',(-0.226064095893355,0.00188074340384874,
-0.00871918526255622));
#29565=CARTESIAN_POINT('Ctrl Pts',(-0.226230228908158,0.00188100630981627,
-0.00872254740843019));
#29566=CARTESIAN_POINT('Ctrl Pts',(-0.226396361723287,0.00188126854571656,
-0.00872591035494955));
#29567=CARTESIAN_POINT('',(-0.226275854855421,0.00233713586297991,-0.0090706994431196));
#29568=CARTESIAN_POINT('Ctrl Pts',(-0.226275826299596,0.00233714530094412,
-0.00907068034054895));
#29569=CARTESIAN_POINT('Ctrl Pts',(-0.226295295393397,0.00225911649706514,
-0.00901557814944029));
#29570=CARTESIAN_POINT('Ctrl Pts',(-0.22631507768356,0.00218209886260719,
-0.00895927286362518));
#29571=CARTESIAN_POINT('Ctrl Pts',(-0.226355247076649,0.0020301452459405,
-0.00884433828949768));
#29572=CARTESIAN_POINT('Ctrl Pts',(-0.226375636754673,0.00195519562172708,
-0.00878570253700721));
#29573=CARTESIAN_POINT('Ctrl Pts',(-0.226396330981692,0.00188126708771283,
-0.00872590858518578));
#29574=CARTESIAN_POINT('',(-0.227050813062771,0.00230629182834679,-0.00906389588700253));
#29575=CARTESIAN_POINT('Ctrl Pts',(-0.227050802694897,0.00230590961093097,
-0.00906362093448274));
#29576=CARTESIAN_POINT('Ctrl Pts',(-0.226921324130421,0.00229945469111778,
-0.0090564308441887));
#29577=CARTESIAN_POINT('Ctrl Pts',(-0.226791421429502,0.00229884660704338,
-0.00905343747495934));
#29578=CARTESIAN_POINT('Ctrl Pts',(-0.226532505026649,0.00230931135191709,
-0.0090558621977966));
#29579=CARTESIAN_POINT('Ctrl Pts',(-0.226403693609709,0.00232032762959314,
-0.00906124325580749));
#29580=CARTESIAN_POINT('Ctrl Pts',(-0.226275841324095,0.00233714970144879,
-0.00907068376606783));
#29581=CARTESIAN_POINT('',(-0.229392048724075,0.00598507781155818,-0.0106610739775155));
#29582=CARTESIAN_POINT('Ctrl Pts',(-0.229392039407141,0.00598506674127622,
-0.0106610718294251));
#29583=CARTESIAN_POINT('Ctrl Pts',(-0.229376263879727,0.00596635918551221,
-0.0106574720776792));
#29584=CARTESIAN_POINT('Ctrl Pts',(-0.229360518248087,0.00594764474891851,
-0.0106538089624593));
#29585=CARTESIAN_POINT('Ctrl Pts',(-0.229344803135537,0.00592892334569771,
-0.0106500820381302));
#29586=CARTESIAN_POINT('Ctrl Pts',(-0.228860120685564,0.00535152146254403,
-0.0105351369616001));
#29587=CARTESIAN_POINT('Ctrl Pts',(-0.22840446889792,0.00476672800595227,
-0.0103604760517174));
#29588=CARTESIAN_POINT('Ctrl Pts',(-0.227996133929565,0.00417509627566239,
-0.0101124588811835));
#29589=CARTESIAN_POINT('Ctrl Pts',(-0.227785346616275,0.00386968901801932,
-0.00998442950070386));
#29590=CARTESIAN_POINT('Ctrl Pts',(-0.227587167224861,0.00356238788559785,
-0.00983691076309596));
#29591=CARTESIAN_POINT('Ctrl Pts',(-0.227429976757087,0.00324829610005773,
-0.0096628079242218));
#29592=CARTESIAN_POINT('Ctrl Pts',(-0.227272786289312,0.0029342043145176,
-0.00948870508534763));
#29593=CARTESIAN_POINT('Ctrl Pts',(-0.227156605059703,0.00261384836770206,
-0.00928704688478299));
#29594=CARTESIAN_POINT('Ctrl Pts',(-0.227050813062771,0.00230629182834679,
-0.00906389588700253));
#29595=CARTESIAN_POINT('',(-0.225010431372201,-0.00147369574979845,-8.4492836099348E-8));
#29596=CARTESIAN_POINT('Ctrl Pts',(-0.229392050505309,0.00598507587768533,
-0.0106610736635327));
#29597=CARTESIAN_POINT('Ctrl Pts',(-0.229409546005236,0.00596627858890805,
-0.0106582040682476));
#29598=CARTESIAN_POINT('Ctrl Pts',(-0.229427042810866,0.00594748970466014,
-0.0106552720634706));
#29599=CARTESIAN_POINT('Ctrl Pts',(-0.229444539825254,0.00592870925509559,
-0.0106522774653289));
#29600=CARTESIAN_POINT('Ctrl Pts',(-0.229679303096811,0.00567672570617227,
-0.0106120979443468));
#29601=CARTESIAN_POINT('Ctrl Pts',(-0.229914103960048,0.00542625026694678,
-0.0105606753677848));
#29602=CARTESIAN_POINT('Ctrl Pts',(-0.230146292910576,0.00517731697708083,
-0.0104978578559838));
#29603=CARTESIAN_POINT('Ctrl Pts',(-0.230395787010163,0.00490983057485797,
-0.0104303585261942));
#29604=CARTESIAN_POINT('Ctrl Pts',(-0.230642262773844,0.00464408630644996,
-0.0103498209007954));
#29605=CARTESIAN_POINT('Ctrl Pts',(-0.230880984377476,0.0043769207193843,
-0.0102539772995695));
#29606=CARTESIAN_POINT('Ctrl Pts',(-0.231119705981108,0.00410975513231864,
-0.0101581336983435));
#29607=CARTESIAN_POINT('Ctrl Pts',(-0.231350667696974,0.00384106818221418,
-0.0100472466834519));
#29608=CARTESIAN_POINT('Ctrl Pts',(-0.231558063831141,0.00356208088917226,
-0.00991289510667101));
#29609=CARTESIAN_POINT('Ctrl Pts',(-0.231661761898224,0.00342258724265129,
-0.00984571931828055));
#29610=CARTESIAN_POINT('Ctrl Pts',(-0.231759570505304,0.00328056322625301,
-0.00977258639660185));
#29611=CARTESIAN_POINT('Ctrl Pts',(-0.231847603316042,0.00313610180678418,
-0.00969249586807556));
#29612=CARTESIAN_POINT('Ctrl Pts',(-0.23193563612678,0.00299164038731536,
-0.00961240533954928));
#29613=CARTESIAN_POINT('Ctrl Pts',(-0.232013892448937,0.00284472310488733,
-0.00952539034512403));
#29614=CARTESIAN_POINT('Ctrl Pts',(-0.232068608495672,0.00269412255633174,
-0.00942902364866202));
#29615=CARTESIAN_POINT('Ctrl Pts',(-0.232120424438827,0.00255150425825015,
-0.00933776465675944));
#29616=CARTESIAN_POINT('Ctrl Pts',(-0.232151133097279,0.00240569654018845,
-0.00923795022913459));
#29617=CARTESIAN_POINT('Ctrl Pts',(-0.232149401495556,0.00226371239656172,
-0.00913346945015538));
#29618=CARTESIAN_POINT('Ctrl Pts',(-0.232149304578969,0.00225576563928716,
-0.00912762173104255));
#29619=CARTESIAN_POINT('Ctrl Pts',(-0.232149106041286,0.00224783059372626,
-0.00912175980534219));
#29620=CARTESIAN_POINT('Ctrl Pts',(-0.232148803895588,0.00223990837733705,
-0.00911588451784818));
#29621=CARTESIAN_POINT('Ctrl Pts',(-0.232143103334322,0.0020904404875636,
-0.00900503588908099));
#29622=CARTESIAN_POINT('Ctrl Pts',(-0.232100523054338,0.00194565874238837,
-0.00888922979231711));
#29623=CARTESIAN_POINT('Ctrl Pts',(-0.232032441227186,0.00181413122320368,
-0.00877725833061356));
#29624=CARTESIAN_POINT('Ctrl Pts',(-0.231896277572882,0.00155107618483428,
-0.00855331540720646));
#29625=CARTESIAN_POINT('Ctrl Pts',(-0.231658075269179,0.00133961295871075,
-0.00834641499925663));
#29626=CARTESIAN_POINT('Ctrl Pts',(-0.231405343490951,0.00115220259560978,
-0.00814850811062457));
#29627=CARTESIAN_POINT('Ctrl Pts',(-0.231235832079804,0.0010265033450625,
-0.008015768665657));
#29628=CARTESIAN_POINT('Ctrl Pts',(-0.231059787339919,0.000911927967415083,
-0.0078867987552611));
#29629=CARTESIAN_POINT('Ctrl Pts',(-0.230879468894514,0.000803917031338677,
-0.00775865188729638));
#29630=CARTESIAN_POINT('Ctrl Pts',(-0.230790942894308,0.000750889865271893,
-0.00769573913516824));
#29631=CARTESIAN_POINT('Ctrl Pts',(-0.230701386819548,0.000699459349445356,
-0.00763300839578708));
#29632=CARTESIAN_POINT('Ctrl Pts',(-0.230611068015914,0.000649165936946226,
-0.00757003102247231));
#29633=CARTESIAN_POINT('Ctrl Pts',(-0.230336779008904,0.000496429965935362,
-0.0073787751544178));
#29634=CARTESIAN_POINT('Ctrl Pts',(-0.230055458506837,0.000354017033221105,
-0.00718541546478645));
#29635=CARTESIAN_POINT('Ctrl Pts',(-0.229779396359619,0.000216017613201449,
-0.00698219836546261));
#29636=CARTESIAN_POINT('Ctrl Pts',(-0.229406479577426,2.96019811534319E-5,
-0.00670768384932898));
#29637=CARTESIAN_POINT('Ctrl Pts',(-0.229043158402296,-0.000148388160636376,
-0.00641509596421757));
#29638=CARTESIAN_POINT('Ctrl Pts',(-0.228694312977108,-0.000315100219245054,
-0.0061008569866271));
#29639=CARTESIAN_POINT('Ctrl Pts',(-0.228526673107328,-0.000395214750719274,
-0.0059498474635566));
#29640=CARTESIAN_POINT('Ctrl Pts',(-0.228362376180949,-0.000472687651889521,
-0.00579383237136698));
#29641=CARTESIAN_POINT('Ctrl Pts',(-0.228201963842599,-0.000547120768336193,
-0.0056324340965861));
#29642=CARTESIAN_POINT('Ctrl Pts',(-0.227783575331477,-0.000741257709973661,
-0.00521147405961152));
#29643=CARTESIAN_POINT('Ctrl Pts',(-0.227391619436755,-0.000914758282893851,
-0.00475369881014943));
#29644=CARTESIAN_POINT('Ctrl Pts',(-0.227033139047913,-0.00105503991125543,
-0.00426160731172168));
#29645=CARTESIAN_POINT('Ctrl Pts',(-0.226968167554637,-0.00108046475221651,
-0.00417241995175197));
#29646=CARTESIAN_POINT('Ctrl Pts',(-0.226904295686128,-0.00110479407840349,
-0.00408211404554795));
#29647=CARTESIAN_POINT('Ctrl Pts',(-0.226841565329479,-0.00112789199908747,
-0.00399070722071771));
#29648=CARTESIAN_POINT('Ctrl Pts',(-0.226687811436992,-0.00118450566116707,
-0.00376666648720267));
#29649=CARTESIAN_POINT('Ctrl Pts',(-0.226540910396871,-0.00123373203013407,
-0.00353600918100793));
#29650=CARTESIAN_POINT('Ctrl Pts',(-0.226401689603115,-0.00127337073319176,
-0.00329931260295964));
#29651=CARTESIAN_POINT('Ctrl Pts',(-0.226355810163533,-0.00128643344769723,
-0.00322131055988149));
#29652=CARTESIAN_POINT('Ctrl Pts',(-0.226310764792651,-0.00129845243507264,
-0.00314265391460194));
#29653=CARTESIAN_POINT('Ctrl Pts',(-0.226266583240457,-0.00130952028889418,
-0.00306340421519403));
#29654=CARTESIAN_POINT('Ctrl Pts',(-0.226131996169734,-0.00134323549243618,
-0.00282199158097784));
#29655=CARTESIAN_POINT('Ctrl Pts',(-0.226005438708994,-0.00136810837940549,
-0.00257479103062637));
#29656=CARTESIAN_POINT('Ctrl Pts',(-0.225887620499229,-0.00138725794483737,
-0.00232303363175134));
#29657=CARTESIAN_POINT('Ctrl Pts',(-0.225849397642494,-0.0013934704912468,
-0.00224135791279094));
#29658=CARTESIAN_POINT('Ctrl Pts',(-0.225812094598808,-0.001399086557685,
-0.00215920486363162));
#29659=CARTESIAN_POINT('Ctrl Pts',(-0.225775735920245,-0.0014042208063698,
-0.00207661730214151));
#29660=CARTESIAN_POINT('Ctrl Pts',(-0.225671099200072,-0.00141899667183484,
-0.0018389383791714));
#29661=CARTESIAN_POINT('Ctrl Pts',(-0.22557429520518,-0.00142977098012393,
-0.00159650160034879));
#29662=CARTESIAN_POINT('Ctrl Pts',(-0.225482531299466,-0.00143967792564172,
-0.00135284436013466));
#29663=CARTESIAN_POINT('Ctrl Pts',(-0.225363801815749,-0.00145249610853613,
-0.00103758643699353));
#29664=CARTESIAN_POINT('Ctrl Pts',(-0.225253510359594,-0.00146400674691899,
-0.000720357869132175));
#29665=CARTESIAN_POINT('Ctrl Pts',(-0.225145577164679,-0.00146962404402618,
-0.000401845801342884));
#29666=CARTESIAN_POINT('Ctrl Pts',(-0.225100262802465,-0.00147198239389232,
-0.000268122610615833));
#29667=CARTESIAN_POINT('Ctrl Pts',(-0.225055364062672,-0.00147329937223217,
-0.000134167155556775));
#29668=CARTESIAN_POINT('Ctrl Pts',(-0.22501043137218,-0.00147369574980066,
-8.44936689116393E-8));
#29669=CARTESIAN_POINT('',(-0.229322739274083,0.00603943600898884,0.0106683693245468));
#29670=CARTESIAN_POINT('Ctrl Pts',(-0.225010431372201,-0.00147369574979845,
-8.4492836099348E-8));
#29671=CARTESIAN_POINT('Ctrl Pts',(-0.225177252440418,-0.00146995924473084,
0.000502352857987205));
#29672=CARTESIAN_POINT('Ctrl Pts',(-0.225343589262149,-0.00145323503816418,
0.00100315816743078));
#29673=CARTESIAN_POINT('Ctrl Pts',(-0.225531292866178,-0.00143309616656037,
0.0014982458852503));
#29674=CARTESIAN_POINT('Ctrl Pts',(-0.225602322658008,-0.00142547532270333,
0.00168559432598046));
#29675=CARTESIAN_POINT('Ctrl Pts',(-0.225676411832131,-0.00141733572264945,
0.00187209120885228));
#29676=CARTESIAN_POINT('Ctrl Pts',(-0.225754737956661,-0.00140663385766833,
0.00205601235174846));
#29677=CARTESIAN_POINT('Ctrl Pts',(-0.225814245385663,-0.00139850323108151,
0.00219574445796982));
#29678=CARTESIAN_POINT('Ctrl Pts',(-0.225876191803857,-0.00138888392204247,
0.00233442708897512));
#29679=CARTESIAN_POINT('Ctrl Pts',(-0.225940507472793,-0.00137697898725081,
0.00247173089544256));
#29680=CARTESIAN_POINT('Ctrl Pts',(-0.226030373988067,-0.00136034454929846,
0.00266358172783048));
#29681=CARTESIAN_POINT('Ctrl Pts',(-0.226124866188928,-0.00133925282069762,
0.00285274028170326));
#29682=CARTESIAN_POINT('Ctrl Pts',(-0.226223799860628,-0.00131321549610233,
0.00303878544699706));
#29683=CARTESIAN_POINT('Ctrl Pts',(-0.226296987449779,-0.00129395401533097,
0.00317641500109331));
#29684=CARTESIAN_POINT('Ctrl Pts',(-0.226372601929934,-0.00127197872634538,
0.00331241011184743));
#29685=CARTESIAN_POINT('Ctrl Pts',(-0.226450485602142,-0.00124712787546466,
0.00344657465293664));
#29686=CARTESIAN_POINT('Ctrl Pts',(-0.226553231728801,-0.00121434399920691,
0.0036235679371649));
#29687=CARTESIAN_POINT('Ctrl Pts',(-0.226659927062532,-0.00117656292596665,
0.00379737392109265));
#29688=CARTESIAN_POINT('Ctrl Pts',(-0.226770209885917,-0.00113435563325404,
0.00396775128429173));
#29689=CARTESIAN_POINT('Ctrl Pts',(-0.227084864123454,-0.00101393158987724,
0.00445386469402914));
#29690=CARTESIAN_POINT('Ctrl Pts',(-0.22742875305635,-0.000857717907044796,
0.00491155504123866));
#29691=CARTESIAN_POINT('Ctrl Pts',(-0.227796711941448,-0.000677481753928545,
0.00533797868158574));
#29692=CARTESIAN_POINT('Ctrl Pts',(-0.227882201087694,-0.000635606872041938,
0.00543705114437668));
#29693=CARTESIAN_POINT('Ctrl Pts',(-0.227968989504244,-0.000592426211065234,
0.00553444710419628));
#29694=CARTESIAN_POINT('Ctrl Pts',(-0.22805701242935,-0.000548074565095271,
0.00563015386475785));
#29695=CARTESIAN_POINT('Ctrl Pts',(-0.228523900026839,-0.000312826379389474,
0.00613779774785378));
#29696=CARTESIAN_POINT('Ctrl Pts',(-0.229025501740472,-4.52917149988218E-5,
0.00659807131512971));
#29697=CARTESIAN_POINT('Ctrl Pts',(-0.229547710152002,0.000243359606321602,
0.00701769548210368));
#29698=CARTESIAN_POINT('Ctrl Pts',(-0.229573852617382,0.000257809885190769,
0.0070387024402748));
#29699=CARTESIAN_POINT('Ctrl Pts',(-0.229600046729066,0.000272313997292378,
0.00705960636108304));
#29700=CARTESIAN_POINT('Ctrl Pts',(-0.229626281725718,0.000286875865311344,
0.00708041461571968));
#29701=CARTESIAN_POINT('Ctrl Pts',(-0.22986207511333,0.000417754181617712,
0.00726743384488521));
#29702=CARTESIAN_POINT('Ctrl Pts',(-0.230101171205871,0.00055316050312438,
0.00744682385458936));
#29703=CARTESIAN_POINT('Ctrl Pts',(-0.230335756719716,0.000696783137501262,
0.00762332499975972));
#29704=CARTESIAN_POINT('Ctrl Pts',(-0.23059644283898,0.000856385606470733,
0.00781946412969107));
#29705=CARTESIAN_POINT('Ctrl Pts',(-0.230851556648128,0.00102597288099953,
0.00801218706259676));
#29706=CARTESIAN_POINT('Ctrl Pts',(-0.231094258515009,0.00121676345105936,
0.00820928893198079));
#29707=CARTESIAN_POINT('Ctrl Pts',(-0.23124674716807,0.00133663643522354,
0.00833312728132895));
#29708=CARTESIAN_POINT('Ctrl Pts',(-0.231394333661979,0.00146485790708328,
0.00845863327908963));
#29709=CARTESIAN_POINT('Ctrl Pts',(-0.231520723189712,0.00160723465436361,
0.00858829560130594));
#29710=CARTESIAN_POINT('Ctrl Pts',(-0.231595496002384,0.0016914656032734,
0.00866500461908271));
#29711=CARTESIAN_POINT('Ctrl Pts',(-0.231662849914153,0.00178067265894138,
0.00874314135189989));
#29712=CARTESIAN_POINT('Ctrl Pts',(-0.231719410813792,0.00187621923147606,
0.0088229581342544));
#29713=CARTESIAN_POINT('Ctrl Pts',(-0.231795494102225,0.0020047443695707,
0.00893032423543671));
#29714=CARTESIAN_POINT('Ctrl Pts',(-0.231852053675257,0.00214485369195234,
0.00904062598124823));
#29715=CARTESIAN_POINT('Ctrl Pts',(-0.231875572818194,0.00229222206788661,
0.00914846641581533));
#29716=CARTESIAN_POINT('Ctrl Pts',(-0.23189909196113,0.00243959044382088,
0.00925630685038242));
#29717=CARTESIAN_POINT('Ctrl Pts',(-0.231889572375894,0.00259430357999544,
0.00936159342295822));
#29718=CARTESIAN_POINT('Ctrl Pts',(-0.231854413493221,0.00274641686514429,
0.00945789529503096));
#29719=CARTESIAN_POINT('Ctrl Pts',(-0.231784095727876,0.00305064343544201,
0.00965049903917647));
#29720=CARTESIAN_POINT('Ctrl Pts',(-0.23161119843415,0.00334377625563083,
0.00980825830993441));
#29721=CARTESIAN_POINT('Ctrl Pts',(-0.231414651287714,0.00362600117395275,
0.00994191747689838));
#29722=CARTESIAN_POINT('Ctrl Pts',(-0.231218104141277,0.00390822609227465,
0.0100755766438623));
#29723=CARTESIAN_POINT('Ctrl Pts',(-0.230997905530183,0.00417947979400734,
0.0101852181167744));
#29724=CARTESIAN_POINT('Ctrl Pts',(-0.230768518905705,0.00444690860942094,
0.0102788235291743));
#29725=CARTESIAN_POINT('Ctrl Pts',(-0.230580860432451,0.0046656889472835,
0.0103554010053859));
#29726=CARTESIAN_POINT('Ctrl Pts',(-0.230387055372245,0.0048819763870309,
0.0104210919474471));
#29727=CARTESIAN_POINT('Ctrl Pts',(-0.23019006072046,0.00509814736951133,
0.0104776704819747));
#29728=CARTESIAN_POINT('Ctrl Pts',(-0.230146256556025,0.00514621562505539,
0.0104902514094645));
#29729=CARTESIAN_POINT('Ctrl Pts',(-0.230102294680889,0.00519427998360542,
0.0105023779101023));
#29730=CARTESIAN_POINT('Ctrl Pts',(-0.230058207604929,0.00524236841651574,
0.0105140660125324));
#29731=CARTESIAN_POINT('Ctrl Pts',(-0.229815853576752,0.00550671857289634,
0.0105783174659109));
#29732=CARTESIAN_POINT('Ctrl Pts',(-0.229569716846853,0.00577172916293637,
0.0106294062710768));
#29733=CARTESIAN_POINT('Ctrl Pts',(-0.229322739274083,0.00603943600898884,
0.0106683693245468));
#29734=CARTESIAN_POINT('',(-0.227049077441917,0.00230637883574136,0.00906391893415159));
#29735=CARTESIAN_POINT('Ctrl Pts',(-0.227049077441917,0.00230637883574136,
0.00906391893415159));
#29736=CARTESIAN_POINT('Ctrl Pts',(-0.227073318810987,0.00238431864578963,
0.00912046235057106));
#29737=CARTESIAN_POINT('Ctrl Pts',(-0.227097908747937,0.00246328116075861,
0.00917575105202224));
#29738=CARTESIAN_POINT('Ctrl Pts',(-0.227123536768961,0.00254286828211047,
0.00922963379678905));
#29739=CARTESIAN_POINT('Ctrl Pts',(-0.227161978800496,0.00266224896413825,
0.00931045791393928));
#29740=CARTESIAN_POINT('Ctrl Pts',(-0.22720277011395,0.00278302753188814,
0.00938814177886813));
#29741=CARTESIAN_POINT('Ctrl Pts',(-0.227248074883203,0.00290385325814463,
0.00946217390253985));
#29742=CARTESIAN_POINT('Ctrl Pts',(-0.227270727267829,0.00296426612127288,
0.00949918996437571));
#29743=CARTESIAN_POINT('Ctrl Pts',(-0.227294504627205,0.00302469536767607,
0.00953528337842167));
#29744=CARTESIAN_POINT('Ctrl Pts',(-0.227319648794279,0.00308496613435269,
0.0095703826343294));
#29745=CARTESIAN_POINT('Ctrl Pts',(-0.227334570957018,0.00312073467606119,
0.00959121278579584));
#29746=CARTESIAN_POINT('Ctrl Pts',(-0.227349973334997,0.00315644549335353,
0.00961169177662436));
#29747=CARTESIAN_POINT('Ctrl Pts',(-0.227365903473589,0.00319205925221374,
0.00963181686044552));
#29748=CARTESIAN_POINT('Ctrl Pts',(-0.227376815963193,0.00321645544758186,
0.00964560297829475));
#29749=CARTESIAN_POINT('Ctrl Pts',(-0.227387975997183,0.00324080613667955,
0.00965922305709978));
#29750=CARTESIAN_POINT('Ctrl Pts',(-0.227399366335057,0.00326510564441096,
0.00967268198785667));
#29751=CARTESIAN_POINT('Ctrl Pts',(-0.22747408111678,0.00342449796765148,
0.00976096567925429));
#29752=CARTESIAN_POINT('Ctrl Pts',(-0.22755866523419,0.00358193498187751,
0.00984210870278841));
#29753=CARTESIAN_POINT('Ctrl Pts',(-0.227649842528156,0.00373843387538247,
0.0099172547990377));
#29754=CARTESIAN_POINT('Ctrl Pts',(-0.227672636851648,0.00377755859875871,
0.00993604132310003));
#29755=CARTESIAN_POINT('Ctrl Pts',(-0.227695847168838,0.00381662280291635,
0.00995445193258686));
#29756=CARTESIAN_POINT('Ctrl Pts',(-0.227719428568754,0.00385563862870273,
0.00997250248056532));
#29757=CARTESIAN_POINT('Ctrl Pts',(-0.22778372902646,0.00396202482565283,
0.0100217217169544));
#29758=CARTESIAN_POINT('Ctrl Pts',(-0.227850789121976,0.00406806057251539,
0.0100682649261601));
#29759=CARTESIAN_POINT('Ctrl Pts',(-0.227919727715055,0.00417393025766419,
0.0101124421201561));
#29760=CARTESIAN_POINT('Ctrl Pts',(-0.227926636258577,0.00418453977687389,
0.0101168692494866));
#29761=CARTESIAN_POINT('Ctrl Pts',(-0.227933563697047,0.00419514762293024,
0.0101212725626095));
#29762=CARTESIAN_POINT('Ctrl Pts',(-0.227940510167508,0.00420575413544571,
0.0101256523527859));
#29763=CARTESIAN_POINT('Ctrl Pts',(-0.228042194869883,0.00436101572828531,
0.0101897651512286));
#29764=CARTESIAN_POINT('Ctrl Pts',(-0.22814789616919,0.00451584292166484,
0.0102489334827523));
#29765=CARTESIAN_POINT('Ctrl Pts',(-0.228257151826692,0.00467012000595043,
0.0103032405028755));
#29766=CARTESIAN_POINT('Ctrl Pts',(-0.228369821723491,0.00482921824911995,
0.0103592446173776));
#29767=CARTESIAN_POINT('Ctrl Pts',(-0.228486270611578,0.00498772752812297,
0.0104100777128712));
#29768=CARTESIAN_POINT('Ctrl Pts',(-0.228605950089108,0.00514546659205433,
0.010456041453186));
#29769=CARTESIAN_POINT('Ctrl Pts',(-0.228834429091665,0.00544660480501419,
0.0105437904119689));
#29770=CARTESIAN_POINT('Ctrl Pts',(-0.229074679740743,0.00574486937382215,
0.0106139556888789));
#29771=CARTESIAN_POINT('Ctrl Pts',(-0.229322729007605,0.00603936778416517,
0.0106687795114693));
#29772=CARTESIAN_POINT('',(-0.226264593472374,0.00233548629481926,0.00906884038940272));
#29773=CARTESIAN_POINT('Ctrl Pts',(-0.226264593480196,0.00233548634321754,
0.0090688404173902));
#29774=CARTESIAN_POINT('Ctrl Pts',(-0.226394576944157,0.00231954970168914,
0.00906006960165041));
#29775=CARTESIAN_POINT('Ctrl Pts',(-0.226525406606473,0.00230915152537602,
0.00905517566549868));
#29776=CARTESIAN_POINT('Ctrl Pts',(-0.226787422427741,0.00229941738241652,
0.0090533391772081));
#29777=CARTESIAN_POINT('Ctrl Pts',(-0.226918425715393,0.00230006314209026,
0.00905638008239629));
#29778=CARTESIAN_POINT('Ctrl Pts',(-0.227049047294151,0.00230621211406783,
0.00906336897528621));
#29779=CARTESIAN_POINT('',(-0.226391079625555,0.00186369918572083,0.00871144032068667));
#29780=CARTESIAN_POINT('Origin',(-0.227683792439033,0.00776639667921597,
0.00188953853444711));
#29781=CARTESIAN_POINT('',(-0.225391399225421,0.00186320400051213,0.00869213916568744));
#29782=CARTESIAN_POINT('Ctrl Pts',(-0.225391399225484,0.00186320400486124,
0.00869213916233772));
#29783=CARTESIAN_POINT('Ctrl Pts',(-0.225558023686355,0.00186328774236531,
0.00869535478842071));
#29784=CARTESIAN_POINT('Ctrl Pts',(-0.225724648220415,0.00186337087834226,
0.00869857114170172));
#29785=CARTESIAN_POINT('Ctrl Pts',(-0.226057875023074,0.0018635359380542,
0.00870500486370907));
#29786=CARTESIAN_POINT('Ctrl Pts',(-0.226224477410293,0.00186361786200745,
0.00870822223453359));
#29787=CARTESIAN_POINT('Ctrl Pts',(-0.226391079625542,0.00186369918634654,
0.00871144032136585));
#29788=CARTESIAN_POINT('',(-0.225269616388151,0.00232397772164353,0.0090411714391037));
#29789=CARTESIAN_POINT('Origin',(-0.226735468554244,0.0077654556471817,
0.00187401233671198));
#29790=CARTESIAN_POINT('',(-0.225014720871232,0.00228334524727118,0.0090072968842552));
#29791=CARTESIAN_POINT('Ctrl Pts',(-0.225014708918058,0.00228338321464125,
0.00900698417674001));
#29792=CARTESIAN_POINT('Ctrl Pts',(-0.225058707715989,0.0022804931552636,
0.00900576569532436));
#29793=CARTESIAN_POINT('Ctrl Pts',(-0.2251029310297,0.00228252149587852,
0.00900809763828351));
#29794=CARTESIAN_POINT('Ctrl Pts',(-0.225188483608375,0.00229619488802783,
0.00901960729698031));
#29795=CARTESIAN_POINT('Ctrl Pts',(-0.225229440181929,0.00230758548139352,
0.00902859347934716));
#29796=CARTESIAN_POINT('Ctrl Pts',(-0.225267894528976,0.00232332530843618,
0.00904055895880893));
#29797=CARTESIAN_POINT('',(-0.22511807106961,0.0030194940701125,0.00948730014603764));
#29798=CARTESIAN_POINT('Ctrl Pts',(-0.225117921444226,0.00301994314685244,
0.00948650676310671));
#29799=CARTESIAN_POINT('Ctrl Pts',(-0.225116735324925,0.00296209933042116,
0.00945287844947561));
#29800=CARTESIAN_POINT('Ctrl Pts',(-0.225114046175496,0.00290467972170827,
0.00941860289759098));
#29801=CARTESIAN_POINT('Ctrl Pts',(-0.225104870506897,0.00277996152311542,
0.00934219611760584));
#29802=CARTESIAN_POINT('Ctrl Pts',(-0.225097762701751,0.00271289768830998,
0.00929983343525847));
#29803=CARTESIAN_POINT('Ctrl Pts',(-0.225071275977785,0.00252250121128088,
0.00917591424648294));
#29804=CARTESIAN_POINT('Ctrl Pts',(-0.225046633679134,0.00240132284164297,
0.00909253401528519));
#29805=CARTESIAN_POINT('Ctrl Pts',(-0.225014708541206,0.00228344637870765,
0.00900702965187676));
#29806=CARTESIAN_POINT('',(-0.225092272969296,0.00749505820794686,0.0106947832387151));
#29807=CARTESIAN_POINT('Ctrl Pts',(-0.225092270893944,0.00749505808259213,
0.0106948888771213));
#29808=CARTESIAN_POINT('Ctrl Pts',(-0.225024225129317,0.00671188196061008,
0.0106929144122287));
#29809=CARTESIAN_POINT('Ctrl Pts',(-0.224968404063802,0.00593093008167228,
0.0105880278895065));
#29810=CARTESIAN_POINT('Ctrl Pts',(-0.224963126040131,0.0051742066094581,
0.0103830238688901));
#29811=CARTESIAN_POINT('Ctrl Pts',(-0.224957869409366,0.00442055029181519,
0.0101788507713812));
#29812=CARTESIAN_POINT('Ctrl Pts',(-0.225002247330816,0.00369017725769303,
0.00987507507293168));
#29813=CARTESIAN_POINT('Ctrl Pts',(-0.22511807106961,0.0030194940701125,
0.00948730014603765));
#29814=CARTESIAN_POINT('',(-0.225114795773928,0.0119223070838394,0.00952049564286698));
#29815=CARTESIAN_POINT('Ctrl Pts',(-0.225114724781785,0.0119219979226124,
0.00951993302627938));
#29816=CARTESIAN_POINT('Ctrl Pts',(-0.225003084530341,0.0112547568345833,
0.00989797239668878));
#29817=CARTESIAN_POINT('Ctrl Pts',(-0.224963984333154,0.0105350672611751,
0.0101933029905569));
#29818=CARTESIAN_POINT('Ctrl Pts',(-0.224969552040664,0.0097879845343096,
0.0103925472293563));
#29819=CARTESIAN_POINT('Ctrl Pts',(-0.224971338108729,0.00954832744052368,
0.0104564629022893));
#29820=CARTESIAN_POINT('Ctrl Pts',(-0.22497772631488,0.00930594816711339,
0.0105104728615714));
#29821=CARTESIAN_POINT('Ctrl Pts',(-0.224987788152167,0.0090617312619527,
0.0105541768374275));
#29822=CARTESIAN_POINT('Ctrl Pts',(-0.225009092495973,0.00854464071849152,
0.0106467130711986));
#29823=CARTESIAN_POINT('Ctrl Pts',(-0.225046866204789,0.00801931179304763,
0.0106930084471554));
#29824=CARTESIAN_POINT('Ctrl Pts',(-0.225092297269035,0.00749505967569209,
0.0106935463466661));
#29825=CARTESIAN_POINT('',(-0.22499258838655,0.0127125317992707,0.00900988833309594));
#29826=CARTESIAN_POINT('Ctrl Pts',(-0.224991938877462,0.0127124272395741,
0.00900994896083489));
#29827=CARTESIAN_POINT('Ctrl Pts',(-0.225025552074485,0.0125862881553428,
0.00910138340065515));
#29828=CARTESIAN_POINT('Ctrl Pts',(-0.225052649372304,0.0124566919536995,
0.00919011728944026));
#29829=CARTESIAN_POINT('Ctrl Pts',(-0.225084070350122,0.0122533061865343,
0.00932132006962372));
#29830=CARTESIAN_POINT('Ctrl Pts',(-0.225093106140568,0.0121818687796175,
0.00936595433272495));
#29831=CARTESIAN_POINT('Ctrl Pts',(-0.225106409122268,0.0120476391460597,
0.00944712668901661));
#29832=CARTESIAN_POINT('Ctrl Pts',(-0.225111167725843,0.0119850807081392,
0.00948390081391465));
#29833=CARTESIAN_POINT('Ctrl Pts',(-0.225114536864462,0.0119220042196567,
0.00951992555793149));
#29834=CARTESIAN_POINT('',(-0.225275995996774,0.0126688942355271,0.00904667010172663));
#29835=CARTESIAN_POINT('Ctrl Pts',(-0.225275292269729,0.0126691944030332,
0.0090464420147403));
#29836=CARTESIAN_POINT('Ctrl Pts',(-0.22523224496111,0.0126875448165675,
0.00903254829052764));
#29837=CARTESIAN_POINT('Ctrl Pts',(-0.22518604351654,0.0127005646461434,
0.00902228805289712));
#29838=CARTESIAN_POINT('Ctrl Pts',(-0.225090148450807,0.0127152484784252,
0.00900984944409604));
#29839=CARTESIAN_POINT('Ctrl Pts',(-0.22504098157506,0.0127167959862583,
0.00900776711024177));
#29840=CARTESIAN_POINT('Ctrl Pts',(-0.224992260310303,0.01271250203545,
0.00900990144007799));
#29841=CARTESIAN_POINT('',(-0.225398010193384,0.013120318400212,0.00870574369815946));
#29842=CARTESIAN_POINT('Ctrl Pts',(-0.225397991300964,0.0131202941880968,
0.00870570880811002));
#29843=CARTESIAN_POINT('Ctrl Pts',(-0.225376967217776,0.013046681933572,
0.00876512827360961));
#29844=CARTESIAN_POINT('Ctrl Pts',(-0.225356173079467,0.0129720714761437,
0.00882339220392176));
#29845=CARTESIAN_POINT('Ctrl Pts',(-0.225315267761045,0.0128216609209388,
0.008936973809279));
#29846=CARTESIAN_POINT('Ctrl Pts',(-0.225295147418202,0.0127458635364527,
0.00899232711753521));
#29847=CARTESIAN_POINT('Ctrl Pts',(-0.225275261888314,0.0126691065284336,
0.00904650388940398));
#29848=CARTESIAN_POINT('',(-0.226397825284883,0.0131187534369297,0.00872595188639632));
#29849=CARTESIAN_POINT('Ctrl Pts',(-0.226397825264573,0.0131187211963479,
0.00872592705145478));
#29850=CARTESIAN_POINT('Ctrl Pts',(-0.226231196957561,0.0131189815906668,
0.00872255626913465));
#29851=CARTESIAN_POINT('Ctrl Pts',(-0.22606456844847,0.0131192426581214,
0.00871918629101479));
#29852=CARTESIAN_POINT('Ctrl Pts',(-0.22573129369429,0.0131197661684618,
0.00871244760079479));
#29853=CARTESIAN_POINT('Ctrl Pts',(-0.22556464732301,0.0131200286116902,
0.00870907888631731));
#29854=CARTESIAN_POINT('Ctrl Pts',(-0.225398001030979,0.0131202917297391,
0.00870571098993131));
#29855=CARTESIAN_POINT('',(-0.226273558818709,0.0126615507097427,0.00907157974325745));
#29856=CARTESIAN_POINT('Ctrl Pts',(-0.226273546976328,0.0126614891951054,
0.00907159303692138));
#29857=CARTESIAN_POINT('Ctrl Pts',(-0.226293819248747,0.0127397767182858,
0.00901634447273793));
#29858=CARTESIAN_POINT('Ctrl Pts',(-0.226314323246947,0.0128170574252013,
0.00895987557181371));
#29859=CARTESIAN_POINT('Ctrl Pts',(-0.226355750293415,0.0129694606248348,
0.0088446407394028));
#29860=CARTESIAN_POINT('Ctrl Pts',(-0.226376675901891,0.0130446000245681,
0.00878587031714395));
#29861=CARTESIAN_POINT('Ctrl Pts',(-0.226397824863347,0.0131187249268725,
0.00872592400672208));
#29862=CARTESIAN_POINT('',(-0.227025820193335,0.0126926713729642,0.00906414398299204));
#29863=CARTESIAN_POINT('Ctrl Pts',(-0.227025585132577,0.0126930612201683,
0.00906385023298042));
#29864=CARTESIAN_POINT('Ctrl Pts',(-0.226900285105079,0.0126994640941745,
0.0090567813192604));
#29865=CARTESIAN_POINT('Ctrl Pts',(-0.226774554286507,0.0127000381325738,
0.00905389459328833));
#29866=CARTESIAN_POINT('Ctrl Pts',(-0.226523261898834,0.0126895110571021,
0.00905651128120664));
#29867=CARTESIAN_POINT('Ctrl Pts',(-0.226397912137852,0.0126784000805961,
0.00906202567587128));
#29868=CARTESIAN_POINT('Ctrl Pts',(-0.226273566680661,0.0126614379936754,
0.00907162982036916));
#29869=CARTESIAN_POINT('',(-0.229319783972502,0.00893282155661927,0.0106733201854368));
#29870=CARTESIAN_POINT('Ctrl Pts',(-0.227025820193335,0.0126926713729642,
0.00906414398299204));
#29871=CARTESIAN_POINT('Ctrl Pts',(-0.227144422003088,0.0123844750755602,
0.00928810910664895));
#29872=CARTESIAN_POINT('Ctrl Pts',(-0.227378539637632,0.0117345865363843,
0.00969884466117373));
#29873=CARTESIAN_POINT('Ctrl Pts',(-0.228060574676232,0.0104466400243243,
0.0103068898455848));
#29874=CARTESIAN_POINT('Ctrl Pts',(-0.228822775788018,0.00954435960659404,
0.0105618645719844));
#29875=CARTESIAN_POINT('Ctrl Pts',(-0.229319782742692,0.00893282246601824,
0.0106733200063927));
#29876=CARTESIAN_POINT('Ctrl Pts',(-0.225870784240265,0.0163857105469993,
0.00232295787970897));
#29877=CARTESIAN_POINT('Ctrl Pts',(-0.225984689281823,0.0163678565223796,
0.00256925331663685));
#29878=CARTESIAN_POINT('Ctrl Pts',(-0.226270571940394,0.0163157306273066,
0.00313797237727359));
#29879=CARTESIAN_POINT('Ctrl Pts',(-0.226951825491954,0.0160791515514167,
0.00430595120672089));
#29880=CARTESIAN_POINT('Ctrl Pts',(-0.228041504483085,0.0155725225710242,
0.00569876179429522));
#29881=CARTESIAN_POINT('Ctrl Pts',(-0.229307422404798,0.0148998081355142,
0.00684612386700789));
#29882=CARTESIAN_POINT('Ctrl Pts',(-0.230375603478029,0.0142953788605102,
0.00764921276950633));
#29883=CARTESIAN_POINT('Ctrl Pts',(-0.231144606670057,0.0137796598506574,
0.00823050330807649));
#29884=CARTESIAN_POINT('Ctrl Pts',(-0.231717625303835,0.0132437427585838,
0.0087371891906484));
#29885=CARTESIAN_POINT('Ctrl Pts',(-0.231921495045492,0.0126777290387282,
0.00917894991078855));
#29886=CARTESIAN_POINT('Ctrl Pts',(-0.231856609050107,0.0120617879112867,
0.00959326671503007));
#29887=CARTESIAN_POINT('Ctrl Pts',(-0.231418479104261,0.0113315161178985,
0.00998183278666155));
#29888=CARTESIAN_POINT('Ctrl Pts',(-0.230760643568965,0.0105292050159737,
0.0103024614441315));
#29889=CARTESIAN_POINT('Ctrl Pts',(-0.230052352200966,0.00973441143097333,
0.0105331538057983));
#29890=CARTESIAN_POINT('Ctrl Pts',(-0.229564237344982,0.00920073542775872,
0.0106348601580364));
#29891=CARTESIAN_POINT('Ctrl Pts',(-0.229319785796903,0.00893282051848101,
0.0106733203943486));
#29892=CARTESIAN_POINT('',(-0.228033577259201,0.00748440686309334,0.0107613524025277));
#29893=CARTESIAN_POINT('',(-0.225970976589886,0.0102590377499324,0.010274952813057));
#29894=CARTESIAN_POINT('Ctrl Pts',(-0.225971973667151,0.0102581014536471,
0.0102752892966652));
#29895=CARTESIAN_POINT('Ctrl Pts',(-0.226258957253418,0.00981106287023984,
0.0104276655150511));
#29896=CARTESIAN_POINT('Ctrl Pts',(-0.226565327801358,0.00936526590846451,
0.0105414574236971));
#29897=CARTESIAN_POINT('Ctrl Pts',(-0.227252132952874,0.00843377550683359,
0.0107077786319585));
#29898=CARTESIAN_POINT('Ctrl Pts',(-0.227634704870478,0.00795248948585582,
0.0107518722875852));
#29899=CARTESIAN_POINT('Ctrl Pts',(-0.228035368651552,0.00748592054835535,
0.0107600046111732));
#29900=CARTESIAN_POINT('',(-0.226096198836323,0.00749455293783961,0.0107162203443074));
#29901=CARTESIAN_POINT('Ctrl Pts',(-0.226096198887514,0.0074945529422081,
0.0107162197568569));
#29902=CARTESIAN_POINT('Ctrl Pts',(-0.226045613969429,0.00800129271977726,
0.0107155800038505));
#29903=CARTESIAN_POINT('Ctrl Pts',(-0.226007580575707,0.0085095391841719,
0.0106722483098859));
#29904=CARTESIAN_POINT('Ctrl Pts',(-0.225976278112083,0.00923709836231164,
0.0105462751057775));
#29905=CARTESIAN_POINT('Ctrl Pts',(-0.225969942789085,0.00946159749189918,
0.0104982904773385));
#29906=CARTESIAN_POINT('Ctrl Pts',(-0.225965415311814,0.00987711744646229,
0.0103926336528987));
#29907=CARTESIAN_POINT('Ctrl Pts',(-0.225966264872201,0.0100685014222969,
0.0103371128225748));
#29908=CARTESIAN_POINT('Ctrl Pts',(-0.225970496220548,0.0102577785740447,
0.0102753623938262));
#29909=CARTESIAN_POINT('',(-0.225969628990936,0.00470142166790465,0.010263376289086));
#29910=CARTESIAN_POINT('Ctrl Pts',(-0.225968196058152,0.0047015146234352,
0.0102629949238911));
#29911=CARTESIAN_POINT('Ctrl Pts',(-0.225963828387184,0.0048913841275601,
0.01032589169753));
#29912=CARTESIAN_POINT('Ctrl Pts',(-0.225962903267804,0.00508303187486879,
0.0103823036863443));
#29913=CARTESIAN_POINT('Ctrl Pts',(-0.225967406633248,0.00550189479405183,
0.0104902436772195));
#29914=CARTESIAN_POINT('Ctrl Pts',(-0.22597386328584,0.00572895222895801,
0.0105393361889391));
#29915=CARTESIAN_POINT('Ctrl Pts',(-0.226005775090408,0.00646530387556126,
0.0106689593848215));
#29916=CARTESIAN_POINT('Ctrl Pts',(-0.226044659416343,0.00698069636745237,
0.0107145458902014));
#29917=CARTESIAN_POINT('Ctrl Pts',(-0.226096198875693,0.00749455293580526,
0.0107162197565836));
#29918=CARTESIAN_POINT('Ctrl Pts',(-0.22803357693545,0.0074844064806642,
0.0107613523945308));
#29919=CARTESIAN_POINT('Ctrl Pts',(-0.228009905277726,0.00745644439420555,
0.0107607676415092));
#29920=CARTESIAN_POINT('Ctrl Pts',(-0.227986276934626,0.00742844114892991,
0.0107600533973566));
#29921=CARTESIAN_POINT('Ctrl Pts',(-0.227962694037332,0.0074003983292184,
0.0107592078475071));
#29922=CARTESIAN_POINT('Ctrl Pts',(-0.227854134533825,0.00727130839820451,
0.0107553155152501));
#29923=CARTESIAN_POINT('Ctrl Pts',(-0.227747285397279,0.00714229162262032,
0.0107486933562038));
#29924=CARTESIAN_POINT('Ctrl Pts',(-0.227640411533435,0.00701114238092464,
0.0107390484382944));
#29925=CARTESIAN_POINT('Ctrl Pts',(-0.227573160013985,0.00692861532087877,
0.0107329792707631));
#29926=CARTESIAN_POINT('Ctrl Pts',(-0.227506577326311,0.0068461340379774,
0.0107257649510492));
#29927=CARTESIAN_POINT('Ctrl Pts',(-0.227440527701029,0.00676345650279847,
0.0107173671751193));
#29928=CARTESIAN_POINT('Ctrl Pts',(-0.227429839358583,0.0067500773836158,
0.0107160082225962));
#29929=CARTESIAN_POINT('Ctrl Pts',(-0.227419164145874,0.00673669198469641,
0.0107146181614928));
#29930=CARTESIAN_POINT('Ctrl Pts',(-0.227408502408266,0.00672330030514739,
0.0107131968807224));
#29931=CARTESIAN_POINT('Ctrl Pts',(-0.227398507029259,0.00671074560557031,
0.0107118644300003));
#29932=CARTESIAN_POINT('Ctrl Pts',(-0.227388523493641,0.00669818538584928,
0.010710504540147));
#29933=CARTESIAN_POINT('Ctrl Pts',(-0.227378552094813,0.00668561963553653,
0.0107091171207398));
#29934=CARTESIAN_POINT('Ctrl Pts',(-0.227344969296733,0.00664329928883968,
0.0107044444136701));
#29935=CARTESIAN_POINT('Ctrl Pts',(-0.227311528164211,0.00660092147569552,
0.0106994594641931));
#29936=CARTESIAN_POINT('Ctrl Pts',(-0.227278249873491,0.00655849689293043,
0.0106941607624104));
#29937=CARTESIAN_POINT('Ctrl Pts',(-0.227169961041194,0.00642044567608853,
0.0106769185839114));
#29938=CARTESIAN_POINT('Ctrl Pts',(-0.227063128893779,0.00628157692716777,
0.0106563233522903));
#29939=CARTESIAN_POINT('Ctrl Pts',(-0.226958472966203,0.0061419247782648,
0.0106322636464153));
#29940=CARTESIAN_POINT('Ctrl Pts',(-0.226952048338015,0.00613335179866265,
0.0106307866668678));
#29941=CARTESIAN_POINT('Ctrl Pts',(-0.226945632209316,0.00612477610935256,
0.0106292966723998));
#29942=CARTESIAN_POINT('Ctrl Pts',(-0.226939224866442,0.00611619781009488,
0.0106277936487921));
#29943=CARTESIAN_POINT('Ctrl Pts',(-0.226897570156155,0.00606042951777538,
0.0106180223576068));
#29944=CARTESIAN_POINT('Ctrl Pts',(-0.226855528870052,0.00600352434119545,
0.0106075108508253));
#29945=CARTESIAN_POINT('Ctrl Pts',(-0.226814483144495,0.00594725365858661,
0.0105965730065991));
#29946=CARTESIAN_POINT('Ctrl Pts',(-0.226770108470221,0.00588641923117389,
0.010584748065799));
#29947=CARTESIAN_POINT('Ctrl Pts',(-0.226727370143022,0.00582698986468138,
0.0105725911069167));
#29948=CARTESIAN_POINT('Ctrl Pts',(-0.226684141557327,0.00576593664027173,
0.0105594687640135));
#29949=CARTESIAN_POINT('Ctrl Pts',(-0.226652936231869,0.00572186428149994,
0.0105499961667847));
#29950=CARTESIAN_POINT('Ctrl Pts',(-0.226621988893697,0.00567768823496359,
0.0105401693083525));
#29951=CARTESIAN_POINT('Ctrl Pts',(-0.226591267477624,0.00563343719839793,
0.0105299865603063));
#29952=CARTESIAN_POINT('Ctrl Pts',(-0.226577826858092,0.00561407736990039,
0.0105255316080361));
#29953=CARTESIAN_POINT('Ctrl Pts',(-0.226564429604295,0.00559470309431951,
0.010521008528986));
#29954=CARTESIAN_POINT('Ctrl Pts',(-0.226551073458115,0.00557531642343092,
0.0105164171576264));
#29955=CARTESIAN_POINT('Ctrl Pts',(-0.226538552071071,0.00555714141947307,
0.0105121127469768));
#29956=CARTESIAN_POINT('Ctrl Pts',(-0.226526066816743,0.0055389555183428,
0.0105077483136463));
#29957=CARTESIAN_POINT('Ctrl Pts',(-0.226513615992729,0.00552076028083763,
0.010503323707922));
#29958=CARTESIAN_POINT('Ctrl Pts',(-0.226473450913159,0.00546206431329363,
0.0104890503842619));
#29959=CARTESIAN_POINT('Ctrl Pts',(-0.226432631356042,0.00540176900244369,
0.0104737572539422));
#29960=CARTESIAN_POINT('Ctrl Pts',(-0.226393664287511,0.00534371303495483,
0.0104584291238958));
#29961=CARTESIAN_POINT('Ctrl Pts',(-0.226367644141469,0.00530494633246592,
0.0104481938098889));
#29962=CARTESIAN_POINT('Ctrl Pts',(-0.226343230956819,0.00526837461445328,
0.0104382944101526));
#29963=CARTESIAN_POINT('Ctrl Pts',(-0.226316946251662,0.00522874762316253,
0.0104272855401428));
#29964=CARTESIAN_POINT('Ctrl Pts',(-0.226291077207928,0.00518974728571816,
0.0104164507623493));
#29965=CARTESIAN_POINT('Ctrl Pts',(-0.226264206467458,0.00514903911302078,
0.0104048478061562));
#29966=CARTESIAN_POINT('Ctrl Pts',(-0.226238708504583,0.00511034574189367,
0.0103935371682146));
#29967=CARTESIAN_POINT('Ctrl Pts',(-0.226233205333744,0.00510199463429003,
0.0103910960173982));
#29968=CARTESIAN_POINT('Ctrl Pts',(-0.226227700333222,0.00509363746989984,
0.0103886398549127));
#29969=CARTESIAN_POINT('Ctrl Pts',(-0.226222196488384,0.00508527941953711,
0.0103861702923412));
#29970=CARTESIAN_POINT('Ctrl Pts',(-0.226182592689434,0.00502513772659641,
0.010368400158467));
#29971=CARTESIAN_POINT('Ctrl Pts',(-0.226143231315418,0.00496523360787539,
0.010350032573918));
#29972=CARTESIAN_POINT('Ctrl Pts',(-0.226103876677456,0.00490537822662242,
0.0103309871000461));
#29973=CARTESIAN_POINT('Ctrl Pts',(-0.226081464749338,0.00487129140556136,
0.0103201409631357));
#29974=CARTESIAN_POINT('Ctrl Pts',(-0.226059075388918,0.00483724771525806,
0.0103090842351201));
#29975=CARTESIAN_POINT('Ctrl Pts',(-0.226036702403961,0.0048032531669151,
0.0102978161090545));
#29976=CARTESIAN_POINT('Ctrl Pts',(-0.226025515911483,0.004786255892744,
0.0102921820460218));
#29977=CARTESIAN_POINT('Ctrl Pts',(-0.226014333561778,0.00476927087634384,
0.0102864951249411));
#29978=CARTESIAN_POINT('Ctrl Pts',(-0.226003154809509,0.00475229874089972,
0.0102807552003522));
#29979=CARTESIAN_POINT('Ctrl Pts',(-0.225997565433375,0.00474381267317885,
0.0102778852380582));
#29980=CARTESIAN_POINT('Ctrl Pts',(-0.225991976958479,0.00473532982465564,
0.0102750020244736));
#29981=CARTESIAN_POINT('Ctrl Pts',(-0.225986389326614,0.0047268502677692,
0.0102721055390739));
#29982=CARTESIAN_POINT('Ctrl Pts',(-0.225980801694748,0.00471837071088277,
0.0102692090536741));
#29983=CARTESIAN_POINT('Ctrl Pts',(-0.225975214905513,0.0047098944449384,
0.0102662992960872));
#29984=CARTESIAN_POINT('Ctrl Pts',(-0.225969628990936,0.00470142166790475,
0.0102633762890857));
#29985=CARTESIAN_POINT('',(-0.226096178744282,0.00750540343988805,-0.0107162180661903));
#29986=CARTESIAN_POINT('',(-0.225967411913371,0.0102623479612313,-0.0102748686137305));
#29987=CARTESIAN_POINT('Ctrl Pts',(-0.225967387201314,0.0102611633020894,
-0.0102752620305393));
#29988=CARTESIAN_POINT('Ctrl Pts',(-0.225963503316852,0.0100728173574592,
-0.010336734102349));
#29989=CARTESIAN_POINT('Ctrl Pts',(-0.22596296794087,0.00988279893284449,
-0.0103918116764779));
#29990=CARTESIAN_POINT('Ctrl Pts',(-0.22596813343084,0.00946801496741777,
-0.0104970323863582));
#29991=CARTESIAN_POINT('Ctrl Pts',(-0.225974821774181,0.00924339636561263,
-0.0105448231600401));
#29992=CARTESIAN_POINT('Ctrl Pts',(-0.226007053817059,0.00851770773012774,
-0.0106704459522781));
#29993=CARTESIAN_POINT('Ctrl Pts',(-0.226045487878963,0.00801086921392995,
-0.0107145664926717));
#29994=CARTESIAN_POINT('Ctrl Pts',(-0.226096168126154,0.00750551040622462,
-0.0107162162799583));
#29995=CARTESIAN_POINT('',(-0.228054819889722,0.00748068141568947,-0.0107604444270658));
#29996=CARTESIAN_POINT('Ctrl Pts',(-0.228054819890027,0.00748068141595342,
-0.0107604444270559));
#29997=CARTESIAN_POINT('Ctrl Pts',(-0.227652037218058,0.00794552320395912,
-0.0107521683783107));
#29998=CARTESIAN_POINT('Ctrl Pts',(-0.227267804242261,0.00842519382017008,
-0.0107081952621097));
#29999=CARTESIAN_POINT('Ctrl Pts',(-0.226574304617479,0.00935827291019254,
-0.0105431611063224));
#30000=CARTESIAN_POINT('Ctrl Pts',(-0.226262051637222,0.00980918637230702,
-0.0104294968164533));
#30001=CARTESIAN_POINT('Ctrl Pts',(-0.225968440683985,0.0102619875384845,
-0.0102750157142978));
#30002=CARTESIAN_POINT('',(-0.225972184946916,0.00467377596756055,-0.010252770733025));
#30003=CARTESIAN_POINT('Ctrl Pts',(-0.225973609942387,0.00467436557371437,
-0.0102529563829087));
#30004=CARTESIAN_POINT('Ctrl Pts',(-0.226285458894388,0.00517297659214837,
-0.0104271136615909));
#30005=CARTESIAN_POINT('Ctrl Pts',(-0.226623269987956,0.00566740906512651,
-0.0105522882614033));
#30006=CARTESIAN_POINT('Ctrl Pts',(-0.227329537494644,0.0066117069902153,
-0.0107122048385642));
#30007=CARTESIAN_POINT('Ctrl Pts',(-0.227687882265678,0.00704950453591529,
-0.0107513952059892));
#30008=CARTESIAN_POINT('Ctrl Pts',(-0.228054819889427,0.00748068141594102,
-0.0107604444270423));
#30009=CARTESIAN_POINT('Ctrl Pts',(-0.226096200187826,0.00750540266069626,
-0.0107162171111456));
#30010=CARTESIAN_POINT('Ctrl Pts',(-0.226044299402367,0.00698548623471811,
-0.0107155583402523));
#30011=CARTESIAN_POINT('Ctrl Pts',(-0.226005601313484,0.00646398203969811,
-0.0106699545805781));
#30012=CARTESIAN_POINT('Ctrl Pts',(-0.225974806245419,0.00571858163159882,
-0.0105374320042732));
#30013=CARTESIAN_POINT('Ctrl Pts',(-0.225968822940153,0.00548862267467334,
-0.0104869806370106));
#30014=CARTESIAN_POINT('Ctrl Pts',(-0.225965434348515,0.00506386537530727,
-0.0103761076146514));
#30015=CARTESIAN_POINT('Ctrl Pts',(-0.225966991269723,0.00486851066308794,
-0.010317937672268));
#30016=CARTESIAN_POINT('Ctrl Pts',(-0.225972142300558,0.00467541771917558,
-0.0102532772611998));
#30017=CARTESIAN_POINT('Ctrl Pts',(-0.224903047769934,0.0163974953490442,
0.00232527569536224));
#30018=CARTESIAN_POINT('Ctrl Pts',(-0.228003678801843,0.0163652528946496,
0.00231821622721085));
#30019=CARTESIAN_POINT('Ctrl Pts',(-0.23110431006382,0.0163330357098684,
0.00231114482972889));
#30020=CARTESIAN_POINT('Ctrl Pts',(-0.234204941533998,0.0163008422866106,
0.00230405918705812));
#30021=CARTESIAN_POINT('Ctrl Pts',(-0.224902923051373,0.016421905903896,
0.001999690061282));
#30022=CARTESIAN_POINT('Ctrl Pts',(-0.228003554472057,0.0163857948128496,
0.00199154431614981));
#30023=CARTESIAN_POINT('Ctrl Pts',(-0.231104186130884,0.0163497065102629,
0.00198339075959686));
#30024=CARTESIAN_POINT('Ctrl Pts',(-0.23420481801057,0.0163136399270852,
0.00197522735965944));
#30025=CARTESIAN_POINT('Ctrl Pts',(-0.224902686634519,0.0164496060066283,
0.00134999605462854));
#30026=CARTESIAN_POINT('Ctrl Pts',(-0.228003316903349,0.0164061218898441,
0.00134119319572166));
#30027=CARTESIAN_POINT('Ctrl Pts',(-0.231103947348719,0.0163626446434222,
0.00133240817680761));
#30028=CARTESIAN_POINT('Ctrl Pts',(-0.234204577993315,0.0163191760221561,
0.00132364096404516));
#30029=CARTESIAN_POINT('Ctrl Pts',(-0.22490247733934,0.0164891827557564,
8.48946422705292E-5));
#30030=CARTESIAN_POINT('Ctrl Pts',(-0.2280031047451,0.0164387037966636,
8.36968421714054E-5));
#30031=CARTESIAN_POINT('Ctrl Pts',(-0.231103732057188,0.01638822192355,
8.25020821930779E-5));
#30032=CARTESIAN_POINT('Ctrl Pts',(-0.234204359262361,0.016337735996471,
8.13110569434896E-5));
#30033=CARTESIAN_POINT('Ctrl Pts',(-0.224902601832635,0.0164577305274795,
-0.00116946331798178));
#30034=CARTESIAN_POINT('Ctrl Pts',(-0.22800323228218,0.0164115731563456,
-0.00115947279336496));
#30035=CARTESIAN_POINT('Ctrl Pts',(-0.231103862912676,0.016365419418937,
-0.00114950763219157));
#30036=CARTESIAN_POINT('Ctrl Pts',(-0.234204493754791,0.0163192718567599,
-0.00113956819841304));
#30037=CARTESIAN_POINT('Ctrl Pts',(-0.2249031047193,0.016401050271707,-0.00247428944274167));
#30038=CARTESIAN_POINT('Ctrl Pts',(-0.228003735976318,0.016370691448232,
-0.00246735407024901));
#30039=CARTESIAN_POINT('Ctrl Pts',(-0.231104367476673,0.0163403620163895,
-0.00246039974613875));
#30040=CARTESIAN_POINT('Ctrl Pts',(-0.234204999188339,0.0163100597051565,
-0.00245342363871553));
#30041=CARTESIAN_POINT('Ctrl Pts',(-0.224903620482978,0.0162331344936927,
-0.00377581649114323));
#30042=CARTESIAN_POINT('Ctrl Pts',(-0.228004247053984,0.0162183248288798,
-0.00377611183675602));
#30043=CARTESIAN_POINT('Ctrl Pts',(-0.231104873706723,0.0162035348039987,
-0.00377640360674382));
#30044=CARTESIAN_POINT('Ctrl Pts',(-0.23420550044494,0.0161887639228305,
-0.00377669038870648));
#30045=CARTESIAN_POINT('Ctrl Pts',(-0.224904244439412,0.0157454055087051,
-0.00535508843351867));
#30046=CARTESIAN_POINT('Ctrl Pts',(-0.228004869356698,0.015745877431058,
-0.00536654194974573));
#30047=CARTESIAN_POINT('Ctrl Pts',(-0.231105494288016,0.0157463686608469,
-0.00537798949180189));
#30048=CARTESIAN_POINT('Ctrl Pts',(-0.234206119236561,0.0157468784277487,
-0.00538942975580705));
#30049=CARTESIAN_POINT('Ctrl Pts',(-0.224904927056323,0.014756116525245,
-0.0070809462510311));
#30050=CARTESIAN_POINT('Ctrl Pts',(-0.228005551277712,0.0147682738612367,
-0.00710847555851588));
#30051=CARTESIAN_POINT('Ctrl Pts',(-0.231106175457583,0.0147804448844733,
-0.00713600323790223));
#30052=CARTESIAN_POINT('Ctrl Pts',(-0.234206799604821,0.014792629252247,
-0.00716352865861212));
#30053=CARTESIAN_POINT('Ctrl Pts',(-0.224905705935764,0.0129587456084716,
-0.00904270204015799));
#30054=CARTESIAN_POINT('Ctrl Pts',(-0.228006331471737,0.0129775263446935,
-0.00909152831654588));
#30055=CARTESIAN_POINT('Ctrl Pts',(-0.231106956961612,0.0129963155259409,
-0.00914035417356039));
#30056=CARTESIAN_POINT('Ctrl Pts',(-0.234207582410669,0.0130151128918419,
-0.00918917939755658));
#30057=CARTESIAN_POINT('Ctrl Pts',(-0.224906344901157,0.00996717482975785,
-0.0106558172504251));
#30058=CARTESIAN_POINT('Ctrl Pts',(-0.228006973196984,0.00997888641244874,
-0.0107253416344494));
#30059=CARTESIAN_POINT('Ctrl Pts',(-0.23110760149003,0.00999060093234777,
-0.0107948661290257));
#30060=CARTESIAN_POINT('Ctrl Pts',(-0.234208229780548,0.0100023182636535,
-0.010864390745125));
#30061=CARTESIAN_POINT('Ctrl Pts',(-0.224906421473904,0.00588448586822914,
-0.0108495989887083));
#30062=CARTESIAN_POINT('Ctrl Pts',(-0.228007050197119,0.00587660352368733,
-0.0109217704181749));
#30063=CARTESIAN_POINT('Ctrl Pts',(-0.231107678925808,0.00586871925150363,
-0.0109939418074081));
#30064=CARTESIAN_POINT('Ctrl Pts',(-0.23420830765933,0.00586083314294305,
-0.0110661131658069));
#30065=CARTESIAN_POINT('Ctrl Pts',(-0.224905896797368,0.00275206275993148,
-0.00952499259309634));
#30066=CARTESIAN_POINT('Ctrl Pts',(-0.22800652301585,0.00273399542249794,
-0.00957977151548));
#30067=CARTESIAN_POINT('Ctrl Pts',(-0.231107149196805,0.00271592133715538,
-0.00963455045765119));
#30068=CARTESIAN_POINT('Ctrl Pts',(-0.234207775344483,0.00269784071003669,
-0.00968932931015458));
#30069=CARTESIAN_POINT('Ctrl Pts',(-0.224905188461513,0.000775386387695849,
-0.00774097724716007));
#30070=CARTESIAN_POINT('Ctrl Pts',(-0.228005812987761,0.000760338332521188,
-0.0077754138708565));
#30071=CARTESIAN_POINT('Ctrl Pts',(-0.231106437467874,0.000745278047377309,
-0.00780984908461508));
#30072=CARTESIAN_POINT('Ctrl Pts',(-0.234207061909447,0.000730205873823641,
-0.00784428237662763));
#30073=CARTESIAN_POINT('Ctrl Pts',(-0.224904545212544,-0.00037433699893992,
-0.00611286595312136));
#30074=CARTESIAN_POINT('Ctrl Pts',(-0.228005169500613,-0.000380655003703386,
-0.00613103039787742));
#30075=CARTESIAN_POINT('Ctrl Pts',(-0.231105793767721,-0.000386989095479687,
-0.00614919200572512));
#30076=CARTESIAN_POINT('Ctrl Pts',(-0.234206418022201,-0.000393338834079428,
-0.00616734988680402));
#30077=CARTESIAN_POINT('Ctrl Pts',(-0.224903937950997,-0.00100476933014151,
-0.00458381173225385));
#30078=CARTESIAN_POINT('Ctrl Pts',(-0.228004563842973,-0.000997949740617374,
-0.00458943898701532));
#30079=CARTESIAN_POINT('Ctrl Pts',(-0.231105189790958,-0.000991151361328939,
-0.00459505880592969));
#30080=CARTESIAN_POINT('Ctrl Pts',(-0.234205815794275,-0.000984373265027772,
-0.00460066961067425));
#30081=CARTESIAN_POINT('Ctrl Pts',(-0.224903434943426,-0.00130314167877163,
-0.00330350941820122));
#30082=CARTESIAN_POINT('Ctrl Pts',(-0.228004062879574,-0.00128286930948369,
-0.00330122419140405));
#30083=CARTESIAN_POINT('Ctrl Pts',(-0.231104690943801,-0.00126261869681616,
-0.0032989320974583));
#30084=CARTESIAN_POINT('Ctrl Pts',(-0.234205319131308,-0.00124238896138437,
-0.00329663139924215));
#30085=CARTESIAN_POINT('Ctrl Pts',(-0.224903041260456,-0.00140805611840559,
-0.00232453718253355));
#30086=CARTESIAN_POINT('Ctrl Pts',(-0.228003673257076,-0.0013756315595115,
-0.00231672000225054));
#30087=CARTESIAN_POINT('Ctrl Pts',(-0.231104305522642,-0.00134323774830377,
-0.00230888218475535));
#30088=CARTESIAN_POINT('Ctrl Pts',(-0.234204938019884,-0.00131087220379368,
-0.00230102069899992));
#30089=CARTESIAN_POINT('Ctrl Pts',(-0.224902686634356,-0.00144960594189391,
-0.00134999602285112));
#30090=CARTESIAN_POINT('Ctrl Pts',(-0.228003316903184,-0.00140612182039602,
-0.00134119316178982));
#30091=CARTESIAN_POINT('Ctrl Pts',(-0.23110394734855,-0.00136264456921374,
-0.00133240814074275));
#30092=CARTESIAN_POINT('Ctrl Pts',(-0.234204577993143,-0.00131917594314456,
-0.00132364092587474));
#30093=CARTESIAN_POINT('Ctrl Pts',(-0.22490247733939,-0.0014891827680679,
-8.48946648711828E-5));
#30094=CARTESIAN_POINT('Ctrl Pts',(-0.228003104745152,-0.00143870380997731,
-8.36968663193096E-5));
#30095=CARTESIAN_POINT('Ctrl Pts',(-0.231103732057244,-0.00138822193789455,
-8.25021078797203E-5));
#30096=CARTESIAN_POINT('Ctrl Pts',(-0.23420435926242,-0.00133773601187166,
-8.1311084157012E-5));
#30097=CARTESIAN_POINT('Ctrl Pts',(-0.22490260183294,-0.0014577307002292,
0.00116946334942344));
#30098=CARTESIAN_POINT('Ctrl Pts',(-0.228003232282475,-0.00141157334093523,
0.00115947282708936));
#30099=CARTESIAN_POINT('Ctrl Pts',(-0.231103862912961,-0.00136541961535455,
0.00114950766822477));
#30100=CARTESIAN_POINT('Ctrl Pts',(-0.234204493755065,-0.001319272064998,
0.00113956823678177));
#30101=CARTESIAN_POINT('Ctrl Pts',(-0.224903104718753,-0.00140104996632292,
0.00247428939345485));
#30102=CARTESIAN_POINT('Ctrl Pts',(-0.228003735975788,-0.00137069112187628,
0.00246735401736931));
#30103=CARTESIAN_POINT('Ctrl Pts',(-0.231104367476161,-0.0013403616690761,
0.00246039968961847));
#30104=CARTESIAN_POINT('Ctrl Pts',(-0.234204999187845,-0.00131005933689176,
0.00245342357850486));
#30105=CARTESIAN_POINT('Ctrl Pts',(-0.224903620487317,-0.00123313642614889,
0.00377581720335721));
#30106=CARTESIAN_POINT('Ctrl Pts',(-0.228004247058324,-0.00121832689931329,
0.00377611259775251));
#30107=CARTESIAN_POINT('Ctrl Pts',(-0.231104873711069,-0.00120353701330459,
0.00377640441621043));
#30108=CARTESIAN_POINT('Ctrl Pts',(-0.234205500449294,-0.00118876627184354,
0.00377669124621538));
#30109=CARTESIAN_POINT('Ctrl Pts',(-0.224904244452509,-0.000745411287960432,
0.00535508951527424));
#30110=CARTESIAN_POINT('Ctrl Pts',(-0.228004869369835,-0.000745883603517816,
0.00536654310520161));
#30111=CARTESIAN_POINT('Ctrl Pts',(-0.231105494301186,-0.000746375225293753,
0.00537799072107391));
#30112=CARTESIAN_POINT('Ctrl Pts',(-0.234206119249757,-0.000746885383007411,
0.00538943105918803));
#30113=CARTESIAN_POINT('Ctrl Pts',(-0.224904927022406,0.000243903830950042,
0.00708094602779947));
#30114=CARTESIAN_POINT('Ctrl Pts',(-0.22800555124417,0.000231747907332828,
0.00710847531073915));
#30115=CARTESIAN_POINT('Ctrl Pts',(-0.231106175424446,0.00021957829815924,
0.00713600296412369));
#30116=CARTESIAN_POINT('Ctrl Pts',(-0.234206799572117,0.000207395346249357,
0.0071635283576419));
#30117=CARTESIAN_POINT('Ctrl Pts',(-0.224905705882564,0.00204129536417242,
0.00904270545084878));
#30118=CARTESIAN_POINT('Ctrl Pts',(-0.228006331417495,0.00202251745037019,
0.00909153197079319));
#30119=CARTESIAN_POINT('Ctrl Pts',(-0.231106956906316,0.00200373108991613,
0.00914035807264341));
#30120=CARTESIAN_POINT('Ctrl Pts',(-0.234207582354303,0.00198493654309014,
0.00918918354252649));
#30121=CARTESIAN_POINT('Ctrl Pts',(-0.224906344934492,0.00503279669879239,
0.0106558220281949));
#30122=CARTESIAN_POINT('Ctrl Pts',(-0.228006973230644,0.00502108315461209,
0.0107253467403358));
#30123=CARTESIAN_POINT('Ctrl Pts',(-0.231107601524016,0.00500936667421796,
0.0107948715627757));
#30124=CARTESIAN_POINT('Ctrl Pts',(-0.234208229814862,0.00499764738343722,
0.0108643965065502));
#30125=CARTESIAN_POINT('Ctrl Pts',(-0.22490642148267,0.00911553811978304,
0.0108495997280891));
#30126=CARTESIAN_POINT('Ctrl Pts',(-0.22800705020616,0.00912342211753167,
0.0109217712057851));
#30127=CARTESIAN_POINT('Ctrl Pts',(-0.231107678935135,0.0091313080421625,
0.0109939426427322));
#30128=CARTESIAN_POINT('Ctrl Pts',(-0.234208307668951,0.00913919580236395,
0.0110661140483708));
#30129=CARTESIAN_POINT('Ctrl Pts',(-0.224905896781363,0.0122479140000228,
0.00952499840433065));
#30130=CARTESIAN_POINT('Ctrl Pts',(-0.228006522998932,0.0122659797356893,
0.00957977773742142));
#30131=CARTESIAN_POINT('Ctrl Pts',(-0.231107149178945,0.012284052220171,
0.00963455709198015));
#30132=CARTESIAN_POINT('Ctrl Pts',(-0.234207775325653,0.0123021312474762,
0.00968933635838273));
#30133=CARTESIAN_POINT('Ctrl Pts',(-0.224905188406661,0.0142245802852993,
0.00774097735435126));
#30134=CARTESIAN_POINT('Ctrl Pts',(-0.228005812932864,0.014239626038719,
0.0077754139801973));
#30135=CARTESIAN_POINT('Ctrl Pts',(-0.231106437412959,0.0142546840218181,
0.00780984919513146));
#30136=CARTESIAN_POINT('Ctrl Pts',(-0.234207061854539,0.014269753892948,
0.00784428248742507));
#30137=CARTESIAN_POINT('Ctrl Pts',(-0.224904545213284,0.0153743354777482,
0.00611286639462737));
#30138=CARTESIAN_POINT('Ctrl Pts',(-0.228005169501712,0.0153806533667306,
0.00613103086359291));
#30139=CARTESIAN_POINT('Ctrl Pts',(-0.231105793769188,0.0153869873403304,
0.0061491924949429));
#30140=CARTESIAN_POINT('Ctrl Pts',(-0.234206418024041,0.0153933369583363,
0.00616735039916125));
#30141=CARTESIAN_POINT('Ctrl Pts',(-0.224903937959543,0.0160047733300576,
0.00458381273421664));
#30142=CARTESIAN_POINT('Ctrl Pts',(-0.228004563851456,0.015997954017428,
0.00458944005855562));
#30143=CARTESIAN_POINT('Ctrl Pts',(-0.231105189799372,0.0159911559151915,
0.00459505994710943));
#30144=CARTESIAN_POINT('Ctrl Pts',(-0.234205815802617,0.0159843780961064,
0.00460067082154373));
#30145=CARTESIAN_POINT('Ctrl Pts',(-0.224903434945887,0.0163031426775171,
0.00330350985910996));
#30146=CARTESIAN_POINT('Ctrl Pts',(-0.228004062882068,0.0162828703806443,
0.0033012246620879));
#30147=CARTESIAN_POINT('Ctrl Pts',(-0.231104690946332,0.0162626198410551,
0.00329893259759974));
#30148=CARTESIAN_POINT('Ctrl Pts',(-0.23420531913388,0.0162423901793082,
0.00329663192843727));
#30149=CARTESIAN_POINT('Ctrl Pts',(-0.224903172488496,0.0163730847941923,
0.00265086132944247));
#30150=CARTESIAN_POINT('Ctrl Pts',(-0.22800380313163,0.0163447109764496,
0.00264488813827189));
#30151=CARTESIAN_POINT('Ctrl Pts',(-0.231104433996755,0.0163163649094739,
0.00263889889986091));
#30152=CARTESIAN_POINT('Ctrl Pts',(-0.234205065057425,0.0162880446461359,
0.00263289101445681));
#30153=CARTESIAN_POINT('Ctrl Pts',(-0.224903047769934,0.0163974953490442,
0.00232527569536224));
#30154=CARTESIAN_POINT('Ctrl Pts',(-0.228003678801843,0.0163652528946496,
0.00231821622721085));
#30155=CARTESIAN_POINT('Ctrl Pts',(-0.23110431006382,0.0163330357098684,
0.00231114482972889));
#30156=CARTESIAN_POINT('Ctrl Pts',(-0.234204941533998,0.0163008422866106,
0.00230405918705812));
#30157=CARTESIAN_POINT('',(-0.225009761049809,0.0164742955512205,-2.91283822632387E-7));
#30158=CARTESIAN_POINT('Ctrl Pts',(-0.225009761049848,0.0164742955512199,
-2.9128306942331E-7));
#30159=CARTESIAN_POINT('Ctrl Pts',(-0.225235788735119,0.0164707797999031,
0.000697174222861705));
#30160=CARTESIAN_POINT('Ctrl Pts',(-0.225493369618686,0.016441583044206,
0.00148467486114592));
#30161=CARTESIAN_POINT('Ctrl Pts',(-0.225831296494198,0.0163919000464353,
0.00223757402366504));
#30162=CARTESIAN_POINT('Ctrl Pts',(-0.225870784240265,0.0163857105469993,
0.00232295787970897));
#30163=CARTESIAN_POINT('Ctrl Pts',(-0.231901468479132,0.0119424667401788,
-0.00964990277379923));
#30164=CARTESIAN_POINT('Ctrl Pts',(-0.23196556433204,0.0120553195071661,
-0.00958547241096005));
#30165=CARTESIAN_POINT('Ctrl Pts',(-0.232092641041587,0.012318056643556,
-0.00942714628191483));
#30166=CARTESIAN_POINT('Ctrl Pts',(-0.232189484894588,0.0127464465580913,
-0.00913453448129261));
#30167=CARTESIAN_POINT('Ctrl Pts',(-0.232026909656826,0.0133298270418654,
-0.00866985986404063));
#30168=CARTESIAN_POINT('Ctrl Pts',(-0.231431264476163,0.0138642223513919,
-0.00814845542092376));
#30169=CARTESIAN_POINT('Ctrl Pts',(-0.230626882102772,0.0143537410803797,
-0.00758117056316697));
#30170=CARTESIAN_POINT('Ctrl Pts',(-0.229503933937131,0.0149270508431769,
-0.00680405147634905));
#30171=CARTESIAN_POINT('Ctrl Pts',(-0.22817297623813,0.0155747191869899,
-0.00568892386192561));
#30172=CARTESIAN_POINT('Ctrl Pts',(-0.227021852380984,0.0160747388453188,
-0.00431844004910359));
#30173=CARTESIAN_POINT('Ctrl Pts',(-0.22625946762174,0.0163293197705724,
-0.00307502577355553));
#30174=CARTESIAN_POINT('Ctrl Pts',(-0.225588510819443,0.0164318308607234,
-0.00175821008748369));
#30175=CARTESIAN_POINT('Ctrl Pts',(-0.225239759337853,0.0164707047194801,
-0.000703191917106053));
#30176=CARTESIAN_POINT('Ctrl Pts',(-0.225009761049809,0.0164742955512205,
-2.91283822632387E-7));
#30177=CARTESIAN_POINT('',(-0.227105547431055,0.0164416356533412,-1.96367613579375E-8));
#30178=CARTESIAN_POINT('Ctrl Pts',(-0.227105547430907,0.0164416356533435,
-1.96363604482556E-8));
#30179=CARTESIAN_POINT('Ctrl Pts',(-0.227140935573775,0.0164410841784684,
-9.60298985735003E-5));
#30180=CARTESIAN_POINT('Ctrl Pts',(-0.227176314604842,0.0164400697376915,
-0.000192131486811683));
#30181=CARTESIAN_POINT('Ctrl Pts',(-0.227212010478261,0.0164386687878891,
-0.000288124301984629));
#30182=CARTESIAN_POINT('Ctrl Pts',(-0.227307348630138,0.016434927067846,
-0.000544506250803369));
#30183=CARTESIAN_POINT('Ctrl Pts',(-0.227404969846049,0.0164285564552437,
-0.00080011931205441));
#30184=CARTESIAN_POINT('Ctrl Pts',(-0.227510944626544,0.0164208305077663,
-0.00105112973174067));
#30185=CARTESIAN_POINT('Ctrl Pts',(-0.227524004952427,0.0164198783624414,
-0.00108206424149788));
#30186=CARTESIAN_POINT('Ctrl Pts',(-0.227537191850656,0.0164189056258689,
-0.00111292900197045));
#30187=CARTESIAN_POINT('Ctrl Pts',(-0.227550505575517,0.0164179103665598,
-0.00114372242291194));
#30188=CARTESIAN_POINT('Ctrl Pts',(-0.227570729683619,0.0164163985258039,
-0.00119049892463991));
#30189=CARTESIAN_POINT('Ctrl Pts',(-0.227591245817737,0.0164148331361413,
-0.00123710938263162));
#30190=CARTESIAN_POINT('Ctrl Pts',(-0.227612055857281,0.0164132070087615,
-0.00128355085207765));
#30191=CARTESIAN_POINT('Ctrl Pts',(-0.227684890995684,0.0164075155629321,
-0.00144609599513877));
#30192=CARTESIAN_POINT('Ctrl Pts',(-0.227761330033667,0.0164011975804018,
-0.00160657657145748));
#30193=CARTESIAN_POINT('Ctrl Pts',(-0.227841439738122,0.016393908424669,
-0.00176485026197984));
#30194=CARTESIAN_POINT('Ctrl Pts',(-0.22788149459035,0.0163902638468026,
-0.00184398710724102));
#30195=CARTESIAN_POINT('Ctrl Pts',(-0.227922466302893,0.0163863523316187,
-0.00192257103644991));
#30196=CARTESIAN_POINT('Ctrl Pts',(-0.227964360185775,0.0163821164167468,
-0.0020005813551573));
#30197=CARTESIAN_POINT('Ctrl Pts',(-0.227994642668365,0.0163790545373139,
-0.00205697016315432));
#30198=CARTESIAN_POINT('Ctrl Pts',(-0.228025406156946,0.0163758205550357,
-0.00211305781216197));
#30199=CARTESIAN_POINT('Ctrl Pts',(-0.228056654057935,0.0163723992572222,
-0.00216883939895636));
#30200=CARTESIAN_POINT('Ctrl Pts',(-0.228068635634597,0.0163710874077623,
-0.0021902280790714));
#30201=CARTESIAN_POINT('Ctrl Pts',(-0.228080688431295,0.0163697480197511,
-0.00221157175871921));
#30202=CARTESIAN_POINT('Ctrl Pts',(-0.228092811031844,0.0163683783499799,
-0.00223286967464982));
#30203=CARTESIAN_POINT('Ctrl Pts',(-0.228286284646469,0.0163465187695721,
-0.00257277898389818));
#30204=CARTESIAN_POINT('Ctrl Pts',(-0.228497453761435,0.016317224118046,
-0.00290123520754679));
#30205=CARTESIAN_POINT('Ctrl Pts',(-0.228724359620867,0.0162698007708276,
-0.00321950024123378));
#30206=CARTESIAN_POINT('Ctrl Pts',(-0.228731950990746,0.0162682141737667,
-0.00323014812664534));
#30207=CARTESIAN_POINT('Ctrl Pts',(-0.228739560119947,0.0162666070912213,
-0.00324078450904247));
#30208=CARTESIAN_POINT('Ctrl Pts',(-0.228747187150802,0.0162649798437748,
-0.00325140938042041));
#30209=CARTESIAN_POINT('Ctrl Pts',(-0.22886498654879,0.0162398470269272,
-0.00341551038850264));
#30210=CARTESIAN_POINT('Ctrl Pts',(-0.228987064650102,0.0162097845462495,
-0.003576845525633));
#30211=CARTESIAN_POINT('Ctrl Pts',(-0.229113100652467,0.0161761306248802,
-0.00373426103364333));
#30212=CARTESIAN_POINT('Ctrl Pts',(-0.229235349109519,0.0161434880474898,
-0.00388694600150465));
#30213=CARTESIAN_POINT('Ctrl Pts',(-0.229361320812065,0.0161074674237774,
-0.00403594274649993));
#30214=CARTESIAN_POINT('Ctrl Pts',(-0.229490644364937,0.0160692846524978,
-0.00418024936974081));
#30215=CARTESIAN_POINT('Ctrl Pts',(-0.229494651113392,0.0160681016602552,
-0.00418472032902758));
#30216=CARTESIAN_POINT('Ctrl Pts',(-0.229498661073176,0.0160669165977826,
-0.00418918679279889));
#30217=CARTESIAN_POINT('Ctrl Pts',(-0.229502674213524,0.0160657294663742,
-0.00419364877005753));
#30218=CARTESIAN_POINT('Ctrl Pts',(-0.229769760214949,0.0159867224659753,
-0.00449060615537639));
#30219=CARTESIAN_POINT('Ctrl Pts',(-0.230050851774607,0.0158986361087921,
-0.00476766623051437));
#30220=CARTESIAN_POINT('Ctrl Pts',(-0.230340579947594,0.0158014507554148,
-0.00503153449351247));
#30221=CARTESIAN_POINT('Ctrl Pts',(-0.230485444034087,0.0157528580787261,
-0.00516346862501151));
#30222=CARTESIAN_POINT('Ctrl Pts',(-0.23063247142736,0.015701991599058,
-0.005292100425029));
#30223=CARTESIAN_POINT('Ctrl Pts',(-0.230781004357612,0.0156488559127553,
-0.00541825073710578));
#30224=CARTESIAN_POINT('Ctrl Pts',(-0.230929537287864,0.0155957202264526,
-0.00554440104918256));
#30225=CARTESIAN_POINT('Ctrl Pts',(-0.231079576062874,0.0155403155041193,
-0.00566806935446317));
#30226=CARTESIAN_POINT('Ctrl Pts',(-0.231230463152709,0.0154826501973941,
-0.00579007476384777));
#30227=CARTESIAN_POINT('Ctrl Pts',(-0.23123663742441,0.0154802905437494,
-0.00579506720254754));
#30228=CARTESIAN_POINT('Ctrl Pts',(-0.231242813084713,0.015477927087919,
-0.00580005681784355));
#30229=CARTESIAN_POINT('Ctrl Pts',(-0.231248990111509,0.0154755598168904,
-0.00580504368212982));
#30230=CARTESIAN_POINT('Ctrl Pts',(-0.231393767503663,0.0154200756272723,
-0.00592192599949613));
#30231=CARTESIAN_POINT('Ctrl Pts',(-0.231539296831414,0.0153624991268241,
-0.00603729915711179));
#30232=CARTESIAN_POINT('Ctrl Pts',(-0.231684621095551,0.0153023668196266,
-0.00615185576425954));
#30233=CARTESIAN_POINT('Ctrl Pts',(-0.231836145719153,0.0152396689262739,
-0.00627130000767094));
#30234=CARTESIAN_POINT('Ctrl Pts',(-0.231987452488494,0.0151741955395839,
-0.00638985441608159));
#30235=CARTESIAN_POINT('Ctrl Pts',(-0.232137421202335,0.0151053986626134,
-0.0065083426471185));
#30236=CARTESIAN_POINT('Ctrl Pts',(-0.232147808330346,0.0151006336556357,
-0.00651654937498939));
#30237=CARTESIAN_POINT('Ctrl Pts',(-0.232158189240001,0.0150958524418954,
-0.00652475591244986));
#30238=CARTESIAN_POINT('Ctrl Pts',(-0.232168563225385,0.0150910549860577,
-0.0065329622985253));
#30239=CARTESIAN_POINT('Ctrl Pts',(-0.232307968201396,0.0150265870702838,
-0.00664323920866527));
#30240=CARTESIAN_POINT('Ctrl Pts',(-0.232446123690228,0.0149591860652729,
-0.00675348212769047));
#30241=CARTESIAN_POINT('Ctrl Pts',(-0.232580949251388,0.0148875018376449,
-0.00686495643825133));
#30242=CARTESIAN_POINT('Ctrl Pts',(-0.232725808015384,0.0148104831438382,
-0.00698472624084943));
#30243=CARTESIAN_POINT('Ctrl Pts',(-0.232866806881461,0.0147285158365232,
-0.00710592568938485));
#30244=CARTESIAN_POINT('Ctrl Pts',(-0.233001397075398,0.0146399654688394,
-0.00723005776422935));
#30245=CARTESIAN_POINT('Ctrl Pts',(-0.23301078614597,0.0146337881566073,
-0.00723871727185641));
#30246=CARTESIAN_POINT('Ctrl Pts',(-0.233020143486601,0.0146275789986391,
-0.00724739024669289));
#30247=CARTESIAN_POINT('Ctrl Pts',(-0.233029468522886,0.0146213373298964,
-0.0072560774060185));
#30248=CARTESIAN_POINT('Ctrl Pts',(-0.23315381576358,0.0145381060949952,
-0.00737191870235509));
#30249=CARTESIAN_POINT('Ctrl Pts',(-0.23327241953563,0.0144490980254842,
-0.00749027865120103));
#30250=CARTESIAN_POINT('Ctrl Pts',(-0.233382525334888,0.0143533124344016,
-0.00761063469097697));
#30251=CARTESIAN_POINT('Ctrl Pts',(-0.233500888177628,0.0142503436995081,
-0.00774001645928322));
#30252=CARTESIAN_POINT('Ctrl Pts',(-0.233609449565788,0.0141395435376383,
-0.00787171593683602));
#30253=CARTESIAN_POINT('Ctrl Pts',(-0.233704718238572,0.0140195979133241,
-0.00800520776939137));
#30254=CARTESIAN_POINT('Ctrl Pts',(-0.233711754187254,0.0140107394792492,
-0.00801506664173452));
#30255=CARTESIAN_POINT('Ctrl Pts',(-0.23371871727556,0.0140018315631178,
-0.00802493503816399));
#30256=CARTESIAN_POINT('Ctrl Pts',(-0.233725606005006,0.0139928736528168,
-0.00803481260910125));
#30257=CARTESIAN_POINT('Ctrl Pts',(-0.233765354917564,0.0139411852832834,
-0.00809180754648525));
#30258=CARTESIAN_POINT('Ctrl Pts',(-0.233802628113303,0.0138878323304247,
-0.00814910802237563));
#30259=CARTESIAN_POINT('Ctrl Pts',(-0.233837278186415,0.0138329085468894,
-0.00820649113639346));
#30260=CARTESIAN_POINT('Ctrl Pts',(-0.233898260900202,0.0137362449306085,
-0.0083074830739002));
#30261=CARTESIAN_POINT('Ctrl Pts',(-0.233951125609911,0.0136347095732914,
-0.00840873442372893));
#30262=CARTESIAN_POINT('Ctrl Pts',(-0.233995079511644,0.0135287531593584,
-0.00850908837254629));
#30263=CARTESIAN_POINT('Ctrl Pts',(-0.234039033413378,0.0134227967454253,
-0.00860944232136365));
#30264=CARTESIAN_POINT('Ctrl Pts',(-0.234074079450773,0.0133124189875615,
-0.00870890006003178));
#30265=CARTESIAN_POINT('Ctrl Pts',(-0.234099371837349,0.0131980565381413,
-0.00880635042806751));
#30266=CARTESIAN_POINT('Ctrl Pts',(-0.234101929684424,0.0131864909369363,
-0.00881620569174632));
#30267=CARTESIAN_POINT('Ctrl Pts',(-0.234104387698283,0.0131748847922406,
-0.00882604066222298));
#30268=CARTESIAN_POINT('Ctrl Pts',(-0.234106744905702,0.0131632387859299,
-0.00883585391535451));
#30269=CARTESIAN_POINT('Ctrl Pts',(-0.234135465605892,0.0130213414488917,
-0.00895542061057182));
#30270=CARTESIAN_POINT('Ctrl Pts',(-0.234149200249736,0.0128735165504675,
-0.00907176004245325));
#30271=CARTESIAN_POINT('Ctrl Pts',(-0.234148122016187,0.0127221513249176,
-0.00918311339548255));
#30272=CARTESIAN_POINT('Ctrl Pts',(-0.234147538652231,0.012640257177773,
-0.0092433596498313));
#30273=CARTESIAN_POINT('Ctrl Pts',(-0.234142623795018,0.0125573369859019,
-0.00930216102216956));
#30274=CARTESIAN_POINT('Ctrl Pts',(-0.2341334317926,0.0124737587188891,
-0.00935924909880171));
#30275=CARTESIAN_POINT('Ctrl Pts',(-0.234128835791391,0.0124319695853827,
-0.00938779313711778));
#30276=CARTESIAN_POINT('Ctrl Pts',(-0.234123170785509,0.0123900143644245,
-0.00941590693239571));
#30277=CARTESIAN_POINT('Ctrl Pts',(-0.23411644470908,0.0123479377552723,
-0.00944355743439764));
#30278=CARTESIAN_POINT('Ctrl Pts',(-0.234109718632652,0.0123058611461201,
-0.00947120793639956));
#30279=CARTESIAN_POINT('Ctrl Pts',(-0.234101931503068,0.01226366317307,
-0.00949839513366344));
#30280=CARTESIAN_POINT('Ctrl Pts',(-0.234093091644146,0.0122213891644512,
-0.00952508926526118));
#30281=CARTESIAN_POINT('Ctrl Pts',(-0.234090670032958,0.0122098085257659,
-0.00953240191677332));
#30282=CARTESIAN_POINT('Ctrl Pts',(-0.234088169321776,0.0121982220309786,
-0.00953967830460782));
#30283=CARTESIAN_POINT('Ctrl Pts',(-0.234085589675658,0.0121866306191717,
-0.00954691779081663));
#30284=CARTESIAN_POINT('Ctrl Pts',(-0.2340682957397,0.0121089218466376,
-0.00959545127374656));
#30285=CARTESIAN_POINT('Ctrl Pts',(-0.234047453702354,0.0120309920728459,
-0.00964232599577092));
#30286=CARTESIAN_POINT('Ctrl Pts',(-0.234023415843097,0.0119530144195835,
-0.00968754222491458));
#30287=CARTESIAN_POINT('Ctrl Pts',(-0.228104649974285,0.0163642118483275,
0.00231798200374011));
#30288=CARTESIAN_POINT('Ctrl Pts',(-0.228080473933464,0.0163672125078731,
0.00227403526561382));
#30289=CARTESIAN_POINT('Ctrl Pts',(-0.228056571982133,0.0163700464923153,
0.00222992337348044));
#30290=CARTESIAN_POINT('Ctrl Pts',(-0.228032949149827,0.0163727324397856,
0.00218564039839086));
#30291=CARTESIAN_POINT('Ctrl Pts',(-0.227887225499328,0.0163893014127747,
0.00191246922648189));
#30292=CARTESIAN_POINT('Ctrl Pts',(-0.227752115936573,0.0164000989794123,
0.00163267292450821));
#30293=CARTESIAN_POINT('Ctrl Pts',(-0.22762725738731,0.0164102722574105,
0.001347528898789));
#30294=CARTESIAN_POINT('Ctrl Pts',(-0.227593613235951,0.0164130135298889,
0.0012706945224726));
#30295=CARTESIAN_POINT('Ctrl Pts',(-0.227560713431936,0.0164157214331456,
0.00119347836067573));
#30296=CARTESIAN_POINT('Ctrl Pts',(-0.227528550504412,0.0164183289449134,
0.00111580340593609));
#30297=CARTESIAN_POINT('Ctrl Pts',(-0.227430952435461,0.0164262414122448,
0.000880099563898515));
#30298=CARTESIAN_POINT('Ctrl Pts',(-0.227340124895196,0.0164332189050637,
0.000640707665641815));
#30299=CARTESIAN_POINT('Ctrl Pts',(-0.227251433179574,0.0164371685419467,
0.000399944878391123));
#30300=CARTESIAN_POINT('Ctrl Pts',(-0.227202427891157,0.0164393508550662,
0.000266914980992263));
#30301=CARTESIAN_POINT('Ctrl Pts',(-0.227154074607713,0.016440605869286,
0.000133457190854296));
#30302=CARTESIAN_POINT('Ctrl Pts',(-0.227105591678119,0.0164410560897492,
1.32243616293715E-9));
#30303=CARTESIAN_POINT('Origin',(-0.226994617004166,0.00749997243979571,
0.00184285919272757));
#30304=CARTESIAN_POINT('',(-0.228031328918381,0.00748423226422772,0.010860760471908));
#30305=CARTESIAN_POINT('',(-0.225968509292903,0.0102911505109728,0.0103703808319117));
#30306=CARTESIAN_POINT('Ctrl Pts',(-0.225969748832453,0.0102900711236161,
0.0103707889115062));
#30307=CARTESIAN_POINT('Ctrl Pts',(-0.226289106570716,0.00978576005587371,
0.0105425714270296));
#30308=CARTESIAN_POINT('Ctrl Pts',(-0.22664061138589,0.00927176167283401,
0.0106681425457542));
#30309=CARTESIAN_POINT('Ctrl Pts',(-0.227339846850015,0.00833009565011997,
0.0108177785145977));
#30310=CARTESIAN_POINT('Ctrl Pts',(-0.227681836252118,0.00789982596134801,
0.0108536050057603));
#30311=CARTESIAN_POINT('Ctrl Pts',(-0.228033703347829,0.00748625084485732,
0.0108608393494597));
#30312=CARTESIAN_POINT('',(-0.225967560871587,0.00467023837789646,0.0103577170409566));
#30313=CARTESIAN_POINT('Ctrl Pts',(-0.228031308457579,0.00748420429971502,
0.0108607824347881));
#30314=CARTESIAN_POINT('Ctrl Pts',(-0.227821724450862,0.00723381073129729,
0.0108556558941106));
#30315=CARTESIAN_POINT('Ctrl Pts',(-0.227529404666869,0.00687470775376698,
0.0108331524160897));
#30316=CARTESIAN_POINT('Ctrl Pts',(-0.227175687258202,0.00641955626299225,
0.0107783812752486));
#30317=CARTESIAN_POINT('Ctrl Pts',(-0.226944206963435,0.00611293830577671,
0.010731009622336));
#30318=CARTESIAN_POINT('Ctrl Pts',(-0.226726702915377,0.00581110890073526,
0.0106729151048354));
#30319=CARTESIAN_POINT('Ctrl Pts',(-0.226565930211992,0.00557919413302389,
0.0106212588865583));
#30320=CARTESIAN_POINT('Ctrl Pts',(-0.226426475018125,0.00537259079248901,
0.0105700841876947));
#30321=CARTESIAN_POINT('Ctrl Pts',(-0.226359986159531,0.00527168795372337,
0.0105432010021426));
#30322=CARTESIAN_POINT('Ctrl Pts',(-0.226210309700029,0.00504332716767546,
0.0104795938046293));
#30323=CARTESIAN_POINT('Ctrl Pts',(-0.226074000007555,0.00483347349684773,
0.0104142248999611));
#30324=CARTESIAN_POINT('Ctrl Pts',(-0.225967561113698,0.00467023900632648,
0.0103577181008014));
#30325=CARTESIAN_POINT('',(-0.226088437963177,0.00749380654222876,0.0108173476998421));
#30326=CARTESIAN_POINT('Ctrl Pts',(-0.225965888685649,0.00467021151082653,
0.010357671607895));
#30327=CARTESIAN_POINT('Ctrl Pts',(-0.225942476168076,0.00559702753572744,
0.010664481305269));
#30328=CARTESIAN_POINT('Ctrl Pts',(-0.225998103434488,0.00657292145943362,
0.0108147034606632));
#30329=CARTESIAN_POINT('Ctrl Pts',(-0.226088521671434,0.00749380377234182,
0.0108173545262585));
#30330=CARTESIAN_POINT('Ctrl Pts',(-0.226088395525365,0.00749423713891311,
0.0108173519914327));
#30331=CARTESIAN_POINT('Ctrl Pts',(-0.226088209593573,0.00749614094361597,
0.010817349043451));
#30332=CARTESIAN_POINT('Ctrl Pts',(-0.226088023861152,0.0074980445644577,
0.0108173454950728));
#30333=CARTESIAN_POINT('Ctrl Pts',(-0.225999185723901,0.00840946053812611,
0.0108153591200668));
#30334=CARTESIAN_POINT('Ctrl Pts',(-0.225945309305692,0.00937289305355034,
0.0106696121468602));
#30335=CARTESIAN_POINT('Ctrl Pts',(-0.225967999251384,0.010289620296038,
0.0103708969367641));
#30336=CARTESIAN_POINT('Ctrl Pts',(-0.185723055456903,0.0169037490465727,
0.00243669718465323));
#30337=CARTESIAN_POINT('Ctrl Pts',(-0.232326704333039,0.0164203047763951,
0.00231142721965166));
#30338=CARTESIAN_POINT('Ctrl Pts',(-0.185723055456903,0.0169917319681535,
0.0020581868105832));
#30339=CARTESIAN_POINT('Ctrl Pts',(-0.232326704333039,0.0164327431878904,
0.00190716238014556));
#30340=CARTESIAN_POINT('Ctrl Pts',(-0.185723055456904,0.0171348389058692,
0.00126455176521327));
#30341=CARTESIAN_POINT('Ctrl Pts',(-0.232326704333039,0.0164529746481233,
0.00113116956517427));
#30342=CARTESIAN_POINT('Ctrl Pts',(-0.185723055456903,0.0172123852537007,
-4.57104323127425E-14));
#30343=CARTESIAN_POINT('Ctrl Pts',(-0.232326704333039,0.0164639376096499,
-5.12643732643055E-15));
#30344=CARTESIAN_POINT('Ctrl Pts',(-0.185723055456904,0.0171348389058572,
-0.00126455176530287));
#30345=CARTESIAN_POINT('Ctrl Pts',(-0.232326704333039,0.0164529746481216,
-0.00113116956518479));
#30346=CARTESIAN_POINT('Ctrl Pts',(-0.185723055456903,0.0169917319681347,
-0.00205818681066974));
#30347=CARTESIAN_POINT('Ctrl Pts',(-0.232326704333039,0.0164327431878878,
-0.00190716238015681));
#30348=CARTESIAN_POINT('Ctrl Pts',(-0.185723055456903,0.0166573800151943,
-0.00349659872622789));
#30349=CARTESIAN_POINT('Ctrl Pts',(-0.232326704333039,0.0163854748419384,
-0.00344344619644609));
#30350=CARTESIAN_POINT('Ctrl Pts',(-0.185723055456904,0.0158049536659853,
-0.00552554202981291));
#30351=CARTESIAN_POINT('Ctrl Pts',(-0.23232670433304,0.0158790365063827,
-0.00570322401511438));
#30352=CARTESIAN_POINT('Ctrl Pts',(-0.185723055456903,0.0136025708308564,
-0.00796594412460981));
#30353=CARTESIAN_POINT('Ctrl Pts',(-0.232326704333039,0.0138912669883084,
-0.00858048214849728));
#30354=CARTESIAN_POINT('Ctrl Pts',(-0.185723055456904,0.0107282744647946,
-0.00954209114738551));
#30355=CARTESIAN_POINT('Ctrl Pts',(-0.23232670433304,0.0109544909042364,
-0.010506785011137));
#30356=CARTESIAN_POINT('Ctrl Pts',(-0.185723055456903,0.00749999999987153,
-0.0100866616277759));
#30357=CARTESIAN_POINT('Ctrl Pts',(-0.232326704333039,0.00749999999987138,
-0.0111842362468306));
#30358=CARTESIAN_POINT('Ctrl Pts',(-0.185723055456904,0.00427172553496278,
-0.00954209114730134));
#30359=CARTESIAN_POINT('Ctrl Pts',(-0.23232670433304,0.00404550909552549,
-0.0105067850110401));
#30360=CARTESIAN_POINT('Ctrl Pts',(-0.185723055456903,0.00139742916894219,
-0.0079659441244508));
#30361=CARTESIAN_POINT('Ctrl Pts',(-0.232326704333039,0.00110873301150744,
-0.00858048214831799));
#30362=CARTESIAN_POINT('Ctrl Pts',(-0.185723055456904,-0.000804953666122893,
-0.00552554202959671));
#30363=CARTESIAN_POINT('Ctrl Pts',(-0.23232670433304,-0.000879036506486045,
-0.00570322401487933));
#30364=CARTESIAN_POINT('Ctrl Pts',(-0.185723055456903,-0.00165738001527906,
-0.00349659872598971));
#30365=CARTESIAN_POINT('Ctrl Pts',(-0.232326704333039,-0.0013854748419783,
-0.00344344619619682));
#30366=CARTESIAN_POINT('Ctrl Pts',(-0.185723055456903,-0.00199173196817847,
-0.00205818681044279));
#30367=CARTESIAN_POINT('Ctrl Pts',(-0.232326704333039,-0.00143274318789395,
-0.00190716237992731));
#30368=CARTESIAN_POINT('Ctrl Pts',(-0.185723055456903,-0.00213483890587743,
-0.00126455176511326));
#30369=CARTESIAN_POINT('Ctrl Pts',(-0.232326704333039,-0.00145297464812447,
-0.001131169564997));
#30370=CARTESIAN_POINT('Ctrl Pts',(-0.185723055456904,-0.00221238525369828,
8.33588010327838E-14));
#30371=CARTESIAN_POINT('Ctrl Pts',(-0.232326704333039,-0.0014639376096495,
1.20148665217339E-13));
#30372=CARTESIAN_POINT('Ctrl Pts',(-0.185723055456903,-0.00213483890585875,
0.00126455176527974));
#30373=CARTESIAN_POINT('Ctrl Pts',(-0.232326704333039,-0.00145297464812182,
0.00113116956523674));
#30374=CARTESIAN_POINT('Ctrl Pts',(-0.185723055456903,-0.00199173196814768,
0.00205818681060856));
#30375=CARTESIAN_POINT('Ctrl Pts',(-0.232326704333039,-0.0014327431878896,
0.00190716238016579));
#30376=CARTESIAN_POINT('Ctrl Pts',(-0.185723055456903,-0.00165738001522438,
0.00349659872621544));
#30377=CARTESIAN_POINT('Ctrl Pts',(-0.232326704333039,-0.00138547484194287,
0.00344344619705013));
#30378=CARTESIAN_POINT('Ctrl Pts',(-0.185723055456904,-0.000804955358563482,
0.00552554230330677));
#30379=CARTESIAN_POINT('Ctrl Pts',(-0.232326704333039,-0.000879051981413446,
0.0057032265164018));
#30380=CARTESIAN_POINT('Ctrl Pts',(-0.185723055456903,0.00139743580946407,
0.00796594412565152));
#30381=CARTESIAN_POINT('Ctrl Pts',(-0.232326704333039,0.00110879372578601,
0.00858048215857438));
#30382=CARTESIAN_POINT('Ctrl Pts',(-0.185723055456904,0.00427172361958147,
0.0095420921652245));
#30383=CARTESIAN_POINT('Ctrl Pts',(-0.232326704333039,0.0040454915818506,
0.0105067943176977));
#30384=CARTESIAN_POINT('Ctrl Pts',(-0.185723055456904,0.00750000000000269,
0.0100866612741451));
#30385=CARTESIAN_POINT('Ctrl Pts',(-0.23232670433304,0.00749999999999982,
0.011184233013541));
#30386=CARTESIAN_POINT('Ctrl Pts',(-0.185723055456904,0.0107282763804236,
0.00954209216522276));
#30387=CARTESIAN_POINT('Ctrl Pts',(-0.232326704333039,0.010954508418149,
0.0105067943176979));
#30388=CARTESIAN_POINT('Ctrl Pts',(-0.185723055456904,0.0136025641905403,
0.00796594412564821));
#30389=CARTESIAN_POINT('Ctrl Pts',(-0.23232670433304,0.0138912062742137,
0.00858048215857484));
#30390=CARTESIAN_POINT('Ctrl Pts',(-0.185723055456904,0.0158049553585666,
0.0055255423033021));
#30391=CARTESIAN_POINT('Ctrl Pts',(-0.232326704333039,0.0158790519814133,
0.00570322651640249));
#30392=CARTESIAN_POINT('Ctrl Pts',(-0.185723055456903,0.0166573800152265,
0.00349659872621015));
#30393=CARTESIAN_POINT('Ctrl Pts',(-0.232326704333039,0.0163854748419429,
0.00344344619705094));
#30394=CARTESIAN_POINT('Ctrl Pts',(-0.185723055456903,0.0169037490465727,
0.00243669718465325));
#30395=CARTESIAN_POINT('Ctrl Pts',(-0.232326704333039,0.0164203047763951,
0.00231142721965168));
#30396=CARTESIAN_POINT('',(-0.214999728174719,0.0156143096410472,-0.00564621361629089));
#30397=CARTESIAN_POINT('Ctrl Pts',(-0.220090794747946,0.0165472343306677,
0.00234431717574848));
#30398=CARTESIAN_POINT('Ctrl Pts',(-0.220117505055273,0.0165517330921288,
0.00228542154256059));
#30399=CARTESIAN_POINT('Ctrl Pts',(-0.220143226024636,0.0165561317703932,
0.00222617711841132));
#30400=CARTESIAN_POINT('Ctrl Pts',(-0.220167930171668,0.0165604182112109,
0.00216658683604705));
#30401=CARTESIAN_POINT('Ctrl Pts',(-0.220302085046398,0.0165836955553021,
0.00184298420951398));
#30402=CARTESIAN_POINT('Ctrl Pts',(-0.220406320979476,0.0166037523754693,
0.00150806229365304));
#30403=CARTESIAN_POINT('Ctrl Pts',(-0.220478938005581,0.0166181019152006,
0.00116601824206587));
#30404=CARTESIAN_POINT('Ctrl Pts',(-0.220559927566779,0.0166341059157574,
0.000784537491144179));
#30405=CARTESIAN_POINT('Ctrl Pts',(-0.220601586758498,0.0166429502091465,
0.000394001417140767));
#30406=CARTESIAN_POINT('Ctrl Pts',(-0.22060155721139,0.0166430032112023,
3.29174539469179E-6));
#30407=CARTESIAN_POINT('Ctrl Pts',(-0.220601527573304,0.0166430563764536,
-0.000388620937738244));
#30408=CARTESIAN_POINT('Ctrl Pts',(-0.220559550159924,0.0166342277778145,
-0.000781963648253663));
#30409=CARTESIAN_POINT('Ctrl Pts',(-0.220478178797353,0.016618112703623,
-0.00116602012469409));
#30410=CARTESIAN_POINT('Ctrl Pts',(-0.220405693171807,0.0166037573924105,
-0.00150813770832684));
#30411=CARTESIAN_POINT('Ctrl Pts',(-0.220301947463313,0.0165836800531986,
-0.00184305410985848));
#30412=CARTESIAN_POINT('Ctrl Pts',(-0.220168746900573,0.0165605041990195,
-0.0021653437607661));
#30413=CARTESIAN_POINT('Ctrl Pts',(-0.220143927401298,0.016556185800627,
-0.00222539656829727));
#30414=CARTESIAN_POINT('Ctrl Pts',(-0.2201180830146,0.0165517570763484,
-0.00228504938166036));
#30415=CARTESIAN_POINT('Ctrl Pts',(-0.22009123609363,0.0165472297523478,
-0.00234431598932238));
#30416=CARTESIAN_POINT('Ctrl Pts',(-0.219965170557077,0.0165259707211935,
-0.00262261519179285));
#30417=CARTESIAN_POINT('Ctrl Pts',(-0.219816999384638,0.0164925356057389,
-0.00288799098246844));
#30418=CARTESIAN_POINT('Ctrl Pts',(-0.219649037008359,0.016450115766149,
-0.00314010411404311));
#30419=CARTESIAN_POINT('Ctrl Pts',(-0.219445305358693,0.0163986621960713,
-0.00344590726672758));
#30420=CARTESIAN_POINT('Ctrl Pts',(-0.219212476942563,0.0163339394016627,
-0.00373144395556523));
#30421=CARTESIAN_POINT('Ctrl Pts',(-0.218955730221358,0.0162632438912369,
-0.00399091800136782));
#30422=CARTESIAN_POINT('Ctrl Pts',(-0.218442236778948,0.0161218528703853,
-0.00450986609297299));
#30423=CARTESIAN_POINT('Ctrl Pts',(-0.217833090583353,0.0159569647380836,
-0.00492410039029786));
#30424=CARTESIAN_POINT('Ctrl Pts',(-0.217158667709042,0.0158301156325255,
-0.00520782050433744));
#30425=CARTESIAN_POINT('Ctrl Pts',(-0.216794280228025,0.0157615796622844,
-0.00536111313661152));
#30426=CARTESIAN_POINT('Ctrl Pts',(-0.216410834738256,0.0157042273221352,
-0.00547647426027126));
#30427=CARTESIAN_POINT('Ctrl Pts',(-0.216017823748763,0.0156661782184681,
-0.00555035855253401));
#30428=CARTESIAN_POINT('Ctrl Pts',(-0.21568343433353,0.0156338045244352,
-0.00561322225341056));
#30429=CARTESIAN_POINT('Ctrl Pts',(-0.215342120180744,0.0156154190771227,
-0.00564609861724332));
#30430=CARTESIAN_POINT('Ctrl Pts',(-0.214999728174719,0.0156143096410472,
-0.00564621361629089));
#30431=CARTESIAN_POINT('',(-0.192768466211737,0.0155323575322467,-0.00565446565602188));
#30432=CARTESIAN_POINT('Ctrl Pts',(-0.192768471267355,0.0155311142648402,
-0.00565367499839099));
#30433=CARTESIAN_POINT('Ctrl Pts',(-0.200178878547941,0.015561682319149,
-0.00565299192900956));
#30434=CARTESIAN_POINT('Ctrl Pts',(-0.207589299767349,0.0155894984464108,
-0.00565023605674504));
#30435=CARTESIAN_POINT('Ctrl Pts',(-0.214999727535123,0.0156143038560219,
-0.00564622471354199));
#30436=CARTESIAN_POINT('',(-0.186116972293536,0.00807761530404598,-0.00989662596793202));
#30437=CARTESIAN_POINT('Ctrl Pts',(-0.192768467297635,0.0155311217264212,
-0.00565366324004662));
#30438=CARTESIAN_POINT('Ctrl Pts',(-0.192553538631542,0.0154928316295278,
-0.00571249831822603));
#30439=CARTESIAN_POINT('Ctrl Pts',(-0.192126359873203,0.015400452164298,
-0.00585256845739566));
#30440=CARTESIAN_POINT('Ctrl Pts',(-0.191427233283813,0.0151794461386251,
-0.00616010599105498));
#30441=CARTESIAN_POINT('Ctrl Pts',(-0.190868940070598,0.0149513426159108,
-0.00645166872819745));
#30442=CARTESIAN_POINT('Ctrl Pts',(-0.190250537576569,0.0146393883647952,
-0.00681374640562836));
#30443=CARTESIAN_POINT('Ctrl Pts',(-0.189729516535842,0.0143200690862221,
-0.00714747621846582));
#30444=CARTESIAN_POINT('Ctrl Pts',(-0.189019762799825,0.0138059199805297,
-0.00763060364735688));
#30445=CARTESIAN_POINT('Ctrl Pts',(-0.188408531961533,0.0132414344427084,
-0.00807836328034344));
#30446=CARTESIAN_POINT('Ctrl Pts',(-0.187828208926315,0.0125602396324074,
-0.00852034249444996));
#30447=CARTESIAN_POINT('Ctrl Pts',(-0.187449134948595,0.0120341789970749,
-0.00881634519754376));
#30448=CARTESIAN_POINT('Ctrl Pts',(-0.187090455089954,0.0114381778019524,
-0.00910151919630248));
#30449=CARTESIAN_POINT('Ctrl Pts',(-0.186797972413645,0.0108473589238396,
-0.00933775607435096));
#30450=CARTESIAN_POINT('Ctrl Pts',(-0.186527846028905,0.0101622086658462,
-0.00955771999823304));
#30451=CARTESIAN_POINT('Ctrl Pts',(-0.186261990169622,0.00925438874498978,
-0.00977599514646285));
#30452=CARTESIAN_POINT('Ctrl Pts',(-0.186150558186061,0.00854952262296873,
-0.00986894325761661));
#30453=CARTESIAN_POINT('Ctrl Pts',(-0.186117379249033,0.0080775870920664,
-0.00989663768469957));
#30454=CARTESIAN_POINT('',(-0.186100495884658,0.00793881407698417,-0.00990361580204106));
#30455=CARTESIAN_POINT('Ctrl Pts',(-0.186100495884658,0.00793881407698417,
-0.00990361580204106));
#30456=CARTESIAN_POINT('Ctrl Pts',(-0.186107265118205,0.00798254987096854,
-0.00990176581450937));
#30457=CARTESIAN_POINT('Ctrl Pts',(-0.186113922409534,0.0080335687668118,
-0.00989921262958112));
#30458=CARTESIAN_POINT('Ctrl Pts',(-0.186116958557054,0.00807758863112322,
-0.00989662810000007));
#30459=CARTESIAN_POINT('',(-0.185999364351498,0.00750000000000023,-0.00991138348459597));
#30460=CARTESIAN_POINT('Ctrl Pts',(-0.185999469845766,0.00749998739549284,
-0.00991138532823997));
#30461=CARTESIAN_POINT('Ctrl Pts',(-0.186001338958666,0.00750760781264758,
-0.00991142760973324));
#30462=CARTESIAN_POINT('Ctrl Pts',(-0.186009114261658,0.00753659870661198,
-0.00991164463711701));
#30463=CARTESIAN_POINT('Ctrl Pts',(-0.18602099569412,0.00758276948028511,
-0.00991151377077237));
#30464=CARTESIAN_POINT('Ctrl Pts',(-0.186026938057374,0.0076058612673871,
-0.00991144831945915));
#30465=CARTESIAN_POINT('Ctrl Pts',(-0.186033907335661,0.00763325051566056,
-0.00991130411162516));
#30466=CARTESIAN_POINT('Ctrl Pts',(-0.186042705129421,0.00766942125256383,
-0.0099108628019639));
#30467=CARTESIAN_POINT('Ctrl Pts',(-0.18605150292318,0.00770559198946711,
-0.00991042149230265));
#30468=CARTESIAN_POINT('Ctrl Pts',(-0.186062131323826,0.00775054205776099,
-0.00990959055677255));
#30469=CARTESIAN_POINT('Ctrl Pts',(-0.186070367106067,0.00778657725573298,
-0.00990869847733454));
#30470=CARTESIAN_POINT('Ctrl Pts',(-0.186086838670548,0.00785864765167694,
-0.00990691431845853));
#30471=CARTESIAN_POINT('Ctrl Pts',(-0.18609372665111,0.00789507828299981,
-0.00990546578957274));
#30472=CARTESIAN_POINT('Ctrl Pts',(-0.186100495884658,0.00793881407698417,
-0.00990361580204106));
#30473=CARTESIAN_POINT('',(-0.186096190050249,0.0070814223423058,-0.00990442392752799));
#30474=CARTESIAN_POINT('Ctrl Pts',(-0.186096190050249,0.0070814223423058,
-0.00990442392752799));
#30475=CARTESIAN_POINT('Ctrl Pts',(-0.186077709288058,0.00718824343638535,
-0.00990892115509886));
#30476=CARTESIAN_POINT('Ctrl Pts',(-0.186046718946517,0.00732820276343046,
-0.00991245346926289));
#30477=CARTESIAN_POINT('Ctrl Pts',(-0.185999469351116,0.00750001479860198,
-0.00991138531705731));
#30478=CARTESIAN_POINT('',(-0.186116972875644,0.00692238473624832,-0.00989662598588015));
#30479=CARTESIAN_POINT('Ctrl Pts',(-0.186116959160015,0.00692241144484341,
-0.00989662811818303));
#30480=CARTESIAN_POINT('Ctrl Pts',(-0.186114180722263,0.00696269561858531,
-0.0098989933157357));
#30481=CARTESIAN_POINT('Ctrl Pts',(-0.186107547814753,0.00701580747228393,
-0.00990194593950673));
#30482=CARTESIAN_POINT('Ctrl Pts',(-0.186096190050249,0.0070814223423058,
-0.00990442392752799));
#30483=CARTESIAN_POINT('',(-0.192768468047837,-0.000531121860071518,-0.00565366303468581));
#30484=CARTESIAN_POINT('Ctrl Pts',(-0.186117379249032,0.00692241290794315,
-0.00989663768470023));
#30485=CARTESIAN_POINT('Ctrl Pts',(-0.186150547404768,0.00645063072958828,
-0.00986895225675147));
#30486=CARTESIAN_POINT('Ctrl Pts',(-0.186261932611995,0.00574597187644414,
-0.00977604664100172));
#30487=CARTESIAN_POINT('Ctrl Pts',(-0.186527643355928,0.00483841251243376,
-0.0095578911982986));
#30488=CARTESIAN_POINT('Ctrl Pts',(-0.186797662606925,0.00415336530792349,
-0.00933800703012731));
#30489=CARTESIAN_POINT('Ctrl Pts',(-0.187089867547376,0.00356288427383543,
-0.00910198973672387));
#30490=CARTESIAN_POINT('Ctrl Pts',(-0.187448677686789,0.00296655606527825,
-0.00881670870907843));
#30491=CARTESIAN_POINT('Ctrl Pts',(-0.18782652671858,0.00244197053597788,
-0.00852164547016561));
#30492=CARTESIAN_POINT('Ctrl Pts',(-0.188405806126936,0.00176150898886227,
-0.00808041909580759));
#30493=CARTESIAN_POINT('Ctrl Pts',(-0.189013908627982,0.00119895188987953,
-0.00763477774095243));
#30494=CARTESIAN_POINT('Ctrl Pts',(-0.189725220968284,0.000682672430095184,
-0.00715027528319919));
#30495=CARTESIAN_POINT('Ctrl Pts',(-0.19024844359526,0.000361785469120427,
-0.00681503282008351));
#30496=CARTESIAN_POINT('Ctrl Pts',(-0.19086389333632,5.11131219040483E-5,
-0.00645458607971318));
#30497=CARTESIAN_POINT('Ctrl Pts',(-0.191418362838009,-0.000176268882400119,
-0.00616437018057724));
#30498=CARTESIAN_POINT('Ctrl Pts',(-0.192123247609021,-0.000399817339443113,
-0.00585356940633785));
#30499=CARTESIAN_POINT('Ctrl Pts',(-0.192552358590443,-0.000492621421588735,
-0.00571282131797196));
#30500=CARTESIAN_POINT('Ctrl Pts',(-0.192768468047837,-0.000531121860071518,
-0.00565366303468581));
#30501=CARTESIAN_POINT('',(-0.214999728174719,-0.000614309641048097,-0.00564621361629096));
#30502=CARTESIAN_POINT('Ctrl Pts',(-0.214999727480966,-0.000614303178801771,
-0.00564622601275543));
#30503=CARTESIAN_POINT('Ctrl Pts',(-0.207589299761315,-0.000589501940551079,
-0.00565022926213394));
#30504=CARTESIAN_POINT('Ctrl Pts',(-0.200178878524307,-0.000561687127315493,
-0.00565298419618518));
#30505=CARTESIAN_POINT('Ctrl Pts',(-0.192768471170869,-0.000531115971629387,
-0.00565367231393811));
#30506=CARTESIAN_POINT('',(-0.214999728175217,-0.000614308556352198,0.00564621407322208));
#30507=CARTESIAN_POINT('Ctrl Pts',(-0.214999728174719,-0.000614309641048097,
-0.00564621361629096));
#30508=CARTESIAN_POINT('Ctrl Pts',(-0.21573850211318,-0.000616703454117696,
-0.0056459654846237));
#30509=CARTESIAN_POINT('Ctrl Pts',(-0.217223304763531,-0.000790930473226734,
-0.00533944491480338));
#30510=CARTESIAN_POINT('Ctrl Pts',(-0.218746260771501,-0.00120277693812265,
-0.00430233875808143));
#30511=CARTESIAN_POINT('Ctrl Pts',(-0.219676141040077,-0.00146568982444615,
-0.00316380099642141));
#30512=CARTESIAN_POINT('Ctrl Pts',(-0.220374968741458,-0.0016004092271873,
-0.00185706856797699));
#30513=CARTESIAN_POINT('Ctrl Pts',(-0.22075211591453,-0.00167135211208185,
-4.24711954689424E-6));
#30514=CARTESIAN_POINT('Ctrl Pts',(-0.220376469572862,-0.0016005504927844,
0.00185335284380898));
#30515=CARTESIAN_POINT('Ctrl Pts',(-0.219678171970889,-0.0014662512330438,
0.00316084634731099));
#30516=CARTESIAN_POINT('Ctrl Pts',(-0.218746792417777,-0.00120287411926783,
0.00430240406335488));
#30517=CARTESIAN_POINT('Ctrl Pts',(-0.217223954144023,-0.000791566407931855,
0.00533790744423129));
#30518=CARTESIAN_POINT('Ctrl Pts',(-0.215744536661587,-0.000616721921800092,
0.00564596392366559));
#30519=CARTESIAN_POINT('Ctrl Pts',(-0.214999728175217,-0.000614308556352198,
0.00564621407322208));
#30520=CARTESIAN_POINT('',(-0.192768467995111,-0.000531121635157075,0.00565366251134238));
#30521=CARTESIAN_POINT('Ctrl Pts',(-0.192768468030036,-0.00053111358431346,
0.00565367517106098));
#30522=CARTESIAN_POINT('Ctrl Pts',(-0.200178876390431,-0.00056168139528131,
0.00565299213563766));
#30523=CARTESIAN_POINT('Ctrl Pts',(-0.20758929868895,-0.000589497383419672,
0.00565023637807718));
#30524=CARTESIAN_POINT('Ctrl Pts',(-0.214999727535667,-0.000614302771609743,
0.00564622516979113));
#30525=CARTESIAN_POINT('Ctrl Pts',(-0.192768462908899,-0.000531120840243836,
0.00565366372878243));
#30526=CARTESIAN_POINT('Ctrl Pts',(-0.192552801493728,-0.000492700078165468,
0.00571269932462467));
#30527=CARTESIAN_POINT('Ctrl Pts',(-0.192124458781824,-0.000400070483159716,
0.00585317259136444));
#30528=CARTESIAN_POINT('Ctrl Pts',(-0.191421518043594,-0.000177397871371761,
0.00616285200383273));
#30529=CARTESIAN_POINT('Ctrl Pts',(-0.190866264373635,5.00112782188013E-5,
0.0064532469370294));
#30530=CARTESIAN_POINT('Ctrl Pts',(-0.190250499708039,0.00036063440493152,
0.00681376176935662));
#30531=CARTESIAN_POINT('Ctrl Pts',(-0.189727113151071,0.000681405916027528,
0.00714901524785936));
#30532=CARTESIAN_POINT('Ctrl Pts',(-0.189015316243516,0.00119775071995663,
0.0076337612796465));
#30533=CARTESIAN_POINT('Ctrl Pts',(-0.188406936412897,0.00176034576435437,
0.00807957177832989));
#30534=CARTESIAN_POINT('Ctrl Pts',(-0.187827448741697,0.0024407808400988,
0.00852093044215746));
#30535=CARTESIAN_POINT('Ctrl Pts',(-0.187449339498272,0.00296554636590169,
0.00881618573576621));
#30536=CARTESIAN_POINT('Ctrl Pts',(-0.187090406949154,0.00356188460332164,
0.00910155665687714));
#30537=CARTESIAN_POINT('Ctrl Pts',(-0.186797998280614,0.00415259607751215,
0.00933773637730888));
#30538=CARTESIAN_POINT('Ctrl Pts',(-0.186527846972215,0.00483778154507395,
0.00955771997476887));
#30539=CARTESIAN_POINT('Ctrl Pts',(-0.186352129082402,0.00543781226559763,
0.0097019893028026));
#30540=CARTESIAN_POINT('Ctrl Pts',(-0.18626928197773,0.0058180982296112,
0.00977044711790262));
#30541=CARTESIAN_POINT('Ctrl Pts',(-0.186240951883218,0.00596786139892777,
0.00979390672266723));
#30542=CARTESIAN_POINT('',(-0.190954534254184,0.00352393167612197,0.00915627380277794));
#30543=CARTESIAN_POINT('Ctrl Pts',(-0.190954534310351,0.00352393181819051,
0.00915627369813247));
#30544=CARTESIAN_POINT('Ctrl Pts',(-0.19094632664236,0.00362759799902633,
0.00920360461773492));
#30545=CARTESIAN_POINT('Ctrl Pts',(-0.19093545240702,0.00376077062731066,
0.00926213843487851));
#30546=CARTESIAN_POINT('Ctrl Pts',(-0.190924142450368,0.00391598246737441,
0.00932477587001288));
#30547=CARTESIAN_POINT('Ctrl Pts',(-0.190918487472042,0.00399358838740629,
0.00935609458758006));
#30548=CARTESIAN_POINT('Ctrl Pts',(-0.190912721390573,0.00407665332153031,
0.0093885448454316));
#30549=CARTESIAN_POINT('Ctrl Pts',(-0.190906716936133,0.00417452738184911,
0.00942477637181333));
#30550=CARTESIAN_POINT('Ctrl Pts',(-0.190904087456934,0.00421738852908344,
0.00944064293320573));
#30551=CARTESIAN_POINT('Ctrl Pts',(-0.190901414383111,0.00426310553578685,
0.00945719956921678));
#30552=CARTESIAN_POINT('Ctrl Pts',(-0.190898866584097,0.00430862868740381,
0.00947328023960344));
#30553=CARTESIAN_POINT('Ctrl Pts',(-0.190895596446577,0.00436705832227904,
0.00949392001663707));
#30554=CARTESIAN_POINT('Ctrl Pts',(-0.19089253268803,0.00442517237653945,
0.00951376128014555));
#30555=CARTESIAN_POINT('Ctrl Pts',(-0.190890032378645,0.00447636934260713,
0.00953078141909249));
#30556=CARTESIAN_POINT('Ctrl Pts',(-0.190885584051554,0.00456745441089561,
0.00956106212979344));
#30557=CARTESIAN_POINT('Ctrl Pts',(-0.190882904338584,0.00463651587043694,
0.00958281759923728));
#30558=CARTESIAN_POINT('Ctrl Pts',(-0.190880531451168,0.00471329694686104,
0.00960615849718409));
#30559=CARTESIAN_POINT('Ctrl Pts',(-0.190878158563751,0.00479007802328515,
0.00962949939513091));
#30560=CARTESIAN_POINT('Ctrl Pts',(-0.190876100121299,0.00487468124703968,
0.00965407619729078));
#30561=CARTESIAN_POINT('Ctrl Pts',(-0.190874739449471,0.00495722266620057,
0.00967681019044906));
#30562=CARTESIAN_POINT('Ctrl Pts',(-0.190873378777642,0.00503976408536146,
0.00969954418360734));
#30563=CARTESIAN_POINT('Ctrl Pts',(-0.190872712070185,0.00512019613320558,
0.0097206091211127));
#30564=CARTESIAN_POINT('Ctrl Pts',(-0.190872856109916,0.00520802569623835,
0.00974229097280704));
#30565=CARTESIAN_POINT('Ctrl Pts',(-0.190873000149648,0.00529585525927111,
0.00976397282450137));
#30566=CARTESIAN_POINT('Ctrl Pts',(-0.190873962538537,0.00539117015513677,
0.00978592595965043));
#30567=CARTESIAN_POINT('Ctrl Pts',(-0.190875081406697,0.00546555964115924,
0.00980214880648675));
#30568=CARTESIAN_POINT('Ctrl Pts',(-0.190876200274857,0.0055399491271817,
0.00981837165332308));
#30569=CARTESIAN_POINT('Ctrl Pts',(-0.190877463096275,0.00559329168544975,
0.00982942944626223));
#30570=CARTESIAN_POINT('Ctrl Pts',(-0.190879780185886,0.00566986525134087,
0.00984441872877178));
#30571=CARTESIAN_POINT('Ctrl Pts',(-0.190882097275498,0.005746438817232,
0.00985940801128134));
#30572=CARTESIAN_POINT('Ctrl Pts',(-0.190885478987397,0.00584632900620433,
0.00987786397855303));
#30573=CARTESIAN_POINT('Ctrl Pts',(-0.19089009347875,0.00595176589423788,
0.00989528793015295));
#30574=CARTESIAN_POINT('Ctrl Pts',(-0.190890175357787,0.00595363675501567,
0.00989559709887227));
#30575=CARTESIAN_POINT('Ctrl Pts',(-0.190890257625829,0.00595550936098245,
0.00989590599388756));
#30576=CARTESIAN_POINT('Ctrl Pts',(-0.190890340272952,0.00595738356554221,
0.00989621458805049));
#30577=CARTESIAN_POINT('',(-0.19155098689841,0.00310490369588466,0.00896382639094083));
#30578=CARTESIAN_POINT('Ctrl Pts',(-0.190954506945739,0.00352390963011318,
0.00915626296509413));
#30579=CARTESIAN_POINT('Ctrl Pts',(-0.190982278824996,0.00349425566396222,
0.00914324986724137));
#30580=CARTESIAN_POINT('Ctrl Pts',(-0.19101331050615,0.00346142897667129,
0.00912863700187908));
#30581=CARTESIAN_POINT('Ctrl Pts',(-0.191107038094531,0.00337454011628438,
0.00908963731875738));
#30582=CARTESIAN_POINT('Ctrl Pts',(-0.191230009334021,0.00328208373715836,
0.00904716953434546));
#30583=CARTESIAN_POINT('Ctrl Pts',(-0.191371313193077,0.00319458454024611,
0.00900637041021926));
#30584=CARTESIAN_POINT('Ctrl Pts',(-0.19149550396465,0.0031312929367007,
0.00897638835379347));
#30585=CARTESIAN_POINT('Ctrl Pts',(-0.19155044938687,0.00310515928473931,
0.00896394806017618));
#30586=CARTESIAN_POINT('',(-0.192244127898258,0.0028370269379133,0.00883272019762234));
#30587=CARTESIAN_POINT('Ctrl Pts',(-0.19155098689841,0.00310490369588466,
0.00896382639094083));
#30588=CARTESIAN_POINT('Ctrl Pts',(-0.191605706721645,0.00307889106552294,
0.00895144323092614));
#30589=CARTESIAN_POINT('Ctrl Pts',(-0.191677276008409,0.00304801612626287,
0.00893663613670419));
#30590=CARTESIAN_POINT('Ctrl Pts',(-0.191792352343094,0.00300073160810067,
0.00891381119032522));
#30591=CARTESIAN_POINT('Ctrl Pts',(-0.19190916590961,0.00295569191589503,
0.00889185169317019));
#30592=CARTESIAN_POINT('Ctrl Pts',(-0.191939972002056,0.00294429797831757,
0.00888625973348703));
#30593=CARTESIAN_POINT('Ctrl Pts',(-0.192048790468399,0.0029037328706347,
0.00886629204061889));
#30594=CARTESIAN_POINT('Ctrl Pts',(-0.192155294606237,0.00286458613052319,
0.00884674800931049));
#30595=CARTESIAN_POINT('Ctrl Pts',(-0.192242576586721,0.00283267476154068,
0.00883054397400312));
#30596=CARTESIAN_POINT('',(-0.19208322262791,0.00464057435056716,0.00960976448008655));
#30597=CARTESIAN_POINT('Ctrl Pts',(-0.19208322262791,0.00464057435056716,
0.00960976448008655));
#30598=CARTESIAN_POINT('Ctrl Pts',(-0.192085206341064,0.00459342467188857,
0.00959502212455125));
#30599=CARTESIAN_POINT('Ctrl Pts',(-0.192087617750331,0.00454199577158409,
0.00957848718067775));
#30600=CARTESIAN_POINT('Ctrl Pts',(-0.192090642929679,0.0044854654686816,
0.00955971369095227));
#30601=CARTESIAN_POINT('Ctrl Pts',(-0.192093681203115,0.0044286904818797,
0.00954085894267279));
#30602=CARTESIAN_POINT('Ctrl Pts',(-0.192097341832823,0.00436678587514305,
0.00951968523993041));
#30603=CARTESIAN_POINT('Ctrl Pts',(-0.192101377292397,0.00430349575245546,
0.00949723790948274));
#30604=CARTESIAN_POINT('Ctrl Pts',(-0.192105910696384,0.00423239611949469,
0.00947202075255517));
#30605=CARTESIAN_POINT('Ctrl Pts',(-0.19211091713946,0.00415955363953229,
0.00944518465642903));
#30606=CARTESIAN_POINT('Ctrl Pts',(-0.19211604569542,0.00409011964816775,
0.00941867243889797));
#30607=CARTESIAN_POINT('Ctrl Pts',(-0.192135433288675,0.00382763679854969,
0.0093184477179726));
#30608=CARTESIAN_POINT('Ctrl Pts',(-0.192156497399979,0.00361313712343995,
0.00922457021543034));
#30609=CARTESIAN_POINT('Ctrl Pts',(-0.192178551157702,0.00340772429612771,
0.00912725829435275));
#30610=CARTESIAN_POINT('Ctrl Pts',(-0.192200186009473,0.00320621323724796,
0.00903179479037128));
#30611=CARTESIAN_POINT('Ctrl Pts',(-0.192222796816838,0.00301409159924088,
0.00893185014394745));
#30612=CARTESIAN_POINT('Ctrl Pts',(-0.19224448913935,0.00284151729909065,
0.00883554521382252));
#30613=CARTESIAN_POINT('',(-0.192075122449827,0.00543334712284603,0.00982163800799055));
#30614=CARTESIAN_POINT('Ctrl Pts',(-0.192075122449827,0.00543334712284603,
0.00982163800799055));
#30615=CARTESIAN_POINT('Ctrl Pts',(-0.192073745904168,0.00537589936645501,
0.00980887345605507));
#30616=CARTESIAN_POINT('Ctrl Pts',(-0.192072795708241,0.00532266174270566,
0.00979647660250808));
#30617=CARTESIAN_POINT('Ctrl Pts',(-0.192072170762121,0.00527270892376701,
0.00978447083173468));
#30618=CARTESIAN_POINT('Ctrl Pts',(-0.192071143546597,0.00519060214775848,
0.00976473710794001));
#30619=CARTESIAN_POINT('Ctrl Pts',(-0.192070999692292,0.0051174235825934,
0.00974584944479457));
#30620=CARTESIAN_POINT('Ctrl Pts',(-0.19207108592788,0.00508480464904163,
0.00973731727043851));
#30621=CARTESIAN_POINT('Ctrl Pts',(-0.192071129045674,0.00506849518226574,
0.00973305118326047));
#30622=CARTESIAN_POINT('Ctrl Pts',(-0.192071228710843,0.00506231357119921,
0.00973141845477906));
#30623=CARTESIAN_POINT('Ctrl Pts',(-0.192071444468926,0.00504813553730963,
0.00972765351664012));
#30624=CARTESIAN_POINT('Ctrl Pts',(-0.19207166022701,0.00503395750342006,
0.00972388857850117));
#30625=CARTESIAN_POINT('Ctrl Pts',(-0.192071992671388,0.00501179032802861,
0.00971796436653364));
#30626=CARTESIAN_POINT('Ctrl Pts',(-0.192072495237599,0.0049858984125824,
0.009710903448484));
#30627=CARTESIAN_POINT('Ctrl Pts',(-0.19207350037002,0.00493411458168996,
0.00969678161238471));
#30628=CARTESIAN_POINT('Ctrl Pts',(-0.192075184614482,0.00486741174909846,
0.00967817636683549));
#30629=CARTESIAN_POINT('Ctrl Pts',(-0.192077858011542,0.00478539381423263,
0.00965389070203072));
#30630=CARTESIAN_POINT('Ctrl Pts',(-0.192079277812855,0.00474183531206385,
0.0096409929475969));
#30631=CARTESIAN_POINT('Ctrl Pts',(-0.192080975907986,0.00469395101363589,
0.00962652426427693));
#30632=CARTESIAN_POINT('Ctrl Pts',(-0.19208322262791,0.00464057435056716,
0.00960976448008655));
#30633=CARTESIAN_POINT('Ctrl Pts',(-0.192094713079881,0.00595467555603429,
0.0099226782462026));
#30634=CARTESIAN_POINT('Ctrl Pts',(-0.192093438683974,0.0059288836017015,
0.00991841040641334));
#30635=CARTESIAN_POINT('Ctrl Pts',(-0.192092050254312,0.00590009560033358,
0.00991353641647854));
#30636=CARTESIAN_POINT('Ctrl Pts',(-0.192090655876427,0.0058695679699555,
0.00990820459990516));
#30637=CARTESIAN_POINT('Ctrl Pts',(-0.192086141620258,0.00577073569120594,
0.00989094300523516));
#30638=CARTESIAN_POINT('Ctrl Pts',(-0.19208157119045,0.00565371489836332,
0.00986856917129485));
#30639=CARTESIAN_POINT('Ctrl Pts',(-0.192078337556395,0.00554975597457726,
0.00984678202053675));
#30640=CARTESIAN_POINT('Ctrl Pts',(-0.192077071228137,0.00550904446530914,
0.00983824992191826));
#30641=CARTESIAN_POINT('Ctrl Pts',(-0.192076008513737,0.00547032319090132,
0.00982987069770896));
#30642=CARTESIAN_POINT('Ctrl Pts',(-0.192075122449827,0.00543334712284603,
0.00982163800799055));
#30643=CARTESIAN_POINT('',(-0.193087902622454,0.00259433627597418,0.00870850447702694));
#30644=CARTESIAN_POINT('Ctrl Pts',(-0.192891760060441,0.00595287508888906,
0.00994024214377629));
#30645=CARTESIAN_POINT('Ctrl Pts',(-0.192890566945838,0.00592739245907241,
0.00993600999446998));
#30646=CARTESIAN_POINT('Ctrl Pts',(-0.192884601854086,0.0057942541567979,
0.00991325429118574));
#30647=CARTESIAN_POINT('Ctrl Pts',(-0.192872041248742,0.0054401365750408,
0.00984514869329706));
#30648=CARTESIAN_POINT('Ctrl Pts',(-0.192866762099152,0.00495868049753787,
0.00972769113725174));
#30649=CARTESIAN_POINT('Ctrl Pts',(-0.192885277880319,0.00432843397316892,
0.00953146350645171));
#30650=CARTESIAN_POINT('Ctrl Pts',(-0.192925778339018,0.00382224510393984,
0.00933240208330745));
#30651=CARTESIAN_POINT('Ctrl Pts',(-0.19296164636954,0.00350616168796143,
0.00919061074969547));
#30652=CARTESIAN_POINT('Ctrl Pts',(-0.192985497265266,0.00331338011994894,
0.00909895014912776));
#30653=CARTESIAN_POINT('Ctrl Pts',(-0.193008594946383,0.00314020797556435,
0.00901202176798678));
#30654=CARTESIAN_POINT('Ctrl Pts',(-0.193020791858502,0.00305306311402364,
0.00896654755713946));
#30655=CARTESIAN_POINT('Ctrl Pts',(-0.193046579479833,0.00287167102747878,
0.0088696212197973));
#30656=CARTESIAN_POINT('Ctrl Pts',(-0.19306986918682,0.00271385629159264,
0.00878009081354476));
#30657=CARTESIAN_POINT('Ctrl Pts',(-0.193087902622454,0.00259433627597418,
0.00870850447702694));
#30658=CARTESIAN_POINT('',(-0.194289733361641,0.00259543694850618,0.00873259552391554));
#30659=CARTESIAN_POINT('',(-0.193087902747045,0.0025943401192753,0.00870849809117663));
#30660=CARTESIAN_POINT('Ctrl Pts',(-0.194289733361641,0.00259543694850618,
0.00873259552391554));
#30661=CARTESIAN_POINT('Ctrl Pts',(-0.194271528725811,0.00271568039656882,
0.00880482321695224));
#30662=CARTESIAN_POINT('Ctrl Pts',(-0.194255897964241,0.00282122439999286,
0.00886474330262958));
#30663=CARTESIAN_POINT('Ctrl Pts',(-0.194242056106171,0.00291670895493246,
0.00891714289225702));
#30664=CARTESIAN_POINT('Ctrl Pts',(-0.194235135148102,0.00296445143268365,
0.00894334279698027));
#30665=CARTESIAN_POINT('Ctrl Pts',(-0.194228662428445,0.00300970838330853,
0.00896761155435052));
#30666=CARTESIAN_POINT('Ctrl Pts',(-0.194223419901485,0.00304661531765659,
0.0089871258554761));
#30667=CARTESIAN_POINT('Ctrl Pts',(-0.194218177374525,0.00308352225200465,
0.00900664015660169));
#30668=CARTESIAN_POINT('Ctrl Pts',(-0.194214162614404,0.00311201443001013,
0.00902152057309972));
#30669=CARTESIAN_POINT('Ctrl Pts',(-0.194208252055201,0.00315520779816521,
0.00904365403355806));
#30670=CARTESIAN_POINT('Ctrl Pts',(-0.194202341495998,0.00319840116632029,
0.0090657874940164));
#30671=CARTESIAN_POINT('Ctrl Pts',(-0.194194539515255,0.00325640731426551,
0.00909495824185457));
#30672=CARTESIAN_POINT('Ctrl Pts',(-0.19418763059952,0.0033095193635379,
0.0091209708909162));
#30673=CARTESIAN_POINT('Ctrl Pts',(-0.194180721683785,0.00336263141281028,
0.00914698353997783));
#30674=CARTESIAN_POINT('Ctrl Pts',(-0.1941747028172,0.00341077872854798,
0.00916998462247426));
#30675=CARTESIAN_POINT('Ctrl Pts',(-0.194168967265586,0.00345787450382826,
0.00919205245244361));
#30676=CARTESIAN_POINT('Ctrl Pts',(-0.194157496162359,0.00355206605438881,
0.00923618811238231));
#30677=CARTESIAN_POINT('Ctrl Pts',(-0.194147158641889,0.00364205090957071,
0.00927657770576536));
#30678=CARTESIAN_POINT('Ctrl Pts',(-0.194137514962956,0.0037358380241254,
0.00931692735652691));
#30679=CARTESIAN_POINT('Ctrl Pts',(-0.194119406580828,0.0039119464284688,
0.0093926937626603));
#30680=CARTESIAN_POINT('Ctrl Pts',(-0.19410375587135,0.0041016834482665,
0.00946781093462956));
#30681=CARTESIAN_POINT('Ctrl Pts',(-0.194092490888446,0.004294996654283,
0.00953690694685357));
#30682=CARTESIAN_POINT('Ctrl Pts',(-0.19409175746337,0.00430758262571006,
0.00954140555537337));
#30683=CARTESIAN_POINT('Ctrl Pts',(-0.194091042628832,0.00432018336915257,
0.00954587951955885));
#30684=CARTESIAN_POINT('Ctrl Pts',(-0.194090346916936,0.00433279593942552,
0.00955032777148575));
#30685=CARTESIAN_POINT('Ctrl Pts',(-0.19407896547467,0.00453913025852806,
0.00962309858763756));
#30686=CARTESIAN_POINT('Ctrl Pts',(-0.194072700655243,0.00474875923096642,
0.00968875779931998));
#30687=CARTESIAN_POINT('Ctrl Pts',(-0.194070631885882,0.00494981833866685,
0.00974471116442283));
#30688=CARTESIAN_POINT('Ctrl Pts',(-0.194068563116522,0.00515087744636728,
0.00980066452952569));
#30689=CARTESIAN_POINT('Ctrl Pts',(-0.19407067236164,0.0053431217362215,
0.00984773853892592));
#30690=CARTESIAN_POINT('Ctrl Pts',(-0.194076586118239,0.00555334261219932,
0.00989187662448376));
#30691=CARTESIAN_POINT('Ctrl Pts',(-0.194079542996539,0.00565845305018821,
0.00991394566726268));
#30692=CARTESIAN_POINT('Ctrl Pts',(-0.19408345578846,0.00576810145447717,
0.00993506549656636));
#30693=CARTESIAN_POINT('Ctrl Pts',(-0.194088151554064,0.00587655136153835,
0.00995399441587651));
#30694=CARTESIAN_POINT('Ctrl Pts',(-0.194089210184997,0.00590100071357329,
0.00995826182213251));
#30695=CARTESIAN_POINT('Ctrl Pts',(-0.194090308396205,0.00592538822477612,
0.00996242241717579));
#30696=CARTESIAN_POINT('Ctrl Pts',(-0.194091473879223,0.00595018587709226,
0.00996655302891216));
#30697=CARTESIAN_POINT('',(-0.19508880402446,0.00259613937631384,0.00874861526161622));
#30698=CARTESIAN_POINT('Ctrl Pts',(-0.194890827700361,0.00594838029502342,
0.00998416681136753));
#30699=CARTESIAN_POINT('Ctrl Pts',(-0.194889713960232,0.00592436947855236,
0.00998014991521366));
#30700=CARTESIAN_POINT('Ctrl Pts',(-0.194883852863042,0.00579261937904974,
0.00995750870450058));
#30701=CARTESIAN_POINT('Ctrl Pts',(-0.19487142704807,0.00543995741384574,
0.00988940370129619));
#30702=CARTESIAN_POINT('Ctrl Pts',(-0.194866284257113,0.0049586687135079,
0.00977150277032712));
#30703=CARTESIAN_POINT('Ctrl Pts',(-0.194885044401134,0.00432865252952493,
0.00957453103971056));
#30704=CARTESIAN_POINT('Ctrl Pts',(-0.19492582233458,0.00382278364537034,
0.00937473168531034));
#30705=CARTESIAN_POINT('Ctrl Pts',(-0.194961893178176,0.00350696808990623,
0.00923242757156718));
#30706=CARTESIAN_POINT('Ctrl Pts',(-0.194985873725367,0.00331435951877626,
0.00914043502989879));
#30707=CARTESIAN_POINT('Ctrl Pts',(-0.195009093344523,0.00314135359488825,
0.00905319208558937));
#30708=CARTESIAN_POINT('Ctrl Pts',(-0.195021352135067,0.00305430708509385,
0.00900755901258544));
#30709=CARTESIAN_POINT('Ctrl Pts',(-0.195047271623395,0.00287311693036189,
0.00891029014674232));
#30710=CARTESIAN_POINT('Ctrl Pts',(-0.195070679357827,0.00271549678394977,
0.00882044735032797));
#30711=CARTESIAN_POINT('Ctrl Pts',(-0.19508880402446,0.00259613937631384,
0.00874861526161622));
#30712=CARTESIAN_POINT('',(-0.19629064847218,0.00259721050736435,0.00877274833518847));
#30713=CARTESIAN_POINT('',(-0.195088804147468,0.0025961431799468,0.00874860897199265));
#30714=CARTESIAN_POINT('Ctrl Pts',(-0.19629064847218,0.00259721050736436,
0.00877274833518847));
#30715=CARTESIAN_POINT('Ctrl Pts',(-0.196272353578319,0.0027173147463442,
0.00884523531704338));
#30716=CARTESIAN_POINT('Ctrl Pts',(-0.196256645487058,0.00282274836854239,
0.00890537208131317));
#30717=CARTESIAN_POINT('Ctrl Pts',(-0.196242734961374,0.00291813783584734,
0.00895796128107918));
#30718=CARTESIAN_POINT('Ctrl Pts',(-0.196235779668928,0.00296583277249766,
0.00898425599287699));
#30719=CARTESIAN_POINT('Ctrl Pts',(-0.196229274785596,0.00301104622815838,
0.0090086126430062));
#30720=CARTESIAN_POINT('Ctrl Pts',(-0.196224006516798,0.00304791619144044,
0.00902819648410093));
#30721=CARTESIAN_POINT('Ctrl Pts',(-0.196218738248,0.00308478615472249,
0.00904778032519565));
#30722=CARTESIAN_POINT('Ctrl Pts',(-0.196214704155585,0.00311324738212467,
0.00906271231000411));
#30723=CARTESIAN_POINT('Ctrl Pts',(-0.196208763690641,0.00315640258061905,
0.00908492642526198));
#30724=CARTESIAN_POINT('Ctrl Pts',(-0.196202823225698,0.00319955777911343,
0.00910714054051985));
#30725=CARTESIAN_POINT('Ctrl Pts',(-0.196194980787967,0.00325751941637139,
0.00913642031755311));
#30726=CARTESIAN_POINT('Ctrl Pts',(-0.196188035587219,0.00331059184700996,
0.00916252984284632));
#30727=CARTESIAN_POINT('Ctrl Pts',(-0.196181090386472,0.00336366427764853,
0.00918863936813953));
#30728=CARTESIAN_POINT('Ctrl Pts',(-0.196175039391781,0.00341177630756539,
0.00921172568002843));
#30729=CARTESIAN_POINT('Ctrl Pts',(-0.196169272892308,0.00345883730293629,
0.00923387466272813));
#30730=CARTESIAN_POINT('Ctrl Pts',(-0.19615773989336,0.00355295929367808,
0.00927817262812752));
#30731=CARTESIAN_POINT('Ctrl Pts',(-0.196147345195326,0.00364287649867495,
0.00931870835293598));
#30732=CARTESIAN_POINT('Ctrl Pts',(-0.196137643728015,0.00373661105067373,
0.00935920966817614));
#30733=CARTESIAN_POINT('Ctrl Pts',(-0.196119713132662,0.00390985456823773,
0.0094340656329037));
#30734=CARTESIAN_POINT('Ctrl Pts',(-0.196104161588853,0.00409635321035026,
0.0095083139085995));
#30735=CARTESIAN_POINT('Ctrl Pts',(-0.196092843570277,0.00428645811893465,
0.00957676005490717));
#30736=CARTESIAN_POINT('Ctrl Pts',(-0.196091914211108,0.00430206824880583,
0.00958238038970547));
#30737=CARTESIAN_POINT('Ctrl Pts',(-0.196091013396839,0.0043177021066952,
0.00958796292404868));
#30738=CARTESIAN_POINT('Ctrl Pts',(-0.196090142154209,0.00433335401676975,
0.009593505584366));
#30739=CARTESIAN_POINT('Ctrl Pts',(-0.19607866065389,0.00453961964745067,
0.00966654844754104));
#30740=CARTESIAN_POINT('Ctrl Pts',(-0.196072313469605,0.00474915014441373,
0.00973243826951178));
#30741=CARTESIAN_POINT('Ctrl Pts',(-0.196070177583228,0.00495016153240564,
0.00978859876622602));
#30742=CARTESIAN_POINT('Ctrl Pts',(-0.196068041696851,0.00515117292039755,
0.00984475926294027));
#30743=CARTESIAN_POINT('Ctrl Pts',(-0.196070099062835,0.00534341906999027,
0.00989201695645952));
#30744=CARTESIAN_POINT('Ctrl Pts',(-0.196075967808123,0.00555364142327267,
0.00993632357023678));
#30745=CARTESIAN_POINT('Ctrl Pts',(-0.196078902180768,0.00565875259991386,
0.0099584768771254));
#30746=CARTESIAN_POINT('Ctrl Pts',(-0.196082794197006,0.0057684019450636,
0.00997967664938378));
#30747=CARTESIAN_POINT('Ctrl Pts',(-0.196087472032619,0.00587685690239138,
0.00999867723685306));
#30748=CARTESIAN_POINT('Ctrl Pts',(-0.196088458447276,0.00589972678674669,
0.0100026838885434));
#30749=CARTESIAN_POINT('Ctrl Pts',(-0.196089479615871,0.0059225427625479,
0.0100065966003908));
#30750=CARTESIAN_POINT('Ctrl Pts',(-0.196090558152439,0.0059456909738631,
0.0100104788652639));
#30751=CARTESIAN_POINT('',(-0.197089662404178,0.00259797405121459,0.00878884347189939));
#30752=CARTESIAN_POINT('Ctrl Pts',(-0.196889861047832,0.00594388566779889,
0.0100280902017948));
#30753=CARTESIAN_POINT('Ctrl Pts',(-0.196888837648877,0.00592159442464991,
0.010024333805948));
#30754=CARTESIAN_POINT('Ctrl Pts',(-0.196883091265258,0.00579144662888638,
0.0100018530788455));
#30755=CARTESIAN_POINT('Ctrl Pts',(-0.196870803496027,0.00544040664358776,
0.00993381410319575));
#30756=CARTESIAN_POINT('Ctrl Pts',(-0.196865788922285,0.00495923422978679,
0.00981549844312244));
#30757=CARTESIAN_POINT('Ctrl Pts',(-0.196884784226902,0.00432929226751012,
0.00961778687411515));
#30758=CARTESIAN_POINT('Ctrl Pts',(-0.196925834282415,0.00382363098333961,
0.00941724253688526));
#30759=CARTESIAN_POINT('Ctrl Pts',(-0.196962104915578,0.00350801189151409,
0.009274415400131));
#30760=CARTESIAN_POINT('Ctrl Pts',(-0.196986213416204,0.00331553231284704,
0.00918208265328692));
#30761=CARTESIAN_POINT('Ctrl Pts',(-0.197009553267731,0.00314265469214262,
0.00909451705606134));
#30762=CARTESIAN_POINT('Ctrl Pts',(-0.19702187385383,0.0030556819289598,
0.00904871761708454));
#30763=CARTESIAN_POINT('Ctrl Pts',(-0.197047923761315,0.00287465209234715,
0.0089510947199911));
#30764=CARTESIAN_POINT('Ctrl Pts',(-0.197071447917473,0.00271719298855498,
0.00886092932785962));
#30765=CARTESIAN_POINT('Ctrl Pts',(-0.197089662404178,0.00259797405121459,
0.00878884347189939));
#30766=CARTESIAN_POINT('',(-0.198291526612024,0.00259925634552079,0.00881316468156375));
#30767=CARTESIAN_POINT('',(-0.197089662528356,0.00259797789988061,0.00878883713767665));
#30768=CARTESIAN_POINT('Ctrl Pts',(-0.198291526612024,0.00259925634552079,
0.00881316468156375));
#30769=CARTESIAN_POINT('Ctrl Pts',(-0.198273132696056,0.00271922866138589,
0.00888590375084709));
#30770=CARTESIAN_POINT('Ctrl Pts',(-0.198257339690863,0.00282455834668754,
0.00894625110008983));
#30771=CARTESIAN_POINT('Ctrl Pts',(-0.19824335373048,0.00291985877639059,
0.00899902457795324));
#30772=CARTESIAN_POINT('Ctrl Pts',(-0.198236360719517,0.00296750920091354,
0.0090254114329924));
#30773=CARTESIAN_POINT('Ctrl Pts',(-0.198229820492752,0.00301268208812486,
0.00904985350188748));
#30774=CARTESIAN_POINT('Ctrl Pts',(-0.198224523869574,0.00304951773520309,
0.00906950500261461));
#30775=CARTESIAN_POINT('Ctrl Pts',(-0.198219227246395,0.00308635338228131,
0.00908915650334175));
#30776=CARTESIAN_POINT('Ctrl Pts',(-0.198215171776289,0.00311478604942531,
0.00910413877179396));
#30777=CARTESIAN_POINT('Ctrl Pts',(-0.198209198476182,0.00315790597635664,
0.00912643125667087));
#30778=CARTESIAN_POINT('Ctrl Pts',(-0.198203225176075,0.00320102590328796,
0.00914872374154777));
#30779=CARTESIAN_POINT('Ctrl Pts',(-0.198195338468025,0.00325894642302733,
0.00917810925876707));
#30780=CARTESIAN_POINT('Ctrl Pts',(-0.198188353589727,0.00331198230778945,
0.00920431265300255));
#30781=CARTESIAN_POINT('Ctrl Pts',(-0.198181368711429,0.00336501819255157,
0.00923051604723802));
#30782=CARTESIAN_POINT('Ctrl Pts',(-0.198175282616766,0.00341309769589153,
0.00925368486756316));
#30783=CARTESIAN_POINT('Ctrl Pts',(-0.198169482305615,0.00346012706315391,
0.00927591255722074));
#30784=CARTESIAN_POINT('Ctrl Pts',(-0.198157881683312,0.00355418579767866,
0.00932036793653589));
#30785=CARTESIAN_POINT('Ctrl Pts',(-0.198147424513911,0.00364404326995715,
0.00936104592055934));
#30786=CARTESIAN_POINT('Ctrl Pts',(-0.198137660544414,0.00373772805993553,
0.00940169259078848));
#30787=CARTESIAN_POINT('Ctrl Pts',(-0.198119913759321,0.00390800755892871,
0.00947557112159327));
#30788=CARTESIAN_POINT('Ctrl Pts',(-0.198104467740312,0.0040911383889277,
0.00954887570378074));
#30789=CARTESIAN_POINT('Ctrl Pts',(-0.19809309874562,0.0042779199997942,
0.00961661122033504));
#30790=CARTESIAN_POINT('Ctrl Pts',(-0.198091957697867,0.00429666631318535,
0.00962340948711916));
#30791=CARTESIAN_POINT('Ctrl Pts',(-0.198090857718422,0.00431544857027613,
0.00963015350494398));
#30792=CARTESIAN_POINT('Ctrl Pts',(-0.198089800603058,0.00433425688018677,
0.00963683962793629));
#30793=CARTESIAN_POINT('Ctrl Pts',(-0.198078210765531,0.0045404645122726,
0.00971014390655727));
#30794=CARTESIAN_POINT('Ctrl Pts',(-0.198071771836712,0.00474993416743466,
0.00977626207010369));
#30795=CARTESIAN_POINT('Ctrl Pts',(-0.198069559753659,0.00495091769207219,
0.00983262144189136));
#30796=CARTESIAN_POINT('Ctrl Pts',(-0.198067347670605,0.00515190121670971,
0.00988898081367903));
#30797=CARTESIAN_POINT('Ctrl Pts',(-0.19806934434283,0.0053441509600576,
0.00993640952736992));
#30798=CARTESIAN_POINT('Ctrl Pts',(-0.19807515731124,0.0055543837248035,
0.00998087296857176));
#30799=CARTESIAN_POINT('Ctrl Pts',(-0.198078063795445,0.00565950010717645,
0.0100031046891727));
#30800=CARTESIAN_POINT('Ctrl Pts',(-0.198081929169107,0.0057691566710522,
0.010024378634757));
#30801=CARTESIAN_POINT('Ctrl Pts',(-0.198086583120904,0.00587762248490804,
0.0100434450536445));
#30802=CARTESIAN_POINT('Ctrl Pts',(-0.198087489992435,0.00589875819128381,
0.0100471603462046));
#30803=CARTESIAN_POINT('Ctrl Pts',(-0.198088426645042,0.00591984801275532,
0.0100507949964277));
#30804=CARTESIAN_POINT('Ctrl Pts',(-0.198089410867419,0.00594119659128827,
0.0100543996135915));
#30805=CARTESIAN_POINT('',(-0.199090540183301,0.00260012944092227,0.00882936615427334));
#30806=CARTESIAN_POINT('Ctrl Pts',(-0.198888606651639,0.00593939180859995,
0.0100720065732061));
#30807=CARTESIAN_POINT('Ctrl Pts',(-0.198887676387017,0.00591893933289523,
0.0100685351665996));
#30808=CARTESIAN_POINT('Ctrl Pts',(-0.198882044030561,0.00579055403993556,
0.0100462494530026));
#30809=CARTESIAN_POINT('Ctrl Pts',(-0.198869890751112,0.00544134676562644,
0.00997834423696948));
#30810=CARTESIAN_POINT('Ctrl Pts',(-0.198865041548557,0.00495992103640058,
0.00985954411932006));
#30811=CARTESIAN_POINT('Ctrl Pts',(-0.19888434673602,0.0043304455028863,
0.00966125441771457));
#30812=CARTESIAN_POINT('Ctrl Pts',(-0.198925750261522,0.00382474303179102,
0.00945991595216248));
#30813=CARTESIAN_POINT('Ctrl Pts',(-0.198962251165325,0.00350936192060643,
0.00931660579371268));
#30814=CARTESIAN_POINT('Ctrl Pts',(-0.198986506970023,0.00331701212666396,
0.00922394949251914));
#30815=CARTESIAN_POINT('Ctrl Pts',(-0.199009982866199,0.00314426989599801,
0.00913607982520711));
#30816=CARTESIAN_POINT('Ctrl Pts',(-0.19902237458798,0.00305736235190651,
0.009090117421809));
#30817=CARTESIAN_POINT('Ctrl Pts',(-0.19904857160634,0.00287649479718902,
0.00899215805150388));
#30818=CARTESIAN_POINT('Ctrl Pts',(-0.19907222585195,0.00271920306422584,
0.00890168902253671));
#30819=CARTESIAN_POINT('Ctrl Pts',(-0.199090540183301,0.00260012944092227,
0.00882936615427334));
#30820=CARTESIAN_POINT('',(-0.200292328770423,0.00260137281375138,0.00885372168982735));
#30821=CARTESIAN_POINT('',(-0.199090540305781,0.00260013324515697,0.00882935992144404));
#30822=CARTESIAN_POINT('Ctrl Pts',(-0.200292328770423,0.00260137281375138,
0.00885372168982735));
#30823=CARTESIAN_POINT('Ctrl Pts',(-0.200273837896757,0.00272121175790609,
0.00892670462618666));
#30824=CARTESIAN_POINT('Ctrl Pts',(-0.200257961423412,0.00282643766557617,
0.00898725675305832));
#30825=CARTESIAN_POINT('Ctrl Pts',(-0.200243900974506,0.00292165061038557,
0.00904021017006671));
#30826=CARTESIAN_POINT('Ctrl Pts',(-0.200236870718853,0.00296925729406923,
0.00906668699607533));
#30827=CARTESIAN_POINT('Ctrl Pts',(-0.200230295497294,0.00301439072573244,
0.00909121268824908));
#30828=CARTESIAN_POINT('Ctrl Pts',(-0.200224970624474,0.00305119417903304,
0.00911093102925758));
#30829=CARTESIAN_POINT('Ctrl Pts',(-0.200219645751654,0.00308799763233363,
0.00913064937026609));
#30830=CARTESIAN_POINT('Ctrl Pts',(-0.200215568764996,0.0031164048833556,
0.00914568206453222));
#30831=CARTESIAN_POINT('Ctrl Pts',(-0.20020956272179,0.00315949117040272,
0.00916805152229006));
#30832=CARTESIAN_POINT('Ctrl Pts',(-0.200203556678583,0.00320257745744984,
0.00919042098004789));
#30833=CARTESIAN_POINT('Ctrl Pts',(-0.200195626022548,0.00326045695423104,
0.00921990933366753));
#30834=CARTESIAN_POINT('Ctrl Pts',(-0.200188601532831,0.00331345701852395,
0.00924620432155298));
#30835=CARTESIAN_POINT('Ctrl Pts',(-0.200181577043113,0.00336645708281686,
0.00927249930943843));
#30836=CARTESIAN_POINT('Ctrl Pts',(-0.200175455659094,0.00341450543872106,
0.00929574895779386));
#30837=CARTESIAN_POINT('Ctrl Pts',(-0.200169621352145,0.00346150318350308,
0.00931805309801738));
#30838=CARTESIAN_POINT('Ctrl Pts',(-0.200157952738249,0.00355549867306711,
0.00936266137846443));
#30839=CARTESIAN_POINT('Ctrl Pts',(-0.20014743274518,0.00364529078631978,
0.00940347505836594));
#30840=CARTESIAN_POINT('Ctrl Pts',(-0.200137604015595,0.00373893481032285,
0.00944426681906609));
#30841=CARTESIAN_POINT('Ctrl Pts',(-0.200120047004139,0.00390621067117079,
0.00951713294116265));
#30842=CARTESIAN_POINT('Ctrl Pts',(-0.200104706208719,0.00408597836688247,
0.00958947556607649));
#30843=CARTESIAN_POINT('Ctrl Pts',(-0.200093286933946,0.00426938216658885,
0.00965646105117785));
#30844=CARTESIAN_POINT('Ctrl Pts',(-0.200091920779482,0.00429132383316669,
0.00966447491556889));
#30845=CARTESIAN_POINT('Ctrl Pts',(-0.200090610752696,0.00431331641716091,
0.00967241458652526));
#30846=CARTESIAN_POINT('Ctrl Pts',(-0.200089359773607,0.00433534378299784,
0.00968027408652165));
#30847=CARTESIAN_POINT('Ctrl Pts',(-0.200077652236101,0.00454149128290405,
0.00975382878601519));
#30848=CARTESIAN_POINT('Ctrl Pts',(-0.200071114735433,0.00475081464251925,
0.00982013994437917));
#30849=CARTESIAN_POINT('Ctrl Pts',(-0.20006882183701,0.00495177345483577,
0.0098766928364664));
#30850=CARTESIAN_POINT('Ctrl Pts',(-0.200066528938587,0.00515273226715229,
0.00993324572855362));
#30851=CARTESIAN_POINT('Ctrl Pts',(-0.20006846267712,0.00534507943381997,
0.00998086237617104));
#30852=CARTESIAN_POINT('Ctrl Pts',(-0.200074226063807,0.00555533499112588,
0.0100254775673568));
#30853=CARTESIAN_POINT('Ctrl Pts',(-0.20007710775715,0.00566046276977883,
0.0100477851629496));
#30854=CARTESIAN_POINT('Ctrl Pts',(-0.200080951668549,0.0057701121703622,
0.0100691264095741));
#30855=CARTESIAN_POINT('Ctrl Pts',(-0.200085588250657,0.00587857122173911,
0.0100882522879767));
#30856=CARTESIAN_POINT('Ctrl Pts',(-0.200086414932592,0.00589790898743928,
0.0100916623468944));
#30857=CARTESIAN_POINT('Ctrl Pts',(-0.200087266677091,0.00591720835943309,
0.0100950045482874));
#30858=CARTESIAN_POINT('Ctrl Pts',(-0.200088157086456,0.00593670244816755,
0.0100983180218859));
#30859=CARTESIAN_POINT('',(-0.201091331877826,0.00260231956762303,0.0088700075790552));
#30860=CARTESIAN_POINT('Ctrl Pts',(-0.200887345683122,0.0059348980442802,
0.0101159223609127));
#30861=CARTESIAN_POINT('Ctrl Pts',(-0.200886506663953,0.00591628097381425,
0.0101127400212251));
#30862=CARTESIAN_POINT('Ctrl Pts',(-0.200880986324111,0.0057896653627417,
0.010090654716993));
#30863=CARTESIAN_POINT('Ctrl Pts',(-0.200868962037106,0.005442297041805,
0.0100228912331785));
#30864=CARTESIAN_POINT('Ctrl Pts',(-0.20086426816572,0.00496065222418959,
0.00990362400826062));
#30865=CARTESIAN_POINT('Ctrl Pts',(-0.200883867541184,0.00433161563399345,
0.00970476368487069));
#30866=CARTESIAN_POINT('Ctrl Pts',(-0.200925609896317,0.00382589679812178,
0.00950265618711336));
#30867=CARTESIAN_POINT('Ctrl Pts',(-0.200962333382757,0.00351075052547446,
0.00935887421941144));
#30868=CARTESIAN_POINT('Ctrl Pts',(-0.200986731782129,0.00331853051675235,
0.00926590227797969));
#30869=CARTESIAN_POINT('Ctrl Pts',(-0.201010339542551,0.00314592329813722,
0.00917773598410989));
#30870=CARTESIAN_POINT('Ctrl Pts',(-0.201022800394077,0.00305908023167697,
0.00913161420213365));
#30871=CARTESIAN_POINT('Ctrl Pts',(-0.201049140182371,0.00287837410448303,
0.0090333264982479));
#30872=CARTESIAN_POINT('Ctrl Pts',(-0.201072920671161,0.00272124883301824,
0.00894256141583152));
#30873=CARTESIAN_POINT('Ctrl Pts',(-0.201091331877826,0.00260231956762303,
0.0088700075790552));
#30874=CARTESIAN_POINT('',(-0.202293065733516,0.00260357610533656,0.00889442911865277));
#30875=CARTESIAN_POINT('',(-0.201091331999189,0.00260232334500957,0.00887000141752919));
#30876=CARTESIAN_POINT('Ctrl Pts',(-0.202293065733516,0.00260357610533656,
0.00889442911865277));
#30877=CARTESIAN_POINT('Ctrl Pts',(-0.202274475468373,0.00272326920892133,
0.00896764049982792));
#30878=CARTESIAN_POINT('Ctrl Pts',(-0.202258513370394,0.00282838010195822,
0.00902838492069327));
#30879=CARTESIAN_POINT('Ctrl Pts',(-0.202244376443369,0.00292349537576616,
0.00908150758113047));
#30880=CARTESIAN_POINT('Ctrl Pts',(-0.202237307948081,0.00297105322646132,
0.00910806903075321));
#30881=CARTESIAN_POINT('Ctrl Pts',(-0.202230696778204,0.00301614236175929,
0.00913267346161789));
#30882=CARTESIAN_POINT('Ctrl Pts',(-0.202225342855067,0.00305290982182173,
0.00915245482498696));
#30883=CARTESIAN_POINT('Ctrl Pts',(-0.20221998893193,0.00308967728188417,
0.00917223618835603));
#30884=CARTESIAN_POINT('Ctrl Pts',(-0.202215889781666,0.00311805638280766,
0.00918731651992855));
#30885=CARTESIAN_POINT('Ctrl Pts',(-0.202209850054849,0.00316110438387033,
0.00920975861098695));
#30886=CARTESIAN_POINT('Ctrl Pts',(-0.202203810328033,0.00320415238493301,
0.00923220070204534));
#30887=CARTESIAN_POINT('Ctrl Pts',(-0.202195834488617,0.00326198425819688,
0.00926178607004551));
#30888=CARTESIAN_POINT('Ctrl Pts',(-0.202188769218574,0.00331494264804402,
0.00928816764310139));
#30889=CARTESIAN_POINT('Ctrl Pts',(-0.202181703948532,0.00336790103789116,
0.00931454921615728));
#30890=CARTESIAN_POINT('Ctrl Pts',(-0.202175546173851,0.00341591316921346,
0.00933787544456852));
#30891=CARTESIAN_POINT('Ctrl Pts',(-0.202169676846241,0.0034628734948644,
0.00936025161595196));
#30892=CARTESIAN_POINT('Ctrl Pts',(-0.202157938191021,0.00355679414616629,
0.00940500395871885));
#30893=CARTESIAN_POINT('Ctrl Pts',(-0.202147353627051,0.00364650633906559,
0.00944594396933934));
#30894=CARTESIAN_POINT('Ctrl Pts',(-0.202137457493401,0.00374010383894624,
0.00948687578309684));
#30895=CARTESIAN_POINT('Ctrl Pts',(-0.202120088590578,0.0039043786898437,
0.00955871603107942));
#30896=CARTESIAN_POINT('Ctrl Pts',(-0.202104850677498,0.00408081733665042,
0.00963009264144663));
#30897=CARTESIAN_POINT('Ctrl Pts',(-0.202093384451066,0.0042608447204149,
0.00969630907557451));
#30898=CARTESIAN_POINT('Ctrl Pts',(-0.202091784646742,0.00428596271268767,
0.0097055478027391));
#30899=CARTESIAN_POINT('Ctrl Pts',(-0.202090258264773,0.00431114910199664,
0.00971468928320473));
#30900=CARTESIAN_POINT('Ctrl Pts',(-0.202088809761387,0.00433637909078407,
0.00972372430600667));
#30901=CARTESIAN_POINT('Ctrl Pts',(-0.202076979445947,0.00454243917237846,
0.00979751575916425));
#30902=CARTESIAN_POINT('Ctrl Pts',(-0.20207034194049,0.00475153493044841,
0.00986399247318988));
#30903=CARTESIAN_POINT('Ctrl Pts',(-0.202067969551709,0.00495244619644365,
0.00992073315628037));
#30904=CARTESIAN_POINT('Ctrl Pts',(-0.202065597162928,0.00515335746243889,
0.00997747383937085));
#30905=CARTESIAN_POINT('Ctrl Pts',(-0.202067472167892,0.00534583912516003,
0.0100252890958902));
#30906=CARTESIAN_POINT('Ctrl Pts',(-0.202073197894455,0.005556098712338,
0.0100700539580997));
#30907=CARTESIAN_POINT('Ctrl Pts',(-0.202076060757737,0.00566122850592697,
0.0100924363892045));
#30908=CARTESIAN_POINT('Ctrl Pts',(-0.202079891079458,0.00577084725715454,
0.0101138415381843));
#30909=CARTESIAN_POINT('Ctrl Pts',(-0.202084519326978,0.00587927387560881,
0.0101330242882825));
#30910=CARTESIAN_POINT('Ctrl Pts',(-0.202085271363521,0.0058968919435591,
0.010136141262689));
#30911=CARTESIAN_POINT('Ctrl Pts',(-0.202086044354192,0.0059144780827782,
0.0101392016200004));
#30912=CARTESIAN_POINT('Ctrl Pts',(-0.202086848594906,0.00593220842806255,
0.0101422352280257));
#30913=CARTESIAN_POINT('',(-0.203091791305043,0.00260433418259679,0.00891063271010805));
#30914=CARTESIAN_POINT('Ctrl Pts',(-0.202885099445385,0.00593040690138148,
0.0101598141695237));
#30915=CARTESIAN_POINT('Ctrl Pts',(-0.202884354971372,0.00591368430258583,
0.0101569360655661));
#30916=CARTESIAN_POINT('Ctrl Pts',(-0.202878992896662,0.00578947217370395,
0.0101351728763029));
#30917=CARTESIAN_POINT('Ctrl Pts',(-0.202867259104593,0.0054454906008289,
0.0100679541944753));
#30918=CARTESIAN_POINT('Ctrl Pts',(-0.202863123060488,0.004959530471194,
0.00994714447823416));
#30919=CARTESIAN_POINT('Ctrl Pts',(-0.202883406117703,0.00433659227554887,
0.00974971310348173));
#30920=CARTESIAN_POINT('Ctrl Pts',(-0.202926463640028,0.00382383543467921,
0.00954412528623439));
#30921=CARTESIAN_POINT('Ctrl Pts',(-0.202963209822097,0.003510675044003,
0.00940051603960522));
#30922=CARTESIAN_POINT('Ctrl Pts',(-0.202987598667131,0.00331891162837778,
0.00930736298217058));
#30923=CARTESIAN_POINT('Ctrl Pts',(-0.203011094368678,0.0031470861154104,
0.00921921390736344));
#30924=CARTESIAN_POINT('Ctrl Pts',(-0.203023587987513,0.00305986178150982,
0.00917269162038482));
#30925=CARTESIAN_POINT('Ctrl Pts',(-0.203049839751636,0.00287944809228144,
0.00907412081376304));
#30926=CARTESIAN_POINT('Ctrl Pts',(-0.2030734973985,0.00272278133299953,
0.00898321135849634));
#30927=CARTESIAN_POINT('Ctrl Pts',(-0.203091791305043,0.00260433418259679,
0.00891063271010805));
#30928=CARTESIAN_POINT('',(-0.204293510165871,0.00260574519043331,0.00893520746292813));
#30929=CARTESIAN_POINT('',(-0.203091791426825,0.00260433798081893,0.00891062654167635));
#30930=CARTESIAN_POINT('Ctrl Pts',(-0.204293510165871,0.00260574519043331,
0.00893520746292813));
#30931=CARTESIAN_POINT('Ctrl Pts',(-0.204275076567995,0.00272501382324815,
0.00900847502531422));
#30932=CARTESIAN_POINT('Ctrl Pts',(-0.204259227819518,0.00282988504055417,
0.0090693498218917));
#30933=CARTESIAN_POINT('Ctrl Pts',(-0.20424517062167,0.00292489404478681,
0.00912264277868882));
#30934=CARTESIAN_POINT('Ctrl Pts',(-0.20423814199043,0.00297239876531212,
0.00914928937959851));
#30935=CARTESIAN_POINT('Ctrl Pts',(-0.204231562274048,0.00301746803417767,
0.00917398932116904));
#30936=CARTESIAN_POINT('Ctrl Pts',(-0.204226221712992,0.00305430402977027,
0.00919389171338426));
#30937=CARTESIAN_POINT('Ctrl Pts',(-0.204220881151935,0.00309114002536287,
0.00921379410559949));
#30938=CARTESIAN_POINT('Ctrl Pts',(-0.204216777274443,0.00311967596045992,
0.00922902065933212));
#30939=CARTESIAN_POINT('Ctrl Pts',(-0.204210753464681,0.00316274908232262,
0.00925156788917228));
#30940=CARTESIAN_POINT('Ctrl Pts',(-0.20420472965492,0.00320582220418532,
0.00927411511901243));
#30941=CARTESIAN_POINT('Ctrl Pts',(-0.204196790365541,0.00326354743608214,
0.00930376547534614));
#30942=CARTESIAN_POINT('Ctrl Pts',(-0.204189744354715,0.00331644916448935,
0.00933022524743304));
#30943=CARTESIAN_POINT('Ctrl Pts',(-0.204182698343888,0.00336935089289657,
0.00935668501951994));
#30944=CARTESIAN_POINT('Ctrl Pts',(-0.204176542556964,0.00341735669267945,
0.00938010148299971));
#30945=CARTESIAN_POINT('Ctrl Pts',(-0.20417067241306,0.00346426236205979,
0.00940254036039787));
#30946=CARTESIAN_POINT('Ctrl Pts',(-0.204158932125252,0.0035580737008205,
0.00944741811519419));
#30947=CARTESIAN_POINT('Ctrl Pts',(-0.204148334510898,0.00364747781089567,
0.00948838331382297));
#30948=CARTESIAN_POINT('Ctrl Pts',(-0.20413834003469,0.00374131254045276,
0.00952957637488636));
#30949=CARTESIAN_POINT('Ctrl Pts',(-0.204121212928019,0.00390211310558426,
0.00960016716285746));
#30950=CARTESIAN_POINT('Ctrl Pts',(-0.20410586914575,0.00407615059995422,
0.00967093159324034));
#30951=CARTESIAN_POINT('Ctrl Pts',(-0.204094147762405,0.00425230443228834,
0.00973617036461655));
#30952=CARTESIAN_POINT('Ctrl Pts',(-0.204092189183428,0.00428173877315499,
0.00974707140610378));
#30953=CARTESIAN_POINT('Ctrl Pts',(-0.20409033174393,0.00431122959651332,
0.0097578240646924));
#30954=CARTESIAN_POINT('Ctrl Pts',(-0.204088584023885,0.00434072179096112,
0.0097684095940632));
#30955=CARTESIAN_POINT('Ctrl Pts',(-0.204076376834576,0.00454671405039965,
0.0098423456694646));
#30956=CARTESIAN_POINT('Ctrl Pts',(-0.204069514965021,0.00475286180502225,
0.0099080404173306));
#30957=CARTESIAN_POINT('Ctrl Pts',(-0.204066816106438,0.00495305084389507,
0.00996477003023813));
#30958=CARTESIAN_POINT('Ctrl Pts',(-0.204064117247854,0.0051532398827679,
0.0100214996431457));
#30959=CARTESIAN_POINT('Ctrl Pts',(-0.204065567196888,0.005347245104113,
0.01006991838009));
#30960=CARTESIAN_POINT('Ctrl Pts',(-0.204071292044941,0.00555973157676272,
0.0101152347804172));
#30961=CARTESIAN_POINT('Ctrl Pts',(-0.204074496107032,0.00567865523126791,
0.0101405972981752));
#30962=CARTESIAN_POINT('Ctrl Pts',(-0.204079049119957,0.00580343197303493,
0.0101647293003646));
#30963=CARTESIAN_POINT('Ctrl Pts',(-0.204084593180221,0.00592771653709633,
0.0101861316274437));
#30964=CARTESIAN_POINT('',(-0.205092331912265,0.00260645114791581,0.00895141913306061));
#30965=CARTESIAN_POINT('Ctrl Pts',(-0.204883316991064,0.00592592657070326,
0.0102036471645642));
#30966=CARTESIAN_POINT('Ctrl Pts',(-0.204882671137622,0.00591144529308884,
0.0102011599238186));
#30967=CARTESIAN_POINT('Ctrl Pts',(-0.20487717178741,0.00578506672453634,
0.0101791477099926));
#30968=CARTESIAN_POINT('Ctrl Pts',(-0.204866209701125,0.00545213555483161,
0.0101133657534363));
#30969=CARTESIAN_POINT('Ctrl Pts',(-0.204861852683361,0.00496215483740597,
0.00999260159629974));
#30970=CARTESIAN_POINT('Ctrl Pts',(-0.204880095936079,0.00442886261065933,
0.00982107008356725));
#30971=CARTESIAN_POINT('Ctrl Pts',(-0.204907085968845,0.00405046827475919,
0.00967788144453791));
#30972=CARTESIAN_POINT('Ctrl Pts',(-0.204937958692689,0.00372990950313333,
0.00954347459787447));
#30973=CARTESIAN_POINT('Ctrl Pts',(-0.204963618489919,0.00351270551424823,
0.00944317167265714));
#30974=CARTESIAN_POINT('Ctrl Pts',(-0.20498815842505,0.00332022837241253,
0.00934936436806583));
#30975=CARTESIAN_POINT('Ctrl Pts',(-0.205011645825832,0.00314877731821974,
0.00926103688660394));
#30976=CARTESIAN_POINT('Ctrl Pts',(-0.205024182885467,0.00306131323278087,
0.00921420176338373));
#30977=CARTESIAN_POINT('Ctrl Pts',(-0.205050437575135,0.00288103174617778,
0.00911528740541476));
#30978=CARTESIAN_POINT('Ctrl Pts',(-0.205074070416774,0.00272461878566508,
0.00902413649647073));
#30979=CARTESIAN_POINT('Ctrl Pts',(-0.205092331912265,0.00260645114791581,
0.00895141913306061));
#30980=CARTESIAN_POINT('',(-0.206293999435804,0.00260759218872069,0.00897588362098812));
#30981=CARTESIAN_POINT('',(-0.20509233202994,0.00260645482550656,0.0089514131859722));
#30982=CARTESIAN_POINT('Ctrl Pts',(-0.206293999435804,0.00260759218872069,
0.00897588362098812));
#30983=CARTESIAN_POINT('Ctrl Pts',(-0.206275606236776,0.00272657234509535,
0.00904928873984808));
#30984=CARTESIAN_POINT('Ctrl Pts',(-0.206251865963918,0.00288355267308425,
0.00914095396549715));
#30985=CARTESIAN_POINT('Ctrl Pts',(-0.206225558203887,0.00306373816500964,
0.00924000226939381));
#30986=CARTESIAN_POINT('Ctrl Pts',(-0.206213206763392,0.00314955254584123,
0.00928606722127801));
#30987=CARTESIAN_POINT('Ctrl Pts',(-0.206189409028581,0.0033223041095643,
0.00937526677216162));
#30988=CARTESIAN_POINT('Ctrl Pts',(-0.206164656195616,0.00351506923364879,
0.00946938213392435));
#30989=CARTESIAN_POINT('Ctrl Pts',(-0.206138728171142,0.00373241945612685,
0.00956991384257538));
#30990=CARTESIAN_POINT('Ctrl Pts',(-0.206107559899463,0.00405172320144206,
0.00970403637599294));
#30991=CARTESIAN_POINT('Ctrl Pts',(-0.206079921416922,0.00443029769141955,
0.00984754120837745));
#30992=CARTESIAN_POINT('Ctrl Pts',(-0.206061315628273,0.00496107403636117,
0.010018644986773));
#30993=CARTESIAN_POINT('Ctrl Pts',(-0.206065539578611,0.00545325447955815,
0.0101402646231475));
#30994=CARTESIAN_POINT('Ctrl Pts',(-0.206076538113247,0.00578510480717584,
0.0102059130522982));
#30995=CARTESIAN_POINT('Ctrl Pts',(-0.20608201684332,0.00591016240860172,
0.0102277486059419));
#30996=CARTESIAN_POINT('Ctrl Pts',(-0.206082602390132,0.00592322960732983,
0.0102300014544386));
#30997=CARTESIAN_POINT('',(-0.207092852170764,0.00260851097558208,0.00899226563559695));
#30998=CARTESIAN_POINT('Ctrl Pts',(-0.206881571004172,0.00592143254235674,
0.0102475607510614));
#30999=CARTESIAN_POINT('Ctrl Pts',(-0.206881020496666,0.00590893384282267,
0.0102453998143091));
#31000=CARTESIAN_POINT('Ctrl Pts',(-0.206875680990742,0.00578499503296741,
0.0102237098597449));
#31001=CARTESIAN_POINT('Ctrl Pts',(-0.206864923140502,0.00545427255237323,
0.0101582379308979));
#31002=CARTESIAN_POINT('Ctrl Pts',(-0.206860949893193,0.0049619143385102,
0.010036492327419));
#31003=CARTESIAN_POINT('Ctrl Pts',(-0.206879692666681,0.00442978956942307,
0.00986470087572262));
#31004=CARTESIAN_POINT('Ctrl Pts',(-0.206907292633342,0.00405093552770489,
0.00972082871068698));
#31005=CARTESIAN_POINT('Ctrl Pts',(-0.206938369196101,0.00373106068533,
0.00958619552651098));
#31006=CARTESIAN_POINT('Ctrl Pts',(-0.206964134873792,0.00351390912494474,
0.00948554071057212));
#31007=CARTESIAN_POINT('Ctrl Pts',(-0.206988721782151,0.00332157558445463,
0.00939143426474644));
#31008=CARTESIAN_POINT('Ctrl Pts',(-0.207012209264182,0.0031503451607018,
0.00930287133695935));
#31009=CARTESIAN_POINT('Ctrl Pts',(-0.207024781376472,0.00306268383339939,
0.0092557414932042));
#31010=CARTESIAN_POINT('Ctrl Pts',(-0.207051031204484,0.00288252984294508,
0.00915648754524844));
#31011=CARTESIAN_POINT('Ctrl Pts',(-0.207074629977899,0.00272638846036655,
0.00906510989893176));
#31012=CARTESIAN_POINT('Ctrl Pts',(-0.207092852170764,0.00260851097558208,
0.00899226563559695));
#31013=CARTESIAN_POINT('',(-0.208294495555528,0.002609557221425,0.00901672737671743));
#31014=CARTESIAN_POINT('',(-0.207092852286225,0.00260851459105031,0.00899225981344203));
#31015=CARTESIAN_POINT('Ctrl Pts',(-0.208294495555528,0.002609557221425,
0.00901672737671743));
#31016=CARTESIAN_POINT('Ctrl Pts',(-0.208276153739984,0.00272818271907759,
0.00909022007273419));
#31017=CARTESIAN_POINT('Ctrl Pts',(-0.208252462664079,0.00288480997457173,
0.00918206687811871));
#31018=CARTESIAN_POINT('Ctrl Pts',(-0.208226174631601,0.0030647907813057,
0.00928141626672825));
#31019=CARTESIAN_POINT('Ctrl Pts',(-0.208213795276203,0.00315076692511177,
0.00932775588295479));
#31020=CARTESIAN_POINT('Ctrl Pts',(-0.208190006020789,0.00332326101084848,
0.00941718226047124));
#31021=CARTESIAN_POINT('Ctrl Pts',(-0.208165206295545,0.00351592866849304,
0.00951162039509459));
#31022=CARTESIAN_POINT('Ctrl Pts',(-0.208139241772671,0.00373263243560695,
0.00961227396471289));
#31023=CARTESIAN_POINT('Ctrl Pts',(-0.20810762277873,0.00405359805798186,
0.00974757364736688));
#31024=CARTESIAN_POINT('Ctrl Pts',(-0.208079658202872,0.00442984491645365,
0.00989065971484939));
#31025=CARTESIAN_POINT('Ctrl Pts',(-0.2080603918466,0.00496098587762989,
0.0100626318644918));
#31026=CARTESIAN_POINT('Ctrl Pts',(-0.208064266452075,0.00545499835628659,
0.0101850488681411));
#31027=CARTESIAN_POINT('Ctrl Pts',(-0.208075055741243,0.00578480551874336,
0.0102504392329819));
#31028=CARTESIAN_POINT('Ctrl Pts',(-0.208080378153632,0.00590756155050767,
0.0102719761801877));
#31029=CARTESIAN_POINT('Ctrl Pts',(-0.208080872472194,0.00591873554374485,
0.0102739153516223));
#31030=CARTESIAN_POINT('',(-0.2090933136672,0.00261035295544765,0.00903306981791057));
#31031=CARTESIAN_POINT('Ctrl Pts',(-0.208879854976475,0.00591693841052602,
0.0102914751265115));
#31032=CARTESIAN_POINT('Ctrl Pts',(-0.208879403882135,0.00590656011569423,
0.0102896689662938));
#31033=CARTESIAN_POINT('Ctrl Pts',(-0.208874225719035,0.00578512936524486,
0.0102683205164887));
#31034=CARTESIAN_POINT('Ctrl Pts',(-0.208863665925877,0.00545665484873855,
0.0102031715204708));
#31035=CARTESIAN_POINT('Ctrl Pts',(-0.208860006423808,0.0049627509677495,
0.0100807435638028));
#31036=CARTESIAN_POINT('Ctrl Pts',(-0.208879357400325,0.00443027031107117,
0.00990816157715126));
#31037=CARTESIAN_POINT('Ctrl Pts',(-0.20890726143644,0.00405355877387217,
0.00976467967278848));
#31038=CARTESIAN_POINT('Ctrl Pts',(-0.208938745865106,0.00373216391169831,
0.00962896700904035));
#31039=CARTESIAN_POINT('Ctrl Pts',(-0.208964558210369,0.00351545759703801,
0.00952812730521938));
#31040=CARTESIAN_POINT('Ctrl Pts',(-0.20898919858518,0.00332310641781344,
0.00943366189332718));
#31041=CARTESIAN_POINT('Ctrl Pts',(-0.209012687715841,0.00315201860638895,
0.00934483181569398));
#31042=CARTESIAN_POINT('Ctrl Pts',(-0.209025296557779,0.00306411948254137,
0.00929738914424859));
#31043=CARTESIAN_POINT('Ctrl Pts',(-0.20905154854399,0.00288399129561906,
0.00919774726681492));
#31044=CARTESIAN_POINT('Ctrl Pts',(-0.209075122591561,0.00272802036343885,
0.00910608875383453));
#31045=CARTESIAN_POINT('Ctrl Pts',(-0.2090933136672,0.00261035295544765,
0.00903306981791057));
#31046=CARTESIAN_POINT('',(-0.210295195412647,0.00261161233680568,0.00905772513090701));
#31047=CARTESIAN_POINT('',(-0.209093313783645,0.00261035660874823,0.00903306395929884));
#31048=CARTESIAN_POINT('Ctrl Pts',(-0.210295195412647,0.00261161233680569,
0.00905772513090701));
#31049=CARTESIAN_POINT('Ctrl Pts',(-0.210276894963234,0.00272994295497824,
0.00913133389119312));
#31050=CARTESIAN_POINT('Ctrl Pts',(-0.210253240828118,0.00288629398964245,
0.00922339455195382));
#31051=CARTESIAN_POINT('Ctrl Pts',(-0.210226962421796,0.00306614095590343,
0.00932306899945819));
#31052=CARTESIAN_POINT('Ctrl Pts',(-0.210214549298879,0.00315232223911781,
0.00936969988198298));
#31053=CARTESIAN_POINT('Ctrl Pts',(-0.210190769979594,0.00332456621842443,
0.00945934060833127));
#31054=CARTESIAN_POINT('Ctrl Pts',(-0.210165926230228,0.00351714624291661,
0.00955409089556758));
#31055=CARTESIAN_POINT('Ctrl Pts',(-0.21013992137214,0.00373332555747361,
0.00965489747215478));
#31056=CARTESIAN_POINT('Ctrl Pts',(-0.210107902642912,0.0040555984786723,
0.00979120813717689));
#31057=CARTESIAN_POINT('Ctrl Pts',(-0.210079607338285,0.00442978955791621,
0.00993395826629711));
#31058=CARTESIAN_POINT('Ctrl Pts',(-0.210059670420687,0.00496117514435055,
0.0101067070575915));
#31059=CARTESIAN_POINT('Ctrl Pts',(-0.210063175312016,0.00545645643098748,
0.0102297840556843));
#31060=CARTESIAN_POINT('Ctrl Pts',(-0.210073732641992,0.00578430958237604,
0.010294942762644));
#31061=CARTESIAN_POINT('Ctrl Pts',(-0.210078893244153,0.00590490128356823,
0.010316200616972));
#31062=CARTESIAN_POINT('Ctrl Pts',(-0.21007929998055,0.00591424122749678,
0.0103178320466886));
#31063=CARTESIAN_POINT('',(-0.21109423145639,0.00261222360480081,0.00907399364715958));
#31064=CARTESIAN_POINT('Ctrl Pts',(-0.210878462469796,0.00591244389125894,
0.0103353945802353));
#31065=CARTESIAN_POINT('Ctrl Pts',(-0.210878081781242,0.00590353255855026,
0.0103338336933755));
#31066=CARTESIAN_POINT('Ctrl Pts',(-0.210873054175543,0.00578382770812169,
0.010312682318795));
#31067=CARTESIAN_POINT('Ctrl Pts',(-0.21086273938801,0.00545688672168629,
0.0102476370857249));
#31068=CARTESIAN_POINT('Ctrl Pts',(-0.21085947521624,0.00496214926258382,
0.0101245977556503));
#31069=CARTESIAN_POINT('Ctrl Pts',(-0.21087951803606,0.00442942772142485,
0.00995120290508484));
#31070=CARTESIAN_POINT('Ctrl Pts',(-0.210907778127693,0.00405467894669112,
0.00980797983942088));
#31071=CARTESIAN_POINT('Ctrl Pts',(-0.210939660748439,0.00373214570960748,
0.00967129247182057));
#31072=CARTESIAN_POINT('Ctrl Pts',(-0.210965515951445,0.00351605213693032,
0.00957032405479985));
#31073=CARTESIAN_POINT('Ctrl Pts',(-0.210990200367711,0.00332387153922504,
0.00947557360729596));
#31074=CARTESIAN_POINT('Ctrl Pts',(-0.21101367907488,0.00315310641654562,
0.0093865593121067));
#31075=CARTESIAN_POINT('Ctrl Pts',(-0.211026321387228,0.00306503577488379,
0.00933883439822843));
#31076=CARTESIAN_POINT('Ctrl Pts',(-0.21105255883218,0.00288513131503311,
0.00923890762798111));
#31077=CARTESIAN_POINT('Ctrl Pts',(-0.211076088510623,0.00272952577556201,
0.00914708390503086));
#31078=CARTESIAN_POINT('Ctrl Pts',(-0.21109423145639,0.00261222360480081,
0.00907399364715958));
#31079=CARTESIAN_POINT('',(-0.212296004165384,0.00261384219706213,0.0090989278724998));
#31080=CARTESIAN_POINT('',(-0.211094231575152,0.00261222733769334,0.00907398768525308));
#31081=CARTESIAN_POINT('Ctrl Pts',(-0.212296004165384,0.00261384219706213,
0.0090989278724998));
#31082=CARTESIAN_POINT('Ctrl Pts',(-0.212277735923486,0.00273194228337272,
0.00917268275309667));
#31083=CARTESIAN_POINT('Ctrl Pts',(-0.212261985492411,0.00283608798183092,
0.00923414686528063));
#31084=CARTESIAN_POINT('Ctrl Pts',(-0.212247974568846,0.00293067459298826,
0.00928807357720397));
#31085=CARTESIAN_POINT('Ctrl Pts',(-0.212240969072873,0.00297796812938874,
0.00931503706476419));
#31086=CARTESIAN_POINT('Ctrl Pts',(-0.212234399475194,0.00302290207516733,
0.00934006570537844));
#31087=CARTESIAN_POINT('Ctrl Pts',(-0.212229041039002,0.00305981228032552,
0.00936033052343684));
#31088=CARTESIAN_POINT('Ctrl Pts',(-0.212223682602811,0.00309672248548371,
0.00938059534149524));
#31089=CARTESIAN_POINT('Ctrl Pts',(-0.212219532847886,0.00312554135293767,
0.00939621760162779));
#31090=CARTESIAN_POINT('Ctrl Pts',(-0.212213495110603,0.00316856811982108,
0.00941909623229276));
#31091=CARTESIAN_POINT('Ctrl Pts',(-0.212207457373319,0.0032115948867045,
0.00944197486295772));
#31092=CARTESIAN_POINT('Ctrl Pts',(-0.212199536090053,0.00326894492966083,
0.00947189457532482));
#31093=CARTESIAN_POINT('Ctrl Pts',(-0.212192466189656,0.00332170276326728,
0.0094986935446409));
#31094=CARTESIAN_POINT('Ctrl Pts',(-0.212185396289258,0.00337446059687373,
0.00952549251395698));
#31095=CARTESIAN_POINT('Ctrl Pts',(-0.212179174818905,0.00342255601183432,
0.00954931216789045));
#31096=CARTESIAN_POINT('Ctrl Pts',(-0.212173291629739,0.00346902581832251,
0.00957188405703276));
#31097=CARTESIAN_POINT('Ctrl Pts',(-0.212161525251405,0.0035619654312989,
0.00961702783531737));
#31098=CARTESIAN_POINT('Ctrl Pts',(-0.212151109901664,0.00364834124124333,
0.00965728405441869));
#31099=CARTESIAN_POINT('Ctrl Pts',(-0.212140505592993,0.00374529742170372,
0.00970048237318596));
#31100=CARTESIAN_POINT('Ctrl Pts',(-0.212129901284321,0.00384225360216411,
0.00974368069195322));
#31101=CARTESIAN_POINT('Ctrl Pts',(-0.212119116554359,0.00394997858201931,
0.00978941616389929));
#31102=CARTESIAN_POINT('Ctrl Pts',(-0.212110151027643,0.00405046555875387,
0.00982991641873049));
#31103=CARTESIAN_POINT('Ctrl Pts',(-0.212105013763328,0.00410804479263682,
0.00985312314383084));
#31104=CARTESIAN_POINT('Ctrl Pts',(-0.212100471309807,0.00416321195017911,
0.00987469792720441));
#31105=CARTESIAN_POINT('Ctrl Pts',(-0.212096372540523,0.00421814681610697,
0.00989559901519815));
#31106=CARTESIAN_POINT('Ctrl Pts',(-0.212093318159167,0.00425908398983895,
0.00991117439625962));
#31107=CARTESIAN_POINT('Ctrl Pts',(-0.212090510162419,0.00429989388723458,
0.00992637191619471));
#31108=CARTESIAN_POINT('Ctrl Pts',(-0.212087886011393,0.00434150293396735,
0.00994152638604518));
#31109=CARTESIAN_POINT('Ctrl Pts',(-0.212075594849675,0.00453639397381732,
0.0100125078340582));
#31110=CARTESIAN_POINT('Ctrl Pts',(-0.212067360748948,0.00474904926940472,
0.0100818793281687));
#31111=CARTESIAN_POINT('Ctrl Pts',(-0.212063881613349,0.00495460319093813,
0.0101409226567405));
#31112=CARTESIAN_POINT('Ctrl Pts',(-0.21206040247775,0.00516015711247153,
0.0101999659853123));
#31113=CARTESIAN_POINT('Ctrl Pts',(-0.212061656540207,0.00535834953744217,
0.0102496659483022));
#31114=CARTESIAN_POINT('Ctrl Pts',(-0.212066560444648,0.00556611709299906,
0.0102944330158904));
#31115=CARTESIAN_POINT('Ctrl Pts',(-0.212069012396869,0.00567000087077749,
0.0103168165496846));
#31116=CARTESIAN_POINT('Ctrl Pts',(-0.212072378553916,0.00577628596176437,
0.0103378898590875));
#31117=CARTESIAN_POINT('Ctrl Pts',(-0.212076975297797,0.00588702112727913,
0.0103577274103283));
#31118=CARTESIAN_POINT('Ctrl Pts',(-0.21207728891332,0.00589457609831334,
0.0103590808387926));
#31119=CARTESIAN_POINT('Ctrl Pts',(-0.212077608279109,0.00590215187063596,
0.0103604284012948));
#31120=CARTESIAN_POINT('Ctrl Pts',(-0.212077933064703,0.00590974366334612,
0.0103617691152544));
#31121=CARTESIAN_POINT('',(-0.213095020058853,0.0026146493650334,0.00911535572166111));
#31122=CARTESIAN_POINT('Ctrl Pts',(-0.212877121847906,0.00590794924227077,
0.0103793151952651));
#31123=CARTESIAN_POINT('Ctrl Pts',(-0.212876817456775,0.00590068523348327,
0.0103780347325747));
#31124=CARTESIAN_POINT('Ctrl Pts',(-0.212871947615568,0.00578279537987255,
0.0103571043018428));
#31125=CARTESIAN_POINT('Ctrl Pts',(-0.212861880781934,0.00545750062331711,
0.0102921968347704));
#31126=CARTESIAN_POINT('Ctrl Pts',(-0.212858979669491,0.00496282289052902,
0.010168825226635));
#31127=CARTESIAN_POINT('Ctrl Pts',(-0.212879715250166,0.00442960172647075,
0.00999463393014085));
#31128=CARTESIAN_POINT('Ctrl Pts',(-0.212908265302508,0.00405688428523701,
0.00985175853701584));
#31129=CARTESIAN_POINT('Ctrl Pts',(-0.212940510942374,0.00373315259093314,
0.00971412549795729));
#31130=CARTESIAN_POINT('Ctrl Pts',(-0.212966389766975,0.00351758829891117,
0.00961302767103597));
#31131=CARTESIAN_POINT('Ctrl Pts',(-0.21299110390974,0.00332551002962964,
0.00951799089112226));
#31132=CARTESIAN_POINT('Ctrl Pts',(-0.213014561259845,0.00315500318886664,
0.00942878763037121));
#31133=CARTESIAN_POINT('Ctrl Pts',(-0.213027232407688,0.00306672600484153,
0.00938077473444571));
#31134=CARTESIAN_POINT('Ctrl Pts',(-0.213053447606084,0.00288696467213194,
0.0092805471432282));
#31135=CARTESIAN_POINT('Ctrl Pts',(-0.213076928211355,0.00273164707469549,
0.00918853718936164));
#31136=CARTESIAN_POINT('Ctrl Pts',(-0.213095020058853,0.0026146493650334,
0.00911535572166111));
#31137=CARTESIAN_POINT('',(-0.214296906974989,0.00261538462477282,0.00913979240089912));
#31138=CARTESIAN_POINT('',(-0.213095020167502,0.00261465278607558,0.00911535027878834));
#31139=CARTESIAN_POINT('Ctrl Pts',(-0.214296906974989,0.00261538462477282,
0.00913979240089912));
#31140=CARTESIAN_POINT('Ctrl Pts',(-0.214278683661499,0.0027331943743573,
0.00921366437608414));
#31141=CARTESIAN_POINT('Ctrl Pts',(-0.214262960945703,0.00283716004480444,
0.00927527307807957));
#31142=CARTESIAN_POINT('Ctrl Pts',(-0.214248964299891,0.00293164466650735,
0.00932935789200659));
#31143=CARTESIAN_POINT('Ctrl Pts',(-0.214241965944719,0.00297888719516994,
0.00935640042364937));
#31144=CARTESIAN_POINT('Ctrl Pts',(-0.214235400126686,0.00302378966695629,
0.00938151165815695));
#31145=CARTESIAN_POINT('Ctrl Pts',(-0.214230038337221,0.00306071935690244,
0.00940186736996042));
#31146=CARTESIAN_POINT('Ctrl Pts',(-0.214224676547756,0.00309764904684859,
0.00942222308176389));
#31147=CARTESIAN_POINT('Ctrl Pts',(-0.214220516304366,0.00312653814109853,
0.00943794444374524));
#31148=CARTESIAN_POINT('Ctrl Pts',(-0.214214476041821,0.00316955964443814,
0.00946090868045039));
#31149=CARTESIAN_POINT('Ctrl Pts',(-0.214208435779277,0.00321258114777775,
0.00948387291715554));
#31150=CARTESIAN_POINT('Ctrl Pts',(-0.214200519934111,0.00326985069535863,
0.00951386507025742));
#31151=CARTESIAN_POINT('Ctrl Pts',(-0.21419344857914,0.00332255570074024,
0.00954073938679254));
#31152=CARTESIAN_POINT('Ctrl Pts',(-0.214186377224168,0.00337526070612183,
0.00956761370332765));
#31153=CARTESIAN_POINT('Ctrl Pts',(-0.214180147412035,0.00342333094238063,
0.00959151115435043));
#31154=CARTESIAN_POINT('Ctrl Pts',(-0.214174255823015,0.00346976009689579,
0.00961414826400449));
#31155=CARTESIAN_POINT('Ctrl Pts',(-0.214162472644975,0.00356261840592612,
0.00965942248331261));
#31156=CARTESIAN_POINT('Ctrl Pts',(-0.214152040175484,0.00364884865052032,
0.00969976288009719));
#31157=CARTESIAN_POINT('Ctrl Pts',(-0.214141374430434,0.0037458485751099,
0.00974313915376534));
#31158=CARTESIAN_POINT('Ctrl Pts',(-0.214130708685383,0.00384284849969948,
0.0097865154274335));
#31159=CARTESIAN_POINT('Ctrl Pts',(-0.214119818429043,0.00395081202920119,
0.00983251236920754));
#31160=CARTESIAN_POINT('Ctrl Pts',(-0.214110754468016,0.00405125305607647,
0.00987313187882039));
#31161=CARTESIAN_POINT('Ctrl Pts',(-0.21410584648218,0.00410564022033151,
0.00989512667526963));
#31162=CARTESIAN_POINT('Ctrl Pts',(-0.214101471672964,0.00415778941429641,
0.00991562349899335));
#31163=CARTESIAN_POINT('Ctrl Pts',(-0.214097498720132,0.00420960497907179,
0.00993546753367953));
#31164=CARTESIAN_POINT('Ctrl Pts',(-0.214094134510461,0.00425348126742845,
0.00995227102876493));
#31165=CARTESIAN_POINT('Ctrl Pts',(-0.214091058445176,0.00429711967373464,
0.00996860379932433));
#31166=CARTESIAN_POINT('Ctrl Pts',(-0.21408819079082,0.00434170808743411,
0.00998489955126376));
#31167=CARTESIAN_POINT('Ctrl Pts',(-0.214075682387318,0.00453619800875275,
0.0100559798891715));
#31168=CARTESIAN_POINT('Ctrl Pts',(-0.214067163840417,0.00474900888568837,
0.0101256532944664));
#31169=CARTESIAN_POINT('Ctrl Pts',(-0.214063467913489,0.00495457669098817,
0.0101849000646645));
#31170=CARTESIAN_POINT('Ctrl Pts',(-0.214059771986562,0.00516014449628797,
0.0102441468348626));
#31171=CARTESIAN_POINT('Ctrl Pts',(-0.214060876327417,0.00535820131743478,
0.0102939778670901));
#31172=CARTESIAN_POINT('Ctrl Pts',(-0.214065643033967,0.00556593470413897,
0.010338888699365));
#31173=CARTESIAN_POINT('Ctrl Pts',(-0.214068026387243,0.00566980139749106,
0.0103613441155025));
#31174=CARTESIAN_POINT('Ctrl Pts',(-0.214071327128676,0.00577609514550041,
0.0103824901485091));
#31175=CARTESIAN_POINT('Ctrl Pts',(-0.214075858954125,0.00588681471194534,
0.0104023917424961));
#31176=CARTESIAN_POINT('Ctrl Pts',(-0.214076109948858,0.00589294690488345,
0.0104034939904368));
#31177=CARTESIAN_POINT('Ctrl Pts',(-0.21407636473448,0.00589909273188374,
0.0104045923486797));
#31178=CARTESIAN_POINT('Ctrl Pts',(-0.214076623138809,0.00590524964646623,
0.0104056862898775));
#31179=CARTESIAN_POINT('',(-0.215095387779062,0.00254083911603525,0.00910817608666392));
#31180=CARTESIAN_POINT('Ctrl Pts',(-0.214881405086202,0.00590343232515273,
0.010423413516648));
#31181=CARTESIAN_POINT('Ctrl Pts',(-0.214880634996676,0.0058860381335411,
0.0104203038817212));
#31182=CARTESIAN_POINT('Ctrl Pts',(-0.214875181880235,0.00575899415021333,
0.0103971687692641));
#31183=CARTESIAN_POINT('Ctrl Pts',(-0.214863259396212,0.00540815197451475,
0.0103257881481459));
#31184=CARTESIAN_POINT('Ctrl Pts',(-0.21485881772863,0.00492199098674758,
0.0102003515580181));
#31185=CARTESIAN_POINT('Ctrl Pts',(-0.214879521846151,0.00428142262289701,
0.00998901365476671));
#31186=CARTESIAN_POINT('Ctrl Pts',(-0.21492306243039,0.00377039219960215,
0.00977517598710994));
#31187=CARTESIAN_POINT('Ctrl Pts',(-0.214961186236713,0.00345337595410416,
0.00962364176435926));
#31188=CARTESIAN_POINT('Ctrl Pts',(-0.214986535367109,0.00326005586289953,
0.00952561866829564));
#31189=CARTESIAN_POINT('Ctrl Pts',(-0.215011018507601,0.00308691740069967,
0.00943286197251718));
#31190=CARTESIAN_POINT('Ctrl Pts',(-0.215024066419253,0.00299903924354964,
0.00938388910997964));
#31191=CARTESIAN_POINT('Ctrl Pts',(-0.215051493871513,0.00281738091061636,
0.00928015442866946));
#31192=CARTESIAN_POINT('Ctrl Pts',(-0.215076239262129,0.00265981257200034,
0.0091845066913352));
#31193=CARTESIAN_POINT('Ctrl Pts',(-0.21509538156927,0.00254083793378764,
0.00910817641020345));
#31194=CARTESIAN_POINT('',(-0.216305478212088,0.00249450055261697,0.0091019248989092));
#31195=CARTESIAN_POINT('',(-0.216305478212094,0.00249450055261262,0.00910192489890646));
#31196=CARTESIAN_POINT('',(-0.216062907480361,0.00488362583018296,0.0102080439741779));
#31197=CARTESIAN_POINT('Ctrl Pts',(-0.216305476043056,0.00249442883403143,
0.00910203441955642));
#31198=CARTESIAN_POINT('Ctrl Pts',(-0.216285528067716,0.00261530638056923,
0.00918082306942033));
#31199=CARTESIAN_POINT('Ctrl Pts',(-0.216268407797524,0.00272160085692102,
0.00924619788180913));
#31200=CARTESIAN_POINT('Ctrl Pts',(-0.216253248996245,0.00281784221559503,
0.00930336533804196));
#31201=CARTESIAN_POINT('Ctrl Pts',(-0.216245669595605,0.00286596289493204,
0.00933194906615837));
#31202=CARTESIAN_POINT('Ctrl Pts',(-0.216238581667216,0.0029116046264753,
0.00935842590971943));
#31203=CARTESIAN_POINT('Ctrl Pts',(-0.216232848132246,0.00294879195706751,
0.00937969025108412));
#31204=CARTESIAN_POINT('Ctrl Pts',(-0.216227114597277,0.00298597928765971,
0.00940095459244882));
#31205=CARTESIAN_POINT('Ctrl Pts',(-0.216222732797858,0.00301463648393093,
0.00941713680921905));
#31206=CARTESIAN_POINT('Ctrl Pts',(-0.216216255707853,0.00305825974051661,
0.00944129560807781));
#31207=CARTESIAN_POINT('Ctrl Pts',(-0.216209778617848,0.00310188299710228,
0.00946545440693656));
#31208=CARTESIAN_POINT('Ctrl Pts',(-0.216201211043208,0.00316060313598794,
0.00949735579945492));
#31209=CARTESIAN_POINT('Ctrl Pts',(-0.216193623289001,0.00321437996309083,
0.00952579235973773));
#31210=CARTESIAN_POINT('Ctrl Pts',(-0.216186035534794,0.00326815679019373,
0.00955422892002053));
#31211=CARTESIAN_POINT('Ctrl Pts',(-0.216179424282587,0.00331690730906704,
0.00957936016153829));
#31212=CARTESIAN_POINT('Ctrl Pts',(-0.216173121802343,0.00336460771594108,
0.00960347034857651));
#31213=CARTESIAN_POINT('Ctrl Pts',(-0.216160516841855,0.00346000852968916,
0.00965169072265294));
#31214=CARTESIAN_POINT('Ctrl Pts',(-0.216149147333713,0.00355120858816052,
0.00969581189039489));
#31215=CARTESIAN_POINT('Ctrl Pts',(-0.21613851162561,0.00364634481300223,
0.00973989636120167));
#31216=CARTESIAN_POINT('Ctrl Pts',(-0.2161190043515,0.00382083704217086,
0.00982075302327328));
#31217=CARTESIAN_POINT('Ctrl Pts',(-0.216101977184963,0.00400880962548444,
0.00990097638128006));
#31218=CARTESIAN_POINT('Ctrl Pts',(-0.216089367063548,0.0042011026592489,
0.00997515160791293));
#31219=CARTESIAN_POINT('Ctrl Pts',(-0.216088226666079,0.00421849269713606,
0.00998185965123713));
#31220=CARTESIAN_POINT('Ctrl Pts',(-0.216087122393437,0.00423591729012979,
0.00998851982343922));
#31221=CARTESIAN_POINT('Ctrl Pts',(-0.216086055678229,0.00425336915853703,
0.00999512922278139));
#31222=CARTESIAN_POINT('Ctrl Pts',(-0.216073203026403,0.00446364345351091,
0.0100747646379956));
#31223=CARTESIAN_POINT('Ctrl Pts',(-0.216065801916377,0.00467803753865652,
0.0101467659415394));
#31224=CARTESIAN_POINT('Ctrl Pts',(-0.216062907480361,0.00488362583018296,
0.0102080439741779));
#31225=CARTESIAN_POINT('Ctrl Pts',(-0.216062901115481,0.00488407842295695,
0.0102081788612459));
#31226=CARTESIAN_POINT('Ctrl Pts',(-0.216060011174114,0.0050898046430285,
0.010269486110157));
#31227=CARTESIAN_POINT('Ctrl Pts',(-0.216061613315435,0.00528640638840204,
0.010320988079685));
#31228=CARTESIAN_POINT('Ctrl Pts',(-0.216067188608646,0.00550199323050043,
0.0103693743259898));
#31229=CARTESIAN_POINT('Ctrl Pts',(-0.216069976255251,0.00560978665154961,
0.0103935674491422));
#31230=CARTESIAN_POINT('Ctrl Pts',(-0.216073762550609,0.00572237856012717,
0.0104167410336067));
#31231=CARTESIAN_POINT('Ctrl Pts',(-0.216078386138244,0.00583381988821942,
0.0104375135503685));
#31232=CARTESIAN_POINT('Ctrl Pts',(-0.21607930894028,0.00585606198517916,
0.0104416594479437));
#31233=CARTESIAN_POINT('Ctrl Pts',(-0.216080264909954,0.00587825743762793,
0.0104457133990444));
#31234=CARTESIAN_POINT('Ctrl Pts',(-0.216081273279547,0.00590074222848906,
0.0104497344249182));
#31235=CARTESIAN_POINT('',(-0.216863172025247,0.00484538612872985,0.0102141167849625));
#31236=CARTESIAN_POINT('Ctrl Pts',(-0.216882060774437,0.00589894167293226,
0.0104673301115656));
#31237=CARTESIAN_POINT('Ctrl Pts',(-0.21688064798073,0.00586753673964817,
0.0104617001234162));
#31238=CARTESIAN_POINT('Ctrl Pts',(-0.216879344316105,0.00583690163752463,
0.0104560440440929));
#31239=CARTESIAN_POINT('Ctrl Pts',(-0.216878102848578,0.00580618452906231,
0.0104502144772882));
#31240=CARTESIAN_POINT('Ctrl Pts',(-0.216873527769665,0.00569298527727355,
0.0104287312507224));
#31241=CARTESIAN_POINT('Ctrl Pts',(-0.216869802272862,0.00557869658909491,
0.0104047720299247));
#31242=CARTESIAN_POINT('Ctrl Pts',(-0.216867065285671,0.00546980918598949,
0.0103798919273287));
#31243=CARTESIAN_POINT('Ctrl Pts',(-0.216861591311289,0.00525203437977865,
0.0103301317221365));
#31244=CARTESIAN_POINT('Ctrl Pts',(-0.216860045750518,0.00505561827550841,
0.0102778374033075));
#31245=CARTESIAN_POINT('Ctrl Pts',(-0.216863157842011,0.00484633783112493,
0.0102144052983154));
#31246=CARTESIAN_POINT('',(-0.217119273430717,0.0024305071256748,0.00907584540398619));
#31247=CARTESIAN_POINT('Ctrl Pts',(-0.216863172025247,0.00484538612872985,
0.0102141167849625));
#31248=CARTESIAN_POINT('Ctrl Pts',(-0.216866293584769,0.00463638521299101,
0.010150743228241));
#31249=CARTESIAN_POINT('Ctrl Pts',(-0.216874088025862,0.00441498954598536,
0.0100749918698983));
#31250=CARTESIAN_POINT('Ctrl Pts',(-0.216887342836659,0.00420167942231494,
0.00999259466276242));
#31251=CARTESIAN_POINT('Ctrl Pts',(-0.216900617768194,0.00398804549490104,
0.00991007237706179));
#31252=CARTESIAN_POINT('Ctrl Pts',(-0.216919362976275,0.0037823580735198,
0.00982120221383172));
#31253=CARTESIAN_POINT('Ctrl Pts',(-0.216941537033173,0.00359082137253702,
0.00973075178358121));
#31254=CARTESIAN_POINT('Ctrl Pts',(-0.216952624061622,0.00349505302204562,
0.00968552656845596));
#31255=CARTESIAN_POINT('Ctrl Pts',(-0.216964565666134,0.00340276546101606,
0.00964003070473679));
#31256=CARTESIAN_POINT('Ctrl Pts',(-0.216977870016699,0.0033064635405045,
0.00959041939952468));
#31257=CARTESIAN_POINT('Ctrl Pts',(-0.216984522191982,0.00325831258024871,
0.00956561374691862));
#31258=CARTESIAN_POINT('Ctrl Pts',(-0.216991514963515,0.00320915775019089,
0.00953978303292521));
#31259=CARTESIAN_POINT('Ctrl Pts',(-0.216999509061169,0.00315526226612399,
0.00951073631106921));
#31260=CARTESIAN_POINT('Ctrl Pts',(-0.217007503158823,0.00310136678205709,
0.00948168958921321));
#31261=CARTESIAN_POINT('Ctrl Pts',(-0.217016501721846,0.00304281090104423,
0.00944927559171635));
#31262=CARTESIAN_POINT('Ctrl Pts',(-0.217023463140776,0.00299839750608262,
0.00942420754471762));
#31263=CARTESIAN_POINT('Ctrl Pts',(-0.217030424559705,0.002953984111121,
0.00939913949771888));
#31264=CARTESIAN_POINT('Ctrl Pts',(-0.217035344236295,0.00292358530827852,
0.00938164187589816));
#31265=CARTESIAN_POINT('Ctrl Pts',(-0.217041614060813,0.00288528083541392,
0.00935929849242598));
#31266=CARTESIAN_POINT('Ctrl Pts',(-0.217047883885331,0.00284697636254933,
0.00933695510895381));
#31267=CARTESIAN_POINT('Ctrl Pts',(-0.217055506430902,0.00280084130501947,
0.0093096393351554));
#31268=CARTESIAN_POINT('Ctrl Pts',(-0.217063632569623,0.00275245324254402,
0.00928030736224485));
#31269=CARTESIAN_POINT('Ctrl Pts',(-0.217079884271406,0.00265568054541311,
0.00922164549430653));
#31270=CARTESIAN_POINT('Ctrl Pts',(-0.217098146072681,0.00254976472927551,
0.00915512598934796));
#31271=CARTESIAN_POINT('Ctrl Pts',(-0.217119270108823,0.00243050678069039,
0.00907584503782427));
#31272=CARTESIAN_POINT('',(-0.217721579458628,0.00223307602259744,0.00895185568871232));
#31273=CARTESIAN_POINT('Ctrl Pts',(-0.21711927235356,0.00243049410780578,
0.00907583661306065));
#31274=CARTESIAN_POINT('Ctrl Pts',(-0.21715405112409,0.0024102994618794,
0.00906302774800916));
#31275=CARTESIAN_POINT('Ctrl Pts',(-0.217180991959541,0.00239439998998887,
0.009052830909679));
#31276=CARTESIAN_POINT('Ctrl Pts',(-0.217281466712797,0.00234147243426244,
0.00901889238814732));
#31277=CARTESIAN_POINT('Ctrl Pts',(-0.21740416090901,0.00229616636516378,
0.00898995712725975));
#31278=CARTESIAN_POINT('Ctrl Pts',(-0.217546627510568,0.00225882515584664,
0.00896664401489687));
#31279=CARTESIAN_POINT('Ctrl Pts',(-0.217667742709476,0.00223981443389805,
0.00895557566262542));
#31280=CARTESIAN_POINT('Ctrl Pts',(-0.217721023725957,0.00223314551106483,
0.0089518940398779));
#31281=CARTESIAN_POINT('',(-0.218374009456864,0.00220395340354362,0.00894382805299407));
#31282=CARTESIAN_POINT('Ctrl Pts',(-0.217721579458628,0.00223307602259744,
0.00895185568871232));
#31283=CARTESIAN_POINT('Ctrl Pts',(-0.21777462485247,0.00222644993024188,
0.00894819969666044));
#31284=CARTESIAN_POINT('Ctrl Pts',(-0.217843500492621,0.00222071614871092,
0.00894546415784734));
#31285=CARTESIAN_POINT('Ctrl Pts',(-0.21795203985176,0.00221399343120396,
0.00894279214610887));
#31286=CARTESIAN_POINT('Ctrl Pts',(-0.218059615657004,0.00221007637826625,
0.00894209068652028));
#31287=CARTESIAN_POINT('Ctrl Pts',(-0.218090952814536,0.00220943320496267,
0.00894224077459141));
#31288=CARTESIAN_POINT('Ctrl Pts',(-0.218193344854828,0.00220709767477518,
0.00894256413753163));
#31289=CARTESIAN_POINT('Ctrl Pts',(-0.218292688378998,0.00220532673074213,
0.00894322944625219));
#31290=CARTESIAN_POINT('Ctrl Pts',(-0.218374009477688,0.0022039549723325,
0.00894382881947807));
#31291=CARTESIAN_POINT('Ctrl Pts',(-0.21837401321167,0.00220395490934618,
0.00894382884699923));
#31292=CARTESIAN_POINT('Ctrl Pts',(-0.218347327019386,0.00233073163754938,
0.00903391891599098));
#31293=CARTESIAN_POINT('Ctrl Pts',(-0.218313244025542,0.00249725023685972,
0.00914542258472829));
#31294=CARTESIAN_POINT('Ctrl Pts',(-0.218276224804953,0.00268641686649291,
0.00926436126954177));
#31295=CARTESIAN_POINT('Ctrl Pts',(-0.218259608411032,0.00277265227047954,
0.00931734129371121));
#31296=CARTESIAN_POINT('Ctrl Pts',(-0.218226397494956,0.00295607982361697,
0.00942555592083442));
#31297=CARTESIAN_POINT('Ctrl Pts',(-0.218193056409799,0.00315860668144401,
0.00953855943967181));
#31298=CARTESIAN_POINT('Ctrl Pts',(-0.218143468698842,0.00350244065109768,
0.00971834447840922));
#31299=CARTESIAN_POINT('Ctrl Pts',(-0.218096988684672,0.00398464218054674,
0.00994167473146692));
#31300=CARTESIAN_POINT('Ctrl Pts',(-0.218064351217329,0.00472231338075253,
0.0102132450057751));
#31301=CARTESIAN_POINT('Ctrl Pts',(-0.218061145319316,0.00533446433286351,
0.010381457620077));
#31302=CARTESIAN_POINT('Ctrl Pts',(-0.218071819718671,0.00573502223192124,
0.0104641816390526));
#31303=CARTESIAN_POINT('Ctrl Pts',(-0.218078126203157,0.00589629686000176,
0.0104933642872807));
#31304=CARTESIAN_POINT('',(-0.218872841325269,0.00457002221966434,0.0101695959270065));
#31305=CARTESIAN_POINT('Ctrl Pts',(-0.218877735683465,0.00589448248302666,
0.0105110260225545));
#31306=CARTESIAN_POINT('Ctrl Pts',(-0.218869908846724,0.00569722419377274,
0.0104751900008672));
#31307=CARTESIAN_POINT('Ctrl Pts',(-0.21885909932305,0.00524620508486855,
0.0103787976603652));
#31308=CARTESIAN_POINT('Ctrl Pts',(-0.218864452106764,0.00481504949286933,
0.0102534457740855));
#31309=CARTESIAN_POINT('Ctrl Pts',(-0.218872841325269,0.00457002221966434,
0.0101695959270065));
#31310=CARTESIAN_POINT('',(-0.219237122161378,0.00196588366579876,0.00878419704042442));
#31311=CARTESIAN_POINT('Ctrl Pts',(-0.218872841325269,0.00457002221966434,
0.0101695959270065));
#31312=CARTESIAN_POINT('Ctrl Pts',(-0.21887288147815,0.00456884945835792,
0.0101691946008402));
#31313=CARTESIAN_POINT('Ctrl Pts',(-0.218881377447727,0.0043214277508718,
0.0100844669395035));
#31314=CARTESIAN_POINT('Ctrl Pts',(-0.218909465557103,0.00380701625999766,
0.00988371263113285));
#31315=CARTESIAN_POINT('Ctrl Pts',(-0.218965255863169,0.00330128827775189,
0.00963459578682774));
#31316=CARTESIAN_POINT('Ctrl Pts',(-0.219023132009435,0.00294578045365914,
0.00943649611216199));
#31317=CARTESIAN_POINT('Ctrl Pts',(-0.219062281129155,0.00273678173079582,
0.00931208982376108));
#31318=CARTESIAN_POINT('Ctrl Pts',(-0.219100727104508,0.00255057403123827,
0.00919488413309952));
#31319=CARTESIAN_POINT('Ctrl Pts',(-0.219121593502578,0.00245608880301823,
0.00913290506119713));
#31320=CARTESIAN_POINT('Ctrl Pts',(-0.219165689106097,0.00226104671154717,
0.0090016478891487));
#31321=CARTESIAN_POINT('Ctrl Pts',(-0.219205899434897,0.00209250238596427,
0.00888065413454422));
#31322=CARTESIAN_POINT('Ctrl Pts',(-0.219237120080246,0.00196588454101197,
0.00878419780604263));
#31323=CARTESIAN_POINT('',(-0.220515396330818,0.00171983677662007,0.00861251054687271));
#31324=CARTESIAN_POINT('Ctrl Pts',(-0.219237121894096,0.00196588334575157,
0.00878419692442275));
#31325=CARTESIAN_POINT('Ctrl Pts',(-0.219299626976512,0.00192469477845702,
0.00875381637932707));
#31326=CARTESIAN_POINT('Ctrl Pts',(-0.219328791989107,0.00190449437925005,
0.00873852202848415));
#31327=CARTESIAN_POINT('Ctrl Pts',(-0.219370104955956,0.00188158207234747,
0.00872130386843637));
#31328=CARTESIAN_POINT('Ctrl Pts',(-0.219411418322426,0.0018586695438135,
0.00870408554183684));
#31329=CARTESIAN_POINT('Ctrl Pts',(-0.21946488229829,0.00183314526670501,
0.00868481535297067));
#31330=CARTESIAN_POINT('Ctrl Pts',(-0.219515065969969,0.00181363474941354,
0.00867012142979744));
#31331=CARTESIAN_POINT('Ctrl Pts',(-0.219565249641647,0.00179412423212207,
0.00865542750662421));
#31332=CARTESIAN_POINT('Ctrl Pts',(-0.219612152255416,0.00178059461885503,
0.00864535024413309));
#31333=CARTESIAN_POINT('Ctrl Pts',(-0.219667138977168,0.0017684847471806,
0.00863654086155548));
#31334=CARTESIAN_POINT('Ctrl Pts',(-0.21972212569892,0.00175637487550616,
0.00862773147897786));
#31335=CARTESIAN_POINT('Ctrl Pts',(-0.219785196792223,0.00174569649105899,
0.0086201757710797));
#31336=CARTESIAN_POINT('Ctrl Pts',(-0.219840326400044,0.00173864261881232,
0.00861542023136484));
#31337=CARTESIAN_POINT('Ctrl Pts',(-0.219895456007866,0.00173158874656564,
0.00861066469164997));
#31338=CARTESIAN_POINT('Ctrl Pts',(-0.219942644030734,0.00172815491285034,
0.00860871469223284));
#31339=CARTESIAN_POINT('Ctrl Pts',(-0.219995935354278,0.00172516870068701,
0.00860724722282935));
#31340=CARTESIAN_POINT('Ctrl Pts',(-0.22002258101605,0.00172367559460533,
0.00860651348812759));
#31341=CARTESIAN_POINT('Ctrl Pts',(-0.220050752516637,0.00172229500271428,
0.00860589965062664));
#31342=CARTESIAN_POINT('Ctrl Pts',(-0.2200834455773,0.00172127519818041,
0.00860566665592181));
#31343=CARTESIAN_POINT('Ctrl Pts',(-0.220116138637963,0.00172025539364654,
0.00860543366121698));
#31344=CARTESIAN_POINT('Ctrl Pts',(-0.220153353257484,0.00171959632170309,
0.00860558157489872));
#31345=CARTESIAN_POINT('Ctrl Pts',(-0.220177426297593,0.0017192735952131,
0.00860576272676545));
#31346=CARTESIAN_POINT('Ctrl Pts',(-0.220201499337701,0.00171895086872311,
0.00860594387863219));
#31347=CARTESIAN_POINT('Ctrl Pts',(-0.220212430798545,0.00171896449443078,
0.00860615826066572));
#31348=CARTESIAN_POINT('Ctrl Pts',(-0.220231151258488,0.00171895355001152,
0.00860649716681914));
#31349=CARTESIAN_POINT('Ctrl Pts',(-0.220249871718431,0.00171894260559226,
0.00860683607297256));
#31350=CARTESIAN_POINT('Ctrl Pts',(-0.220276381177714,0.00171890710174357,
0.0086072994902706));
#31351=CARTESIAN_POINT('Ctrl Pts',(-0.220305446991561,0.00171893726234777,
0.00860786466002522));
#31352=CARTESIAN_POINT('Ctrl Pts',(-0.220363496787337,0.00171899749864198,
0.00860899340835503));
#31353=CARTESIAN_POINT('Ctrl Pts',(-0.220431743233002,0.00171931965465264,
0.00861052802037448));
#31354=CARTESIAN_POINT('Ctrl Pts',(-0.220515396906419,0.0017198140099196,
0.00861249175807416));
#31355=CARTESIAN_POINT('',(-0.220090123052826,0.00418422702945123,0.0100543441066292));
#31356=CARTESIAN_POINT('Ctrl Pts',(-0.220515730216856,0.00171988949744531,
0.00861256027472298));
#31357=CARTESIAN_POINT('Ctrl Pts',(-0.2204787502135,0.00185191957789771,
0.00872086836689029));
#31358=CARTESIAN_POINT('Ctrl Pts',(-0.220431475220976,0.00202642732684206,
0.0088552288217874));
#31359=CARTESIAN_POINT('Ctrl Pts',(-0.220380060197333,0.00222577410457095,
0.00899883778024211));
#31360=CARTESIAN_POINT('Ctrl Pts',(-0.220356866873776,0.00231728500818783,
0.00906316072720875));
#31361=CARTESIAN_POINT('Ctrl Pts',(-0.220310804517265,0.0025107909266704,
0.00919355179597007));
#31362=CARTESIAN_POINT('Ctrl Pts',(-0.22026427845596,0.00272565546041714,
0.00933016407728968));
#31363=CARTESIAN_POINT('Ctrl Pts',(-0.220214048696187,0.00298877544138231,
0.0094869312743888));
#31364=CARTESIAN_POINT('Ctrl Pts',(-0.220168303850216,0.00329732711792897,
0.00965475980118518));
#31365=CARTESIAN_POINT('Ctrl Pts',(-0.220124020098812,0.00368476694613528,
0.0098472904300802));
#31366=CARTESIAN_POINT('Ctrl Pts',(-0.220100733172946,0.00399954421165778,
0.00998183202500825));
#31367=CARTESIAN_POINT('Ctrl Pts',(-0.220090123052826,0.00418422702945123,
0.0100543441066292));
#31368=CARTESIAN_POINT('Ctrl Pts',(-0.220090123052826,0.00418422702945123,
0.0100543441066292));
#31369=CARTESIAN_POINT('Ctrl Pts',(-0.220085741756582,0.00426048913833528,
0.0100842869260536));
#31370=CARTESIAN_POINT('Ctrl Pts',(-0.22006865820386,0.00459786319220902,
0.0102119119804006));
#31371=CARTESIAN_POINT('Ctrl Pts',(-0.220057266568638,0.00515049295929986,
0.0103826020783711));
#31372=CARTESIAN_POINT('Ctrl Pts',(-0.220068242884761,0.00565866356698218,
0.0104949899253311));
#31373=CARTESIAN_POINT('Ctrl Pts',(-0.220077799936617,0.00589176565002776,
0.0105374974776579));
#31374=CARTESIAN_POINT('',(-0.220878064831259,0.00441518816723556,0.010159021015619));
#31375=CARTESIAN_POINT('Ctrl Pts',(-0.220877304433504,0.005889967920973,
0.0105550654063144));
#31376=CARTESIAN_POINT('Ctrl Pts',(-0.220867873084289,0.00565698015616214,
0.0105124902878897));
#31377=CARTESIAN_POINT('Ctrl Pts',(-0.220857137503969,0.00515102574076155,
0.0104003859982906));
#31378=CARTESIAN_POINT('Ctrl Pts',(-0.220866927623,0.00467143026566601,
0.010252099464527));
#31379=CARTESIAN_POINT('Ctrl Pts',(-0.220878064831259,0.00441518816723555,
0.010159021015619));
#31380=CARTESIAN_POINT('',(-0.22131162872866,0.00171848461492949,0.00862620042871455));
#31381=CARTESIAN_POINT('Ctrl Pts',(-0.220878064831259,0.00441518816723555,
0.010159021015619));
#31382=CARTESIAN_POINT('Ctrl Pts',(-0.220878125769484,0.00441378611580685,
0.0101585117286085));
#31383=CARTESIAN_POINT('Ctrl Pts',(-0.220889418682641,0.00415468323385347,
0.0100643205656675));
#31384=CARTESIAN_POINT('Ctrl Pts',(-0.220915691899767,0.00375090589786667,
0.00989718271122343));
#31385=CARTESIAN_POINT('Ctrl Pts',(-0.220966875360685,0.00329663029328944,
0.00967108003973233));
#31386=CARTESIAN_POINT('Ctrl Pts',(-0.221011932596698,0.00298750926251152,
0.00950262161274992));
#31387=CARTESIAN_POINT('Ctrl Pts',(-0.221061613606449,0.00272319363643506,
0.00934478944388032));
#31388=CARTESIAN_POINT('Ctrl Pts',(-0.221107658471592,0.00250831974463547,
0.00920780036239895));
#31389=CARTESIAN_POINT('Ctrl Pts',(-0.22115290161688,0.00231659335985024,
0.00907833412010607));
#31390=CARTESIAN_POINT('Ctrl Pts',(-0.221176749851974,0.0022219001842754,
0.0090116372053751));
#31391=CARTESIAN_POINT('Ctrl Pts',(-0.221228087258136,0.00202224227626237,
0.00886734674608652));
#31392=CARTESIAN_POINT('Ctrl Pts',(-0.221275053893402,0.0018488960404024,
0.00873344289084019));
#31393=CARTESIAN_POINT('Ctrl Pts',(-0.221311628647049,0.00171848099653553,
0.00862620480166822));
#31394=CARTESIAN_POINT('',(-0.222515290917713,0.00171959987501164,0.00864956777322578));
#31395=CARTESIAN_POINT('',(-0.222515294138235,0.0017195974700428,0.00864957427254232));
#31396=CARTESIAN_POINT('',(-0.222078164866776,0.00441016936810972,0.0101832963470285));
#31397=CARTESIAN_POINT('Ctrl Pts',(-0.222515294294555,0.001719604422929,
0.00864956589294009));
#31398=CARTESIAN_POINT('Ctrl Pts',(-0.222478295083331,0.00185148585221865,
0.00875829495302256));
#31399=CARTESIAN_POINT('Ctrl Pts',(-0.222431004461355,0.00202580118070899,
0.00889315927644579));
#31400=CARTESIAN_POINT('Ctrl Pts',(-0.222379582487375,0.00222492582905654,
0.00903728689367557));
#31401=CARTESIAN_POINT('Ctrl Pts',(-0.222356400503344,0.00231628042355402,
0.00910180240101161));
#31402=CARTESIAN_POINT('Ctrl Pts',(-0.222310329407263,0.00250961375404974,
0.00923268188529682));
#31403=CARTESIAN_POINT('Ctrl Pts',(-0.222263805202746,0.00272427901799516,
0.00936978963283741));
#31404=CARTESIAN_POINT('Ctrl Pts',(-0.222213573950343,0.00298724356776438,
0.00952716266338013));
#31405=CARTESIAN_POINT('Ctrl Pts',(-0.222167882126563,0.00329538526363372,
0.00969550364880327));
#31406=CARTESIAN_POINT('Ctrl Pts',(-0.222116050585726,0.00374888191031054,
0.00992184840756128));
#31407=CARTESIAN_POINT('Ctrl Pts',(-0.22208954781103,0.00415219063406005,
0.0100892050101901));
#31408=CARTESIAN_POINT('Ctrl Pts',(-0.222078164866776,0.00441016936810972,
0.0101832963470285));
#31409=CARTESIAN_POINT('Ctrl Pts',(-0.222078164866776,0.00441016936810972,
0.0101832963470285));
#31410=CARTESIAN_POINT('Ctrl Pts',(-0.222066781922521,0.00466814810215939,
0.010277387683867));
#31411=CARTESIAN_POINT('Ctrl Pts',(-0.222056884058924,0.00514792738117401,
0.0104261488910504));
#31412=CARTESIAN_POINT('Ctrl Pts',(-0.222067759901967,0.00565493991166382,
0.0105388114001075));
#31413=CARTESIAN_POINT('Ctrl Pts',(-0.222077231673906,0.00588727068028781,
0.0105814273450436));
#31414=CARTESIAN_POINT('',(-0.222877366335621,0.00441446037918135,0.010202254105996));
#31415=CARTESIAN_POINT('Ctrl Pts',(-0.222876594854072,0.00588547347265862,
0.0105989910637735));
#31416=CARTESIAN_POINT('Ctrl Pts',(-0.222867236637191,0.0056535094866434,
0.0105563517608772));
#31417=CARTESIAN_POINT('Ctrl Pts',(-0.222856543043364,0.00514894106148145,
0.0104440457130052));
#31418=CARTESIAN_POINT('Ctrl Pts',(-0.222866259370916,0.00467063128315652,
0.0102956405003283));
#31419=CARTESIAN_POINT('Ctrl Pts',(-0.222877366335621,0.00441446037918135,
0.010202254105996));
#31420=CARTESIAN_POINT('',(-0.223310598441629,0.00172037808899711,0.00866504596072886));
#31421=CARTESIAN_POINT('Ctrl Pts',(-0.222877366335621,0.00441446037918135,
0.010202254105996));
#31422=CARTESIAN_POINT('Ctrl Pts',(-0.222877427216057,0.00441305623351044,
0.0102017422285763));
#31423=CARTESIAN_POINT('Ctrl Pts',(-0.222888689808771,0.00415402014935639,
0.0101072373799785));
#31424=CARTESIAN_POINT('Ctrl Pts',(-0.222914911877449,0.00375031358671893,
0.00993952094031038));
#31425=CARTESIAN_POINT('Ctrl Pts',(-0.222966020223457,0.00329641991277213,
0.00971274202800391));
#31426=CARTESIAN_POINT('Ctrl Pts',(-0.223010999642036,0.00298774591557504,
0.00954388284591602));
#31427=CARTESIAN_POINT('Ctrl Pts',(-0.223060660360825,0.00272361201166209,
0.00938554249185679));
#31428=CARTESIAN_POINT('Ctrl Pts',(-0.22310667914932,0.00250900816207285,
0.00924817752991824));
#31429=CARTESIAN_POINT('Ctrl Pts',(-0.223151897149871,0.00231757035963003,
0.00911838245209231));
#31430=CARTESIAN_POINT('Ctrl Pts',(-0.223175741921343,0.00222299932167633,
0.00905149866904686));
#31431=CARTESIAN_POINT('Ctrl Pts',(-0.223227067761469,0.00202363190136062,
0.00890682204395355));
#31432=CARTESIAN_POINT('Ctrl Pts',(-0.223274027990358,0.00185055987416555,
0.008772564000113));
#31433=CARTESIAN_POINT('Ctrl Pts',(-0.223310598360652,0.00172037449465496,
0.00866505028583386));
#31434=CARTESIAN_POINT('',(-0.22451413759973,0.00172149826865404,0.00868849301140827));
#31435=CARTESIAN_POINT('',(-0.224514141137082,0.00172149591023567,0.00868849946384148));
#31436=CARTESIAN_POINT('',(-0.224077512165814,0.00440948083533129,0.0102265543111367));
#31437=CARTESIAN_POINT('Ctrl Pts',(-0.224514141292166,0.00172150281505916,
0.00868849117770473));
#31438=CARTESIAN_POINT('Ctrl Pts',(-0.224477127539949,0.00185316341858383,
0.00879750297306098));
#31439=CARTESIAN_POINT('Ctrl Pts',(-0.224429821708012,0.0020272114172923,
0.00893272203677245));
#31440=CARTESIAN_POINT('Ctrl Pts',(-0.224378393526143,0.00222604404169074,
0.00907722494518334));
#31441=CARTESIAN_POINT('Ctrl Pts',(-0.224355212184233,0.00231725880918394,
0.00914190243096556));
#31442=CARTESIAN_POINT('Ctrl Pts',(-0.224309153980272,0.00251031221158726,
0.0092731150758879));
#31443=CARTESIAN_POINT('Ctrl Pts',(-0.224262658189644,0.00272469317168506,
0.00941058427657283));
#31444=CARTESIAN_POINT('Ctrl Pts',(-0.224212448790665,0.00298758394571889,
0.00956851511516764));
#31445=CARTESIAN_POINT('Ctrl Pts',(-0.22416695331413,0.00329483890266449,
0.00973701079873431));
#31446=CARTESIAN_POINT('Ctrl Pts',(-0.224115276532478,0.00374784709684887,
0.00996400980407875));
#31447=CARTESIAN_POINT('Ctrl Pts',(-0.224088854784422,0.00415138504334779,
0.0101320881672501));
#31448=CARTESIAN_POINT('Ctrl Pts',(-0.224077512165814,0.00440948083533129,
0.0102265543111367));
#31449=CARTESIAN_POINT('Ctrl Pts',(-0.224077512165814,0.00440948083533129,
0.0102265543111367));
#31450=CARTESIAN_POINT('Ctrl Pts',(-0.224066169547205,0.00466757662731479,
0.0103210204550233));
#31451=CARTESIAN_POINT('Ctrl Pts',(-0.224056346761501,0.00514637502274445,
0.0104699487051214));
#31452=CARTESIAN_POINT('Ctrl Pts',(-0.224067139686817,0.00565155572807021,
0.0105826959046413));
#31453=CARTESIAN_POINT('Ctrl Pts',(-0.224076522719914,0.00588277614622425,
0.010625353510046));
#31454=CARTESIAN_POINT('',(-0.224861013570565,0.00514872644714179,0.0104774172001444));
#31455=CARTESIAN_POINT('Ctrl Pts',(-0.224876132721504,0.00588096715315318,
0.010642983684972));
#31456=CARTESIAN_POINT('Ctrl Pts',(-0.224873876977941,0.00582530573000602,
0.0106327721265318));
#31457=CARTESIAN_POINT('Ctrl Pts',(-0.224871939109516,0.00577104612314958,
0.0106222934022558));
#31458=CARTESIAN_POINT('Ctrl Pts',(-0.224870228490649,0.00571703883957485,
0.0106113664450536));
#31459=CARTESIAN_POINT('Ctrl Pts',(-0.224864186040655,0.00552626793404857,
0.0105727689563051));
#31460=CARTESIAN_POINT('Ctrl Pts',(-0.224860982253214,0.0053386745032014,
0.010528627448495));
#31461=CARTESIAN_POINT('Ctrl Pts',(-0.224861013570565,0.00514872644714179,
0.0104774172001444));
#31462=CARTESIAN_POINT('',(-0.225016038273092,0.00296527551678717,0.00956936417862582));
#31463=CARTESIAN_POINT('Ctrl Pts',(-0.224861013572329,0.00514871576703485,
0.0104774143207667));
#31464=CARTESIAN_POINT('Ctrl Pts',(-0.224861045011535,0.00495876406267532,
0.0104262028476539));
#31465=CARTESIAN_POINT('Ctrl Pts',(-0.224864318374763,0.00476651357778983,
0.0103676238876547));
#31466=CARTESIAN_POINT('Ctrl Pts',(-0.224870299865164,0.00457982853857772,
0.0103039536618325));
#31467=CARTESIAN_POINT('Ctrl Pts',(-0.224874787677354,0.00443976187652935,
0.0102561829564754));
#31468=CARTESIAN_POINT('Ctrl Pts',(-0.224880794323499,0.00430277850927414,
0.0102057344389205));
#31469=CARTESIAN_POINT('Ctrl Pts',(-0.224888888524025,0.00416354177025105,
0.0101504648328106));
#31470=CARTESIAN_POINT('Ctrl Pts',(-0.22489158251621,0.00411719961630877,
0.0101320694537414));
#31471=CARTESIAN_POINT('Ctrl Pts',(-0.224894507758821,0.00407061140369965,
0.0101131309480136));
#31472=CARTESIAN_POINT('Ctrl Pts',(-0.224897685220289,0.00402359104486503,
0.0100935454711003));
#31473=CARTESIAN_POINT('Ctrl Pts',(-0.224910409483873,0.00383529625498036,
0.0100151146944838));
#31474=CARTESIAN_POINT('Ctrl Pts',(-0.224927195735951,0.00364029587212845,
0.00992575724485829));
#31475=CARTESIAN_POINT('Ctrl Pts',(-0.224947037735793,0.00346158123324218,
0.00983655079837782));
#31476=CARTESIAN_POINT('Ctrl Pts',(-0.224966879735635,0.00328286659435591,
0.00974734435189736));
#31477=CARTESIAN_POINT('Ctrl Pts',(-0.224989763415531,0.00312007330588168,
0.00965896274411867));
#31478=CARTESIAN_POINT('Ctrl Pts',(-0.225016038256768,0.00296527508664285,
0.00956936496560957));
#31479=CARTESIAN_POINT('',(-0.224916806541977,0.00225236367453649,0.00910630060086145));
#31480=CARTESIAN_POINT('Ctrl Pts',(-0.224916806541977,0.00225236367453649,
0.00910630060086145));
#31481=CARTESIAN_POINT('Ctrl Pts',(-0.224925107451042,0.0022867865741508,
0.00913108304394155));
#31482=CARTESIAN_POINT('Ctrl Pts',(-0.224934577499929,0.00232677962479607,
0.00915938195723326));
#31483=CARTESIAN_POINT('Ctrl Pts',(-0.224940840264972,0.00235358065782448,
0.00917812690403259));
#31484=CARTESIAN_POINT('Ctrl Pts',(-0.224943971647494,0.00236698117433867,
0.00918749937743225));
#31485=CARTESIAN_POINT('Ctrl Pts',(-0.224946300530641,0.00237706002817518,
0.00919451756818138));
#31486=CARTESIAN_POINT('Ctrl Pts',(-0.224949803337872,0.00239269484820365,
0.00920532904796304));
#31487=CARTESIAN_POINT('Ctrl Pts',(-0.224953306145103,0.00240832966823212,
0.00921614052774471));
#31488=CARTESIAN_POINT('Ctrl Pts',(-0.224957983354394,0.00242953672177531,
0.0092307213123541));
#31489=CARTESIAN_POINT('Ctrl Pts',(-0.224962642765517,0.0024523455269545,
0.00924621970596788));
#31490=CARTESIAN_POINT('Ctrl Pts',(-0.224967302176641,0.00247515433213368,
0.00926171809958165));
#31491=CARTESIAN_POINT('Ctrl Pts',(-0.224971944115544,0.00249957632337157,
0.00927811764714866));
#31492=CARTESIAN_POINT('Ctrl Pts',(-0.22497502021215,0.002516263112879,
0.00928924524523537));
#31493=CARTESIAN_POINT('Ctrl Pts',(-0.224978096308756,0.00253294990238644,
0.00930037284332207));
#31494=CARTESIAN_POINT('Ctrl Pts',(-0.224979605738828,0.00254187416662664,
0.00930626963940711));
#31495=CARTESIAN_POINT('Ctrl Pts',(-0.224981323970798,0.00255244156080663,
0.00931323962525843));
#31496=CARTESIAN_POINT('Ctrl Pts',(-0.224984760434737,0.00257357634916661,
0.00932717959696107));
#31497=CARTESIAN_POINT('Ctrl Pts',(-0.224989033102982,0.00260131561018695,
0.00934536288226375));
#31498=CARTESIAN_POINT('Ctrl Pts',(-0.224993267136316,0.00263670970994627,
0.00936812186650835));
#31499=CARTESIAN_POINT('Ctrl Pts',(-0.22499750116965,0.00267210380970558,
0.00939088085075294));
#31500=CARTESIAN_POINT('Ctrl Pts',(-0.225001697732016,0.00271519019647569,
0.00941815775499642));
#31501=CARTESIAN_POINT('Ctrl Pts',(-0.225004924284085,0.00275672452315482,
0.00944392421210905));
#31502=CARTESIAN_POINT('Ctrl Pts',(-0.225011377388222,0.00283979317651308,
0.0094954571263343));
#31503=CARTESIAN_POINT('Ctrl Pts',(-0.225013949525124,0.00291662592926665,
0.00954099361814959));
#31504=CARTESIAN_POINT('Ctrl Pts',(-0.225016038255883,0.00296527505804455,
0.00956936494893859));
#31505=CARTESIAN_POINT('',(-0.224893951312673,0.00215954182917785,0.00903842305818316));
#31506=CARTESIAN_POINT('Ctrl Pts',(-0.224894117235589,0.00215936362032008,
0.0090384489139208));
#31507=CARTESIAN_POINT('Ctrl Pts',(-0.224901382162618,0.00218904986783135,
0.00906039555723563));
#31508=CARTESIAN_POINT('Ctrl Pts',(-0.22490851174212,0.00221796610908876,
0.00908153639687648));
#31509=CARTESIAN_POINT('Ctrl Pts',(-0.224916806541977,0.00225236367453649,
0.00910630060086145));
#31510=CARTESIAN_POINT('',(-0.225192864116067,0.00215336578416129,0.0090401066669318));
#31511=CARTESIAN_POINT('Ctrl Pts',(-0.225192864116067,0.00215336578416129,
0.0090401066669318));
#31512=CARTESIAN_POINT('Ctrl Pts',(-0.225178650597281,0.00215018411373376,
0.0090375238652442));
#31513=CARTESIAN_POINT('Ctrl Pts',(-0.225106377344745,0.00214366180682612,
0.00903105599729165));
#31514=CARTESIAN_POINT('Ctrl Pts',(-0.225029554110752,0.00214766777237138,
0.00903226288021996));
#31515=CARTESIAN_POINT('Ctrl Pts',(-0.224982815408334,0.0021501049729653,
0.00903299713910372));
#31516=CARTESIAN_POINT('Ctrl Pts',(-0.224934623015444,0.00215576840919723,
0.00903656911590101));
#31517=CARTESIAN_POINT('Ctrl Pts',(-0.224894101884154,0.00215924465310947,
0.0090384761514828));
#31518=CARTESIAN_POINT('',(-0.225309762150681,0.00172192258384158,0.00870374069204483));
#31519=CARTESIAN_POINT('Ctrl Pts',(-0.225309727116455,0.00172192354877486,
0.0087037407145231));
#31520=CARTESIAN_POINT('Ctrl Pts',(-0.22530317830787,0.00174518401655161,
0.00872303397847708));
#31521=CARTESIAN_POINT('Ctrl Pts',(-0.225294343614693,0.00177668638927144,
0.00874892851577175));
#31522=CARTESIAN_POINT('Ctrl Pts',(-0.225285108854914,0.0018098826098087,
0.0087757558166547));
#31523=CARTESIAN_POINT('Ctrl Pts',(-0.225275874095134,0.00184307883034596,
0.00880258311753764));
#31524=CARTESIAN_POINT('Ctrl Pts',(-0.225266236284159,0.00187783685288663,
0.00883050216082895));
#31525=CARTESIAN_POINT('Ctrl Pts',(-0.225250743755804,0.00193502853970644,
0.00887505746406453));
#31526=CARTESIAN_POINT('Ctrl Pts',(-0.225242997491627,0.00196362438311634,
0.00889733511568232));
#31527=CARTESIAN_POINT('Ctrl Pts',(-0.22523378933279,0.00199790200373627,
0.00892367851192004));
#31528=CARTESIAN_POINT('Ctrl Pts',(-0.225226379114346,0.00202573868501456,
0.00894479940232736));
#31529=CARTESIAN_POINT('Ctrl Pts',(-0.225218968895902,0.00205357536629284,
0.00896592029273469));
#31530=CARTESIAN_POINT('Ctrl Pts',(-0.225213355324292,0.00207492092211016,
0.00898188540034371));
#31531=CARTESIAN_POINT('Ctrl Pts',(-0.225208692897504,0.0020927133473497,
0.00899512574048781));
#31532=CARTESIAN_POINT('Ctrl Pts',(-0.225199368044517,0.00212829819557704,
0.00902160641910038));
#31533=CARTESIAN_POINT('Ctrl Pts',(-0.225193848093542,0.00214968062354274,
0.00903717209931391));
#31534=CARTESIAN_POINT('Ctrl Pts',(-0.225192867237934,0.00215347928706473,
0.00903994966696521));
#31535=CARTESIAN_POINT('',(-0.226513589418857,0.00172251996741961,0.00872682375665345));
#31536=CARTESIAN_POINT('',(-0.226513566923304,0.00172248770006411,0.00872680494013574));
#31537=CARTESIAN_POINT('',(-0.226388511915541,0.00218154661642265,0.00908391582781536));
#31538=CARTESIAN_POINT('Origin',(-0.227809208820185,0.0077947739147323,
0.00186791552810384));
#31539=CARTESIAN_POINT('',(-0.227126457729194,0.00216864693516063,0.00908890020183529));
#31540=CARTESIAN_POINT('Ctrl Pts',(-0.227126457686547,0.00216864674301375,
0.00908890049261823));
#31541=CARTESIAN_POINT('Ctrl Pts',(-0.227069511598769,0.00216683783452681,
0.00908645418986856));
#31542=CARTESIAN_POINT('Ctrl Pts',(-0.226996374298308,0.00216473238471204,
0.00908347211408987));
#31543=CARTESIAN_POINT('Ctrl Pts',(-0.226950724459553,0.00216328058498747,
0.00908150913472941));
#31544=CARTESIAN_POINT('Ctrl Pts',(-0.226927899540175,0.00216255468512519,
0.00908052764504917));
#31545=CARTESIAN_POINT('Ctrl Pts',(-0.226911946486128,0.00216199220282908,
0.0090798009302647));
#31546=CARTESIAN_POINT('Ctrl Pts',(-0.226878445021426,0.00216151559286356,
0.00907879431088333));
#31547=CARTESIAN_POINT('Ctrl Pts',(-0.226844943556723,0.00216103898289804,
0.00907778769150196));
#31548=CARTESIAN_POINT('Ctrl Pts',(-0.22679389368015,0.00216064819788032,
0.00907650123031305));
#31549=CARTESIAN_POINT('Ctrl Pts',(-0.226755321775082,0.00216082600807531,
0.0090758780305106));
#31550=CARTESIAN_POINT('Ctrl Pts',(-0.226716749870014,0.00216100381827029,
0.00907525483070816));
#31551=CARTESIAN_POINT('Ctrl Pts',(-0.226690655937283,0.00216175025630935,
0.00907529484930442));
#31552=CARTESIAN_POINT('Ctrl Pts',(-0.226660619377659,0.00216286586100168,
0.00907552918802821));
#31553=CARTESIAN_POINT('Ctrl Pts',(-0.226645601097847,0.00216342366334784,
0.0090756463573901));
#31554=CARTESIAN_POINT('Ctrl Pts',(-0.226629597161646,0.00216407376972869,
0.00907581208977323));
#31555=CARTESIAN_POINT('Ctrl Pts',(-0.226616481400393,0.00216469456716155,
0.00907601255758363));
#31556=CARTESIAN_POINT('Ctrl Pts',(-0.22660336563914,0.0021653153645944,
0.00907621302539404));
#31557=CARTESIAN_POINT('Ctrl Pts',(-0.226593138052681,0.0021659068472081,
0.00907644823658608));
#31558=CARTESIAN_POINT('Ctrl Pts',(-0.226584540496384,0.0021663878207974,
0.00907663392975817));
#31559=CARTESIAN_POINT('Ctrl Pts',(-0.226575942940087,0.00216686879438671,
0.00907681962293026));
#31560=CARTESIAN_POINT('Ctrl Pts',(-0.226568975411353,0.00216723916088945,
0.00907695593104604));
#31561=CARTESIAN_POINT('Ctrl Pts',(-0.226550639842415,0.00216850438230813,
0.00907752745248047));
#31562=CARTESIAN_POINT('Ctrl Pts',(-0.226532304273477,0.00216976960372682,
0.00907809897391489));
#31563=CARTESIAN_POINT('Ctrl Pts',(-0.226502600673821,0.00217193003788991,
0.00907910522340853));
#31564=CARTESIAN_POINT('Ctrl Pts',(-0.226479110584875,0.00217375905389338,
0.00907998802605441));
#31565=CARTESIAN_POINT('Ctrl Pts',(-0.226432130408324,0.00217741708579578,
0.00908175363129572));
#31566=CARTESIAN_POINT('Ctrl Pts',(-0.226410004232402,0.00217974791219932,
0.00908302753406069));
#31567=CARTESIAN_POINT('Ctrl Pts',(-0.226389230132104,0.00218171579433513,
0.0090840616145203));
#31568=CARTESIAN_POINT('',(-0.227456889100304,0.00310986692736372,0.00970247513229321));
#31569=CARTESIAN_POINT('Ctrl Pts',(-0.227126457802366,0.00216864671205002,
0.00908890047209336));
#31570=CARTESIAN_POINT('Ctrl Pts',(-0.227159535805671,0.00227599956143099,
0.00916856953561649));
#31571=CARTESIAN_POINT('Ctrl Pts',(-0.227187513613841,0.00236732543188503,
0.00923287923821631));
#31572=CARTESIAN_POINT('Ctrl Pts',(-0.227212366497972,0.00244695262818679,
0.00928748991883584));
#31573=CARTESIAN_POINT('Ctrl Pts',(-0.227224792950202,0.0024867662589028,
0.00931479528147973));
#31574=CARTESIAN_POINT('Ctrl Pts',(-0.227236439141077,0.00252368956619642,
0.00933962692867829));
#31575=CARTESIAN_POINT('Ctrl Pts',(-0.227245326881853,0.00255182296877999,
0.0093583577637486));
#31576=CARTESIAN_POINT('Ctrl Pts',(-0.227254214622629,0.00257995637136356,
0.0093770885988189));
#31577=CARTESIAN_POINT('Ctrl Pts',(-0.227260341931496,0.00259923427900408,
0.00938981725628631));
#31578=CARTESIAN_POINT('Ctrl Pts',(-0.227271624596063,0.00263280783658688,
0.00941167475306709));
#31579=CARTESIAN_POINT('Ctrl Pts',(-0.22728290726063,0.00266638139416968,
0.00943353224984788));
#31580=CARTESIAN_POINT('Ctrl Pts',(-0.227299349172753,0.00271437568475871,
0.00946432593436038));
#31581=CARTESIAN_POINT('Ctrl Pts',(-0.227313897631145,0.00275564085759007,
0.00949028007023457));
#31582=CARTESIAN_POINT('Ctrl Pts',(-0.227328446089537,0.00279690603042142,
0.00951623420610876));
#31583=CARTESIAN_POINT('Ctrl Pts',(-0.227341097755956,0.00283134072815765,
0.00953751239998761));
#31584=CARTESIAN_POINT('Ctrl Pts',(-0.227355539970987,0.00286855708676149,
0.00956020192181762));
#31585=CARTESIAN_POINT('Ctrl Pts',(-0.227384424401048,0.00294298980396916,
0.00960558096547763));
#31586=CARTESIAN_POINT('Ctrl Pts',(-0.227420479239962,0.00302878982864503,
0.00965620512905418));
#31587=CARTESIAN_POINT('Ctrl Pts',(-0.227454425262618,0.00310438966814835,
0.00969935154573664));
#31588=CARTESIAN_POINT('Ctrl Pts',(-0.227455247752368,0.00310622140242,
0.0097003969549684));
#31589=CARTESIAN_POINT('Ctrl Pts',(-0.227456068999624,0.00310804702874932,
0.0097014381899936));
#31590=CARTESIAN_POINT('Ctrl Pts',(-0.227456889100304,0.00310986692736372,
0.00970247513229321));
#31591=CARTESIAN_POINT('',(-0.227996742054428,0.00407722443014096,0.010182633458461));
#31592=CARTESIAN_POINT('Ctrl Pts',(-0.227456889100304,0.00310986692736372,
0.00970247513229321));
#31593=CARTESIAN_POINT('Ctrl Pts',(-0.227489916419944,0.00318315234385685,
0.0097442455461831));
#31594=CARTESIAN_POINT('Ctrl Pts',(-0.227521084158742,0.00324691103035285,
0.00977946177872144));
#31595=CARTESIAN_POINT('Ctrl Pts',(-0.227556657287862,0.00331641920530898,
0.00981682420858073));
#31596=CARTESIAN_POINT('Ctrl Pts',(-0.227593113732605,0.00338765333629757,
0.00985511438415112));
#31597=CARTESIAN_POINT('Ctrl Pts',(-0.227634201182863,0.0034650263648679,
0.00989546321334494));
#31598=CARTESIAN_POINT('Ctrl Pts',(-0.227677579152443,0.00354337392575307,
0.00993486812925494));
#31599=CARTESIAN_POINT('Ctrl Pts',(-0.227720957122022,0.00362172148663825,
0.00997427304516493));
#31600=CARTESIAN_POINT('Ctrl Pts',(-0.227766623657143,0.00370099813863763,
0.0100128262267389));
#31601=CARTESIAN_POINT('Ctrl Pts',(-0.22781719085636,0.0037856188794736,
0.0100523849767061));
#31602=CARTESIAN_POINT('Ctrl Pts',(-0.227867758055577,0.00387023962030957,
0.0100919437266733));
#31603=CARTESIAN_POINT('Ctrl Pts',(-0.227923229539478,0.003960286039776,
0.0101323378246218));
#31604=CARTESIAN_POINT('Ctrl Pts',(-0.227975492399613,0.00404349318073738,
0.01016818210575));
#31605=CARTESIAN_POINT('Ctrl Pts',(-0.227982632850327,0.00405486141599234,
0.0101730793563429));
#31606=CARTESIAN_POINT('Ctrl Pts',(-0.227989713277371,0.0040661009235916,
0.0101778942512805));
#31607=CARTESIAN_POINT('Ctrl Pts',(-0.227996742054428,0.00407722443014096,
0.010182633458461));
#31608=CARTESIAN_POINT('',(-0.229324382301549,0.00587096534799219,0.0107407249786847));
#31609=CARTESIAN_POINT('Ctrl Pts',(-0.227996742054428,0.00407722443014096,
0.010182633458461));
#31610=CARTESIAN_POINT('Ctrl Pts',(-0.228012423148243,0.00410204034163872,
0.0101932074978731));
#31611=CARTESIAN_POINT('Ctrl Pts',(-0.228027847164962,0.00412627831447172,
0.0102034059753793));
#31612=CARTESIAN_POINT('Ctrl Pts',(-0.22804310708817,0.00415007794112182,
0.0102133064578917));
#31613=CARTESIAN_POINT('Ctrl Pts',(-0.228121134654993,0.00427177101477283,
0.0102639299472963));
#31614=CARTESIAN_POINT('Ctrl Pts',(-0.228194871969436,0.0043818969845919,
0.0103070169724305));
#31615=CARTESIAN_POINT('Ctrl Pts',(-0.228276749669893,0.00450012916764758,
0.0103506786545054));
#31616=CARTESIAN_POINT('Ctrl Pts',(-0.228381817769972,0.00465184850969786,
0.0104067067299922));
#31617=CARTESIAN_POINT('Ctrl Pts',(-0.228500318179664,0.00481723537212066,
0.0104627171434107));
#31618=CARTESIAN_POINT('Ctrl Pts',(-0.228612318903402,0.00496837639600633,
0.0105095656396236));
#31619=CARTESIAN_POINT('Ctrl Pts',(-0.22872431962714,0.00511951741989199,
0.0105564141358366));
#31620=CARTESIAN_POINT('Ctrl Pts',(-0.228829799907357,0.00525615538408106,
0.0105950375950328));
#31621=CARTESIAN_POINT('Ctrl Pts',(-0.228946501527974,0.00540372976852625,
0.0106330700434848));
#31622=CARTESIAN_POINT('Ctrl Pts',(-0.22906320314859,0.00555130415297142,
0.0106711024919367));
#31623=CARTESIAN_POINT('Ctrl Pts',(-0.229191139018856,0.00570993073471519,
0.0107079668985551));
#31624=CARTESIAN_POINT('Ctrl Pts',(-0.229324382301549,0.00587096534799219,
0.0107407249786847));
#31625=CARTESIAN_POINT('',(-0.224906597392078,-0.00157591257448374,-2.26466145009483E-7));
#31626=CARTESIAN_POINT('Ctrl Pts',(-0.229324382301549,0.00587096534799201,
0.0107407249786846));
#31627=CARTESIAN_POINT('Ctrl Pts',(-0.229485744817183,0.0056945111294132,
0.0107117116946865));
#31628=CARTESIAN_POINT('Ctrl Pts',(-0.229627896419902,0.00553927467669799,
0.0106807434520244));
#31629=CARTESIAN_POINT('Ctrl Pts',(-0.229747893835773,0.00540811338586742,
0.0106519514001228));
#31630=CARTESIAN_POINT('Ctrl Pts',(-0.229807892543708,0.00534253274045213,
0.010637555374172));
#31631=CARTESIAN_POINT('Ctrl Pts',(-0.229862352234134,0.00528296668078184,
0.0106237244445399));
#31632=CARTESIAN_POINT('Ctrl Pts',(-0.229914217593376,0.00522607416888484,
0.0106099639475152));
#31633=CARTESIAN_POINT('Ctrl Pts',(-0.229940150272997,0.00519762791293634,
0.0106030836990029));
#31634=CARTESIAN_POINT('Ctrl Pts',(-0.229965434797737,0.00516985488092608,
0.0105962018001159));
#31635=CARTESIAN_POINT('Ctrl Pts',(-0.229986021469801,0.00514724062456104,
0.0105905104176317));
#31636=CARTESIAN_POINT('Ctrl Pts',(-0.230006608141864,0.005124626368196,
0.0105848190351475));
#31637=CARTESIAN_POINT('Ctrl Pts',(-0.230022495585796,0.00510715427844391,
0.0105803802154135));
#31638=CARTESIAN_POINT('Ctrl Pts',(-0.23005025334464,0.00507646845205036,
0.0105723820814782));
#31639=CARTESIAN_POINT('Ctrl Pts',(-0.230078011103483,0.00504578262565681,
0.0105643839475428));
#31640=CARTESIAN_POINT('Ctrl Pts',(-0.230117641989443,0.0050019184211765,
0.0105526994501915));
#31641=CARTESIAN_POINT('Ctrl Pts',(-0.230153258691976,0.00496237482800372,
0.0105418193756453));
#31642=CARTESIAN_POINT('Ctrl Pts',(-0.230188875394509,0.00492283123483093,
0.0105309393010992));
#31643=CARTESIAN_POINT('Ctrl Pts',(-0.230220475803366,0.00488757956722113,
0.0105209592922955));
#31644=CARTESIAN_POINT('Ctrl Pts',(-0.230251831073634,0.00485249570357078,
0.0105108075114764));
#31645=CARTESIAN_POINT('Ctrl Pts',(-0.23031454161417,0.00478232797627009,
0.010490503949838));
#31646=CARTESIAN_POINT('Ctrl Pts',(-0.230376273367701,0.0047128594595253,
0.010469432600821));
#31647=CARTESIAN_POINT('Ctrl Pts',(-0.230435676939916,0.0046452906084165,
0.0104480309058724));
#31648=CARTESIAN_POINT('Ctrl Pts',(-0.230495080512131,0.0045777217573077,
0.0104266292109238));
#31649=CARTESIAN_POINT('Ctrl Pts',(-0.230552156757354,0.00451206165996326,
0.0104048588721916));
#31650=CARTESIAN_POINT('Ctrl Pts',(-0.230601790943484,0.00445464998250786,
0.0103851864819408));
#31651=CARTESIAN_POINT('Ctrl Pts',(-0.230651425129614,0.00439723830505247,
0.01036551409169));
#31652=CARTESIAN_POINT('Ctrl Pts',(-0.230693612158977,0.00434799447567126,
0.0103481724261956));
#31653=CARTESIAN_POINT('Ctrl Pts',(-0.230750173084339,0.00428034173840896,
0.0103233211117964));
#31654=CARTESIAN_POINT('Ctrl Pts',(-0.230785698409411,0.00423784976240384,
0.0103077122613954));
#31655=CARTESIAN_POINT('Ctrl Pts',(-0.230826898018337,0.00418813941981296,
0.0102890255602644));
#31656=CARTESIAN_POINT('Ctrl Pts',(-0.230868043325356,0.0041380196585314,
0.0102695877777448));
#31657=CARTESIAN_POINT('Ctrl Pts',(-0.230892406683903,0.00410834225902144,
0.0102580780892971));
#31658=CARTESIAN_POINT('Ctrl Pts',(-0.230916751003245,0.00407851845553815,
0.0102463132904993));
#31659=CARTESIAN_POINT('Ctrl Pts',(-0.230939886965452,0.00404993141261438,
0.0102348560676729));
#31660=CARTESIAN_POINT('Ctrl Pts',(-0.231002095384207,0.00397306602351662,
0.010204049667274));
#31661=CARTESIAN_POINT('Ctrl Pts',(-0.231055560302718,0.00390508230307037,
0.0101755863206212));
#31662=CARTESIAN_POINT('Ctrl Pts',(-0.231107716218532,0.00383663463987516,
0.0101459342198134));
#31663=CARTESIAN_POINT('Ctrl Pts',(-0.231159872134346,0.00376818697667996,
0.0101162821190056));
#31664=CARTESIAN_POINT('Ctrl Pts',(-0.231210722559944,0.00369934908414583,
0.0100852775894019));
#31665=CARTESIAN_POINT('Ctrl Pts',(-0.23125366084358,0.0036401127425717,
0.0100578020810351));
#31666=CARTESIAN_POINT('Ctrl Pts',(-0.231296599127216,0.00358087640099757,
0.0100303265726683));
#31667=CARTESIAN_POINT('Ctrl Pts',(-0.231331618607131,0.00353109481495246,
0.010006692012866));
#31668=CARTESIAN_POINT('Ctrl Pts',(-0.231377720840595,0.0034600055015645,
0.00997160014698702));
#31669=CARTESIAN_POINT('Ctrl Pts',(-0.231423823074059,0.00338891618817653,
0.00993650828110805));
#31670=CARTESIAN_POINT('Ctrl Pts',(-0.23148101976334,0.00329679652888858,
0.00988940692844755));
#31671=CARTESIAN_POINT('Ctrl Pts',(-0.231528065134197,0.00321433493027825,
0.00984527396904159));
#31672=CARTESIAN_POINT('Ctrl Pts',(-0.231575110505053,0.00313187333166792,
0.00980114100963563));
#31673=CARTESIAN_POINT('Ctrl Pts',(-0.231611996080783,0.00305884309754429,
0.00976038232476601));
#31674=CARTESIAN_POINT('Ctrl Pts',(-0.231644324891522,0.00298614562233681,
0.00971846121248706));
#31675=CARTESIAN_POINT('Ctrl Pts',(-0.231676653702261,0.00291344814712933,
0.00967654010020812));
#31676=CARTESIAN_POINT('Ctrl Pts',(-0.231704428636809,0.00284116801872021,
0.00963331648308124));
#31677=CARTESIAN_POINT('Ctrl Pts',(-0.231726500112571,0.00277498507141569,
0.00959250676879874));
#31678=CARTESIAN_POINT('Ctrl Pts',(-0.231748571588332,0.00270880212411118,
0.00955169705451624));
#31679=CARTESIAN_POINT('Ctrl Pts',(-0.231764936016148,0.002648611310996,
0.00951347529255092));
#31680=CARTESIAN_POINT('Ctrl Pts',(-0.231774590797342,0.0025803707591514,
0.00946864508580836));
#31681=CARTESIAN_POINT('Ctrl Pts',(-0.23179390035973,0.00244388965546221,
0.00937898467232322));
#31682=CARTESIAN_POINT('Ctrl Pts',(-0.231786404517407,0.00227626681505629,
0.00926125907006112));
#31683=CARTESIAN_POINT('Ctrl Pts',(-0.231750544825356,0.00213535898381207,
0.00915480893757784));
#31684=CARTESIAN_POINT('Ctrl Pts',(-0.23173261497933,0.00206490506818996,
0.00910158387133621));
#31685=CARTESIAN_POINT('Ctrl Pts',(-0.231707586904214,0.00200084815486611,
0.00905154880698267));
#31686=CARTESIAN_POINT('Ctrl Pts',(-0.231673809741403,0.00193360097644109,
0.00899738195505023));
#31687=CARTESIAN_POINT('Ctrl Pts',(-0.231640032578592,0.00186635379801606,
0.00894321510311779));
#31688=CARTESIAN_POINT('Ctrl Pts',(-0.231597510631657,0.00179609770624624,
0.00888469242584056));
#31689=CARTESIAN_POINT('Ctrl Pts',(-0.231556525129873,0.00173699192756572,
0.00883408314100965));
#31690=CARTESIAN_POINT('Ctrl Pts',(-0.231515539628089,0.0016778861488852,
0.00878347385617874));
#31691=CARTESIAN_POINT('Ctrl Pts',(-0.231476085454303,0.00162970072198407,
0.00874104870017571));
#31692=CARTESIAN_POINT('Ctrl Pts',(-0.231426392419699,0.0015747691240097,
0.00869151559050962));
#31693=CARTESIAN_POINT('Ctrl Pts',(-0.231376699385095,0.00151983752603534,
0.00864198248084354));
#31694=CARTESIAN_POINT('Ctrl Pts',(-0.231316772114654,0.00145838108383666,
0.00858509258491536));
#31695=CARTESIAN_POINT('Ctrl Pts',(-0.23125919197483,0.00140349285592715,
0.00853288079893833));
#31696=CARTESIAN_POINT('Ctrl Pts',(-0.231210636673531,0.00135720754901295,
0.0084888524411187));
#31697=CARTESIAN_POINT('Ctrl Pts',(-0.23116374812206,0.00131548725337962,
0.00844826339887426));
#31698=CARTESIAN_POINT('Ctrl Pts',(-0.231113995310445,0.00127324558096312,
0.00840637618589869));
#31699=CARTESIAN_POINT('Ctrl Pts',(-0.231104747894015,0.00126539423904196,
0.0083985907263659));
#31700=CARTESIAN_POINT('Ctrl Pts',(-0.231095401527076,0.00125752597447957,
0.00839075932832244));
#31701=CARTESIAN_POINT('Ctrl Pts',(-0.231085927115632,0.00124960959671496,
0.00838285012440887));
#31702=CARTESIAN_POINT('Ctrl Pts',(-0.23102547861739,0.00119910164166131,
0.0083323879398523));
#31703=CARTESIAN_POINT('Ctrl Pts',(-0.230959820200585,0.0011467024285488,
0.00827868812707598));
#31704=CARTESIAN_POINT('Ctrl Pts',(-0.230900331854038,0.00110097593680334,
0.00823078821303766));
#31705=CARTESIAN_POINT('Ctrl Pts',(-0.230840843507491,0.00105524944505788,
0.00818288829899935));
#31706=CARTESIAN_POINT('Ctrl Pts',(-0.230787522564886,0.00101604021632565,
0.00814094057038923));
#31707=CARTESIAN_POINT('Ctrl Pts',(-0.230723706818146,0.00097086547440946,
0.00809157173241625));
#31708=CARTESIAN_POINT('Ctrl Pts',(-0.230659891071407,0.000925690732493274,
0.00804220289444327));
#31709=CARTESIAN_POINT('Ctrl Pts',(-0.230585583966631,0.000874763691592227,
0.00798521205356764));
#31710=CARTESIAN_POINT('Ctrl Pts',(-0.230523287813335,0.000833165462424795,
0.0079376563861729));
#31711=CARTESIAN_POINT('Ctrl Pts',(-0.230460991660039,0.000791567233257364,
0.00789010071877815));
#31712=CARTESIAN_POINT('Ctrl Pts',(-0.230410702851443,0.000759054428482579,
0.00785219731383282));
#31713=CARTESIAN_POINT('Ctrl Pts',(-0.230346995596142,0.000718726127249372,
0.00780428928871881));
#31714=CARTESIAN_POINT('Ctrl Pts',(-0.230283288340841,0.00067839782601616,
0.00775638126360478));
#31715=CARTESIAN_POINT('Ctrl Pts',(-0.230206165710844,0.000630473690801921,
0.00769827947888727));
#31716=CARTESIAN_POINT('Ctrl Pts',(-0.230134314763537,0.000586713602453529,
0.00764390620766072));
#31717=CARTESIAN_POINT('Ctrl Pts',(-0.229990612868923,0.000499193425756742,
0.00753515966520764));
#31718=CARTESIAN_POINT('Ctrl Pts',(-0.229867988787896,0.000427617586995964,
0.00744190204492346));
#31719=CARTESIAN_POINT('Ctrl Pts',(-0.229741940634664,0.000354928579326137,
0.00734383067639073));
#31720=CARTESIAN_POINT('Ctrl Pts',(-0.229615892481431,0.00028223957165631,
0.00724575930785799));
#31721=CARTESIAN_POINT('Ctrl Pts',(-0.229486422667975,0.000208701022860158,
0.00714269334481202));
#31722=CARTESIAN_POINT('Ctrl Pts',(-0.229352791967108,0.000133484776569742,
0.0070323021258392));
#31723=CARTESIAN_POINT('Ctrl Pts',(-0.22921916126624,5.82685302793252E-5,
0.00692191090686637));
#31724=CARTESIAN_POINT('Ctrl Pts',(-0.2290813721816,-1.84076324743832E-5,
0.00680402683203074));
#31725=CARTESIAN_POINT('Ctrl Pts',(-0.228955658434579,-8.75292797473743E-5,
0.00669278534604856));
#31726=CARTESIAN_POINT('Ctrl Pts',(-0.228829944687559,-0.000156650927020365,
0.00658154386006638));
#31727=CARTESIAN_POINT('Ctrl Pts',(-0.228716302957634,-0.000218638491031281,
0.00647721522647426));
#31728=CARTESIAN_POINT('Ctrl Pts',(-0.228596767895078,-0.000283494680059439,
0.00636287399597081));
#31729=CARTESIAN_POINT('Ctrl Pts',(-0.228477232832522,-0.000348350869087597,
0.00624853276546736));
#31730=CARTESIAN_POINT('Ctrl Pts',(-0.22835180668064,-0.000415691458055748,
0.0061239593033855));
#31731=CARTESIAN_POINT('Ctrl Pts',(-0.228232000846924,-0.000479070930306836,
0.0059999892371026));
#31732=CARTESIAN_POINT('Ctrl Pts',(-0.228112195013208,-0.000542450402557927,
0.00587601917081969));
#31733=CARTESIAN_POINT('Ctrl Pts',(-0.2279980084523,-0.000602119731771134,
0.00575278162222749));
#31734=CARTESIAN_POINT('Ctrl Pts',(-0.227883788318796,-0.000660850298491323,
0.00562412203559087));
#31735=CARTESIAN_POINT('Ctrl Pts',(-0.227876478715098,-0.000664608805459833,
0.00561588836818488));
#31736=CARTESIAN_POINT('Ctrl Pts',(-0.227869168977206,-0.000668363094667602,
0.00560763228811735));
#31737=CARTESIAN_POINT('Ctrl Pts',(-0.227861859699312,-0.000672112681594339,
0.00559935444695225));
#31738=CARTESIAN_POINT('Ctrl Pts',(-0.227640738892288,-0.000785545458312897,
0.0053489325933084));
#31739=CARTESIAN_POINT('Ctrl Pts',(-0.227420039070301,-0.000894106965719931,
0.00507834839397145));
#31740=CARTESIAN_POINT('Ctrl Pts',(-0.227216211219934,-0.000988261310786297,
0.00480738120895063));
#31741=CARTESIAN_POINT('Ctrl Pts',(-0.227005645720493,-0.00108552798292046,
0.00452745704479274));
#31742=CARTESIAN_POINT('Ctrl Pts',(-0.226813087273762,-0.00116864465803599,
0.00424754273693657));
#31743=CARTESIAN_POINT('Ctrl Pts',(-0.226626103958878,-0.00124135927987506,
0.00394958116680215));
#31744=CARTESIAN_POINT('Ctrl Pts',(-0.226439120643995,-0.00131407390171413,
0.00365161959666774));
#31745=CARTESIAN_POINT('Ctrl Pts',(-0.226257707321489,-0.00137553841474053,
0.00333545181780753));
#31746=CARTESIAN_POINT('Ctrl Pts',(-0.226089207901399,-0.00142040472594693,
0.00300946340189435));
#31747=CARTESIAN_POINT('Ctrl Pts',(-0.226004958191353,-0.00144283788155013,
0.00284646919393776));
#31748=CARTESIAN_POINT('Ctrl Pts',(-0.225923937374762,-0.00146113181346843,
0.00268101115962903));
#31749=CARTESIAN_POINT('Ctrl Pts',(-0.225847547993418,-0.00147482232186643,
0.00251597950542847));
#31750=CARTESIAN_POINT('Ctrl Pts',(-0.225818640550089,-0.00148000311517418,
0.00245352785171381));
#31751=CARTESIAN_POINT('Ctrl Pts',(-0.225790395885862,-0.00148452982481028,
0.00239113705018023));
#31752=CARTESIAN_POINT('Ctrl Pts',(-0.225762905281085,-0.0014883945315704,
0.0023290706209163));
#31753=CARTESIAN_POINT('Ctrl Pts',(-0.225717750572063,-0.00149474250792893,
0.00222712337107818));
#31754=CARTESIAN_POINT('Ctrl Pts',(-0.22567463029465,-0.00150078983555668,
0.00212686157789403));
#31755=CARTESIAN_POINT('Ctrl Pts',(-0.225633948962841,-0.00150645162391577,
0.00202917774223495));
#31756=CARTESIAN_POINT('Ctrl Pts',(-0.225568500459705,-0.00151556036142999,
0.00187202308332373));
#31757=CARTESIAN_POINT('Ctrl Pts',(-0.22550935008619,-0.00152369977831173,
0.00172226264086029));
#31758=CARTESIAN_POINT('Ctrl Pts',(-0.225446995528993,-0.00153173773051723,
0.00155812389680787));
#31759=CARTESIAN_POINT('Ctrl Pts',(-0.225415818250395,-0.00153575670661998,
0.00147605452478166));
#31760=CARTESIAN_POINT('Ctrl Pts',(-0.225383839889912,-0.00153973931552829,
0.00139038950423513));
#31761=CARTESIAN_POINT('Ctrl Pts',(-0.225350428018386,-0.00154367377477953,
0.00129873283310492));
#31762=CARTESIAN_POINT('Ctrl Pts',(-0.225333143387235,-0.00154570914944814,
0.00125131699913256));
#31763=CARTESIAN_POINT('Ctrl Pts',(-0.225315474932153,-0.00154772690563975,
0.00120229607496713));
#31764=CARTESIAN_POINT('Ctrl Pts',(-0.22529824089363,-0.00154961912800569,
0.00115406788678273));
#31765=CARTESIAN_POINT('Ctrl Pts',(-0.225282160858165,-0.00155138464586217,
0.00110906909120891));
#31766=CARTESIAN_POINT('Ctrl Pts',(-0.225266459009404,-0.00155304119210587,
0.00106475974768948));
#31767=CARTESIAN_POINT('Ctrl Pts',(-0.225251799978657,-0.0015545307347765,
0.00102308441757244));
#31768=CARTESIAN_POINT('Ctrl Pts',(-0.225221429894213,-0.00155761671893654,
0.000936742877217953));
#31769=CARTESIAN_POINT('Ctrl Pts',(-0.225195537030683,-0.00156003488278947,
0.000861712337668546));
#31770=CARTESIAN_POINT('Ctrl Pts',(-0.225167559666854,-0.00156240338782803,
0.000779963840828957));
#31771=CARTESIAN_POINT('Ctrl Pts',(-0.22515357098494,-0.00156358764034731,
0.000739089592409159));
#31772=CARTESIAN_POINT('Ctrl Pts',(-0.225139061085489,-0.00156475364739107,
0.000696535807052153));
#31773=CARTESIAN_POINT('Ctrl Pts',(-0.225123079429075,-0.00156594368006901,
0.00064931564366595));
#31774=CARTESIAN_POINT('Ctrl Pts',(-0.225107097772661,-0.00156713371274695,
0.000602095480279747));
#31775=CARTESIAN_POINT('Ctrl Pts',(-0.225089643911978,-0.0015683181027373,
0.000550208270623167));
#31776=CARTESIAN_POINT('Ctrl Pts',(-0.225077025803377,-0.00156911396238647,
0.00051259631297856));
#31777=CARTESIAN_POINT('Ctrl Pts',(-0.225064407694775,-0.00156990982203563,
0.000474984355333953));
#31778=CARTESIAN_POINT('Ctrl Pts',(-0.2250566260427,-0.00157036307013134,
0.000451648374351342));
#31779=CARTESIAN_POINT('Ctrl Pts',(-0.225045952903868,-0.00157095070842386,
0.000419612674057864));
#31780=CARTESIAN_POINT('Ctrl Pts',(-0.225035279765036,-0.00157153834671639,
0.000387576973764386));
#31781=CARTESIAN_POINT('Ctrl Pts',(-0.225021714740738,-0.00157223455280892,
0.000346841231436762));
#31782=CARTESIAN_POINT('Ctrl Pts',(-0.225007189961945,-0.0015728802645566,
0.000303151418613095));
#31783=CARTESIAN_POINT('Ctrl Pts',(-0.224978140533459,-0.00157417168231261,
0.000215772181298103));
#31784=CARTESIAN_POINT('Ctrl Pts',(-0.22494525294181,-0.00157531381840194,
0.000116577087333678));
#31785=CARTESIAN_POINT('Ctrl Pts',(-0.224906594466267,-0.00157591540148865,
-2.25483220937621E-7));
#31786=CARTESIAN_POINT('',(-0.229393975477449,0.00581660464796595,-0.0107320544081557));
#31787=CARTESIAN_POINT('Ctrl Pts',(-0.224906594128032,-0.00157591540674423,
-2.27571033939348E-7));
#31788=CARTESIAN_POINT('Ctrl Pts',(-0.224946111868523,-0.00157529870331805,
-0.000118551128803213));
#31789=CARTESIAN_POINT('Ctrl Pts',(-0.224996629368199,-0.0015735663266729,
-0.000269517258642752));
#31790=CARTESIAN_POINT('Ctrl Pts',(-0.225052344323161,-0.00157067899600388,
-0.000435194557733859));
#31791=CARTESIAN_POINT('Ctrl Pts',(-0.225076556525918,-0.00156927633644708,
-0.000507075806777329));
#31792=CARTESIAN_POINT('Ctrl Pts',(-0.225130207366057,-0.0015656398299004,
-0.000664819935409192));
#31793=CARTESIAN_POINT('Ctrl Pts',(-0.225189841162327,-0.00156078991738676,
-0.000837533395631968));
#31794=CARTESIAN_POINT('Ctrl Pts',(-0.22525653713051,-0.00155462574186823,
-0.00102810784797744));
#31795=CARTESIAN_POINT('Ctrl Pts',(-0.225363879872858,-0.00154285643018889,
-0.00132367096100794));
#31796=CARTESIAN_POINT('Ctrl Pts',(-0.225495863486334,-0.0015265971055308,
-0.00166960190534258));
#31797=CARTESIAN_POINT('Ctrl Pts',(-0.225649782636847,-0.00150521381488585,
-0.00204850589559849));
#31798=CARTESIAN_POINT('Ctrl Pts',(-0.225872675355422,-0.00147720345367394,
-0.00254160361791802));
#31799=CARTESIAN_POINT('Ctrl Pts',(-0.226211629687716,-0.00140171665460475,
-0.00320349500780991));
#31800=CARTESIAN_POINT('Ctrl Pts',(-0.22667852249447,-0.00124920977011111,
-0.00397750653063482));
#31801=CARTESIAN_POINT('Ctrl Pts',(-0.227300714792837,-0.000994842482836054,
-0.00483218755095857));
#31802=CARTESIAN_POINT('Ctrl Pts',(-0.227912194052181,-0.000713115698522522,
-0.00552491953200038));
#31803=CARTESIAN_POINT('Ctrl Pts',(-0.228385701343969,-0.000485499178486317,
-0.00599498793797899));
#31804=CARTESIAN_POINT('Ctrl Pts',(-0.22878733542391,-0.000288437462414136,
-0.00636169114342147));
#31805=CARTESIAN_POINT('Ctrl Pts',(-0.229095506495693,-0.000134908177801581,
-0.00662084785225318));
#31806=CARTESIAN_POINT('Ctrl Pts',(-0.22936465511862,5.49838883985097E-7,
-0.00683645790999942));
#31807=CARTESIAN_POINT('Ctrl Pts',(-0.229591473222452,0.000115907254181684,
-0.00701093248054787));
#31808=CARTESIAN_POINT('Ctrl Pts',(-0.229758410587813,0.000201141186053844,
-0.00713536492284351));
#31809=CARTESIAN_POINT('Ctrl Pts',(-0.230084575118053,0.000369860873483232,
-0.00737136885461296));
#31810=CARTESIAN_POINT('Ctrl Pts',(-0.230320772955051,0.000494986606296006,
-0.00753599937709786));
#31811=CARTESIAN_POINT('Ctrl Pts',(-0.230655165569622,0.000682641774099848,
-0.00776837208130201));
#31812=CARTESIAN_POINT('Ctrl Pts',(-0.230862751346926,0.000807699941341247,
-0.00791571647726933));
#31813=CARTESIAN_POINT('Ctrl Pts',(-0.231060043316746,0.000935072905748187,
-0.00805946248585124));
#31814=CARTESIAN_POINT('Ctrl Pts',(-0.231207688046934,0.00103564097302385,
-0.00816957954198867));
#31815=CARTESIAN_POINT('Ctrl Pts',(-0.231430184389937,0.00120414395145074,
-0.00834535138518368));
#31816=CARTESIAN_POINT('Ctrl Pts',(-0.231579649993422,0.0013299767587557,
-0.00847062997824837));
#31817=CARTESIAN_POINT('Ctrl Pts',(-0.231768906738338,0.00152108066299523,
-0.00865138265776975));
#31818=CARTESIAN_POINT('Ctrl Pts',(-0.231885959839634,0.00167553057426468,
-0.0087894024681425));
#31819=CARTESIAN_POINT('Ctrl Pts',(-0.231994956950233,0.00188925368178171,
-0.00896980965249575));
#31820=CARTESIAN_POINT('Ctrl Pts',(-0.232067192729006,0.0021640031232806,
-0.00918668383711871));
#31821=CARTESIAN_POINT('Ctrl Pts',(-0.232024116308641,0.00249499966508092,
-0.00941975370458247));
#31822=CARTESIAN_POINT('Ctrl Pts',(-0.231920307934533,0.00274915188946458,
-0.00958185777628863));
#31823=CARTESIAN_POINT('Ctrl Pts',(-0.23178568627637,0.00300417566545555,
-0.00973340850727868));
#31824=CARTESIAN_POINT('Ctrl Pts',(-0.231668546496582,0.00319162004613365,
-0.00983699860767679));
#31825=CARTESIAN_POINT('Ctrl Pts',(-0.231502360598737,0.00343046561885037,
-0.00996031520102549));
#31826=CARTESIAN_POINT('Ctrl Pts',(-0.231381050326924,0.00358962237924073,
-0.0100368548962065));
#31827=CARTESIAN_POINT('Ctrl Pts',(-0.231220721639087,0.00379124967224796,
-0.0101287847241368));
#31828=CARTESIAN_POINT('Ctrl Pts',(-0.231053491019977,0.00399213949104106,
-0.010214286829562));
#31829=CARTESIAN_POINT('Ctrl Pts',(-0.230834786572646,0.00424485552231371,
-0.0103123580263811));
#31830=CARTESIAN_POINT('Ctrl Pts',(-0.230710779400135,0.00438412063471161,
-0.010362189532424));
#31831=CARTESIAN_POINT('Ctrl Pts',(-0.230536082718158,0.00457821904778256,
-0.0104284136644632));
#31832=CARTESIAN_POINT('Ctrl Pts',(-0.230376741888428,0.00475273926911148,
-0.0104825778295121));
#31833=CARTESIAN_POINT('Ctrl Pts',(-0.230245352068406,0.00489588458011249,
-0.0105243177957444));
#31834=CARTESIAN_POINT('Ctrl Pts',(-0.230120102425176,0.00503177140546183,
-0.0105614595581269));
#31835=CARTESIAN_POINT('Ctrl Pts',(-0.230072497203735,0.00508324860927118,
-0.010574824436958));
#31836=CARTESIAN_POINT('Ctrl Pts',(-0.229969032924836,0.00519505476708446,
-0.0106033757685201));
#31837=CARTESIAN_POINT('Ctrl Pts',(-0.229775084763404,0.00540432824391078,
-0.0106533278777229));
#31838=CARTESIAN_POINT('Ctrl Pts',(-0.229558050447209,0.00563880049780806,
-0.0107017175610709));
#31839=CARTESIAN_POINT('Ctrl Pts',(-0.229393975477449,0.00581660464796576,
-0.0107320544081557));
#31840=CARTESIAN_POINT('',(-0.228121493224293,0.00414974478032743,-0.0102148629362556));
#31841=CARTESIAN_POINT('Ctrl Pts',(-0.229393975477449,0.00581660464796602,
-0.0107320544081557));
#31842=CARTESIAN_POINT('Ctrl Pts',(-0.229260858960321,0.00565614753223228,
-0.01069838602159));
#31843=CARTESIAN_POINT('Ctrl Pts',(-0.229132855290044,0.00549873829411337,
-0.0106607741833732));
#31844=CARTESIAN_POINT('Ctrl Pts',(-0.229015768989325,0.00535237650556446,
-0.0106221138981469));
#31845=CARTESIAN_POINT('Ctrl Pts',(-0.228898682688606,0.00520601471701555,
-0.0105834536129206));
#31846=CARTESIAN_POINT('Ctrl Pts',(-0.228792501999893,0.00507058293729866,
-0.0105442720151909));
#31847=CARTESIAN_POINT('Ctrl Pts',(-0.228679848627723,0.00492249068197044,
-0.0104974436642677));
#31848=CARTESIAN_POINT('Ctrl Pts',(-0.228567195255553,0.00477439842664221,
-0.0104506153133446));
#31849=CARTESIAN_POINT('Ctrl Pts',(-0.228448084803687,0.00461386570734565,
-0.0103954316370884));
#31850=CARTESIAN_POINT('Ctrl Pts',(-0.228337596129134,0.0044593359696114,
-0.0103374414505981));
#31851=CARTESIAN_POINT('Ctrl Pts',(-0.228282351791858,0.00438207110074427,
-0.010308446357353));
#31852=CARTESIAN_POINT('Ctrl Pts',(-0.228229261601845,0.00430627978839228,
-0.0102788100670567));
#31853=CARTESIAN_POINT('Ctrl Pts',(-0.228179294360642,0.00423396073728532,
-0.0102494906607338));
#31854=CARTESIAN_POINT('Ctrl Pts',(-0.228159733383576,0.0042056495624831,
-0.0102380128160331));
#31855=CARTESIAN_POINT('Ctrl Pts',(-0.228140650513694,0.00417786961955901,
-0.0102265896495175));
#31856=CARTESIAN_POINT('Ctrl Pts',(-0.228121493224293,0.00414974478032743,
-0.0102148629362556));
#31857=CARTESIAN_POINT('',(-0.227485893353239,0.00309654395920274,-0.00969559727848083));
#31858=CARTESIAN_POINT('Ctrl Pts',(-0.228121493224293,0.00414974478032743,
-0.0102148629362556));
#31859=CARTESIAN_POINT('Ctrl Pts',(-0.228091714466324,0.00410602655052453,
-0.0101966345246728));
#31860=CARTESIAN_POINT('Ctrl Pts',(-0.228061755890881,0.00406146956532859,
-0.0101776840835163));
#31861=CARTESIAN_POINT('Ctrl Pts',(-0.228029542246017,0.00401285950391605,
-0.010156492775014));
#31862=CARTESIAN_POINT('Ctrl Pts',(-0.227976604898777,0.00393297758706865,
-0.0101216686605307));
#31863=CARTESIAN_POINT('Ctrl Pts',(-0.227917584474054,0.00384224359990983,
-0.0100805623915113));
#31864=CARTESIAN_POINT('Ctrl Pts',(-0.227864344213728,0.00375821752094305,
-0.0100408730610387));
#31865=CARTESIAN_POINT('Ctrl Pts',(-0.227811103953402,0.00367419144197628,
-0.0100011837305661));
#31866=CARTESIAN_POINT('Ctrl Pts',(-0.227763638776,0.00359676247856459,
-0.00996314948809607));
#31867=CARTESIAN_POINT('Ctrl Pts',(-0.227718266368965,0.00352005373481683,
-0.00992422989423481));
#31868=CARTESIAN_POINT('Ctrl Pts',(-0.227672893961929,0.00344334499106908,
-0.00988531030037355));
#31869=CARTESIAN_POINT('Ctrl Pts',(-0.227629616652783,0.00336741097886024,
-0.00984539544653163));
#31870=CARTESIAN_POINT('Ctrl Pts',(-0.227591308711727,0.00329798459064695,
-0.00980781213905574));
#31871=CARTESIAN_POINT('Ctrl Pts',(-0.227553856941985,0.00323010986196881,
-0.00977106880754444));
#31872=CARTESIAN_POINT('Ctrl Pts',(-0.227521150813476,0.00316835468101453,
-0.00973674788899397));
#31873=CARTESIAN_POINT('Ctrl Pts',(-0.227485893353239,0.00309654395920274,
-0.00969559727848083));
#31874=CARTESIAN_POINT('',(-0.227126281777643,0.00216860537756898,-0.00908887068682453));
#31875=CARTESIAN_POINT('Ctrl Pts',(-0.227485893353239,0.00309654395920274,
-0.00969559727848083));
#31876=CARTESIAN_POINT('Ctrl Pts',(-0.227485087345238,0.00309490218844343,
-0.00969465677495352));
#31877=CARTESIAN_POINT('Ctrl Pts',(-0.227484280003889,0.0030932552914689,
-0.00969371248168514));
#31878=CARTESIAN_POINT('Ctrl Pts',(-0.227483471242014,0.00309160294606555,
-0.00969276450874163));
#31879=CARTESIAN_POINT('Ctrl Pts',(-0.227447284556303,0.00301767153853937,
-0.00965034905863751));
#31880=CARTESIAN_POINT('Ctrl Pts',(-0.227408261758414,0.00293304001203312,
-0.00960019540130323));
#31881=CARTESIAN_POINT('Ctrl Pts',(-0.227376939924427,0.00285973054341183,
-0.0095553277649556));
#31882=CARTESIAN_POINT('Ctrl Pts',(-0.227361279007434,0.00282307580910118,
-0.00953289394678179));
#31883=CARTESIAN_POINT('Ctrl Pts',(-0.227347541293956,0.00278919165650028,
-0.00951188095760037));
#31884=CARTESIAN_POINT('Ctrl Pts',(-0.227331697400134,0.00274851693980081,
-0.00948621499946682));
#31885=CARTESIAN_POINT('Ctrl Pts',(-0.227315853506312,0.00270784222310134,
-0.00946054904133327));
#31886=CARTESIAN_POINT('Ctrl Pts',(-0.227297906689983,0.0026604761335986,
-0.00943007037660862));
#31887=CARTESIAN_POINT('Ctrl Pts',(-0.22728557185282,0.0026273161128947,
-0.00940842406727091));
#31888=CARTESIAN_POINT('Ctrl Pts',(-0.227273237015657,0.00259415609219081,
-0.00938677775793319));
#31889=CARTESIAN_POINT('Ctrl Pts',(-0.227266510364656,0.00257508000662186,
-0.00937415162267746));
#31890=CARTESIAN_POINT('Ctrl Pts',(-0.227256761271677,0.00254726774721839,
-0.0093555911838289));
#31891=CARTESIAN_POINT('Ctrl Pts',(-0.227247012178699,0.00251945548781492,
-0.00933703074498034));
#31892=CARTESIAN_POINT('Ctrl Pts',(-0.22723424257423,0.0024829710433869,
-0.00931243989623622));
#31893=CARTESIAN_POINT('Ctrl Pts',(-0.227220609376841,0.00244362879544726,
-0.00928540540934555));
#31894=CARTESIAN_POINT('Ctrl Pts',(-0.227193343013809,0.00236494439117793,
-0.00923133649851507));
#31895=CARTESIAN_POINT('Ctrl Pts',(-0.227162618503677,0.00227469484764093,
-0.00916768385327356));
#31896=CARTESIAN_POINT('Ctrl Pts',(-0.227126281773003,0.00216860010539621,
-0.00908887778676522));
#31897=CARTESIAN_POINT('',(-0.226399236752868,0.00218270468350247,-0.00908497199103554));
#31898=CARTESIAN_POINT('Ctrl Pts',(-0.226399237323331,0.00218270481409039,
-0.00908497209528306));
#31899=CARTESIAN_POINT('Ctrl Pts',(-0.226402015621168,0.00218242237783528,
-0.00908481942012229));
#31900=CARTESIAN_POINT('Ctrl Pts',(-0.226426871610067,0.0021791724381742,
-0.00908292829527202));
#31901=CARTESIAN_POINT('Ctrl Pts',(-0.226650682773869,0.00216138573969967,
-0.00907425334358046));
#31902=CARTESIAN_POINT('Ctrl Pts',(-0.226703737969127,0.0021601993779741,
-0.00907442059635822));
#31903=CARTESIAN_POINT('Ctrl Pts',(-0.2268930731039,0.00216094231513602,
-0.00907868413393107));
#31904=CARTESIAN_POINT('Ctrl Pts',(-0.226966948755117,0.00216362473656388,
-0.00908207388280154));
#31905=CARTESIAN_POINT('Ctrl Pts',(-0.22707003478252,0.00216671281664232,
-0.00908640974873301));
#31906=CARTESIAN_POINT('Ctrl Pts',(-0.227126282004474,0.00216861511471869,
-0.00908885732195361));
#31907=CARTESIAN_POINT('',(-0.22652065327516,0.00174024863118734,-0.00874177656924924));
#31908=CARTESIAN_POINT('Origin',(-0.228263370666261,0.00775028046455406,
-0.00208932932211252));
#31909=CARTESIAN_POINT('',(-0.225316604397604,0.00173833991161196,-0.00871757580529813));
#31910=CARTESIAN_POINT('',(-0.225316604396809,0.00173833991161069,-0.00871757580528216));
#31911=CARTESIAN_POINT('',(-0.225202513398594,0.00215390640396955,-0.00904067530421461));
#31912=CARTESIAN_POINT('Origin',(-0.226677373856487,0.00780210962717219,
-0.00184344636966992));
#31913=CARTESIAN_POINT('',(-0.224906358055501,0.00215779401747845,-0.00903767194051428));
#31914=CARTESIAN_POINT('Ctrl Pts',(-0.224906358055501,0.00215779401747845,
-0.00903767194051428));
#31915=CARTESIAN_POINT('Ctrl Pts',(-0.224965738450647,0.00215287276425,
-0.00903547806035347));
#31916=CARTESIAN_POINT('Ctrl Pts',(-0.225032844119037,0.00215141623484859,
-0.00903399244325265));
#31917=CARTESIAN_POINT('Ctrl Pts',(-0.225088313767917,0.00215087702492171,
-0.00903517782487992));
#31918=CARTESIAN_POINT('Ctrl Pts',(-0.225147134576941,0.00215030523900321,
-0.00903643482051134));
#31919=CARTESIAN_POINT('Ctrl Pts',(-0.225192860176731,0.0021516122887076,
-0.0090388265130241));
#31920=CARTESIAN_POINT('Ctrl Pts',(-0.225202513203785,0.00215390610473247,
-0.00904067508301585));
#31921=CARTESIAN_POINT('',(-0.224895681452505,0.00215874544783754,-0.00903810107358197));
#31922=CARTESIAN_POINT('Ctrl Pts',(-0.224895681757744,0.00215874503503595,
-0.00903810076696465));
#31923=CARTESIAN_POINT('Ctrl Pts',(-0.224899208684984,0.00215842069526572,
-0.00903796212742679));
#31924=CARTESIAN_POINT('Ctrl Pts',(-0.224902768068525,0.00215810962985243,
-0.00903782571768279));
#31925=CARTESIAN_POINT('Ctrl Pts',(-0.224906358055501,0.00215779401747845,
-0.00903767194051428));
#31926=CARTESIAN_POINT('',(-0.224918679572961,0.00225276421039843,-0.00910663697272384));
#31927=CARTESIAN_POINT('Ctrl Pts',(-0.224918679572961,0.00225276421039843,
-0.00910663697272384));
#31928=CARTESIAN_POINT('Ctrl Pts',(-0.224910263452399,0.00221796952208274,
-0.00908158964469767));
#31929=CARTESIAN_POINT('Ctrl Pts',(-0.224903043299005,0.00218876974680351,
-0.0090602399920936));
#31930=CARTESIAN_POINT('Ctrl Pts',(-0.224895680110049,0.00215877571930383,
-0.00903806209673358));
#31931=CARTESIAN_POINT('',(-0.22502122058335,0.00297339373605577,-0.00957419677215159));
#31932=CARTESIAN_POINT('Ctrl Pts',(-0.225021220587936,0.00297339370675859,
-0.00957419675522714));
#31933=CARTESIAN_POINT('Ctrl Pts',(-0.225018822681216,0.00292404131059288,
-0.00954547825756419));
#31934=CARTESIAN_POINT('Ctrl Pts',(-0.225015786101244,0.00284658987129514,
-0.00949966911370489));
#31935=CARTESIAN_POINT('Ctrl Pts',(-0.225008834761646,0.00276240820049218,
-0.00944752370527374));
#31936=CARTESIAN_POINT('Ctrl Pts',(-0.225005359091848,0.00272031736509071,
-0.00942145100105817));
#31937=CARTESIAN_POINT('Ctrl Pts',(-0.225000905055243,0.00267655359290298,
-0.00939377841014082));
#31938=CARTESIAN_POINT('Ctrl Pts',(-0.224996511017835,0.00264085188948549,
-0.00937084674685504));
#31939=CARTESIAN_POINT('Ctrl Pts',(-0.224992116980427,0.00260515018606799,
-0.00934791508356925));
#31940=CARTESIAN_POINT('Ctrl Pts',(-0.224987781650824,0.00257746907246234,
-0.00932978843303144));
#31941=CARTESIAN_POINT('Ctrl Pts',(-0.22498421438809,0.00255588184289646,
-0.00931556310125919));
#31942=CARTESIAN_POINT('Ctrl Pts',(-0.224982430756723,0.00254508822811351,
-0.00930845043537307));
#31943=CARTESIAN_POINT('Ctrl Pts',(-0.224980838910431,0.00253581068869719,
-0.00930232458184892));
#31944=CARTESIAN_POINT('Ctrl Pts',(-0.224977703366424,0.00251896760981262,
-0.00929110098797916));
#31945=CARTESIAN_POINT('Ctrl Pts',(-0.224974567822417,0.00250212453092805,
-0.00927987739410941));
#31946=CARTESIAN_POINT('Ctrl Pts',(-0.22496988938007,0.00247774239373384,
-0.00926351615899424));
#31947=CARTESIAN_POINT('Ctrl Pts',(-0.224965165668848,0.00245478699071914,
-0.00924792855998076));
#31948=CARTESIAN_POINT('Ctrl Pts',(-0.224960441957625,0.00243183158770443,
-0.00923234096096728));
#31949=CARTESIAN_POINT('Ctrl Pts',(-0.224955672693692,0.00241029291869914,
-0.00921754133956075));
#31950=CARTESIAN_POINT('Ctrl Pts',(-0.22495211515215,0.00239447540665665,
-0.0092066089723048));
#31951=CARTESIAN_POINT('Ctrl Pts',(-0.224948557610609,0.00237865789461416,
-0.00919567660504884));
#31952=CARTESIAN_POINT('Ctrl Pts',(-0.224946211283118,0.00236854422866547,
-0.00918863700259461));
#31953=CARTESIAN_POINT('Ctrl Pts',(-0.224943044205686,0.0023550400623941,
-0.00917919588349946));
#31954=CARTESIAN_POINT('Ctrl Pts',(-0.224936710050824,0.00232803172985139,
-0.00916031364530917));
#31955=CARTESIAN_POINT('Ctrl Pts',(-0.224927095693523,0.00228755889871412,
-0.00913168430075001));
#31956=CARTESIAN_POINT('Ctrl Pts',(-0.224918679572961,0.00225276421039843,
-0.00910663697272384));
#31957=CARTESIAN_POINT('',(-0.224873561887543,0.00458479712506902,-0.0103057155136081));
#31958=CARTESIAN_POINT('Ctrl Pts',(-0.22502122058335,0.00297339373605577,
-0.00957419677215159));
#31959=CARTESIAN_POINT('Ctrl Pts',(-0.224994800587243,0.00312706788500571,
-0.00966292275481428));
#31960=CARTESIAN_POINT('Ctrl Pts',(-0.224971751786512,0.00328898460622665,
-0.00975067902641553));
#31961=CARTESIAN_POINT('Ctrl Pts',(-0.224951688553439,0.00346762396572364,
-0.00983967477566947));
#31962=CARTESIAN_POINT('Ctrl Pts',(-0.224931625320365,0.00364626332522062,
-0.00992867052492342));
#31963=CARTESIAN_POINT('Ctrl Pts',(-0.22491456271264,0.00384201360972133,
-0.0100181849127952));
#31964=CARTESIAN_POINT('Ctrl Pts',(-0.22490161244035,0.00403033493817414,
-0.0100964406799755));
#31965=CARTESIAN_POINT('Ctrl Pts',(-0.22489853339978,0.00407510998209125,
-0.010115046673471));
#31966=CARTESIAN_POINT('Ctrl Pts',(-0.224895685788583,0.00411945175020758,
-0.0101330494887832));
#31967=CARTESIAN_POINT('Ctrl Pts',(-0.224893049692661,0.00416352534378688,
-0.0101505428737757));
#31968=CARTESIAN_POINT('Ctrl Pts',(-0.224884598516693,0.00430482281780293,
-0.0102066256868774));
#31969=CARTESIAN_POINT('Ctrl Pts',(-0.224878321311043,0.00444332778718251,
-0.0102575634943944));
#31970=CARTESIAN_POINT('Ctrl Pts',(-0.224873561887543,0.00458479712506902,
-0.0103057155136081));
#31971=CARTESIAN_POINT('',(-0.224989661033144,0.00750493775356048,-0.010792594548104));
#31972=CARTESIAN_POINT('Ctrl Pts',(-0.224873561887543,0.00458479712506902,
-0.0103057155136081));
#31973=CARTESIAN_POINT('Ctrl Pts',(-0.224867317901785,0.00477039366441729,
-0.0103688871397866));
#31974=CARTESIAN_POINT('Ctrl Pts',(-0.224863695490022,0.00496116495721837,
-0.0104269636390426));
#31975=CARTESIAN_POINT('Ctrl Pts',(-0.224863318658598,0.00515133401433211,
-0.0104781654954328));
#31976=CARTESIAN_POINT('Ctrl Pts',(-0.224862941827173,0.00534150307144586,
-0.010529367351823));
#31977=CARTESIAN_POINT('Ctrl Pts',(-0.224865806202762,0.00553104234508341,
-0.0105738883450165));
#31978=CARTESIAN_POINT('Ctrl Pts',(-0.224871561595658,0.00572270826827539,
-0.0106125334130875));
#31979=CARTESIAN_POINT('Ctrl Pts',(-0.224874439292107,0.00581854122987138,
-0.010631855947123));
#31980=CARTESIAN_POINT('Ctrl Pts',(-0.224878038558442,0.00591488770775002,
-0.010649763323073));
#31981=CARTESIAN_POINT('Ctrl Pts',(-0.224882845453478,0.00601827962750455,
-0.0106671096183221));
#31982=CARTESIAN_POINT('Ctrl Pts',(-0.224887652348514,0.00612167154725909,
-0.0106844559135711));
#31983=CARTESIAN_POINT('Ctrl Pts',(-0.224893675898609,0.00623218238819598,
-0.010700838010295));
#31984=CARTESIAN_POINT('Ctrl Pts',(-0.224898904237491,0.00632012556458434,
-0.0107125924563936));
#31985=CARTESIAN_POINT('Ctrl Pts',(-0.224904132576373,0.0064080687409727,
-0.0107243469024922));
#31986=CARTESIAN_POINT('Ctrl Pts',(-0.224908551189283,0.00647336006007754,
-0.0107321190251052));
#31987=CARTESIAN_POINT('Ctrl Pts',(-0.224914213769459,0.00655341180453011,
-0.0107407320671868));
#31988=CARTESIAN_POINT('Ctrl Pts',(-0.224919876349636,0.00663346354898268,
-0.0107493451092684));
#31989=CARTESIAN_POINT('Ctrl Pts',(-0.224926791877645,0.00672831496636562,
-0.0107584006712993));
#31990=CARTESIAN_POINT('Ctrl Pts',(-0.22493444307939,0.00682862505175741,
-0.0107661102157719));
#31991=CARTESIAN_POINT('Ctrl Pts',(-0.224949745482882,0.00702924522254099,
-0.010781529304717));
#31992=CARTESIAN_POINT('Ctrl Pts',(-0.224967975196583,0.00725167285755061,
-0.0107922449054418));
#31993=CARTESIAN_POINT('Ctrl Pts',(-0.224989661033144,0.00750493775356048,
-0.010792594548104));
#31994=CARTESIAN_POINT('',(-0.224861052242961,0.00980960902579858,-0.0104885393712655));
#31995=CARTESIAN_POINT('Ctrl Pts',(-0.224989619839449,0.00750541590997777,
-0.0107925933390392));
#31996=CARTESIAN_POINT('Ctrl Pts',(-0.224968308830846,0.00775278936281719,
-0.0107919616726235));
#31997=CARTESIAN_POINT('Ctrl Pts',(-0.224950341443786,0.00797012061575864,
-0.0107814799560685));
#31998=CARTESIAN_POINT('Ctrl Pts',(-0.224935172802778,0.00816640892122435,
-0.0107664984290652));
#31999=CARTESIAN_POINT('Ctrl Pts',(-0.224927583595994,0.00826461630437055,
-0.0107590028395596));
#32000=CARTESIAN_POINT('Ctrl Pts',(-0.224920698710054,0.00835754960891373,
-0.0107502157304149));
#32001=CARTESIAN_POINT('Ctrl Pts',(-0.224915052876814,0.00843590726060768,
-0.010741876735001));
#32002=CARTESIAN_POINT('Ctrl Pts',(-0.224909407043574,0.00851426491230164,
-0.0107335377395871));
#32003=CARTESIAN_POINT('Ctrl Pts',(-0.224904991495846,0.00857808469234472,
-0.0107260357632222));
#32004=CARTESIAN_POINT('Ctrl Pts',(-0.22489968241033,0.00866461685109938,
-0.0107146156992334));
#32005=CARTESIAN_POINT('Ctrl Pts',(-0.224894373324813,0.00875114900985405,
-0.0107031956352445));
#32006=CARTESIAN_POINT('Ctrl Pts',(-0.224888185038604,0.00886031180744275,
-0.0106872201606962));
#32007=CARTESIAN_POINT('Ctrl Pts',(-0.224883184114701,0.00896206883700661,
-0.0106703715492553));
#32008=CARTESIAN_POINT('Ctrl Pts',(-0.224878183190799,0.00906382586657046,
-0.0106535229378145));
#32009=CARTESIAN_POINT('Ctrl Pts',(-0.224874360588758,0.00915824882136895,
-0.0106362047479502));
#32010=CARTESIAN_POINT('Ctrl Pts',(-0.224871246701787,0.00925206036384027,
-0.0106175595945488));
#32011=CARTESIAN_POINT('Ctrl Pts',(-0.224865018927847,0.00943968344878292,
-0.010580269287746));
#32012=CARTESIAN_POINT('Ctrl Pts',(-0.224861631620231,0.00962479695162405,
-0.010537419086996));
#32013=CARTESIAN_POINT('Ctrl Pts',(-0.224861054524101,0.00980887667976263,
-0.0104887330969168));
#32014=CARTESIAN_POINT('',(-0.225003674467847,0.0119594514142438,-0.00961246062240638));
#32015=CARTESIAN_POINT('Ctrl Pts',(-0.224861052242961,0.00980960902579858,
-0.0104885393712655));
#32016=CARTESIAN_POINT('Ctrl Pts',(-0.224859994130178,0.0101515267552638,
-0.0103980785545349));
#32017=CARTESIAN_POINT('Ctrl Pts',(-0.22486861966081,0.0104899749483281,
-0.0102879912445166));
#32018=CARTESIAN_POINT('Ctrl Pts',(-0.224888950367126,0.0108364571580695,
-0.0101504612032825));
#32019=CARTESIAN_POINT('Ctrl Pts',(-0.224890495888814,0.0108627964185675,
-0.0101400062954098));
#32020=CARTESIAN_POINT('Ctrl Pts',(-0.224892109053557,0.0108891803588371,
-0.0101293892361149));
#32021=CARTESIAN_POINT('Ctrl Pts',(-0.224893790749427,0.01091561328614,
-0.0101186052814899));
#32022=CARTESIAN_POINT('Ctrl Pts',(-0.22490570050544,0.0111028110550533,
-0.0100422334055061));
#32023=CARTESIAN_POINT('Ctrl Pts',(-0.224921059623722,0.0112923339255128,
-0.00995711388322306));
#32024=CARTESIAN_POINT('Ctrl Pts',(-0.224939425953085,0.0114679404137457,
-0.0098713483279965));
#32025=CARTESIAN_POINT('Ctrl Pts',(-0.224957792282447,0.0116435469019786,
-0.00978558277276994));
#32026=CARTESIAN_POINT('Ctrl Pts',(-0.224979156068591,0.0118054886917652,
-0.00969963800962885));
#32027=CARTESIAN_POINT('Ctrl Pts',(-0.225003674449545,0.0119594518698436,
-0.00961246147151369));
#32028=CARTESIAN_POINT('',(-0.22485135503735,0.0128342630404597,-0.00904243198075601));
#32029=CARTESIAN_POINT('Ctrl Pts',(-0.224851353464631,0.0128342017223001,
-0.00904235060666903));
#32030=CARTESIAN_POINT('Ctrl Pts',(-0.22485925916006,0.0128021299727841,
-0.00906601576353804));
#32031=CARTESIAN_POINT('Ctrl Pts',(-0.224867008714604,0.0127708336008954,
-0.00908883359846289));
#32032=CARTESIAN_POINT('Ctrl Pts',(-0.224876088403718,0.0127334705285249,
-0.00911562313894002));
#32033=CARTESIAN_POINT('Ctrl Pts',(-0.224885168862013,0.0126961042909622,
-0.00914241494887834));
#32034=CARTESIAN_POINT('Ctrl Pts',(-0.224895582294414,0.0126525747563171,
-0.00917304599903577));
#32035=CARTESIAN_POINT('Ctrl Pts',(-0.224902470444808,0.0126234398800092,
-0.00919329013210234));
#32036=CARTESIAN_POINT('Ctrl Pts',(-0.224905914520005,0.0126088724418552,
-0.00920341219863562));
#32037=CARTESIAN_POINT('Ctrl Pts',(-0.224908476469182,0.0125979315046998,
-0.00921097808108285));
#32038=CARTESIAN_POINT('Ctrl Pts',(-0.224912358910093,0.0125809508958258,
-0.00922263290293978));
#32039=CARTESIAN_POINT('Ctrl Pts',(-0.224916241351003,0.0125639702869518,
-0.00923428772479671));
#32040=CARTESIAN_POINT('Ctrl Pts',(-0.22492144485436,0.0125409307741997,
-0.00925000290292928));
#32041=CARTESIAN_POINT('Ctrl Pts',(-0.22492671945306,0.0125162396970512,
-0.00926663390298052));
#32042=CARTESIAN_POINT('Ctrl Pts',(-0.224931994051759,0.0124915486199026,
-0.00928326490303176));
#32043=CARTESIAN_POINT('Ctrl Pts',(-0.224937340105205,0.0124651934712332,
-0.00930079361002119));
#32044=CARTESIAN_POINT('Ctrl Pts',(-0.224940932961824,0.0124470857933336,
-0.00931274715591608));
#32045=CARTESIAN_POINT('Ctrl Pts',(-0.224944525818442,0.012428978115434,
-0.00932470070181097));
#32046=CARTESIAN_POINT('Ctrl Pts',(-0.224946364530775,0.0124191489015504,
-0.00933112626801354));
#32047=CARTESIAN_POINT('Ctrl Pts',(-0.224948466183687,0.0124076180730514,
-0.0093386492942931));
#32048=CARTESIAN_POINT('Ctrl Pts',(-0.224952669489511,0.0123845564160533,
-0.00935369534685221));
#32049=CARTESIAN_POINT('Ctrl Pts',(-0.224957925683046,0.0123546528503569,
-0.00937307558661003));
#32050=CARTESIAN_POINT('Ctrl Pts',(-0.22496368028001,0.0123163102277348,
-0.00939742191162186));
#32051=CARTESIAN_POINT('Ctrl Pts',(-0.224969434876974,0.0122779676051128,
-0.0094217682366337));
#32052=CARTESIAN_POINT('Ctrl Pts',(-0.224975689291671,0.0122311411163537,
-0.0094510106343654));
#32053=CARTESIAN_POINT('Ctrl Pts',(-0.224981041882397,0.0121859897564173,
-0.00947859648540025));
#32054=CARTESIAN_POINT('Ctrl Pts',(-0.22499174706385,0.0120956870365444,
-0.00953376818746994));
#32055=CARTESIAN_POINT('Ctrl Pts',(-0.224998843833919,0.0120121173691427,
-0.00958236813765755));
#32056=CARTESIAN_POINT('Ctrl Pts',(-0.225003674451785,0.0119594518981984,
-0.00961246145541169));
#32057=CARTESIAN_POINT('',(-0.225189992040237,0.012835362403236,-0.00904829323284222));
#32058=CARTESIAN_POINT('Ctrl Pts',(-0.225189991984345,0.0128353624762501,
-0.00904829317995413));
#32059=CARTESIAN_POINT('Ctrl Pts',(-0.225177557949143,0.0128382138898305,
-0.00904599628478506));
#32060=CARTESIAN_POINT('Ctrl Pts',(-0.225123424484218,0.0128399799233524,
-0.00904304785851361));
#32061=CARTESIAN_POINT('Ctrl Pts',(-0.225057128079432,0.0128399711268489,
-0.00904126425642094));
#32062=CARTESIAN_POINT('Ctrl Pts',(-0.224990831901919,0.0128399623303756,
-0.00903948066044271));
#32063=CARTESIAN_POINT('Ctrl Pts',(-0.224912370630193,0.0128387738011947,
-0.00904015806168038));
#32064=CARTESIAN_POINT('Ctrl Pts',(-0.224851352869637,0.0128342685710829,
-0.00904242811423944));
#32065=CARTESIAN_POINT('',(-0.225309783756647,0.0132780506578484,-0.00870378498324709));
#32066=CARTESIAN_POINT('Ctrl Pts',(-0.225309747301439,0.0132780497391535,
-0.00870378504917953));
#32067=CARTESIAN_POINT('Ctrl Pts',(-0.225296300432129,0.0132302881562321,
-0.0087433986075426));
#32068=CARTESIAN_POINT('Ctrl Pts',(-0.225278030237819,0.0131658512022134,
-0.00879661521430529));
#32069=CARTESIAN_POINT('Ctrl Pts',(-0.225249280048583,0.0130594725678051,
-0.00887935672594214));
#32070=CARTESIAN_POINT('Ctrl Pts',(-0.225234904953965,0.013006283250601,
-0.00892072748176057));
#32071=CARTESIAN_POINT('Ctrl Pts',(-0.225217916472581,0.0129423241724453,
-0.00896912175258144));
#32072=CARTESIAN_POINT('Ctrl Pts',(-0.225207088659046,0.0129010582597847,
-0.00899977330256321));
#32073=CARTESIAN_POINT('Ctrl Pts',(-0.225196260845511,0.012859792347124,
-0.00903042485254499));
#32074=CARTESIAN_POINT('Ctrl Pts',(-0.225191586980628,0.012841462054515,
-0.00904366530876166));
#32075=CARTESIAN_POINT('Ctrl Pts',(-0.22518999470407,0.0128352773201681,
-0.00904817273968199));
#32076=CARTESIAN_POINT('',(-0.226513610415091,0.0132774514495838,-0.0087268701182885));
#32077=CARTESIAN_POINT('',(-0.226513587963189,0.0132774837566105,-0.00872685128052572));
#32078=CARTESIAN_POINT('',(-0.226387839413824,0.0128159440895836,-0.00908574126323817));
#32079=CARTESIAN_POINT('Origin',(-0.227813772544845,0.00720553420671457,
-0.00186973940970176));
#32080=CARTESIAN_POINT('',(-0.227080811026755,0.0128302386724515,-0.00908882599726657));
#32081=CARTESIAN_POINT('Ctrl Pts',(-0.227080576518632,0.0128308674881957,
-0.00908834620576183));
#32082=CARTESIAN_POINT('Ctrl Pts',(-0.226974397707285,0.012833937009542,
-0.00908410442899972));
#32083=CARTESIAN_POINT('Ctrl Pts',(-0.226856526383581,0.0128356891942227,
-0.00908035969467839));
#32084=CARTESIAN_POINT('Ctrl Pts',(-0.22673763939975,0.0128339634601437,
-0.00907931775934973));
#32085=CARTESIAN_POINT('Ctrl Pts',(-0.226618752415919,0.0128322377260647,
-0.00907827582402107));
#32086=CARTESIAN_POINT('Ctrl Pts',(-0.226498852018804,0.0128269680083964,
-0.00907983666977414));
#32087=CARTESIAN_POINT('Ctrl Pts',(-0.226388621137425,0.012815771215702,
-0.00908588121603269));
#32088=CARTESIAN_POINT('',(-0.229388968164796,0.00914967754123552,-0.0107383249628337));
#32089=CARTESIAN_POINT('Ctrl Pts',(-0.227080816141077,0.0128302296664822,
-0.00908884892398524));
#32090=CARTESIAN_POINT('Ctrl Pts',(-0.227118042045205,0.0127291087233939,
-0.0091639799482189));
#32091=CARTESIAN_POINT('Ctrl Pts',(-0.227166371368342,0.0125968433379446,
-0.009257729975268));
#32092=CARTESIAN_POINT('Ctrl Pts',(-0.227221508256631,0.0124478282471741,
-0.00935830862716436));
#32093=CARTESIAN_POINT('Ctrl Pts',(-0.227246597063904,0.01238023390187,
-0.00940311751157318));
#32094=CARTESIAN_POINT('Ctrl Pts',(-0.227301913293252,0.0122375017599441,
-0.00949488477515939));
#32095=CARTESIAN_POINT('Ctrl Pts',(-0.22736642320277,0.0120811836283352,
-0.00959127878264262));
#32096=CARTESIAN_POINT('Ctrl Pts',(-0.227484064229483,0.0118170422191122,
-0.00974673980499964));
#32097=CARTESIAN_POINT('Ctrl Pts',(-0.227636777896552,0.0115356572943751,
-0.00989754184678776));
#32098=CARTESIAN_POINT('Ctrl Pts',(-0.227828855086766,0.0112221796454634,
-0.0100508460071324));
#32099=CARTESIAN_POINT('Ctrl Pts',(-0.228009339223509,0.0109504965145836,
-0.0101726617716261));
#32100=CARTESIAN_POINT('Ctrl Pts',(-0.228139625684295,0.0107643904939703,
-0.0102501751694497));
#32101=CARTESIAN_POINT('Ctrl Pts',(-0.228304573361481,0.0105360288702207,
-0.0103394978935565));
#32102=CARTESIAN_POINT('Ctrl Pts',(-0.228472261507887,0.0103111456105014,
-0.0104209620829437));
#32103=CARTESIAN_POINT('Ctrl Pts',(-0.228685514219872,0.0100334503409072,
-0.0105116594987286));
#32104=CARTESIAN_POINT('Ctrl Pts',(-0.228804955859185,0.00988138379631196,
-0.010557077979536));
#32105=CARTESIAN_POINT('Ctrl Pts',(-0.229037084164035,0.0095881542493913,
-0.0106396138852661));
#32106=CARTESIAN_POINT('Ctrl Pts',(-0.22923748765341,0.0093381851229799,
-0.0106996220901668));
#32107=CARTESIAN_POINT('Ctrl Pts',(-0.229388968164794,0.00914967754123375,
-0.010738324962834));
#32108=CARTESIAN_POINT('',(-0.224906163263034,0.0165759221188024,-4.45014041372842E-7));
#32109=CARTESIAN_POINT('Ctrl Pts',(-0.229388968164796,0.00914967754123552,
-0.0107383249628337));
#32110=CARTESIAN_POINT('Ctrl Pts',(-0.229564104670247,0.00934079850670889,
-0.010706443305865));
#32111=CARTESIAN_POINT('Ctrl Pts',(-0.229713942021003,0.00950375582513596,
-0.0106729165575947));
#32112=CARTESIAN_POINT('Ctrl Pts',(-0.22983517785877,0.00963556162626185,
-0.0106432950332153));
#32113=CARTESIAN_POINT('Ctrl Pts',(-0.229895795777654,0.00970146452682479,
-0.0106284842710256));
#32114=CARTESIAN_POINT('Ctrl Pts',(-0.229949263009114,0.00975958209528396,
-0.0106146636081862));
#32115=CARTESIAN_POINT('Ctrl Pts',(-0.229998882838972,0.009813654019032,
-0.0106013255935172));
#32116=CARTESIAN_POINT('Ctrl Pts',(-0.230023692753901,0.00984068998090601,
-0.0105946565861827));
#32117=CARTESIAN_POINT('Ctrl Pts',(-0.230047541270744,0.00986670929317547,
-0.0105880878678036));
#32118=CARTESIAN_POINT('Ctrl Pts',(-0.230065885362377,0.00988671999043132,
-0.0105829693501056));
#32119=CARTESIAN_POINT('Ctrl Pts',(-0.23008422945401,0.00990673068768717,
-0.0105778508324077));
#32120=CARTESIAN_POINT('Ctrl Pts',(-0.23009706777556,0.0099207493068319,
-0.010574243222264));
#32121=CARTESIAN_POINT('Ctrl Pts',(-0.230122987907983,0.00994921599646166,
-0.0105667347448726));
#32122=CARTESIAN_POINT('Ctrl Pts',(-0.230148908040407,0.00997768268609141,
-0.0105592262674811));
#32123=CARTESIAN_POINT('Ctrl Pts',(-0.230187912816546,0.0100205614301913,
-0.0105476888864162));
#32124=CARTESIAN_POINT('Ctrl Pts',(-0.230222885609791,0.0100590946893514,
-0.0105369864609402));
#32125=CARTESIAN_POINT('Ctrl Pts',(-0.230257858403037,0.0100976279485115,
-0.0105262840354641));
#32126=CARTESIAN_POINT('Ctrl Pts',(-0.230288797031605,0.0101318456076922,
-0.0105165154836512));
#32127=CARTESIAN_POINT('Ctrl Pts',(-0.230319797319392,0.0101662100052759,
-0.0105064944662422));
#32128=CARTESIAN_POINT('Ctrl Pts',(-0.230381797894966,0.0102349388004433,
-0.010486452431424));
#32129=CARTESIAN_POINT('Ctrl Pts',(-0.2304440470754,0.0103042237496369,
-0.0104653107292336));
#32130=CARTESIAN_POINT('Ctrl Pts',(-0.230504662761974,0.0103721813001915,
-0.0104436457352738));
#32131=CARTESIAN_POINT('Ctrl Pts',(-0.230565278448548,0.0104401388507461,
-0.0104219807413139));
#32132=CARTESIAN_POINT('Ctrl Pts',(-0.230624261164103,0.0105067646109838,
-0.010399769209469));
#32133=CARTESIAN_POINT('Ctrl Pts',(-0.23067758423573,0.0105672084133487,
-0.0103788991236485));
#32134=CARTESIAN_POINT('Ctrl Pts',(-0.230730907307356,0.0106276522157137,
-0.0103580290378279));
#32135=CARTESIAN_POINT('Ctrl Pts',(-0.230778566444075,0.0106819821383055,
-0.0103386963744288));
#32136=CARTESIAN_POINT('Ctrl Pts',(-0.230838561740658,0.0107513942951081,
-0.0103129298682109));
#32137=CARTESIAN_POINT('Ctrl Pts',(-0.230868153891086,0.0107856312287117,
-0.010300220766474));
#32138=CARTESIAN_POINT('Ctrl Pts',(-0.230900749272715,0.0108235170458618,
-0.0102858937333083));
#32139=CARTESIAN_POINT('Ctrl Pts',(-0.230933926070351,0.0108622600474418,
-0.0102708948460321));
#32140=CARTESIAN_POINT('Ctrl Pts',(-0.230968012103738,0.0109020648308885,
-0.0102554849026716));
#32141=CARTESIAN_POINT('Ctrl Pts',(-0.231002711858128,0.0109427731882278,
-0.0102393637094851));
#32142=CARTESIAN_POINT('Ctrl Pts',(-0.231035398896431,0.0109814222351681,
-0.0102237263817688));
#32143=CARTESIAN_POINT('Ctrl Pts',(-0.231099901055102,0.0110576893761418,
-0.010192868847837));
#32144=CARTESIAN_POINT('Ctrl Pts',(-0.231156559478863,0.0111259983585293,
-0.0101640205438184));
#32145=CARTESIAN_POINT('Ctrl Pts',(-0.231211835149342,0.0111940704020128,
-0.0101342874093605));
#32146=CARTESIAN_POINT('Ctrl Pts',(-0.231267110819821,0.0112621424454963,
-0.0101045542749026));
#32147=CARTESIAN_POINT('Ctrl Pts',(-0.23132100653357,0.0113299180323245,
-0.010073805833687));
#32148=CARTESIAN_POINT('Ctrl Pts',(-0.23136787049939,0.011389691696947,
-0.0100458771804067));
#32149=CARTESIAN_POINT('Ctrl Pts',(-0.231414734465211,0.0114494653615695,
-0.0100179485271265));
#32150=CARTESIAN_POINT('Ctrl Pts',(-0.231454561628712,0.0115013491391876,
-0.00999307644786312));
#32151=CARTESIAN_POINT('Ctrl Pts',(-0.231503504946577,0.0115686589515727,
-0.00995964927974371));
#32152=CARTESIAN_POINT('Ctrl Pts',(-0.231552448264441,0.0116359687639579,
-0.0099262221116243));
#32153=CARTESIAN_POINT('Ctrl Pts',(-0.23161051693924,0.0117184863969086,
-0.00988380564676722));
#32154=CARTESIAN_POINT('Ctrl Pts',(-0.231658296470953,0.0117892053597625,
-0.00984606356092155));
#32155=CARTESIAN_POINT('Ctrl Pts',(-0.231706076002667,0.0118599243226163,
-0.00980832147507588));
#32156=CARTESIAN_POINT('Ctrl Pts',(-0.231743556658961,0.0119190988785855,
-0.00977571832815352));
#32157=CARTESIAN_POINT('Ctrl Pts',(-0.231784756299534,0.0119911418525335,
-0.00973463888789059));
#32158=CARTESIAN_POINT('Ctrl Pts',(-0.231825955940108,0.0120631848264815,
-0.00969355944762766));
#32159=CARTESIAN_POINT('Ctrl Pts',(-0.231870883582506,0.0121478440626175,
-0.00964356931092481));
#32160=CARTESIAN_POINT('Ctrl Pts',(-0.231906811484744,0.0122229265082499,
-0.00959750935911378));
#32161=CARTESIAN_POINT('Ctrl Pts',(-0.231942739386982,0.0122980089538823,
-0.00955144940730275));
#32162=CARTESIAN_POINT('Ctrl Pts',(-0.231969660030808,0.0123637434774996,
-0.00950968646531456));
#32163=CARTESIAN_POINT('Ctrl Pts',(-0.231991468015951,0.0124353497128256,
-0.00946264718223883));
#32164=CARTESIAN_POINT('Ctrl Pts',(-0.232035083986235,0.0125785621834778,
-0.00936856861608737));
#32165=CARTESIAN_POINT('Ctrl Pts',(-0.23205827808065,0.0127443218159472,
-0.0092519649420025));
#32166=CARTESIAN_POINT('Ctrl Pts',(-0.232043483449447,0.0128903437766426,
-0.0091412056146135));
#32167=CARTESIAN_POINT('Ctrl Pts',(-0.232036086133846,0.0129633547569904,
-0.009085825950919));
#32168=CARTESIAN_POINT('Ctrl Pts',(-0.232019186068209,0.0130316500789959,
-0.0090321924318841));
#32169=CARTESIAN_POINT('Ctrl Pts',(-0.231991634815625,0.0131027443802735,
-0.00897444119022315));
#32170=CARTESIAN_POINT('Ctrl Pts',(-0.23196408356304,0.0131738386815511,
-0.0089166899485622));
#32171=CARTESIAN_POINT('Ctrl Pts',(-0.231925885937843,0.0132475287214381,
-0.00885457037433584));
#32172=CARTESIAN_POINT('Ctrl Pts',(-0.231889750347582,0.013306209782967,
-0.00880373558487667));
#32173=CARTESIAN_POINT('Ctrl Pts',(-0.23185361475732,0.0133648908444959,
-0.00875290079541749));
#32174=CARTESIAN_POINT('Ctrl Pts',(-0.231819535158648,0.0134088405277549,
-0.00871367215862119));
#32175=CARTESIAN_POINT('Ctrl Pts',(-0.231777056882382,0.013458357573902,
-0.00866858901449053));
#32176=CARTESIAN_POINT('Ctrl Pts',(-0.231734578606116,0.0135078746200491,
-0.00862350587035986));
#32177=CARTESIAN_POINT('Ctrl Pts',(-0.231683705298113,0.0135627803727237,
-0.00857237091817839));
#32178=CARTESIAN_POINT('Ctrl Pts',(-0.231628986423714,0.0136163616562068,
-0.00852107800022125));
#32179=CARTESIAN_POINT('Ctrl Pts',(-0.231590792768567,0.013653761275373,
-0.00848527565520792));
#32180=CARTESIAN_POINT('Ctrl Pts',(-0.231550724619769,0.0136905495698959,
-0.00844943454284152));
#32181=CARTESIAN_POINT('Ctrl Pts',(-0.231506147015012,0.0137288292478143,
-0.00841142376562983));
#32182=CARTESIAN_POINT('Ctrl Pts',(-0.231486859657217,0.0137453916864714,
-0.00839497767203373));
#32183=CARTESIAN_POINT('Ctrl Pts',(-0.231466728117272,0.0137622314440902,
-0.00837812360215855));
#32184=CARTESIAN_POINT('Ctrl Pts',(-0.23144553897158,0.0137795097865656,
-0.00836068050978691));
#32185=CARTESIAN_POINT('Ctrl Pts',(-0.231375376743527,0.0138367224284889,
-0.00830292234234003));
#32186=CARTESIAN_POINT('Ctrl Pts',(-0.231293622555022,0.0138985813194139,
-0.00823853409137215));
#32187=CARTESIAN_POINT('Ctrl Pts',(-0.231226714525978,0.013947040708293,
-0.0081868881426923));
#32188=CARTESIAN_POINT('Ctrl Pts',(-0.231159806496934,0.0139955000971721,
-0.00813524219401245));
#32189=CARTESIAN_POINT('Ctrl Pts',(-0.231107739434246,0.0140308717053663,
-0.00809663782142736));
#32190=CARTESIAN_POINT('Ctrl Pts',(-0.231041587164618,0.0140742389559795,
-0.00804842920666416));
#32191=CARTESIAN_POINT('Ctrl Pts',(-0.23097543489499,0.0141176062065926,
-0.00800022059190097));
#32192=CARTESIAN_POINT('Ctrl Pts',(-0.230895202143996,0.0141686670137287,
-0.00794212927864545));
#32193=CARTESIAN_POINT('Ctrl Pts',(-0.230830248345273,0.0142088152135737,
-0.007895472402854));
#32194=CARTESIAN_POINT('Ctrl Pts',(-0.230765294546549,0.0142489634134188,
-0.00784881552706254));
#32195=CARTESIAN_POINT('Ctrl Pts',(-0.230715615487131,0.014278491958761,
-0.00781384935289027));
#32196=CARTESIAN_POINT('Ctrl Pts',(-0.2306479977017,0.0143177721079901,
-0.0077664766629716));
#32197=CARTESIAN_POINT('Ctrl Pts',(-0.230580379916268,0.0143570522572192,
-0.00771910397305294));
#32198=CARTESIAN_POINT('Ctrl Pts',(-0.230494827219163,0.0144058030335849,
-0.00765908731777351));
#32199=CARTESIAN_POINT('Ctrl Pts',(-0.230419563342902,0.0144478003300146,
-0.0076061272432004));
#32200=CARTESIAN_POINT('Ctrl Pts',(-0.23034429946664,0.0144897976264443,
-0.0075531671686273));
#32201=CARTESIAN_POINT('Ctrl Pts',(-0.23027932188938,0.0145252487348904,
-0.00750742818708478));
#32202=CARTESIAN_POINT('Ctrl Pts',(-0.230211958684545,0.0145614671965424,
-0.00745988023620919));
#32203=CARTESIAN_POINT('Ctrl Pts',(-0.230144595479711,0.0145976856581944,
-0.0074123322853336));
#32204=CARTESIAN_POINT('Ctrl Pts',(-0.23007484731461,0.0146346073714077,
-0.00736292855388468));
#32205=CARTESIAN_POINT('Ctrl Pts',(-0.23000379887155,0.0146717813647277,
-0.00731212793154391));
#32206=CARTESIAN_POINT('Ctrl Pts',(-0.229932750428491,0.0147089553580477,
-0.00726132730920313));
#32207=CARTESIAN_POINT('Ctrl Pts',(-0.22986040194103,0.014746365348263,
-0.00720911560519303));
#32208=CARTESIAN_POINT('Ctrl Pts',(-0.229791588342911,0.0147817912340649,
-0.00715866362205958));
#32209=CARTESIAN_POINT('Ctrl Pts',(-0.229722774744791,0.0148172171198668,
-0.00710821163892614));
#32210=CARTESIAN_POINT('Ctrl Pts',(-0.229657495501249,0.0148507081915223,
-0.00705955615765789));
#32211=CARTESIAN_POINT('Ctrl Pts',(-0.229589479953617,0.0148855070542966,
-0.00700795588366666));
#32212=CARTESIAN_POINT('Ctrl Pts',(-0.229453448858355,0.0149551047798453,
-0.0069047553356842));
#32213=CARTESIAN_POINT('Ctrl Pts',(-0.22930647593101,0.0150295874152323,
-0.00678953050805577));
#32214=CARTESIAN_POINT('Ctrl Pts',(-0.229171345764821,0.0150973553358833,
-0.00667973005196626));
#32215=CARTESIAN_POINT('Ctrl Pts',(-0.229036215598631,0.0151651232565343,
-0.00656992959587674));
#32216=CARTESIAN_POINT('Ctrl Pts',(-0.228912924944156,0.0152266020801001,
-0.00646582291419951));
#32217=CARTESIAN_POINT('Ctrl Pts',(-0.228784731269557,0.0152901893183376,
-0.00635310900734669));
#32218=CARTESIAN_POINT('Ctrl Pts',(-0.228656537594957,0.015353776556575,
-0.00624039510049387));
#32219=CARTESIAN_POINT('Ctrl Pts',(-0.228523442779258,0.0154191443299652,
-0.00611888796668704));
#32220=CARTESIAN_POINT('Ctrl Pts',(-0.228396736144486,0.0154805617283158,
-0.00599843481886273));
#32221=CARTESIAN_POINT('Ctrl Pts',(-0.228270029509714,0.0155419791266665,
-0.00587798167103842));
#32222=CARTESIAN_POINT('Ctrl Pts',(-0.228149709917567,0.0155997207953437,
-0.00575872349910771));
#32223=CARTESIAN_POINT('Ctrl Pts',(-0.228026646433393,0.0156579298630215,
-0.00563126705671706));
#32224=CARTESIAN_POINT('Ctrl Pts',(-0.228016605549242,0.015662679204461,
-0.00562086774630496));
#32225=CARTESIAN_POINT('Ctrl Pts',(-0.228006546404433,0.0156674307478862,
-0.00561041336623902));
#32226=CARTESIAN_POINT('Ctrl Pts',(-0.227996474915176,0.0156721811407406,
-0.00559990996590028));
#32227=CARTESIAN_POINT('Ctrl Pts',(-0.227883107816741,0.0157256527019563,
-0.00548168117274438));
#32228=CARTESIAN_POINT('Ctrl Pts',(-0.227768176640571,0.0157788534865566,
-0.00535719105107656));
#32229=CARTESIAN_POINT('Ctrl Pts',(-0.227660119078464,0.0158278578958162,
-0.00523542087007314));
#32230=CARTESIAN_POINT('Ctrl Pts',(-0.227542461724258,0.015881215837875,
-0.00510283267320184));
#32231=CARTESIAN_POINT('Ctrl Pts',(-0.227432953141424,0.0159299038159691,
-0.00497359566486382));
#32232=CARTESIAN_POINT('Ctrl Pts',(-0.227323539266157,0.0159777270605206,
-0.00483732653405633));
#32233=CARTESIAN_POINT('Ctrl Pts',(-0.227104711515624,0.0160733735496236,
-0.00456478827244135));
#32234=CARTESIAN_POINT('Ctrl Pts',(-0.226886262490342,0.0161640968769926,
-0.00426357577786167));
#32235=CARTESIAN_POINT('Ctrl Pts',(-0.226686889965372,0.016238216528244,
-0.00396147808314125));
#32236=CARTESIAN_POINT('Ctrl Pts',(-0.226487517440402,0.0163123361794955,
-0.00365938038842082));
#32237=CARTESIAN_POINT('Ctrl Pts',(-0.226307228819621,0.0163715748698451,
-0.00335681294423736));
#32238=CARTESIAN_POINT('Ctrl Pts',(-0.22613006964741,0.0164173393056575,
-0.00302983300065918));
#32239=CARTESIAN_POINT('Ctrl Pts',(-0.226041490061305,0.0164402215235637,
-0.00286634302887009));
#32240=CARTESIAN_POINT('Ctrl Pts',(-0.225953689054931,0.0164593064887217,
-0.00269670427482913));
#32241=CARTESIAN_POINT('Ctrl Pts',(-0.225873228778512,0.0164732474391017,
-0.00253266872281594));
#32242=CARTESIAN_POINT('Ctrl Pts',(-0.225839509654998,0.0164790897832831,
-0.00246392504848051));
#32243=CARTESIAN_POINT('Ctrl Pts',(-0.225807079371206,0.0164840666076802,
-0.00239619099430726));
#32244=CARTESIAN_POINT('Ctrl Pts',(-0.225775739961391,0.0164882613906457,
-0.00232903612135096));
#32245=CARTESIAN_POINT('Ctrl Pts',(-0.22573229754672,0.0164940761619552,
-0.00223594662619258));
#32246=CARTESIAN_POINT('Ctrl Pts',(-0.225690951274861,0.0164996201239921,
-0.00214463734262893));
#32247=CARTESIAN_POINT('Ctrl Pts',(-0.225651173843744,0.0165049400475781,
-0.00205378107599625));
#32248=CARTESIAN_POINT('Ctrl Pts',(-0.225582700926324,0.016514097770391,
-0.00189738099013219));
#32249=CARTESIAN_POINT('Ctrl Pts',(-0.2255188625694,0.0165225938264315,
-0.00174296906619653));
#32250=CARTESIAN_POINT('Ctrl Pts',(-0.22545387460209,0.0165308013835412,
-0.00157727287014463));
#32251=CARTESIAN_POINT('Ctrl Pts',(-0.225421380618434,0.0165349051620961,
-0.00149442477211867));
#32252=CARTESIAN_POINT('Ctrl Pts',(-0.225388599309305,0.0165389341830696,
-0.0014087549278449));
#32253=CARTESIAN_POINT('Ctrl Pts',(-0.225354400970614,0.0165429393029416,
-0.0013165744898758));
#32254=CARTESIAN_POINT('Ctrl Pts',(-0.225334634352807,0.0165452542596561,
-0.00126329425591231));
#32255=CARTESIAN_POINT('Ctrl Pts',(-0.225314394059584,0.016547552895731,
-0.0012078361574181));
#32256=CARTESIAN_POINT('Ctrl Pts',(-0.225294998104697,0.0165496652083673,
-0.00115407592783882));
#32257=CARTESIAN_POINT('Ctrl Pts',(-0.225280837006934,0.0165512074199223,
-0.00111482527628472));
#32258=CARTESIAN_POINT('Ctrl Pts',(-0.225267125987414,0.0165526516895471,
-0.00107647865586791));
#32259=CARTESIAN_POINT('Ctrl Pts',(-0.225254377998706,0.0165539545376519,
-0.00104054141329506));
#32260=CARTESIAN_POINT('Ctrl Pts',(-0.225224169540618,0.0165570418507387,
-0.000955382200266533));
#32261=CARTESIAN_POINT('Ctrl Pts',(-0.225199370447548,0.0165594075983991,
-0.000883760964632949));
#32262=CARTESIAN_POINT('Ctrl Pts',(-0.225169605988872,0.0165619809696788,
-0.000796234956166043));
#32263=CARTESIAN_POINT('Ctrl Pts',(-0.225139841530196,0.0165645543409585,
-0.000708708947699136));
#32264=CARTESIAN_POINT('Ctrl Pts',(-0.225105109287165,0.016567173521703,
-0.000605273992315721));
#32265=CARTESIAN_POINT('Ctrl Pts',(-0.225077485368256,0.0165689500200869,
-0.000522302514831214));
#32266=CARTESIAN_POINT('Ctrl Pts',(-0.225049861449347,0.0165707265184708,
-0.000439331037346707));
#32267=CARTESIAN_POINT('Ctrl Pts',(-0.225029348756218,0.0165718486883789,
-0.000376825865973877));
#32268=CARTESIAN_POINT('Ctrl Pts',(-0.225002310730227,0.0165730394231567,
-0.000294349705289951));
#32269=CARTESIAN_POINT('Ctrl Pts',(-0.224975272938767,0.0165742301476059,
-0.000211874260014666));
#32270=CARTESIAN_POINT('Ctrl Pts',(-0.224941708010107,0.0165753666276692,
-0.000109427566739171));
#32271=CARTESIAN_POINT('Ctrl Pts',(-0.224906163263034,0.0165759221188024,
-4.4501404137285E-7));
#32272=CARTESIAN_POINT('Ctrl Pts',(-0.224906162751896,0.016575922126827,
-4.40896898322947E-7));
#32273=CARTESIAN_POINT('Ctrl Pts',(-0.224941316351692,0.0165753758643503,
0.000108387621803853));
#32274=CARTESIAN_POINT('Ctrl Pts',(-0.225007616272799,0.0165730232478589,
0.00031277968645102));
#32275=CARTESIAN_POINT('Ctrl Pts',(-0.225067714507346,0.0165698105290274,
0.000497786035753373));
#32276=CARTESIAN_POINT('Ctrl Pts',(-0.225170449863763,0.0165620461258707,
0.00080734815416336));
#32277=CARTESIAN_POINT('Ctrl Pts',(-0.225244110283856,0.0165549138835177,
0.00102286209902418));
#32278=CARTESIAN_POINT('Ctrl Pts',(-0.225347914701633,0.0165433851135797,
0.00131538426692397));
#32279=CARTESIAN_POINT('Ctrl Pts',(-0.225461777579014,0.0165291028114222,
0.00162079186653887));
#32280=CARTESIAN_POINT('Ctrl Pts',(-0.225605867979303,0.0165102324611029,
0.00197868258918669));
#32281=CARTESIAN_POINT('Ctrl Pts',(-0.225719822319268,0.0164937064301101,
0.00223747884891758));
#32282=CARTESIAN_POINT('Ctrl Pts',(-0.225761332775488,0.0164871798990637,
0.00232893089033043));
#32283=CARTESIAN_POINT('',(-0.204292068243473,0.00260972885206963,-0.00893763826762711));
#32284=CARTESIAN_POINT('',(-0.203101435073175,0.00260940702415168,-0.00891395394943401));
#32285=CARTESIAN_POINT('',(-0.204292066964792,0.00260973006230206,-0.00893763333202277));
#32286=CARTESIAN_POINT('',(-0.203011006310301,0.00748198867741155,-0.0102941239933332));
#32287=CARTESIAN_POINT('Ctrl Pts',(-0.203013460631671,0.00748225597834897,
-0.01029589855914));
#32288=CARTESIAN_POINT('Ctrl Pts',(-0.202890737335905,0.00646872173921062,
-0.0102911781864089));
#32289=CARTESIAN_POINT('Ctrl Pts',(-0.202862048102838,0.00560185800414398,
-0.0101217239278096));
#32290=CARTESIAN_POINT('Ctrl Pts',(-0.202882559174494,0.00402897744691195,
-0.00967756834064981));
#32291=CARTESIAN_POINT('Ctrl Pts',(-0.20298717036797,0.00325117937997227,
-0.00930626342577085));
#32292=CARTESIAN_POINT('Ctrl Pts',(-0.203101405362522,0.00261009398323347,
-0.00891437067179455));
#32293=CARTESIAN_POINT('',(-0.203091797564858,0.0123956741229182,-0.00891063212388402));
#32294=CARTESIAN_POINT('Ctrl Pts',(-0.202996531950095,0.00750041510153064,
-0.0102955329893099));
#32295=CARTESIAN_POINT('Ctrl Pts',(-0.202973028026754,0.00777693274683738,
-0.0102949893546688));
#32296=CARTESIAN_POINT('Ctrl Pts',(-0.202943195461771,0.00814713734367451,
-0.0102756841645984));
#32297=CARTESIAN_POINT('Ctrl Pts',(-0.202918432522134,0.00848992946228484,
-0.0102417477030021));
#32298=CARTESIAN_POINT('Ctrl Pts',(-0.202906521722816,0.00867191060366439,
-0.0102195296512017));
#32299=CARTESIAN_POINT('Ctrl Pts',(-0.202900439779019,0.0087699904262681,
-0.0102066421178496));
#32300=CARTESIAN_POINT('Ctrl Pts',(-0.202890125869248,0.00895850416585149,
-0.0101787708011005));
#32301=CARTESIAN_POINT('Ctrl Pts',(-0.202880281088442,0.00917285871040499,
-0.0101425325315666));
#32302=CARTESIAN_POINT('Ctrl Pts',(-0.20286726104683,0.00955455309447455,
-0.0100679416187396));
#32303=CARTESIAN_POINT('Ctrl Pts',(-0.202863125830161,0.0100404412202094,
-0.00994714991380413));
#32304=CARTESIAN_POINT('Ctrl Pts',(-0.202883413807161,0.0106634592954592,
-0.00974969172924713));
#32305=CARTESIAN_POINT('Ctrl Pts',(-0.202926466180208,0.011176146849084,
-0.00954413107948249));
#32306=CARTESIAN_POINT('Ctrl Pts',(-0.202963217506325,0.0114893497038527,
-0.00940050398062725));
#32307=CARTESIAN_POINT('Ctrl Pts',(-0.202987606167699,0.0116811097923209,
-0.00930735232445663));
#32308=CARTESIAN_POINT('Ctrl Pts',(-0.203011098769037,0.0118529110797574,
-0.00921921645915818));
#32309=CARTESIAN_POINT('Ctrl Pts',(-0.203023596144259,0.0119401612959071,
-0.00917268091639791));
#32310=CARTESIAN_POINT('Ctrl Pts',(-0.20304984841018,0.0121205772363098,
-0.00907410908661622));
#32311=CARTESIAN_POINT('Ctrl Pts',(-0.203073505202074,0.0122772375631162,
-0.00898320363019314));
#32312=CARTESIAN_POINT('Ctrl Pts',(-0.203091797564858,0.0123956741229182,
-0.00891063212388402));
#32313=CARTESIAN_POINT('',(-0.204293520825211,0.0123942668896669,-0.00893520818590632));
#32314=CARTESIAN_POINT('',(-0.203091797686605,0.0123956703258418,-0.00891062595725835));
#32315=CARTESIAN_POINT('',(-0.20419682992175,0.00750016549753868,-0.0103226607303034));
#32316=CARTESIAN_POINT('Ctrl Pts',(-0.204293519302538,0.0123942655493259,
-0.00893520562090602));
#32317=CARTESIAN_POINT('Ctrl Pts',(-0.204275098485375,0.0122750823755585,
-0.0090084200287585));
#32318=CARTESIAN_POINT('Ctrl Pts',(-0.204259255211995,0.012170250463801,
-0.00906927480190584));
#32319=CARTESIAN_POINT('Ctrl Pts',(-0.20424519845668,0.0120752472755363,
-0.00912256605009863));
#32320=CARTESIAN_POINT('Ctrl Pts',(-0.204238170046716,0.0120277454630579,
-0.00914921179667441));
#32321=CARTESIAN_POINT('Ctrl Pts',(-0.204231589290253,0.0119826708213253,
-0.0091739156221354));
#32322=CARTESIAN_POINT('Ctrl Pts',(-0.20422624416428,0.0119458045626052,
-0.00919383477161695));
#32323=CARTESIAN_POINT('Ctrl Pts',(-0.204220899038308,0.0119089383038851,
-0.0092137539210985));
#32324=CARTESIAN_POINT('Ctrl Pts',(-0.204216787075737,0.0118803470916992,
-0.0092290098761559));
#32325=CARTESIAN_POINT('Ctrl Pts',(-0.20421076071024,0.0118372591327625,
-0.00925156467436655));
#32326=CARTESIAN_POINT('Ctrl Pts',(-0.204204734344742,0.0117941711738258,
-0.0092741194725772));
#32327=CARTESIAN_POINT('Ctrl Pts',(-0.204196798018096,0.0117364718292927,
-0.00930375609662389));
#32328=CARTESIAN_POINT('Ctrl Pts',(-0.204189753233104,0.0116835824953197,
-0.00933020964390826));
#32329=CARTESIAN_POINT('Ctrl Pts',(-0.204182708448112,0.0116306931613467,
-0.00935666319119263));
#32330=CARTESIAN_POINT('Ctrl Pts',(-0.204176552159317,0.0115826860432461,
-0.00938008049394186));
#32331=CARTESIAN_POINT('Ctrl Pts',(-0.204170681369622,0.0115357770237326,
-0.00940252102891353));
#32332=CARTESIAN_POINT('Ctrl Pts',(-0.204158939790232,0.0114419589847058,
-0.00944740209885687));
#32333=CARTESIAN_POINT('Ctrl Pts',(-0.204148340304367,0.0113525401346867,
-0.00948837408639008));
#32334=CARTESIAN_POINT('Ctrl Pts',(-0.20413834448362,0.011258693490137,
-0.00952957213746872));
#32335=CARTESIAN_POINT('Ctrl Pts',(-0.204121215724028,0.0110978786202386,
-0.00960016879285344));
#32336=CARTESIAN_POINT('Ctrl Pts',(-0.204105871698475,0.0109238361022606,
-0.00967093396616449));
#32337=CARTESIAN_POINT('Ctrl Pts',(-0.204094150246153,0.0107476948613483,
-0.00973616780463667));
#32338=CARTESIAN_POINT('Ctrl Pts',(-0.204092191135597,0.0107182548094752,
-0.00974707091613151));
#32339=CARTESIAN_POINT('Ctrl Pts',(-0.204090333223107,0.0106887587382086,
-0.00975782541208224));
#32340=CARTESIAN_POINT('Ctrl Pts',(-0.204088585089726,0.0106592618421083,
-0.00976841253402361));
#32341=CARTESIAN_POINT('Ctrl Pts',(-0.204076377790565,0.0104532836033615,
-0.00984234291379877));
#32342=CARTESIAN_POINT('Ctrl Pts',(-0.204069516229899,0.010247177684889,
-0.00990802601270076));
#32343=CARTESIAN_POINT('Ctrl Pts',(-0.204066818073886,0.0100469521393359,
-0.00996476619728215));
#32344=CARTESIAN_POINT('Ctrl Pts',(-0.204064119917873,0.00984672659378275,
-0.0100215063818635));
#32345=CARTESIAN_POINT('Ctrl Pts',(-0.204065571120084,0.00965260417818384,
-0.0100699507180676));
#32346=CARTESIAN_POINT('Ctrl Pts',(-0.204071293829835,0.00944014979634324,
-0.0101152576551124));
#32347=CARTESIAN_POINT('Ctrl Pts',(-0.204077016539586,0.00922769541450265,
-0.0101605645921573));
#32348=CARTESIAN_POINT('Ctrl Pts',(-0.204087041836827,0.00899660628102227,
-0.0102013362099875));
#32349=CARTESIAN_POINT('Ctrl Pts',(-0.204099347318883,0.00878303173230227,
-0.0102313445479147));
#32350=CARTESIAN_POINT('Ctrl Pts',(-0.204105500059911,0.00867624445794228,
-0.0102463487168783));
#32351=CARTESIAN_POINT('Ctrl Pts',(-0.204112216295476,0.00857387041820424,
-0.0102589531602456));
#32352=CARTESIAN_POINT('Ctrl Pts',(-0.204119551135905,0.00846894111221058,
-0.0102701237466303));
#32353=CARTESIAN_POINT('Ctrl Pts',(-0.204123218556119,0.00841647645921375,
-0.0102757090398227));
#32354=CARTESIAN_POINT('Ctrl Pts',(-0.20412704193822,0.00836336762879549,
-0.0102808777182749));
#32355=CARTESIAN_POINT('Ctrl Pts',(-0.204130486733839,0.00831673252746664,
-0.0102850758848288));
#32356=CARTESIAN_POINT('Ctrl Pts',(-0.204133931529458,0.0082700974261378,
-0.0102892740513827));
#32357=CARTESIAN_POINT('Ctrl Pts',(-0.204136995799708,0.00822994345958339,
-0.0102925877238228));
#32358=CARTESIAN_POINT('Ctrl Pts',(-0.204140419329825,0.00818593090051333,
-0.0102959302516981));
#32359=CARTESIAN_POINT('Ctrl Pts',(-0.204154113448717,0.0080098806844698,
-0.0103093003616625));
#32360=CARTESIAN_POINT('Ctrl Pts',(-0.204173578333277,0.00777202871891889,
-0.0103221303376117));
#32361=CARTESIAN_POINT('Ctrl Pts',(-0.204196829918995,0.00750016549729199,
-0.0103226607246193));
#32362=CARTESIAN_POINT('Ctrl Pts',(-0.204196829927013,0.00750016540354124,
-0.0103226607248022));
#32363=CARTESIAN_POINT('Ctrl Pts',(-0.204185296600283,0.00736627557242382,
-0.0103224024649696));
#32364=CARTESIAN_POINT('Ctrl Pts',(-0.204170173720485,0.00718828267231201,
-0.0103179549294819));
#32365=CARTESIAN_POINT('Ctrl Pts',(-0.204153088630003,0.00698026742655806,
-0.0103073072515267));
#32366=CARTESIAN_POINT('Ctrl Pts',(-0.204144365129465,0.00687195683859182,
-0.0103005485999431));
#32367=CARTESIAN_POINT('Ctrl Pts',(-0.204129528175449,0.00667906286088234,
-0.0102853466214339));
#32368=CARTESIAN_POINT('Ctrl Pts',(-0.204114088107036,0.00646341547837495,
-0.0102635347495406));
#32369=CARTESIAN_POINT('Ctrl Pts',(-0.204098618494934,0.00622876334523883,
-0.0102348069970239));
#32370=CARTESIAN_POINT('Ctrl Pts',(-0.204080493922748,0.00587940935304134,
-0.0101798881435763));
#32371=CARTESIAN_POINT('Ctrl Pts',(-0.204066164101744,0.0054538486912532,
-0.0100959729412001));
#32372=CARTESIAN_POINT('Ctrl Pts',(-0.204061500170532,0.00496565424176834,
-0.00997598165923886));
#32373=CARTESIAN_POINT('Ctrl Pts',(-0.204079665330309,0.00443189461430586,
-0.00980478175309179));
#32374=CARTESIAN_POINT('Ctrl Pts',(-0.204106657151681,0.00405435642971818,
-0.00966232705712367));
#32375=CARTESIAN_POINT('Ctrl Pts',(-0.204137703479563,0.00373318001710212,
-0.00952804466465791));
#32376=CARTESIAN_POINT('Ctrl Pts',(-0.204163349720393,0.00351683255250259,
-0.00942841282273942));
#32377=CARTESIAN_POINT('Ctrl Pts',(-0.204187933392733,0.00332430267970029,
-0.00933487767638302));
#32378=CARTESIAN_POINT('Ctrl Pts',(-0.204211586788645,0.00315180164980181,
-0.00924625546080158));
#32379=CARTESIAN_POINT('Ctrl Pts',(-0.204223864452251,0.00306614233221466,
-0.0092005126880041));
#32380=CARTESIAN_POINT('Ctrl Pts',(-0.204250056460208,0.00288600567993886,
-0.00910201089232994));
#32381=CARTESIAN_POINT('Ctrl Pts',(-0.204273721709538,0.00272888562244924,
-0.00901075832037522));
#32382=CARTESIAN_POINT('Ctrl Pts',(-0.204292066659032,0.00260972723221402,
-0.0089376405099374));
#32383=CARTESIAN_POINT('',(-0.206293207427109,0.00261116688226644,-0.00897808488880184));
#32384=CARTESIAN_POINT('',(-0.205091220874504,0.00261029994409268,-0.00895378396279216));
#32385=CARTESIAN_POINT('',(-0.206293206209515,0.00261116809564738,-0.00897808010478434));
#32386=CARTESIAN_POINT('',(-0.204995830964606,0.00750018061144568,-0.01034071880922));
#32387=CARTESIAN_POINT('Ctrl Pts',(-0.205091218737904,0.00261030113134024,
-0.00895378149630639));
#32388=CARTESIAN_POINT('Ctrl Pts',(-0.205073038446696,0.0027283973634415,
-0.00902637612295405));
#32389=CARTESIAN_POINT('Ctrl Pts',(-0.205049507187242,0.00288473012510694,
-0.00911738532094257));
#32390=CARTESIAN_POINT('Ctrl Pts',(-0.205023348755059,0.00306502113689564,
-0.00921619836789005));
#32391=CARTESIAN_POINT('Ctrl Pts',(-0.205010861943808,0.00315244889182092,
-0.00926296620515238));
#32392=CARTESIAN_POINT('Ctrl Pts',(-0.204987412224421,0.00332423590481222,
-0.00935136480094043));
#32393=CARTESIAN_POINT('Ctrl Pts',(-0.204962930879865,0.00351688601712408,
-0.00944514868659994));
#32394=CARTESIAN_POINT('Ctrl Pts',(-0.204937222363819,0.00373534002291959,
-0.00954583931029786));
#32395=CARTESIAN_POINT('Ctrl Pts',(-0.204906755137115,0.00405272141224298,
-0.00967875941234199));
#32396=CARTESIAN_POINT('Ctrl Pts',(-0.204879536268564,0.00443330123098864,
-0.00982262592539781));
#32397=CARTESIAN_POINT('Ctrl Pts',(-0.204861383847208,0.00496277755586631,
-0.00999271395898353));
#32398=CARTESIAN_POINT('Ctrl Pts',(-0.204865634488468,0.00545524074413209,
-0.0101140737523899));
#32399=CARTESIAN_POINT('Ctrl Pts',(-0.204879709034891,0.00588082021089614,
-0.0101979873791187));
#32400=CARTESIAN_POINT('Ctrl Pts',(-0.204897593596836,0.00622967416483981,
-0.0102528606149596));
#32401=CARTESIAN_POINT('Ctrl Pts',(-0.204912950260743,0.00646383985211491,
-0.0102815531993233));
#32402=CARTESIAN_POINT('Ctrl Pts',(-0.204928345204359,0.00667926356803342,
-0.0103033631066581));
#32403=CARTESIAN_POINT('Ctrl Pts',(-0.20494314048499,0.0068716218281429,
-0.0103185488470304));
#32404=CARTESIAN_POINT('Ctrl Pts',(-0.20495195108621,0.006980845097099,
-0.0103253770145249));
#32405=CARTESIAN_POINT('Ctrl Pts',(-0.204969098328994,0.00718899852828588,
-0.0103360288719754));
#32406=CARTESIAN_POINT('Ctrl Pts',(-0.204984270571741,0.00736672617235706,
-0.0103404601549147));
#32407=CARTESIAN_POINT('Ctrl Pts',(-0.204995830964606,0.00750018061144568,
-0.01034071880922));
#32408=CARTESIAN_POINT('',(-0.205092341371519,0.0123935602159587,-0.00895141703515626));
#32409=CARTESIAN_POINT('Ctrl Pts',(-0.204995831063211,0.00750018174974929,
-0.0103407188114261));
#32410=CARTESIAN_POINT('Ctrl Pts',(-0.204984334367631,0.00763376142047935,
-0.0103404563384653));
#32411=CARTESIAN_POINT('Ctrl Pts',(-0.204969242259353,0.00781169707145735,
-0.0103360126094618));
#32412=CARTESIAN_POINT('Ctrl Pts',(-0.204952175210056,0.00802021735232026,
-0.0103253230549911));
#32413=CARTESIAN_POINT('Ctrl Pts',(-0.204943403020839,0.00812966122370435,
-0.010318469780649));
#32414=CARTESIAN_POINT('Ctrl Pts',(-0.204928658061841,0.00832258199862167,
-0.0103032092465372));
#32415=CARTESIAN_POINT('Ctrl Pts',(-0.204913319337647,0.00853854827886881,
-0.0102812989237937));
#32416=CARTESIAN_POINT('Ctrl Pts',(-0.204898006317538,0.00877356793052689,
-0.0102524253354524));
#32417=CARTESIAN_POINT('Ctrl Pts',(-0.20488022415611,0.00912228369014853,
-0.0101974532003693));
#32418=CARTESIAN_POINT('Ctrl Pts',(-0.20486621057911,0.00954790324330249,
-0.0101133538141053));
#32419=CARTESIAN_POINT('Ctrl Pts',(-0.204861855720688,0.010037836615467,
-0.00999260025333758));
#32420=CARTESIAN_POINT('Ctrl Pts',(-0.204880098002849,0.0105711418094981,
-0.00982106567079185));
#32421=CARTESIAN_POINT('Ctrl Pts',(-0.204907090184449,0.0109495407743111,
-0.00967787507932532));
#32422=CARTESIAN_POINT('Ctrl Pts',(-0.204937963378322,0.0112700899770492,
-0.00954347334300635));
#32423=CARTESIAN_POINT('Ctrl Pts',(-0.204963627185177,0.0114873226245486,
-0.00944315781658447));
#32424=CARTESIAN_POINT('Ctrl Pts',(-0.20498816737331,0.0116797965093522,
-0.00934935193686226));
#32425=CARTESIAN_POINT('Ctrl Pts',(-0.205011652075311,0.0118512232809713,
-0.00926103771969262));
#32426=CARTESIAN_POINT('Ctrl Pts',(-0.205024193079732,0.0119387130080461,
-0.00921418941879961));
#32427=CARTESIAN_POINT('Ctrl Pts',(-0.205050448708611,0.0121189966104724,
-0.0091152741114829));
#32428=CARTESIAN_POINT('Ctrl Pts',(-0.205074081100572,0.0122754031260107,
-0.00902412724127784));
#32429=CARTESIAN_POINT('Ctrl Pts',(-0.205092341371519,0.0123935602159587,
-0.00895141703515626));
#32430=CARTESIAN_POINT('',(-0.20629401114421,0.0123924210579408,-0.00897588382629872));
#32431=CARTESIAN_POINT('',(-0.205092341489181,0.0123935565388823,-0.00895141108884611));
#32432=CARTESIAN_POINT('',(-0.206196247266385,0.00750007921659101,-0.0103678492122642));
#32433=CARTESIAN_POINT('Ctrl Pts',(-0.206294009778539,0.0123924197511446,
-0.00897588136592045));
#32434=CARTESIAN_POINT('Ctrl Pts',(-0.206275629933268,0.0122735287593914,
-0.00904923077174543));
#32435=CARTESIAN_POINT('Ctrl Pts',(-0.206251898274911,0.0121166099521123,
-0.00914086409857169));
#32436=CARTESIAN_POINT('Ctrl Pts',(-0.206225586245474,0.0119364025232917,
-0.00923992860321053));
#32437=CARTESIAN_POINT('Ctrl Pts',(-0.20621320957114,0.011850415602355,
-0.00928608543340328));
#32438=CARTESIAN_POINT('Ctrl Pts',(-0.206189421186814,0.0116777449991496,
-0.00937524164969374));
#32439=CARTESIAN_POINT('Ctrl Pts',(-0.206164666829607,0.0114849804098469,
-0.0094693586360107));
#32440=CARTESIAN_POINT('Ctrl Pts',(-0.206138729986972,0.0112675531340228,
-0.00956992324979396));
#32441=CARTESIAN_POINT('Ctrl Pts',(-0.206107574836102,0.0109483810244031,
-0.00970399210164722));
#32442=CARTESIAN_POINT('Ctrl Pts',(-0.206079918334012,0.0105696487151287,
-0.00984755873583954));
#32443=CARTESIAN_POINT('Ctrl Pts',(-0.206061320221384,0.0100390013969364,
-0.0100186198580634));
#32444=CARTESIAN_POINT('Ctrl Pts',(-0.206065538394757,0.00954660497520976,
-0.0101402971232334));
#32445=CARTESIAN_POINT('Ctrl Pts',(-0.206079659153249,0.00912064692309937,
-0.0102245493877391));
#32446=CARTESIAN_POINT('Ctrl Pts',(-0.206097649530151,0.00877166321992288,
-0.0102796197167479));
#32447=CARTESIAN_POINT('Ctrl Pts',(-0.206113124691997,0.00853683963756153,
-0.0103084791137337));
#32448=CARTESIAN_POINT('Ctrl Pts',(-0.206128578247856,0.00832144144316739,
-0.0103303502197896));
#32449=CARTESIAN_POINT('Ctrl Pts',(-0.206143442183771,0.0081289230195232,
-0.0103455919214823));
#32450=CARTESIAN_POINT('Ctrl Pts',(-0.206152196968296,0.0080207509803179,
-0.0103523791392198));
#32451=CARTESIAN_POINT('Ctrl Pts',(-0.20616937593705,0.00781267213620248,
-0.010363092481908));
#32452=CARTESIAN_POINT('Ctrl Pts',(-0.206184614854141,0.00763433161462997,
-0.0103675851511799));
#32453=CARTESIAN_POINT('Ctrl Pts',(-0.206196247269383,0.00750007928854104,
-0.0103678492126068));
#32454=CARTESIAN_POINT('Ctrl Pts',(-0.206196247263134,0.00750007921687407,
-0.0103678492124662));
#32455=CARTESIAN_POINT('Ctrl Pts',(-0.206184538016218,0.00736579215378392,
-0.0103675857323272));
#32456=CARTESIAN_POINT('Ctrl Pts',(-0.20616920962137,0.00718753481197185,
-0.0103630948863018));
#32457=CARTESIAN_POINT('Ctrl Pts',(-0.206151939567772,0.00697963270310972,
-0.0103523925616913));
#32458=CARTESIAN_POINT('Ctrl Pts',(-0.206143177224608,0.00687203383816881,
-0.010345652193588));
#32459=CARTESIAN_POINT('Ctrl Pts',(-0.206128179901813,0.00667889666688518,
-0.0103303743273525));
#32460=CARTESIAN_POINT('Ctrl Pts',(-0.206112637080238,0.00646336544810845,
-0.0103084932875251));
#32461=CARTESIAN_POINT('Ctrl Pts',(-0.206097083534865,0.00622820103627389,
-0.0102795775402357));
#32462=CARTESIAN_POINT('Ctrl Pts',(-0.206079166473915,0.00588103593041778,
-0.0102248175800093));
#32463=CARTESIAN_POINT('Ctrl Pts',(-0.206065099208172,0.0054560678829398,
-0.010140868723724));
#32464=CARTESIAN_POINT('Ctrl Pts',(-0.206060944985599,0.00496475893419326,
-0.0100196997915405));
#32465=CARTESIAN_POINT('Ctrl Pts',(-0.20607975759831,0.00443234740802005,
-0.00984824726940087));
#32466=CARTESIAN_POINT('Ctrl Pts',(-0.206107426047253,0.00405426418978633,
-0.00970505346746708));
#32467=CARTESIAN_POINT('Ctrl Pts',(-0.206138707262331,0.00373379004888558,
-0.00957052329097599));
#32468=CARTESIAN_POINT('Ctrl Pts',(-0.206164472409347,0.00351745989703588,
-0.00947050613876221));
#32469=CARTESIAN_POINT('Ctrl Pts',(-0.206189109621405,0.00332506288356478,
-0.00937664775095104));
#32470=CARTESIAN_POINT('Ctrl Pts',(-0.206212763871631,0.00315278593877367,
-0.00928777221922359));
#32471=CARTESIAN_POINT('Ctrl Pts',(-0.206225080280031,0.0030669007354627,
-0.00924171469636897));
#32472=CARTESIAN_POINT('Ctrl Pts',(-0.206251269492468,0.00288687783244609,
-0.0091428463681189));
#32473=CARTESIAN_POINT('Ctrl Pts',(-0.206274900907247,0.00273002804570731,
-0.00905134588017306));
#32474=CARTESIAN_POINT('Ctrl Pts',(-0.206293205915242,0.00261116529613781,
-0.00897808708453545));
#32475=CARTESIAN_POINT('',(-0.208294281955803,0.00261264102269791,-0.00901864434210674));
#32476=CARTESIAN_POINT('',(-0.20709233610443,0.00261177385669708,-0.00899428899190795));
#32477=CARTESIAN_POINT('',(-0.208294280799351,0.00261264227468941,-0.00901863964824329));
#32478=CARTESIAN_POINT('',(-0.206995159908711,0.00750002205440221,-0.0103859052997544));
#32479=CARTESIAN_POINT('Ctrl Pts',(-0.207092334177755,0.0026117750543677,
-0.00899428657135199));
#32480=CARTESIAN_POINT('Ctrl Pts',(-0.207074189408243,0.00272957361446454,
-0.00906701495139803));
#32481=CARTESIAN_POINT('Ctrl Pts',(-0.207050686386804,0.00288563070243773,
-0.00915826339207637));
#32482=CARTESIAN_POINT('Ctrl Pts',(-0.207024524692812,0.0030657969487444,
-0.00925743433152502));
#32483=CARTESIAN_POINT('Ctrl Pts',(-0.207011996627476,0.00315344113935562,
-0.00930451415959934));
#32484=CARTESIAN_POINT('Ctrl Pts',(-0.206988540251261,0.00332499174150683,
-0.00939315711270464));
#32485=CARTESIAN_POINT('Ctrl Pts',(-0.206963992767868,0.00351757661523681,
-0.00948728809442778));
#32486=CARTESIAN_POINT('Ctrl Pts',(-0.206938222613739,0.00373542462863214,
-0.00958812909678874));
#32487=CARTESIAN_POINT('Ctrl Pts',(-0.206907280012449,0.00405444268434713,
-0.00972222069990457));
#32488=CARTESIAN_POINT('Ctrl Pts',(-0.206879699677835,0.00443263550097346,
-0.00986566273753742));
#32489=CARTESIAN_POINT('Ctrl Pts',(-0.206860828660484,0.00496231258650676,
-0.0100365956434048));
#32490=CARTESIAN_POINT('Ctrl Pts',(-0.206864635917835,0.00545699157383567,
-0.0101588612972589));
#32491=CARTESIAN_POINT('Ctrl Pts',(-0.206878443249798,0.00588212796561463,
-0.0102428714297392));
#32492=CARTESIAN_POINT('Ctrl Pts',(-0.206896114734401,0.0062290841634208,
-0.0102976326277652));
#32493=CARTESIAN_POINT('Ctrl Pts',(-0.206911530121765,0.0064637966547499,
-0.0103265148036063));
#32494=CARTESIAN_POINT('Ctrl Pts',(-0.206927002746087,0.00667909031637067,
-0.010348390628485));
#32495=CARTESIAN_POINT('Ctrl Pts',(-0.206941927161123,0.00687158087442238,
-0.0103636439973363));
#32496=CARTESIAN_POINT('Ctrl Pts',(-0.206950771218564,0.0069801693552064,
-0.0103704600676468));
#32497=CARTESIAN_POINT('Ctrl Pts',(-0.206968081273249,0.00718821308792682,
-0.0103811664345483));
#32498=CARTESIAN_POINT('Ctrl Pts',(-0.206983439481071,0.00736619442711862,
-0.0103856407315178));
#32499=CARTESIAN_POINT('Ctrl Pts',(-0.206995159908711,0.00750002205440221,
-0.0103859052997544));
#32500=CARTESIAN_POINT('',(-0.207092865232531,0.0123914993286869,-0.00899226456837298));
#32501=CARTESIAN_POINT('Ctrl Pts',(-0.206995160031523,0.00750002345672208,
-0.0103859053025266));
#32502=CARTESIAN_POINT('Ctrl Pts',(-0.20698349311307,0.00763394443319968,
-0.0103856412779244));
#32503=CARTESIAN_POINT('Ctrl Pts',(-0.206968199965542,0.00781210259696279,
-0.0103811621280426));
#32504=CARTESIAN_POINT('Ctrl Pts',(-0.206950949156072,0.00802049676584612,
-0.0103704272461815));
#32505=CARTESIAN_POINT('Ctrl Pts',(-0.206942129888732,0.00812932220630246,
-0.0103635892330472));
#32506=CARTESIAN_POINT('Ctrl Pts',(-0.2069272342099,0.00832235552725582,
-0.0103482700117016));
#32507=CARTESIAN_POINT('Ctrl Pts',(-0.206911789920796,0.00853818425630776,
-0.010326302799079));
#32508=CARTESIAN_POINT('Ctrl Pts',(-0.206896386071748,0.00877369921132409,
-0.0102972571016713));
#32509=CARTESIAN_POINT('Ctrl Pts',(-0.206878751394063,0.00912063966793892,
-0.0102423901690412));
#32510=CARTESIAN_POINT('Ctrl Pts',(-0.206864923342377,0.00954576442995532,
-0.0101582262883187));
#32511=CARTESIAN_POINT('Ctrl Pts',(-0.20686095225699,0.0100380835322156,
-0.0100364882851224));
#32512=CARTESIAN_POINT('Ctrl Pts',(-0.206879694411204,0.0105701995383101,
-0.00986470231345221));
#32513=CARTESIAN_POINT('Ctrl Pts',(-0.206907300051337,0.0109490997977367,
-0.00972081160777631));
#32514=CARTESIAN_POINT('Ctrl Pts',(-0.206938373989643,0.0112689311788443,
-0.00958619717352718));
#32515=CARTESIAN_POINT('Ctrl Pts',(-0.20696414502829,0.0114861193909925,
-0.00948552661292593));
#32516=CARTESIAN_POINT('Ctrl Pts',(-0.206988732505316,0.0116784484693535,
-0.00939142218364685));
#32517=CARTESIAN_POINT('Ctrl Pts',(-0.207012217724842,0.0118496547665064,
-0.00930287261316598));
#32518=CARTESIAN_POINT('Ctrl Pts',(-0.207024793977032,0.0119373414710472,
-0.00925572972841337));
#32519=CARTESIAN_POINT('Ctrl Pts',(-0.2070510451993,0.0121174974653495,
-0.00915647501397999));
#32520=CARTESIAN_POINT('Ctrl Pts',(-0.207074643938323,0.0122736323678574,
-0.00906510156350076));
#32521=CARTESIAN_POINT('Ctrl Pts',(-0.207092865232531,0.0123914993286869,
-0.00899226456837298));
#32522=CARTESIAN_POINT('',(-0.208294510632333,0.0123904527314057,-0.00901672992862032));
#32523=CARTESIAN_POINT('',(-0.207092865348001,0.0123914957129992,-0.00899225874580488));
#32524=CARTESIAN_POINT('',(-0.208195607947799,0.00749997628122267,-0.0104130364120898));
#32525=CARTESIAN_POINT('Ctrl Pts',(-0.208294509417452,0.0123904514344384,
-0.00901672753192577));
#32526=CARTESIAN_POINT('Ctrl Pts',(-0.208276181164632,0.0122719181404718,
-0.00909016225797937));
#32527=CARTESIAN_POINT('Ctrl Pts',(-0.208252498633871,0.0121153542506921,
-0.00918197594062883));
#32528=CARTESIAN_POINT('Ctrl Pts',(-0.208226205748594,0.0119353502174475,
-0.00928134228950543));
#32529=CARTESIAN_POINT('Ctrl Pts',(-0.208213799926976,0.0118491943161256,
-0.00932777792712348));
#32530=CARTESIAN_POINT('Ctrl Pts',(-0.208190020192328,0.0116767848974124,
-0.00941715861423961));
#32531=CARTESIAN_POINT('Ctrl Pts',(-0.208165218664378,0.0114841186574925,
-0.00951159792424035));
#32532=CARTESIAN_POINT('Ctrl Pts',(-0.20813924384415,0.0112673281691524,
-0.00961228834450963));
#32533=CARTESIAN_POINT('Ctrl Pts',(-0.208107640684676,0.0109465229857111,
-0.00974752224379483));
#32534=CARTESIAN_POINT('Ctrl Pts',(-0.208079653839285,0.0105700841576997,
-0.00989068383234901));
#32535=CARTESIAN_POINT('Ctrl Pts',(-0.208060396592719,0.0100390834471602,
-0.0100626074030206));
#32536=CARTESIAN_POINT('Ctrl Pts',(-0.20806426493074,0.00954487186568535,
-0.0101850785676279));
#32537=CARTESIAN_POINT('Ctrl Pts',(-0.208078190088483,0.00911929227250148,
-0.0102694456505221));
#32538=CARTESIAN_POINT('Ctrl Pts',(-0.208096036535253,0.00877188338428215,
-0.0103244430295817));
#32539=CARTESIAN_POINT('Ctrl Pts',(-0.208111592493633,0.00853669280746013,
-0.0103534605517206));
#32540=CARTESIAN_POINT('Ctrl Pts',(-0.208127155320244,0.00832140634310011,
-0.0103753960639456));
#32541=CARTESIAN_POINT('Ctrl Pts',(-0.208142180512124,0.00812869235806478,
-0.0103907052740522));
#32542=CARTESIAN_POINT('Ctrl Pts',(-0.208150979455223,0.00802119205908008,
-0.010397474514162));
#32543=CARTESIAN_POINT('Ctrl Pts',(-0.208168348636477,0.00781321983289299,
-0.0104082377911213));
#32544=CARTESIAN_POINT('Ctrl Pts',(-0.208183797114821,0.00763461668549679,
-0.0104127698308575));
#32545=CARTESIAN_POINT('Ctrl Pts',(-0.208195607954992,0.007499976450901,
-0.0104130364190918));
#32546=CARTESIAN_POINT('Ctrl Pts',(-0.208195607940087,0.00749997628188942,
-0.0104130364187545));
#32547=CARTESIAN_POINT('Ctrl Pts',(-0.208183719664188,0.00736516411101924,
-0.0104127673845096));
#32548=CARTESIAN_POINT('Ctrl Pts',(-0.20817336389066,0.00724604273358998,
-0.0104096613586105));
#32549=CARTESIAN_POINT('Ctrl Pts',(-0.208164092614058,0.00713701838909442,
-0.0104051382902462));
#32550=CARTESIAN_POINT('Ctrl Pts',(-0.20815945697382,0.00708250619406622,
-0.010402876755119));
#32551=CARTESIAN_POINT('Ctrl Pts',(-0.208155093639217,0.00703051928157966,
-0.010400208702842));
#32552=CARTESIAN_POINT('Ctrl Pts',(-0.208151447072726,0.00698669776957684,
-0.0103976757432969));
#32553=CARTESIAN_POINT('Ctrl Pts',(-0.208147800506235,0.00694287625757402,
-0.0103951427837518));
#32554=CARTESIAN_POINT('Ctrl Pts',(-0.208144867772773,0.00690721346999065,
-0.0103928748950214));
#32555=CARTESIAN_POINT('Ctrl Pts',(-0.20814087628415,0.00685714754652952,
-0.0103892788868975));
#32556=CARTESIAN_POINT('Ctrl Pts',(-0.208136884795528,0.00680708162306839,
-0.0103856828787736));
#32557=CARTESIAN_POINT('Ctrl Pts',(-0.208131839666141,0.00674262825539959,
-0.010380532083281));
#32558=CARTESIAN_POINT('Ctrl Pts',(-0.20812736491757,0.00668347219054577,
-0.0103751684672179));
#32559=CARTESIAN_POINT('Ctrl Pts',(-0.208122890168998,0.00662431612569194,
-0.0103698048511548));
#32560=CARTESIAN_POINT('Ctrl Pts',(-0.208118982565773,0.00657044290211078,
-0.0103643720707445));
#32561=CARTESIAN_POINT('Ctrl Pts',(-0.208115338133192,0.00651881723080284,
-0.0103587675237056));
#32562=CARTESIAN_POINT('Ctrl Pts',(-0.20810804926803,0.00641556588818696,
-0.010347558429628));
#32563=CARTESIAN_POINT('Ctrl Pts',(-0.208101810000662,0.00632129812238758,
-0.0103357986961478));
#32564=CARTESIAN_POINT('Ctrl Pts',(-0.208095738311044,0.00621657821790559,
-0.0103209758955231));
#32565=CARTESIAN_POINT('Ctrl Pts',(-0.208089666621426,0.0061118583134236,
-0.0103061530948985));
#32566=CARTESIAN_POINT('Ctrl Pts',(-0.208083771217597,0.00599673817473072,
-0.0102878795171945));
#32567=CARTESIAN_POINT('Ctrl Pts',(-0.208079101993661,0.00588611975357556,
-0.0102681842171327));
#32568=CARTESIAN_POINT('Ctrl Pts',(-0.208074432769725,0.00577550133242041,
-0.0102484889170709));
#32569=CARTESIAN_POINT('Ctrl Pts',(-0.208070985265817,0.00566934369931672,
-0.0102275720520985));
#32570=CARTESIAN_POINT('Ctrl Pts',(-0.208068443190351,0.005565699150329,
-0.0102053859028492));
#32571=CARTESIAN_POINT('Ctrl Pts',(-0.208063359039417,0.00535841005235356,
-0.0101610136043507));
#32572=CARTESIAN_POINT('Ctrl Pts',(-0.208061889044625,0.00516113746489649,
-0.0101118982807474));
#32573=CARTESIAN_POINT('Ctrl Pts',(-0.208065058125948,0.00495584654660638,
-0.0100533710595396));
#32574=CARTESIAN_POINT('Ctrl Pts',(-0.208068227207272,0.00475055562831626,
-0.00999484383833177));
#32575=CARTESIAN_POINT('Ctrl Pts',(-0.208076057362027,0.00453750921082217,
-0.00992590844977681));
#32576=CARTESIAN_POINT('Ctrl Pts',(-0.208088021136334,0.00434138309898768,
-0.0098549933278441));
#32577=CARTESIAN_POINT('Ctrl Pts',(-0.208090202592185,0.00430562177121669,
-0.00984206277568236));
#32578=CARTESIAN_POINT('Ctrl Pts',(-0.208092520725194,0.00427041573162259,
-0.00982908721933613));
#32579=CARTESIAN_POINT('Ctrl Pts',(-0.208095012174201,0.00423522751845692,
-0.00981587670658352));
#32580=CARTESIAN_POINT('Ctrl Pts',(-0.208099352661212,0.00417392424401928,
-0.00979286196341021));
#32581=CARTESIAN_POINT('Ctrl Pts',(-0.208104219179505,0.00411266917946915,
-0.00976914801243592));
#32582=CARTESIAN_POINT('Ctrl Pts',(-0.208109805460969,0.00404869361284434,
-0.00974354225869674));
#32583=CARTESIAN_POINT('Ctrl Pts',(-0.208118598280172,0.00394799593151293,
-0.00970323874649185));
#32584=CARTESIAN_POINT('Ctrl Pts',(-0.208129181422691,0.00384066403524311,
-0.00965798872173971));
#32585=CARTESIAN_POINT('Ctrl Pts',(-0.20813963760985,0.00374392741908631,
-0.00961520867146894));
#32586=CARTESIAN_POINT('Ctrl Pts',(-0.208150093797009,0.00364719080292951,
-0.00957242862119817));
#32587=CARTESIAN_POINT('Ctrl Pts',(-0.208160414835794,0.0035608696244637,
-0.0095325080696441));
#32588=CARTESIAN_POINT('Ctrl Pts',(-0.208172085514657,0.00346802947437642,
-0.00948776714366573));
#32589=CARTESIAN_POINT('Ctrl Pts',(-0.208177920854088,0.00342160939933278,
-0.00946539668067656));
#32590=CARTESIAN_POINT('Ctrl Pts',(-0.208184094105983,0.00337357425884607,
-0.00944179621201782));
#32591=CARTESIAN_POINT('Ctrl Pts',(-0.208191119790713,0.00332085407877749,
-0.00941523251609465));
#32592=CARTESIAN_POINT('Ctrl Pts',(-0.208198145475443,0.00326813389870892,
-0.00938866882017148));
#32593=CARTESIAN_POINT('Ctrl Pts',(-0.208206026523807,0.0032107980187599,
-0.00935900113952639));
#32594=CARTESIAN_POINT('Ctrl Pts',(-0.208212027615872,0.00316783533406424,
-0.00933634570123583));
#32595=CARTESIAN_POINT('Ctrl Pts',(-0.208218028707937,0.00312487264936858,
-0.00931369026294528));
#32596=CARTESIAN_POINT('Ctrl Pts',(-0.208222145445723,0.00309616936839642,
-0.00929826115868092));
#32597=CARTESIAN_POINT('Ctrl Pts',(-0.208227474789829,0.00305931342216926,
-0.00927819758755507));
#32598=CARTESIAN_POINT('Ctrl Pts',(-0.208232804133935,0.0030224574759421,
-0.00925813401642922));
#32599=CARTESIAN_POINT('Ctrl Pts',(-0.208239348542458,0.00297751550620315,
-0.00923331539613978));
#32600=CARTESIAN_POINT('Ctrl Pts',(-0.208246332691185,0.00293017920813089,
-0.00920656032436194));
#32601=CARTESIAN_POINT('Ctrl Pts',(-0.208260300947443,0.00283550689119974,
-0.00915305033862115));
#32602=CARTESIAN_POINT('Ctrl Pts',(-0.208276024103448,0.00273113766315477,
-0.00909199637027481));
#32603=CARTESIAN_POINT('Ctrl Pts',(-0.208294280514564,0.00261263945190299,
-0.00901864652104168));
#32604=CARTESIAN_POINT('',(-0.210295596274888,0.0026140133424121,-0.00905923595863249));
#32605=CARTESIAN_POINT('',(-0.209093405037848,0.00261320592886496,-0.00903485853905873));
#32606=CARTESIAN_POINT('',(-0.210295595172847,0.00261401461120539,-0.00905923137572964));
#32607=CARTESIAN_POINT('',(-0.208994544730133,0.00749998715785556,-0.0104310930514343));
#32608=CARTESIAN_POINT('Ctrl Pts',(-0.209093403325743,0.00261320712931955,
-0.00903485617757382));
#32609=CARTESIAN_POINT('Ctrl Pts',(-0.209075287163041,0.00273078952585028,
-0.00910776338190552));
#32610=CARTESIAN_POINT('Ctrl Pts',(-0.209051803949458,0.00288667849406431,
-0.009199304375793));
#32611=CARTESIAN_POINT('Ctrl Pts',(-0.209025633252355,0.00306682577244403,
-0.00929887864898022));
#32612=CARTESIAN_POINT('Ctrl Pts',(-0.209013059146288,0.0031547547392515,
-0.00934630105910322));
#32613=CARTESIAN_POINT('Ctrl Pts',(-0.20898960376665,0.00332609194728352,
-0.00943518469474632));
#32614=CARTESIAN_POINT('Ctrl Pts',(-0.208964997943753,0.00351864509772977,
-0.00952966373552731));
#32615=CARTESIAN_POINT('Ctrl Pts',(-0.208939169709193,0.00373601100206904,
-0.00963068732037389));
#32616=CARTESIAN_POINT('Ctrl Pts',(-0.20890779757303,0.0040564040909896,
-0.00976582079672488));
#32617=CARTESIAN_POINT('Ctrl Pts',(-0.208879854701294,0.00443241802618406,
-0.00990888934421124));
#32618=CARTESIAN_POINT('Ctrl Pts',(-0.208860246398243,0.00496217141417863,
-0.0100805792723302));
#32619=CARTESIAN_POINT('Ctrl Pts',(-0.208863596164369,0.00545882350114872,
-0.0102036806673025));
#32620=CARTESIAN_POINT('Ctrl Pts',(-0.208877129956472,0.0058835563834354,
-0.0102877866011816));
#32621=CARTESIAN_POINT('Ctrl Pts',(-0.208894583868389,0.00622875777336524,
-0.0103424460616012));
#32622=CARTESIAN_POINT('Ctrl Pts',(-0.20891006127027,0.00646408490751225,
-0.0103715160371586));
#32623=CARTESIAN_POINT('Ctrl Pts',(-0.208925621038673,0.00667921457685546,
-0.0103934454631171));
#32624=CARTESIAN_POINT('Ctrl Pts',(-0.208940687029599,0.0068717606575439,
-0.0104087544437141));
#32625=CARTESIAN_POINT('Ctrl Pts',(-0.208949572232236,0.0069796541515509,
-0.0104155521292759));
#32626=CARTESIAN_POINT('Ctrl Pts',(-0.208967069010806,0.00718754014657644,
-0.0104263074860422));
#32627=CARTESIAN_POINT('Ctrl Pts',(-0.208982640861888,0.00736577272041199,
-0.0104308238271735));
#32628=CARTESIAN_POINT('Ctrl Pts',(-0.208994544730133,0.00749998715785556,
-0.0104310930514343));
#32629=CARTESIAN_POINT('',(-0.209093329064524,0.0123896542664875,-0.00903307101714839));
#32630=CARTESIAN_POINT('Ctrl Pts',(-0.208994544893321,0.00749998899777242,
-0.0104310930551249));
#32631=CARTESIAN_POINT('Ctrl Pts',(-0.208982705999951,0.00763413924716552,
-0.010430825647875));
#32632=CARTESIAN_POINT('Ctrl Pts',(-0.208967210984714,0.00781236163842383,
-0.0104263159156353));
#32633=CARTESIAN_POINT('Ctrl Pts',(-0.208949777667206,0.00802044089467235,
-0.0104155518224826));
#32634=CARTESIAN_POINT('Ctrl Pts',(-0.20894091592414,0.008128513175511,
-0.0104087429341645));
#32635=CARTESIAN_POINT('Ctrl Pts',(-0.208925867851496,0.00832154817731363,
-0.0103933857795959));
#32636=CARTESIAN_POINT('Ctrl Pts',(-0.2089103172045,0.00853716190381373,
-0.0103713854659244));
#32637=CARTESIAN_POINT('Ctrl Pts',(-0.208894824616601,0.00877315451964924,
-0.0103421906059869));
#32638=CARTESIAN_POINT('Ctrl Pts',(-0.208877320801299,0.00911860720596101,
-0.010287412183992));
#32639=CARTESIAN_POINT('Ctrl Pts',(-0.208863666216549,0.00954338077158189,
-0.0102031599596682));
#32640=CARTESIAN_POINT('Ctrl Pts',(-0.208860009499849,0.0100372452975142,
-0.0100807397059271));
#32641=CARTESIAN_POINT('Ctrl Pts',(-0.208879360438715,0.0105697164377529,
-0.00990816362194018));
#32642=CARTESIAN_POINT('Ctrl Pts',(-0.208907270581647,0.0109464746140233,
-0.00976466308937504));
#32643=CARTESIAN_POINT('Ctrl Pts',(-0.208938752514271,0.0112678251463805,
-0.00962896977344753));
#32644=CARTESIAN_POINT('Ctrl Pts',(-0.208964570384985,0.0114845683051079,
-0.00952811433689885));
#32645=CARTESIAN_POINT('Ctrl Pts',(-0.208989211407872,0.011676914863895,
-0.00943365116768143));
#32646=CARTESIAN_POINT('Ctrl Pts',(-0.209012698322003,0.0118479783561038,
-0.00934483474583016));
#32647=CARTESIAN_POINT('Ctrl Pts',(-0.209025311339803,0.0119359028386126,
-0.0092973790754351));
#32648=CARTESIAN_POINT('Ctrl Pts',(-0.209051564781441,0.0121160329579314,
-0.009197736640123));
#32649=CARTESIAN_POINT('Ctrl Pts',(-0.209075138847902,0.0122719973881306,
-0.00910608251841254));
#32650=CARTESIAN_POINT('Ctrl Pts',(-0.209093329064524,0.0123896542664875,
-0.00903307101714839));
#32651=CARTESIAN_POINT('',(-0.210295214238121,0.0123883927066978,-0.00905773115010187));
#32652=CARTESIAN_POINT('',(-0.209093329180995,0.012389650612435,-0.00903306515726067));
#32653=CARTESIAN_POINT('',(-0.210194950898403,0.00749992261723267,-0.0104582232103857));
#32654=CARTESIAN_POINT('Ctrl Pts',(-0.210295213170193,0.0123883913778837,
-0.00905772874839569));
#32655=CARTESIAN_POINT('Ctrl Pts',(-0.210276926508739,0.0122701560805008,
-0.00913127718769082));
#32656=CARTESIAN_POINT('Ctrl Pts',(-0.210253280898068,0.0121138705649328,
-0.0092233032752109));
#32657=CARTESIAN_POINT('Ctrl Pts',(-0.210226997140627,0.0119339996830231,
-0.00932299508710102));
#32658=CARTESIAN_POINT('Ctrl Pts',(-0.210214556449654,0.0118476323651082,
-0.00936972564086559));
#32659=CARTESIAN_POINT('Ctrl Pts',(-0.210190786792116,0.011675476606061,
-0.00945931840457171));
#32660=CARTESIAN_POINT('Ctrl Pts',(-0.210165940955667,0.0114828988779726,
-0.00955406939877045));
#32661=CARTESIAN_POINT('Ctrl Pts',(-0.210139924515179,0.0112666251945686,
-0.00965491597491719));
#32662=CARTESIAN_POINT('Ctrl Pts',(-0.210107923610646,0.0109445348858429,
-0.00979115138124437));
#32663=CARTESIAN_POINT('Ctrl Pts',(-0.210079602583789,0.010570125790686,
-0.00993398760550886));
#32664=CARTESIAN_POINT('Ctrl Pts',(-0.210059675792393,0.0100388881977446,
-0.0101066833814956));
#32665=CARTESIAN_POINT('Ctrl Pts',(-0.210063174055939,0.00954342433810476,
-0.0102298110037676));
#32666=CARTESIAN_POINT('Ctrl Pts',(-0.210076870548468,0.00911815800952164,
-0.0103143191211735));
#32667=CARTESIAN_POINT('Ctrl Pts',(-0.210094543901722,0.00877197614815612,
-0.0103692938412502));
#32668=CARTESIAN_POINT('Ctrl Pts',(-0.210110144111369,0.00853643895794477,
-0.0103984590221526));
#32669=CARTESIAN_POINT('Ctrl Pts',(-0.210125789774286,0.00832128382381539,
-0.0104204528663754));
#32670=CARTESIAN_POINT('Ctrl Pts',(-0.210140952603249,0.00812844154018853,
-0.0104358217663535));
#32671=CARTESIAN_POINT('Ctrl Pts',(-0.210149784035195,0.00802163519906834,
-0.0104425708482792));
#32672=CARTESIAN_POINT('Ctrl Pts',(-0.210167324477964,0.0078138027892246,
-0.0104533816768634));
#32673=CARTESIAN_POINT('Ctrl Pts',(-0.210182969923806,0.00763494796693094,
-0.0104579535863278));
#32674=CARTESIAN_POINT('Ctrl Pts',(-0.210194950908977,0.00749992286606277,
-0.0104582232242195));
#32675=CARTESIAN_POINT('Ctrl Pts',(-0.210194950886893,0.00749992261823137,
-0.0104582232237183));
#32676=CARTESIAN_POINT('Ctrl Pts',(-0.210182901046186,0.00736469672032039,
-0.0104579497398173));
#32677=CARTESIAN_POINT('Ctrl Pts',(-0.210172422497674,0.00724538734312025,
-0.0104548136618292));
#32678=CARTESIAN_POINT('Ctrl Pts',(-0.210163059345851,0.00713634177118728,
-0.0104502645999214));
#32679=CARTESIAN_POINT('Ctrl Pts',(-0.21015837776708,0.00708181895191274,
-0.010447990067578));
#32680=CARTESIAN_POINT('Ctrl Pts',(-0.21015397623712,0.00702986313799503,
-0.0104453092305155));
#32681=CARTESIAN_POINT('Ctrl Pts',(-0.210150307054415,0.00698617324694343,
-0.0104427721414516));
#32682=CARTESIAN_POINT('Ctrl Pts',(-0.210146637871711,0.00694248335589182,
-0.0104402350523877));
#32683=CARTESIAN_POINT('Ctrl Pts',(-0.210143698071857,0.00690705261103447,
-0.0104379729864375));
#32684=CARTESIAN_POINT('Ctrl Pts',(-0.210139683756397,0.00685708316826792,
-0.0104343707561762));
#32685=CARTESIAN_POINT('Ctrl Pts',(-0.210135669440937,0.00680711372550136,
-0.0104307685259148));
#32686=CARTESIAN_POINT('Ctrl Pts',(-0.210130585779747,0.0067426214917892,
-0.010425597011124));
#32687=CARTESIAN_POINT('Ctrl Pts',(-0.210126084760253,0.0066834609985755,
-0.0104202141619642));
#32688=CARTESIAN_POINT('Ctrl Pts',(-0.21012158374076,0.00662430050536181,
-0.0104148313128045));
#32689=CARTESIAN_POINT('Ctrl Pts',(-0.210117662082953,0.00657045706783954,
-0.0104093827532257));
#32690=CARTESIAN_POINT('Ctrl Pts',(-0.210114007159558,0.00651881912761199,
-0.010403757618497));
#32691=CARTESIAN_POINT('Ctrl Pts',(-0.210106697312767,0.0064155432471569,
-0.0103925073490395));
#32692=CARTESIAN_POINT('Ctrl Pts',(-0.21010045146602,0.00632108335076086,
-0.0103806806744025));
#32693=CARTESIAN_POINT('Ctrl Pts',(-0.21009441614451,0.0062164869318611,
-0.0103658243556338));
#32694=CARTESIAN_POINT('Ctrl Pts',(-0.210088380822999,0.00611189051296133,
-0.0103509680368652));
#32695=CARTESIAN_POINT('Ctrl Pts',(-0.21008256450481,0.00599720823621759,
-0.0103327046426888));
#32696=CARTESIAN_POINT('Ctrl Pts',(-0.210077972266854,0.00588684360592312,
-0.0103129973582448));
#32697=CARTESIAN_POINT('Ctrl Pts',(-0.210073380028898,0.00577647897562865,
-0.0102932900738008));
#32698=CARTESIAN_POINT('Ctrl Pts',(-0.210070007557372,0.0056703922517969,
-0.0102723324599391));
#32699=CARTESIAN_POINT('Ctrl Pts',(-0.210067545901141,0.00556669841361688,
-0.0102500722841563));
#32700=CARTESIAN_POINT('Ctrl Pts',(-0.210062622588677,0.00535931073725686,
-0.0102055519325907));
#32701=CARTESIAN_POINT('Ctrl Pts',(-0.210061335223825,0.0051614609530984,
-0.0101561444787735));
#32702=CARTESIAN_POINT('Ctrl Pts',(-0.210064745705541,0.00495583019273618,
-0.0100973149994839));
#32703=CARTESIAN_POINT('Ctrl Pts',(-0.210068156187256,0.00475019943237396,
-0.0100384855201942));
#32704=CARTESIAN_POINT('Ctrl Pts',(-0.210076286548203,0.00453705079573793,
-0.00996923671869086));
#32705=CARTESIAN_POINT('Ctrl Pts',(-0.210088476640698,0.00434154248511133,
-0.00989828957217904));
#32706=CARTESIAN_POINT('Ctrl Pts',(-0.210090891234621,0.00430281651325807,
-0.0098842364754586));
#32707=CARTESIAN_POINT('Ctrl Pts',(-0.210093464184377,0.00426477369336213,
-0.00987014248265051));
#32708=CARTESIAN_POINT('Ctrl Pts',(-0.210096245101527,0.00422668528530898,
-0.00985574713506132));
#32709=CARTESIAN_POINT('Ctrl Pts',(-0.210100483923172,0.00416862891046109,
-0.00983380498157101));
#32710=CARTESIAN_POINT('Ctrl Pts',(-0.210105205925359,0.00411046210709376,
-0.00981117299353445));
#32711=CARTESIAN_POINT('Ctrl Pts',(-0.210110586800972,0.00404967136736714,
-0.00978675728446723));
#32712=CARTESIAN_POINT('Ctrl Pts',(-0.210119497848536,0.00394899831486044,
-0.00974632342937738));
#32713=CARTESIAN_POINT('Ctrl Pts',(-0.210130223391488,0.00384123851543098,
-0.00970072961136996));
#32714=CARTESIAN_POINT('Ctrl Pts',(-0.210140763295786,0.00374438794995144,
-0.00965773465427805));
#32715=CARTESIAN_POINT('Ctrl Pts',(-0.210151303200083,0.00364753738447191,
-0.00961473969718614));
#32716=CARTESIAN_POINT('Ctrl Pts',(-0.210161648934644,0.0035614083089465,
-0.00957474870491259));
#32717=CARTESIAN_POINT('Ctrl Pts',(-0.21017334863502,0.00346865401672289,
-0.00952987258160654));
#32718=CARTESIAN_POINT('Ctrl Pts',(-0.210179198485208,0.00342227687061109,
-0.00950743451995351));
#32719=CARTESIAN_POINT('Ctrl Pts',(-0.210185387361134,0.00337425893918527,
-0.00948374876968531));
#32720=CARTESIAN_POINT('Ctrl Pts',(-0.210192421901137,0.00332158610454488,
-0.00945710265711653));
#32721=CARTESIAN_POINT('Ctrl Pts',(-0.21019945644114,0.00326891326990449,
-0.00943045654454775));
#32722=CARTESIAN_POINT('Ctrl Pts',(-0.210207339569676,0.00321165486863207,
-0.00940070981763388));
#32723=CARTESIAN_POINT('Ctrl Pts',(-0.210213348898254,0.00316869390487509,
-0.00937796337721139));
#32724=CARTESIAN_POINT('Ctrl Pts',(-0.210219358226833,0.00312573294111812,
-0.0093552169367889));
#32725=CARTESIAN_POINT('Ctrl Pts',(-0.210223489356426,0.00309695532981657,
-0.00933968458140724));
#32726=CARTESIAN_POINT('Ctrl Pts',(-0.210228826901985,0.00306007614923581,
-0.00931952500679846));
#32727=CARTESIAN_POINT('Ctrl Pts',(-0.210234164447545,0.00302319696865506,
-0.00929936543218968));
#32728=CARTESIAN_POINT('Ctrl Pts',(-0.210240710870133,0.00297828310429532,
-0.00927445811629131));
#32729=CARTESIAN_POINT('Ctrl Pts',(-0.21024769392878,0.00293099466147187,
-0.00924761742954498));
#32730=CARTESIAN_POINT('Ctrl Pts',(-0.210261660006699,0.00283641804245922,
-0.00919393620739263));
#32731=CARTESIAN_POINT('Ctrl Pts',(-0.210277368573352,0.00273222337063102,
-0.00913272268177796));
#32732=CARTESIAN_POINT('Ctrl Pts',(-0.210295594897407,0.00261401179386915,
-0.00905923810805346));
#32733=CARTESIAN_POINT('',(-0.194290184740893,0.00259891003340495,-0.00873469929757838));
#32734=CARTESIAN_POINT('',(-0.193089420205241,0.00259786897112515,-0.0087106653108531));
#32735=CARTESIAN_POINT('',(-0.194290183626354,0.00259891156440595,-0.0087346940896404));
#32736=CARTESIAN_POINT('',(-0.193001281131681,0.00750326240626864,-0.0100696314931372));
#32737=CARTESIAN_POINT('Ctrl Pts',(-0.193089417595358,0.00259787021585085,
-0.00871066257746708));
#32738=CARTESIAN_POINT('Ctrl Pts',(-0.193071520109316,0.00271737164203461,
-0.0087821698526072));
#32739=CARTESIAN_POINT('Ctrl Pts',(-0.193048393887614,0.00287523277332858,
-0.00887164272095586));
#32740=CARTESIAN_POINT('Ctrl Pts',(-0.193022765375995,0.003056792294895,
-0.00896856117898018));
#32741=CARTESIAN_POINT('Ctrl Pts',(-0.193010614506598,0.00314422540462343,
-0.00901413520726188));
#32742=CARTESIAN_POINT('Ctrl Pts',(-0.192987664968883,0.00331741658030568,
-0.00910097335122508));
#32743=CARTESIAN_POINT('Ctrl Pts',(-0.192963930400356,0.00351035925151311,
-0.00919259941855622));
#32744=CARTESIAN_POINT('Ctrl Pts',(-0.192928202941401,0.00382656270556843,
-0.00933427847044191));
#32745=CARTESIAN_POINT('Ctrl Pts',(-0.192887551610886,0.00433451593535043,
-0.00953365458093566));
#32746=CARTESIAN_POINT('Ctrl Pts',(-0.192868658917011,0.00496327969818103,
-0.0097289927725957));
#32747=CARTESIAN_POINT('Ctrl Pts',(-0.192873508297919,0.00544626414837375,
-0.00984654654740827));
#32748=CARTESIAN_POINT('Ctrl Pts',(-0.192886802235328,0.00582975166215757,
-0.00992002089963444));
#32749=CARTESIAN_POINT('Ctrl Pts',(-0.192896729854821,0.00604524879215619,
-0.00995568577848646));
#32750=CARTESIAN_POINT('Ctrl Pts',(-0.192907093637035,0.00623542839851351,
-0.00998317555330493));
#32751=CARTESIAN_POINT('Ctrl Pts',(-0.192913112747442,0.00633340690348751,
-0.00999574270740675));
#32752=CARTESIAN_POINT('Ctrl Pts',(-0.192924889956533,0.00651567014394898,
-0.0100174697902547));
#32753=CARTESIAN_POINT('Ctrl Pts',(-0.192949223880671,0.00685826224465497,
-0.0100505308306341));
#32754=CARTESIAN_POINT('Ctrl Pts',(-0.192978374135323,0.0072276364985116,
-0.0100692092264082));
#32755=CARTESIAN_POINT('Ctrl Pts',(-0.193001281131681,0.00750326240626864,
-0.0100696314931372));
#32756=CARTESIAN_POINT('',(-0.193087908899462,0.0124055063694067,-0.00870860190565759));
#32757=CARTESIAN_POINT('Ctrl Pts',(-0.193001281190772,0.00750326311727974,
-0.0100696314942265));
#32758=CARTESIAN_POINT('Ctrl Pts',(-0.192978210832965,0.00777866827952415,
-0.0100690146904097));
#32759=CARTESIAN_POINT('Ctrl Pts',(-0.192948830761218,0.008147788785168,
-0.0100501046519563));
#32760=CARTESIAN_POINT('Ctrl Pts',(-0.19292426502221,0.00849020464720827,
-0.0100168410848431));
#32761=CARTESIAN_POINT('Ctrl Pts',(-0.192912354662967,0.0086724362908473,
-0.00999500023200311));
#32762=CARTESIAN_POINT('Ctrl Pts',(-0.192906265760605,0.00877033231534428,
-0.00998238250180546));
#32763=CARTESIAN_POINT('Ctrl Pts',(-0.192895737826648,0.00896075376316357,
-0.00995473360888943));
#32764=CARTESIAN_POINT('Ctrl Pts',(-0.192885628503617,0.00917632356298331,
-0.00991891150020981));
#32765=CARTESIAN_POINT('Ctrl Pts',(-0.192872013216822,0.00955987628497917,
-0.00984514265529782));
#32766=CARTESIAN_POINT('Ctrl Pts',(-0.192866715571841,0.0100411414659507,
-0.00972773826890768));
#32767=CARTESIAN_POINT('Ctrl Pts',(-0.192885220267161,0.0106715812642055,
-0.0095314555019776));
#32768=CARTESIAN_POINT('Ctrl Pts',(-0.19292571236353,0.0111775914430577,
-0.00933246725911518));
#32769=CARTESIAN_POINT('Ctrl Pts',(-0.19296159843528,0.011493722472007,
-0.00919066330427862));
#32770=CARTESIAN_POINT('Ctrl Pts',(-0.192985458260683,0.0116864938887278,
-0.00909901104930757));
#32771=CARTESIAN_POINT('Ctrl Pts',(-0.193008563102243,0.0118596393209108,
-0.00901210051369803));
#32772=CARTESIAN_POINT('Ctrl Pts',(-0.193020768112869,0.0119467998890343,
-0.00896662056560247));
#32773=CARTESIAN_POINT('Ctrl Pts',(-0.19304656776878,0.0121281882483118,
-0.00886970079861718));
#32774=CARTESIAN_POINT('Ctrl Pts',(-0.193069867896834,0.0122859955607241,
-0.00878017895815907));
#32775=CARTESIAN_POINT('Ctrl Pts',(-0.193087908899462,0.0124055063694067,
-0.00870860190565759));
#32776=CARTESIAN_POINT('',(-0.194289761930591,0.0124043673425885,-0.00873272050667267));
#32777=CARTESIAN_POINT('',(-0.193087909024505,0.0124055025124637,-0.00870859549681853));
#32778=CARTESIAN_POINT('',(-0.194201350807346,0.00750361794929087,-0.0100967539450016));
#32779=CARTESIAN_POINT('Ctrl Pts',(-0.194289760087428,0.0124043660030698,
-0.00873271781171757));
#32780=CARTESIAN_POINT('Ctrl Pts',(-0.194271557560553,0.0122841918170491,
-0.00880489926922499));
#32781=CARTESIAN_POINT('Ctrl Pts',(-0.194255924507852,0.0121786813739423,
-0.00886479899873608));
#32782=CARTESIAN_POINT('Ctrl Pts',(-0.194242077346723,0.0120832044547145,
-0.00891719261876354));
#32783=CARTESIAN_POINT('Ctrl Pts',(-0.194235153737023,0.0120354657942032,
-0.00894338953902113));
#32784=CARTESIAN_POINT('Ctrl Pts',(-0.19422867761032,0.0119902062506205,
-0.00896765903205084));
#32785=CARTESIAN_POINT('Ctrl Pts',(-0.194223429540068,0.0119532774812538,
-0.00898718409458635));
#32786=CARTESIAN_POINT('Ctrl Pts',(-0.194218181469815,0.0119163487118872,
-0.00900670915712187));
#32787=CARTESIAN_POINT('Ctrl Pts',(-0.194214159033718,0.0118878153593697,
-0.00902161018266591));
#32788=CARTESIAN_POINT('Ctrl Pts',(-0.194208244185811,0.0118446120395155,
-0.00904374737452372));
#32789=CARTESIAN_POINT('Ctrl Pts',(-0.194202329337904,0.0118014087196613,
-0.00906588456638152));
#32790=CARTESIAN_POINT('Ctrl Pts',(-0.194194526447476,0.011743424062956,
-0.00909504257821868));
#32791=CARTESIAN_POINT('Ctrl Pts',(-0.194187615787879,0.0116903232532915,
-0.00912104827855453));
#32792=CARTESIAN_POINT('Ctrl Pts',(-0.194180705128282,0.011637222443627,
-0.00914705397889038));
#32793=CARTESIAN_POINT('Ctrl Pts',(-0.194174683690572,0.0115890759491422,
-0.00917005356254145));
#32794=CARTESIAN_POINT('Ctrl Pts',(-0.19416894561689,0.0115419790292713,
-0.00919212077082414));
#32795=CARTESIAN_POINT('Ctrl Pts',(-0.194157469469527,0.0114477851895296,
-0.00923625518738952));
#32796=CARTESIAN_POINT('Ctrl Pts',(-0.194147127099538,0.0113577901971368,
-0.00927664711652409));
#32797=CARTESIAN_POINT('Ctrl Pts',(-0.194137479955741,0.0112640004553303,
-0.00931699556663056));
#32798=CARTESIAN_POINT('Ctrl Pts',(-0.194119369196314,0.0110879272582998,
-0.00939274244969722));
#32799=CARTESIAN_POINT('Ctrl Pts',(-0.194103719839443,0.0108982588085448,
-0.00946782936055712));
#32800=CARTESIAN_POINT('Ctrl Pts',(-0.194092456058785,0.0107050027776539,
-0.00953690472670395));
#32801=CARTESIAN_POINT('Ctrl Pts',(-0.194091719976914,0.0106923736023294,
-0.00954141876388897));
#32802=CARTESIAN_POINT('Ctrl Pts',(-0.194091002623868,0.0106797294941558,
-0.00954590800925234));
#32803=CARTESIAN_POINT('Ctrl Pts',(-0.194090304536643,0.010667073418177,
-0.00955037138673742));
#32804=CARTESIAN_POINT('Ctrl Pts',(-0.194078924076026,0.0104607496681452,
-0.00962313491803084));
#32805=CARTESIAN_POINT('Ctrl Pts',(-0.194072662679182,0.0102511157066591,
-0.00968879287497787));
#32806=CARTESIAN_POINT('Ctrl Pts',(-0.194070598391485,0.0100500588759178,
-0.00974474285896947));
#32807=CARTESIAN_POINT('Ctrl Pts',(-0.194068534103787,0.00984900204517659,
-0.00980069284296108));
#32808=CARTESIAN_POINT('Ctrl Pts',(-0.194070648874117,0.00965676744371061,
-0.00984776204665912));
#32809=CARTESIAN_POINT('Ctrl Pts',(-0.194076567237035,0.00944655516440553,
-0.00989189619201452));
#32810=CARTESIAN_POINT('Ctrl Pts',(-0.194079526418495,0.009341449024753,
-0.00991396326469222));
#32811=CARTESIAN_POINT('Ctrl Pts',(-0.19408344128464,0.00923180464711715,
-0.0099350813053663));
#32812=CARTESIAN_POINT('Ctrl Pts',(-0.194088139064564,0.00912335820941506,
-0.00995400868302609));
#32813=CARTESIAN_POINT('Ctrl Pts',(-0.194090487954526,0.00906913499056402,
-0.00996347237185598));
#32814=CARTESIAN_POINT('Ctrl Pts',(-0.194093031522886,0.0090152195964702,
-0.00997243543958158));
#32815=CARTESIAN_POINT('Ctrl Pts',(-0.194096071829517,0.00895644906944938,
-0.00998163393309338));
#32816=CARTESIAN_POINT('Ctrl Pts',(-0.194099112136148,0.00889767854242856,
-0.00999083242660519));
#32817=CARTESIAN_POINT('Ctrl Pts',(-0.19410265263027,0.00883402824504551,
-0.0100001121226521));
#32818=CARTESIAN_POINT('Ctrl Pts',(-0.194105435828594,0.00878603171415256,
-0.0100067460210346));
#32819=CARTESIAN_POINT('Ctrl Pts',(-0.194108219026918,0.0087380351832596,
-0.010013379919417));
#32820=CARTESIAN_POINT('Ctrl Pts',(-0.194110240099272,0.00870572131166556,
-0.0100175833341403));
#32821=CARTESIAN_POINT('Ctrl Pts',(-0.194112740675617,0.00866684824967951,
-0.0100224633622123));
#32822=CARTESIAN_POINT('Ctrl Pts',(-0.194115241251962,0.00862797518769346,
-0.0100273433902844));
#32823=CARTESIAN_POINT('Ctrl Pts',(-0.194118223924051,0.00858252925364297,
-0.0100327846897015));
#32824=CARTESIAN_POINT('Ctrl Pts',(-0.194121383971891,0.00853594848017848,
-0.0100379828379812));
#32825=CARTESIAN_POINT('Ctrl Pts',(-0.194127704067573,0.0084427869332495,
-0.0100483791345406));
#32826=CARTESIAN_POINT('Ctrl Pts',(-0.194134730458665,0.00834509945083744,
-0.0100579452337754));
#32827=CARTESIAN_POINT('Ctrl Pts',(-0.194142685912192,0.00823888424106794,
-0.0100664533359255));
#32828=CARTESIAN_POINT('Ctrl Pts',(-0.194158596817806,0.00802645384076312,
-0.010083469538685));
#32829=CARTESIAN_POINT('Ctrl Pts',(-0.194178226891711,0.00777991114448582,
-0.0100961249381803));
#32830=CARTESIAN_POINT('Ctrl Pts',(-0.194201351177526,0.00750361798025657,
-0.0100967539377924));
#32831=CARTESIAN_POINT('Ctrl Pts',(-0.194201351183807,0.00750361790520686,
-0.0100967539379632));
#32832=CARTESIAN_POINT('Ctrl Pts',(-0.1941784036171,0.00722720869209292,
-0.0100963417181278));
#32833=CARTESIAN_POINT('Ctrl Pts',(-0.19415892327886,0.00698052577256948,
-0.0100838676069228));
#32834=CARTESIAN_POINT('Ctrl Pts',(-0.194143133295327,0.00676793924744402,
-0.0100669960050715));
#32835=CARTESIAN_POINT('Ctrl Pts',(-0.194135238303561,0.00666164598488129,
-0.0100585602041459));
#32836=CARTESIAN_POINT('Ctrl Pts',(-0.194128265168655,0.0065638764940593,
-0.0100490573230068));
#32837=CARTESIAN_POINT('Ctrl Pts',(-0.194121992959818,0.00647062775368298,
-0.010038718058705));
#32838=CARTESIAN_POINT('Ctrl Pts',(-0.194118856855399,0.00642400338349483,
-0.0100335484265541));
#32839=CARTESIAN_POINT('Ctrl Pts',(-0.194115896785519,0.00637851253535828,
-0.0100281340490187));
#32840=CARTESIAN_POINT('Ctrl Pts',(-0.194113414944245,0.00633959584073668,
-0.0100232759418804));
#32841=CARTESIAN_POINT('Ctrl Pts',(-0.194110933102972,0.00630067914611507,
-0.0100184178347421));
#32842=CARTESIAN_POINT('Ctrl Pts',(-0.194108926894298,0.00626832298245323,
-0.0100142315214387));
#32843=CARTESIAN_POINT('Ctrl Pts',(-0.194106165030128,0.00622027508395902,
-0.0100076237304598));
#32844=CARTESIAN_POINT('Ctrl Pts',(-0.194103403165958,0.0061722271854648,
-0.010001015939481));
#32845=CARTESIAN_POINT('Ctrl Pts',(-0.194099890484652,0.00610851634466332,
-0.00999177100812512));
#32846=CARTESIAN_POINT('Ctrl Pts',(-0.194096874427416,0.00604969047262855,
-0.00998260367179467));
#32847=CARTESIAN_POINT('Ctrl Pts',(-0.194093858370181,0.00599086460059379,
-0.00997343633546422));
#32848=CARTESIAN_POINT('Ctrl Pts',(-0.194091335481784,0.00593689912204222,
-0.00996450107264417));
#32849=CARTESIAN_POINT('Ctrl Pts',(-0.194089006191789,0.00588262685159719,
-0.00995506487481372));
#32850=CARTESIAN_POINT('Ctrl Pts',(-0.194084347611799,0.00577408231070712,
-0.00993619247915282));
#32851=CARTESIAN_POINT('Ctrl Pts',(-0.194080467634741,0.00566434390043965,
-0.00991512777454408));
#32852=CARTESIAN_POINT('Ctrl Pts',(-0.194077536821785,0.00555915963491658,
-0.00989311214193168));
#32853=CARTESIAN_POINT('Ctrl Pts',(-0.194071675195875,0.00534879110387044,
-0.00984908087670686));
#32854=CARTESIAN_POINT('Ctrl Pts',(-0.194069591003107,0.00515646375103136,
-0.00980211034402297));
#32855=CARTESIAN_POINT('Ctrl Pts',(-0.194071666486789,0.00495527116389036,
-0.00974624901355076));
#32856=CARTESIAN_POINT('Ctrl Pts',(-0.19407374197047,0.00475407857674936,
-0.00969038768307855));
#32857=CARTESIAN_POINT('Ctrl Pts',(-0.194079995256821,0.00454426636275194,
-0.00962480503332397));
#32858=CARTESIAN_POINT('Ctrl Pts',(-0.19409134999362,0.00433775402585064,
-0.00955210057146974));
#32859=CARTESIAN_POINT('Ctrl Pts',(-0.194092134644621,0.00432348331974186,
-0.00954707644543695));
#32860=CARTESIAN_POINT('Ctrl Pts',(-0.194092943662198,0.00430922775133401,
-0.00954201941471674));
#32861=CARTESIAN_POINT('Ctrl Pts',(-0.194093776278021,0.0042949915867727,
-0.0095369310292579));
#32862=CARTESIAN_POINT('Ctrl Pts',(-0.194104992501138,0.00410321526746275,
-0.00946838505043592));
#32863=CARTESIAN_POINT('Ctrl Pts',(-0.194120491089499,0.00391504859850539,
-0.00939394859554914));
#32864=CARTESIAN_POINT('Ctrl Pts',(-0.194138393795351,0.00374031506574058,
-0.00931887929995244));
#32865=CARTESIAN_POINT('Ctrl Pts',(-0.194148009635601,0.00364646278713287,
-0.00927855833617551));
#32866=CARTESIAN_POINT('Ctrl Pts',(-0.194158315848446,0.0035564231592988,
-0.00923819860106988));
#32867=CARTESIAN_POINT('Ctrl Pts',(-0.194169754463968,0.0034621532928448,
-0.00919408287663085));
#32868=CARTESIAN_POINT('Ctrl Pts',(-0.194175473771729,0.0034150183596178,
-0.00917202501441133));
#32869=CARTESIAN_POINT('Ctrl Pts',(-0.194181476100521,0.0033668260329514,
-0.00914903136473678));
#32870=CARTESIAN_POINT('Ctrl Pts',(-0.194188366540259,0.00331365880698595,
-0.0091230233186226));
#32871=CARTESIAN_POINT('Ctrl Pts',(-0.194195256979996,0.0032604915810205,
-0.00909701527250842));
#32872=CARTESIAN_POINT('Ctrl Pts',(-0.194203038554286,0.00320242016548369,
-0.00906784595621892));
#32873=CARTESIAN_POINT('Ctrl Pts',(-0.194208933111204,0.00315918193490789,
-0.00904571485433129));
#32874=CARTESIAN_POINT('Ctrl Pts',(-0.194214827668121,0.00311594370433209,
-0.00902358375244366));
#32875=CARTESIAN_POINT('Ctrl Pts',(-0.194218830819376,0.00308742695170646,
-0.00900870709690693));
#32876=CARTESIAN_POINT('Ctrl Pts',(-0.194224058435703,0.0030504868152752,
-0.00898919675401521));
#32877=CARTESIAN_POINT('Ctrl Pts',(-0.19422928605203,0.00301354667884394,
-0.00896968641112348));
#32878=CARTESIAN_POINT('Ctrl Pts',(-0.194235740564667,0.00296824795435302,
-0.00894542157318903));
#32879=CARTESIAN_POINT('Ctrl Pts',(-0.194242641940655,0.00292046237651401,
-0.00891922568503443));
#32880=CARTESIAN_POINT('Ctrl Pts',(-0.194256444653212,0.00282489149378098,
-0.00886683405835275));
#32881=CARTESIAN_POINT('Ctrl Pts',(-0.194272030765503,0.00271925573908181,
-0.0088069226691576));
#32882=CARTESIAN_POINT('Ctrl Pts',(-0.194290183336391,0.00259890843439175,
-0.00873470160911481));
#32883=CARTESIAN_POINT('',(-0.214298629851053,0.00261569271051004,-0.00914002418897946));
#32884=CARTESIAN_POINT('',(-0.213096481634368,0.00261552650153193,-0.00911594495457058));
#32885=CARTESIAN_POINT('',(-0.214298628831032,0.00261569386335166,-0.00914002001605525));
#32886=CARTESIAN_POINT('',(-0.212993232294335,0.0075001970402567,-0.0105214666975835));
#32887=CARTESIAN_POINT('Ctrl Pts',(-0.21309648029403,0.00261552762645514,
-0.00911594282477631));
#32888=CARTESIAN_POINT('Ctrl Pts',(-0.213078430112302,0.00273245414128495,
-0.00918906108432047));
#32889=CARTESIAN_POINT('Ctrl Pts',(-0.213054995693056,0.00288771851498538,
-0.0092810210476475));
#32890=CARTESIAN_POINT('Ctrl Pts',(-0.21302880695443,0.00306756366400709,
-0.00938127103149015));
#32891=CARTESIAN_POINT('Ctrl Pts',(-0.213016143252952,0.00315590799634756,
-0.00942930968362297));
#32892=CARTESIAN_POINT('Ctrl Pts',(-0.212992660269334,0.003326786139957,
-0.00951867735662309));
#32893=CARTESIAN_POINT('Ctrl Pts',(-0.21296791706596,0.0035191922936703,
-0.00961383729171739));
#32894=CARTESIAN_POINT('Ctrl Pts',(-0.212941949550837,0.00373557892325479,
-0.00971524319924369));
#32895=CARTESIAN_POINT('Ctrl Pts',(-0.212909725136388,0.00405845154500544,
-0.0098524131824994));
#32896=CARTESIAN_POINT('Ctrl Pts',(-0.212881015567256,0.00443089820167271,
-0.00999509170778643));
#32897=CARTESIAN_POINT('Ctrl Pts',(-0.212859850566388,0.00496168574833953,
-0.0101685244860136));
#32898=CARTESIAN_POINT('Ctrl Pts',(-0.212862265028007,0.00545958577045319,
-0.0102927065215424));
#32899=CARTESIAN_POINT('Ctrl Pts',(-0.212875146008631,0.0058842422052161,
-0.0103772957691917));
#32900=CARTESIAN_POINT('Ctrl Pts',(-0.212892085155633,0.00622799509361403,
-0.0104320981575625));
#32901=CARTESIAN_POINT('Ctrl Pts',(-0.212907529886643,0.00646460503686682,
-0.0104615313468541));
#32902=CARTESIAN_POINT('Ctrl Pts',(-0.212923143490097,0.00667948099614421,
-0.0104835687423165));
#32903=CARTESIAN_POINT('Ctrl Pts',(-0.212938368518025,0.00687187013964289,
-0.010498964812566));
#32904=CARTESIAN_POINT('Ctrl Pts',(-0.212947295699535,0.00697855992041427,
-0.010505738088064));
#32905=CARTESIAN_POINT('Ctrl Pts',(-0.212965076377683,0.00718624194132101,
-0.0105165930048715));
#32906=CARTESIAN_POINT('Ctrl Pts',(-0.212981009572996,0.00736511552634172,
-0.0105211933895291));
#32907=CARTESIAN_POINT('Ctrl Pts',(-0.212993232294335,0.0075001970402567,
-0.0105214666975835));
#32908=CARTESIAN_POINT('',(-0.21309504262537,0.0123853440218161,-0.00911536634304113));
#32909=CARTESIAN_POINT('Ctrl Pts',(-0.212993232518998,0.00750019952315436,
-0.0105214667026068));
#32910=CARTESIAN_POINT('Ctrl Pts',(-0.212981061653907,0.00763520971852247,
-0.0105211886623164));
#32911=CARTESIAN_POINT('Ctrl Pts',(-0.212965184756485,0.00781408229962534,
-0.0105165863100814));
#32912=CARTESIAN_POINT('Ctrl Pts',(-0.212947437584023,0.00802198453578981,
-0.0105057108565127));
#32913=CARTESIAN_POINT('Ctrl Pts',(-0.212938511769387,0.00812893139569496,
-0.0104989147874754));
#32914=CARTESIAN_POINT('Ctrl Pts',(-0.212923276308821,0.00832174278934911,
-0.010483464014518));
#32915=CARTESIAN_POINT('Ctrl Pts',(-0.212907629501198,0.00853704573621329,
-0.0104613497492999));
#32916=CARTESIAN_POINT('Ctrl Pts',(-0.21289211318811,0.00877418254637154,
-0.0104317971122061));
#32917=CARTESIAN_POINT('Ctrl Pts',(-0.212875016315916,0.00911806924975992,
-0.0103768834350925));
#32918=CARTESIAN_POINT('Ctrl Pts',(-0.212861881278273,0.0095425186563387,
-0.0102921897492956));
#32919=CARTESIAN_POINT('Ctrl Pts',(-0.212858990654386,0.0100372170775486,
-0.0101688017016576));
#32920=CARTESIAN_POINT('Ctrl Pts',(-0.212879702219452,0.0105702101667965,
-0.00999470542822341));
#32921=CARTESIAN_POINT('Ctrl Pts',(-0.212908308029409,0.0109434177167843,
-0.00985163308745656));
#32922=CARTESIAN_POINT('Ctrl Pts',(-0.212940513214306,0.011266746511133,
-0.00971416489421704));
#32923=CARTESIAN_POINT('Ctrl Pts',(-0.212966407470973,0.0114824337087737,
-0.00961301708601186));
#32924=CARTESIAN_POINT('Ctrl Pts',(-0.212991121561868,0.0116744958348988,
-0.00951798776478114));
#32925=CARTESIAN_POINT('Ctrl Pts',(-0.213014577453931,0.0118449807481599,
-0.00942879779089917));
#32926=CARTESIAN_POINT('Ctrl Pts',(-0.213027252935726,0.0119332823145633,
-0.00938077251897972));
#32927=CARTESIAN_POINT('Ctrl Pts',(-0.213053470144755,0.012113045655154,
-0.00928054494139649));
#32928=CARTESIAN_POINT('Ctrl Pts',(-0.213076951250776,0.0122683567168384,
-0.00918853996606421));
#32929=CARTESIAN_POINT('Ctrl Pts',(-0.21309504262537,0.0123853440218161,
-0.00911536634304113));
#32930=CARTESIAN_POINT('',(-0.214296931244579,0.0123846052054983,-0.00913980847830293));
#32931=CARTESIAN_POINT('',(-0.213095042734061,0.0123853405995523,-0.00911536089812739));
#32932=CARTESIAN_POINT('',(-0.214193730601714,0.00750035257190656,-0.0105485989207064));
#32933=CARTESIAN_POINT('Ctrl Pts',(-0.214296930448721,0.0123846039446203,
-0.0091398062710915));
#32934=CARTESIAN_POINT('Ctrl Pts',(-0.214278721771776,0.0122668959833074,
-0.00921361292919597));
#32935=CARTESIAN_POINT('Ctrl Pts',(-0.214263005072048,0.0121629773635556,
-0.00927519657157546));
#32936=CARTESIAN_POINT('Ctrl Pts',(-0.21424900854385,0.0120685001738844,
-0.00932927853847729));
#32937=CARTESIAN_POINT('Ctrl Pts',(-0.214242010247462,0.0120212613610989,
-0.00935631964669018));
#32938=CARTESIAN_POINT('Ctrl Pts',(-0.214235443009659,0.0119763528144547,
-0.00938143520479044));
#32939=CARTESIAN_POINT('Ctrl Pts',(-0.214230075611608,0.0119393872627358,
-0.00940181100398319));
#32940=CARTESIAN_POINT('Ctrl Pts',(-0.214224708213557,0.0119024217110168,
-0.00942218680317593));
#32941=CARTESIAN_POINT('Ctrl Pts',(-0.214220538178746,0.011873466807046,
-0.00943794372517518));
#32942=CARTESIAN_POINT('Ctrl Pts',(-0.214214494776839,0.0118304283104676,
-0.00946091659507249));
#32943=CARTESIAN_POINT('Ctrl Pts',(-0.214208451374932,0.0117873898138891,
-0.00948388946496979));
#32944=CARTESIAN_POINT('Ctrl Pts',(-0.214200539028783,0.0117301524518821,
-0.00951386398846413));
#32945=CARTESIAN_POINT('Ctrl Pts',(-0.214193469042124,0.0116774632250146,
-0.00954073002665238));
#32946=CARTESIAN_POINT('Ctrl Pts',(-0.214186399055465,0.011624773998147,
-0.00956759606484063));
#32947=CARTESIAN_POINT('Ctrl Pts',(-0.214180168492324,0.0115767028581632,
-0.00959149404375981));
#32948=CARTESIAN_POINT('Ctrl Pts',(-0.21417427591499,0.0115302697149787,
-0.00961413300801649));
#32949=CARTESIAN_POINT('Ctrl Pts',(-0.214162490760321,0.0114374034286095,
-0.00965941093652985));
#32950=CARTESIAN_POINT('Ctrl Pts',(-0.214152055361112,0.0113511529333559,
-0.00969976052723715));
#32951=CARTESIAN_POINT('Ctrl Pts',(-0.214141387483464,0.0112541405327512,
-0.00974314176318902));
#32952=CARTESIAN_POINT('Ctrl Pts',(-0.214130719605816,0.0111571281321464,
-0.00978652299914088));
#32953=CARTESIAN_POINT('Ctrl Pts',(-0.214119828009397,0.0110491600093937,
-0.00983252088936748));
#32954=CARTESIAN_POINT('Ctrl Pts',(-0.214110763409328,0.0109487202024644,
-0.00987313923237703));
#32955=CARTESIAN_POINT('Ctrl Pts',(-0.214105855700514,0.010894340602476,
-0.00989513060524584));
#32956=CARTESIAN_POINT('Ctrl Pts',(-0.21410148123821,0.0108422001052795,
-0.00991562376018389));
#32957=CARTESIAN_POINT('Ctrl Pts',(-0.214097508592728,0.0107903940484817,
-0.00993546403750088));
#32958=CARTESIAN_POINT('Ctrl Pts',(-0.214094143711908,0.0107465136650769,
-0.00995226900258296));
#32959=CARTESIAN_POINT('Ctrl Pts',(-0.214091067106676,0.0107028718786788,
-0.00996860292194799));
#32960=CARTESIAN_POINT('Ctrl Pts',(-0.214088198910818,0.01065827961437,
-0.00998489994682812));
#32961=CARTESIAN_POINT('Ctrl Pts',(-0.214075690020502,0.0104638020505384,
-0.0100559751825337));
#32962=CARTESIAN_POINT('Ctrl Pts',(-0.21406716976087,0.0102510002344298,
-0.0101256466000661));
#32963=CARTESIAN_POINT('Ctrl Pts',(-0.214063472264175,0.0100454113775732,
-0.0101848993120509));
#32964=CARTESIAN_POINT('Ctrl Pts',(-0.214059774767479,0.00983982252071662,
-0.0102441520240357));
#32965=CARTESIAN_POINT('Ctrl Pts',(-0.214060877726939,0.00964171398316327,
-0.0102939948760628));
#32966=CARTESIAN_POINT('Ctrl Pts',(-0.214065644163786,0.00943396330360745,
-0.0103389073683293));
#32967=CARTESIAN_POINT('Ctrl Pts',(-0.21406802738221,0.00933008796382954,
-0.0103613636144626));
#32968=CARTESIAN_POINT('Ctrl Pts',(-0.214071328264685,0.00922379415886723,
-0.0103825080238672));
#32969=CARTESIAN_POINT('Ctrl Pts',(-0.21407585910803,0.00911310620040166,
-0.0104024031717887));
#32970=CARTESIAN_POINT('Ctrl Pts',(-0.214080389951375,0.00900241824193609,
-0.0104222983197102));
#32971=CARTESIAN_POINT('Ctrl Pts',(-0.214086155225572,0.00888729480678718,
-0.0104407437416028));
#32972=CARTESIAN_POINT('Ctrl Pts',(-0.214092160048566,0.0087824703095477,
-0.0104557182416041));
#32973=CARTESIAN_POINT('Ctrl Pts',(-0.21409816487156,0.00867764581230821,
-0.0104706927416053));
#32974=CARTESIAN_POINT('Ctrl Pts',(-0.21410440059583,0.00858317218749535,
-0.0104825812100531));
#32975=CARTESIAN_POINT('Ctrl Pts',(-0.214111730246791,0.00848006693797604,
-0.0104938751473267));
#32976=CARTESIAN_POINT('Ctrl Pts',(-0.214115395072272,0.00842851431321638,
-0.0104995221159635));
#32977=CARTESIAN_POINT('Ctrl Pts',(-0.214119334123338,0.00837480225013233,
-0.0105049875567496));
#32978=CARTESIAN_POINT('Ctrl Pts',(-0.214123864686976,0.00831582647206328,
-0.0105103853131636));
#32979=CARTESIAN_POINT('Ctrl Pts',(-0.214128395250614,0.00825685069399423,
-0.0105157830695775));
#32980=CARTESIAN_POINT('Ctrl Pts',(-0.21413352061064,0.00819259641006701,
-0.0105209673652426));
#32981=CARTESIAN_POINT('Ctrl Pts',(-0.214137565354542,0.00814289901357351,
-0.0105245745801381));
#32982=CARTESIAN_POINT('Ctrl Pts',(-0.214141610098444,0.00809320161708002,
-0.0105281817950336));
#32983=CARTESIAN_POINT('Ctrl Pts',(-0.214144569038739,0.00805807717990574,
-0.0105304418179341));
#32984=CARTESIAN_POINT('Ctrl Pts',(-0.214148279134351,0.00801458612955796,
-0.0105329887781426));
#32985=CARTESIAN_POINT('Ctrl Pts',(-0.214151989229963,0.00797109507921019,
-0.0105355357383511));
#32986=CARTESIAN_POINT('Ctrl Pts',(-0.214156453463961,0.00791923052684874,
-0.0105382375369189));
#32987=CARTESIAN_POINT('Ctrl Pts',(-0.214161211273031,0.00786472646875704,
-0.0105405341258496));
#32988=CARTESIAN_POINT('Ctrl Pts',(-0.214170726891171,0.00775571835257365,
-0.0105451273037108));
#32989=CARTESIAN_POINT('Ctrl Pts',(-0.214181411936434,0.00763615658959353,
-0.0105483152401436));
#32990=CARTESIAN_POINT('Ctrl Pts',(-0.214193730627006,0.00750035314621932,
-0.0105485989486921));
#32991=CARTESIAN_POINT('Ctrl Pts',(-0.214193730574935,0.00750035257429044,
-0.0105485989475376));
#32992=CARTESIAN_POINT('Ctrl Pts',(-0.214181345616963,0.00736432013461061,
-0.0105483243338446));
#32993=CARTESIAN_POINT('Ctrl Pts',(-0.214170615447453,0.00724467154441374,
-0.0105451359586704));
#32994=CARTESIAN_POINT('Ctrl Pts',(-0.214161069591025,0.0071356472345695,
-0.0105405459272893));
#32995=CARTESIAN_POINT('Ctrl Pts',(-0.214156296656122,0.00708113500325122,
-0.0105382509083823));
#32996=CARTESIAN_POINT('Ctrl Pts',(-0.214151821033651,0.00702927995572575,
-0.0105355509097294));
#32997=CARTESIAN_POINT('Ctrl Pts',(-0.214148109500974,0.00698588746795613,
-0.0105330117591464));
#32998=CARTESIAN_POINT('Ctrl Pts',(-0.214144397968298,0.00694249498018651,
-0.0105304726085634));
#32999=CARTESIAN_POINT('Ctrl Pts',(-0.214141447512222,0.00690755810329318,
-0.0105282277386009));
#33000=CARTESIAN_POINT('Ctrl Pts',(-0.214137396362883,0.0068578514447973,
-0.0105246238289852));
#33001=CARTESIAN_POINT('Ctrl Pts',(-0.214133345213544,0.00680814478630143,
-0.0105210199193695));
#33002=CARTESIAN_POINT('Ctrl Pts',(-0.214128198626389,0.00674368458937078,
-0.0105158240713284));
#33003=CARTESIAN_POINT('Ctrl Pts',(-0.214123657729659,0.00668457551066981,
-0.0105104167347357));
#33004=CARTESIAN_POINT('Ctrl Pts',(-0.214119116832928,0.00662546643196883,
-0.0105050093981429));
#33005=CARTESIAN_POINT('Ctrl Pts',(-0.214115178280762,0.00657169344874913,
-0.0104995391005902));
#33006=CARTESIAN_POINT('Ctrl Pts',(-0.214111515099688,0.00652003053578507,
-0.0104938808240976));
#33007=CARTESIAN_POINT('Ctrl Pts',(-0.214104188737539,0.00641670470985695,
-0.0104825642711124));
#33008=CARTESIAN_POINT('Ctrl Pts',(-0.214097961137331,0.00632181412899653,
-0.0104706161469304));
#33009=CARTESIAN_POINT('Ctrl Pts',(-0.214092017849508,0.00621714983984993,
-0.0104556612666314));
#33010=CARTESIAN_POINT('Ctrl Pts',(-0.214086074561685,0.00611248555070334,
-0.0104407063863325));
#33011=CARTESIAN_POINT('Ctrl Pts',(-0.214080423805992,0.00599809690955629,
-0.010422378897594));
#33012=CARTESIAN_POINT('Ctrl Pts',(-0.214075994597286,0.00588787166133225,
-0.0104025810141776));
#33013=CARTESIAN_POINT('Ctrl Pts',(-0.214071565388579,0.0057776464131082,
-0.0103827831307611));
#33014=CARTESIAN_POINT('Ctrl Pts',(-0.214068353557564,0.0056715458111831,
-0.0103617018577092));
#33015=CARTESIAN_POINT('Ctrl Pts',(-0.214066060271609,0.00556779765735659,
-0.0103392962444784));
#33016=CARTESIAN_POINT('Ctrl Pts',(-0.2140614736997,0.00536030134970358,
-0.0102944850180168));
#33017=CARTESIAN_POINT('Ctrl Pts',(-0.214060553859486,0.00516218037746964,
-0.0102447055306988));
#33018=CARTESIAN_POINT('Ctrl Pts',(-0.214064458399895,0.00495623279761624,
-0.0101853953614391));
#33019=CARTESIAN_POINT('Ctrl Pts',(-0.214068362940304,0.00475028521776285,
-0.0101260851921794));
#33020=CARTESIAN_POINT('Ctrl Pts',(-0.214077114659975,0.00453678428426086,
-0.0100562132639311));
#33021=CARTESIAN_POINT('Ctrl Pts',(-0.214089782012679,0.004342031475676,
-0.00998504834678421));
#33022=CARTESIAN_POINT('Ctrl Pts',(-0.214092690231091,0.00429731939438625,
-0.00996871003780899));
#33023=CARTESIAN_POINT('Ctrl Pts',(-0.214095803503907,0.00425358214047101,
-0.00995234173959868));
#33024=CARTESIAN_POINT('Ctrl Pts',(-0.214099204596534,0.00420959871191655,
-0.00993549782678036));
#33025=CARTESIAN_POINT('Ctrl Pts',(-0.21410321058855,0.00415779263576576,
-0.00991565814945591));
#33026=CARTESIAN_POINT('Ctrl Pts',(-0.214107615884805,0.00410564313783565,
-0.00989516236796775));
#33027=CARTESIAN_POINT('Ctrl Pts',(-0.214112555731078,0.00405120821435422,
-0.00987314859199749));
#33028=CARTESIAN_POINT('Ctrl Pts',(-0.214121689513501,0.00395055796738748,
-0.00983244509052506));
#33029=CARTESIAN_POINT('Ctrl Pts',(-0.214132658894906,0.00384220786214466,
-0.00978627536711066));
#33030=CARTESIAN_POINT('Ctrl Pts',(-0.214143350697998,0.00374517508066676,
-0.00974287572751151));
#33031=CARTESIAN_POINT('Ctrl Pts',(-0.214154042501091,0.00364814229918887,
-0.00969947608791235));
#33032=CARTESIAN_POINT('Ctrl Pts',(-0.21416444770987,0.00356222737904924,
-0.00965927365907892));
#33033=CARTESIAN_POINT('Ctrl Pts',(-0.21417620969836,0.00346954930648967,
-0.00961408480996121));
#33034=CARTESIAN_POINT('Ctrl Pts',(-0.214182090692604,0.0034232102702099,
-0.00959149038540235));
#33035=CARTESIAN_POINT('Ctrl Pts',(-0.214188311461854,0.00337519720913805,
-0.00956762083501447));
#33036=CARTESIAN_POINT('Ctrl Pts',(-0.21419536566459,0.00332258178985352,
-0.00954079257226103));
#33037=CARTESIAN_POINT('Ctrl Pts',(-0.214202419867326,0.00326996637056899,
-0.0095139643095076));
#33038=CARTESIAN_POINT('Ctrl Pts',(-0.214210310421654,0.00321281808848199,
-0.00948403777143926));
#33039=CARTESIAN_POINT('Ctrl Pts',(-0.214216339274854,0.00316982536706485,
-0.00946109081517068));
#33040=CARTESIAN_POINT('Ctrl Pts',(-0.214222368128053,0.00312683264564772,
-0.00943814385890211));
#33041=CARTESIAN_POINT('Ctrl Pts',(-0.214226530873441,0.00309788065642511,
-0.0094223899883824));
#33042=CARTESIAN_POINT('Ctrl Pts',(-0.214231888387702,0.00306092283807243,
-0.00940202005736926));
#33043=CARTESIAN_POINT('Ctrl Pts',(-0.214237245901962,0.00302396501971975,
-0.00938165012635613));
#33044=CARTESIAN_POINT('Ctrl Pts',(-0.214243800654996,0.00297906883286363,
-0.00935654357939838));
#33045=CARTESIAN_POINT('Ctrl Pts',(-0.214250786332799,0.00293183529864835,
-0.00932950779425316));
#33046=CARTESIAN_POINT('Ctrl Pts',(-0.214264757651952,0.00283736847668207,
-0.00927543636503528));
#33047=CARTESIAN_POINT('Ctrl Pts',(-0.214280448620716,0.00273343208000158,
-0.00921384815061718));
#33048=CARTESIAN_POINT('Ctrl Pts',(-0.214298628577443,0.00261569126736467,
-0.0091400261770453));
#33049=CARTESIAN_POINT('',(-0.224520431112711,0.00173717640815345,-0.00870165576114943));
#33050=CARTESIAN_POINT('',(-0.223316843015392,0.00173498433150003,-0.00867730364596437));
#33051=CARTESIAN_POINT('',(-0.223316842847435,0.00173497690009322,-0.00867731262527063));
#33052=CARTESIAN_POINT('',(-0.222880624396322,0.00442263472015358,-0.0102052666341114));
#33053=CARTESIAN_POINT('Ctrl Pts',(-0.223316843015392,0.00173498433150003,
-0.00867730364596437));
#33054=CARTESIAN_POINT('Ctrl Pts',(-0.223279812530346,0.00186517669334324,
-0.00878435058928567));
#33055=CARTESIAN_POINT('Ctrl Pts',(-0.223232277207935,0.00203819990847103,
-0.00891798594929538));
#33056=CARTESIAN_POINT('Ctrl Pts',(-0.223180379664801,0.00223735359889598,
-0.00906189282015912));
#33057=CARTESIAN_POINT('Ctrl Pts',(-0.223156273797957,0.00233181413205371,
-0.00912841520280122));
#33058=CARTESIAN_POINT('Ctrl Pts',(-0.223110681833087,0.00252272373509083,
-0.00925731540364347));
#33059=CARTESIAN_POINT('Ctrl Pts',(-0.223064310367951,0.00273688688368519,
-0.00939387105231042));
#33060=CARTESIAN_POINT('Ctrl Pts',(-0.223014089616156,0.00300235697175274,
-0.00955231904645436));
#33061=CARTESIAN_POINT('Ctrl Pts',(-0.22296962319346,0.00330683358017323,
-0.00971821280969721));
#33062=CARTESIAN_POINT('Ctrl Pts',(-0.222918488070061,0.00375942200152719,
-0.00994375002725347));
#33063=CARTESIAN_POINT('Ctrl Pts',(-0.222892083013316,0.00416376038165397,
-0.010111187965774));
#33064=CARTESIAN_POINT('Ctrl Pts',(-0.222880624396322,0.00442263472015358,
-0.0102052666341114));
#33065=CARTESIAN_POINT('',(-0.222990249020465,0.00750413602119545,-0.0107474065933957));
#33066=CARTESIAN_POINT('Ctrl Pts',(-0.222880624396322,0.00442263472015358,
-0.0102052666341114));
#33067=CARTESIAN_POINT('Ctrl Pts',(-0.222869165779329,0.0046815090586532,
-0.0102993453024488));
#33068=CARTESIAN_POINT('Ctrl Pts',(-0.222858538053683,0.00517788857248262,
-0.0104524093911042));
#33069=CARTESIAN_POINT('Ctrl Pts',(-0.222872218454889,0.005825756390809,
-0.0105939424252743));
#33070=CARTESIAN_POINT('Ctrl Pts',(-0.222894283711276,0.00623987313934977,
-0.0106579681688692));
#33071=CARTESIAN_POINT('Ctrl Pts',(-0.222910771496852,0.00650106062914115,
-0.0106909307204901));
#33072=CARTESIAN_POINT('Ctrl Pts',(-0.222927661448382,0.00673784986174582,
-0.0107142151130225));
#33073=CARTESIAN_POINT('Ctrl Pts',(-0.222937668479361,0.00686760687829407,
-0.0107242714777256));
#33074=CARTESIAN_POINT('Ctrl Pts',(-0.222957834975291,0.00712122554238282,
-0.010740444183054));
#33075=CARTESIAN_POINT('Ctrl Pts',(-0.222976136323122,0.00733939368582136,
-0.0107471639425212));
#33076=CARTESIAN_POINT('Ctrl Pts',(-0.222990249020465,0.00750413602119545,
-0.0107474065933957));
#33077=CARTESIAN_POINT('',(-0.222877378469082,0.0105855117421594,-0.0102022589418487));
#33078=CARTESIAN_POINT('Ctrl Pts',(-0.222990244138736,0.00750419266379995,
-0.0107474064566597));
#33079=CARTESIAN_POINT('Ctrl Pts',(-0.222976039113982,0.00766901363741887,
-0.0107470080875829));
#33080=CARTESIAN_POINT('Ctrl Pts',(-0.222957602873573,0.0078873936039232,
-0.0107400749543394));
#33081=CARTESIAN_POINT('Ctrl Pts',(-0.222937255048052,0.00814141129479029,
-0.0107236237028279));
#33082=CARTESIAN_POINT('Ctrl Pts',(-0.222927131990394,0.00827164133562222,
-0.0107133928644021));
#33083=CARTESIAN_POINT('Ctrl Pts',(-0.222910062603263,0.00850863202679079,
-0.0106898315254736));
#33084=CARTESIAN_POINT('Ctrl Pts',(-0.222893339477359,0.00877024695059987,
-0.0106565146658551));
#33085=CARTESIAN_POINT('Ctrl Pts',(-0.222870855927369,0.00918444368936968,
-0.0105920366667686));
#33086=CARTESIAN_POINT('Ctrl Pts',(-0.222856249020398,0.00983626402533809,
-0.0104486341552913));
#33087=CARTESIAN_POINT('Ctrl Pts',(-0.222866269191294,0.0103293456390423,
-0.0102956441034219));
#33088=CARTESIAN_POINT('Ctrl Pts',(-0.222877378469082,0.0105855117421594,
-0.0102022589418487));
#33089=CARTESIAN_POINT('',(-0.22331062247459,0.0132796121775377,-0.0086650768419741));
#33090=CARTESIAN_POINT('Ctrl Pts',(-0.222877378469082,0.0105855117421594,
-0.0102022589418487));
#33091=CARTESIAN_POINT('Ctrl Pts',(-0.222877439347042,0.010586915512061,
-0.0102017471985795));
#33092=CARTESIAN_POINT('Ctrl Pts',(-0.222888704245993,0.0108459462110236,
-0.0101072438214903));
#33093=CARTESIAN_POINT('Ctrl Pts',(-0.222914931562689,0.0112496955499137,
-0.0099395147505797));
#33094=CARTESIAN_POINT('Ctrl Pts',(-0.222966043253251,0.0117035833443654,
-0.00971273963873267));
#33095=CARTESIAN_POINT('Ctrl Pts',(-0.223011019189053,0.0120122134010204,
-0.00954390981295897));
#33096=CARTESIAN_POINT('Ctrl Pts',(-0.223060691065504,0.0122764008889023,
-0.00938554157135033));
#33097=CARTESIAN_POINT('Ctrl Pts',(-0.223106708820329,0.0124909981044285,
-0.0092481825342308));
#33098=CARTESIAN_POINT('Ctrl Pts',(-0.223151918814857,0.0126824022555419,
-0.00911841361702317));
#33099=CARTESIAN_POINT('Ctrl Pts',(-0.223175770367161,0.0127770012983113,
-0.00905151203694784));
#33100=CARTESIAN_POINT('Ctrl Pts',(-0.223227096344508,0.0129763708623679,
-0.00890683647480226));
#33101=CARTESIAN_POINT('Ctrl Pts',(-0.223274054708729,0.0131494382524228,
-0.00877258438081807));
#33102=CARTESIAN_POINT('Ctrl Pts',(-0.223310622067065,0.0132796145543947,
-0.00866508035255934));
#33103=CARTESIAN_POINT('',(-0.224514160940373,0.0132784691364097,-0.00868853601036365));
#33104=CARTESIAN_POINT('',(-0.224514160785051,0.0132784760514594,-0.00868854430898473));
#33105=CARTESIAN_POINT('',(-0.224077522253103,0.0105904549332816,-0.010226572185957));
#33106=CARTESIAN_POINT('Ctrl Pts',(-0.224514160940373,0.0132784691364097,
-0.00868853601036365));
#33107=CARTESIAN_POINT('Ctrl Pts',(-0.224477211330273,0.0131470369833515,
-0.00879735581073573));
#33108=CARTESIAN_POINT('Ctrl Pts',(-0.224429947924994,0.0129731504511415,
-0.00893246460129079));
#33109=CARTESIAN_POINT('Ctrl Pts',(-0.224378503318962,0.0127742662803209,
-0.00907701980843753));
#33110=CARTESIAN_POINT('Ctrl Pts',(-0.224355204002411,0.012682587246764,
-0.00914202253367616));
#33111=CARTESIAN_POINT('Ctrl Pts',(-0.224309198807288,0.012489784381346,
-0.00927305835532011));
#33112=CARTESIAN_POINT('Ctrl Pts',(-0.224262698143804,0.0122754037092251,
-0.0094105335025692));
#33113=CARTESIAN_POINT('Ctrl Pts',(-0.224212453791538,0.012012311248366,
-0.00956858000955867));
#33114=CARTESIAN_POINT('Ctrl Pts',(-0.224166966590675,0.0117051190396636,
-0.0097370321999535));
#33115=CARTESIAN_POINT('Ctrl Pts',(-0.224115284552749,0.0112520802508404,
-0.00996403935026655));
#33116=CARTESIAN_POINT('Ctrl Pts',(-0.224088864698508,0.010848572764703,
-0.010132103654354));
#33117=CARTESIAN_POINT('Ctrl Pts',(-0.224077522253103,0.0105904549332816,
-0.010226572185957));
#33118=CARTESIAN_POINT('',(-0.224190652839191,0.00750467962157126,-0.0107745363515886));
#33119=CARTESIAN_POINT('Ctrl Pts',(-0.224077522253103,0.0105904549332816,
-0.010226572185957));
#33120=CARTESIAN_POINT('Ctrl Pts',(-0.224066179807698,0.0103323371018601,
-0.0103210407175601));
#33121=CARTESIAN_POINT('Ctrl Pts',(-0.224056036498401,0.00983787575769098,
-0.010474829105189));
#33122=CARTESIAN_POINT('Ctrl Pts',(-0.224070822277838,0.00918506719538518,
-0.0106187627126106));
#33123=CARTESIAN_POINT('Ctrl Pts',(-0.224093495468947,0.00877092269132658,
-0.0106833806781232));
#33124=CARTESIAN_POINT('Ctrl Pts',(-0.224110305171158,0.00850937751485411,
-0.0107167762264158));
#33125=CARTESIAN_POINT('Ctrl Pts',(-0.224127483217192,0.0082719805659879,
-0.0107404318766813));
#33126=CARTESIAN_POINT('Ctrl Pts',(-0.224137553020629,0.00814288141660961,
-0.0107506002887076));
#33127=CARTESIAN_POINT('Ctrl Pts',(-0.224157926592086,0.00788901316584556,
-0.010767122229214));
#33128=CARTESIAN_POINT('Ctrl Pts',(-0.224176402851754,0.00767017484618538,
-0.0107741274603846));
#33129=CARTESIAN_POINT('Ctrl Pts',(-0.224190654114418,0.00750468128569608,
-0.0107745364705206));
#33130=CARTESIAN_POINT('',(-0.224080543674127,0.00442370045670947,-0.0102317785325732));
#33131=CARTESIAN_POINT('Ctrl Pts',(-0.224190653963733,0.00750467952515814,
-0.0107745364680395));
#33132=CARTESIAN_POINT('Ctrl Pts',(-0.224176492634204,0.00733922436874332,
-0.0107743032793675));
#33133=CARTESIAN_POINT('Ctrl Pts',(-0.224158150009196,0.0071205751719775,
-0.0107675345622608));
#33134=CARTESIAN_POINT('Ctrl Pts',(-0.224137959599138,0.00686713230331976,
-0.0107513204960082));
#33135=CARTESIAN_POINT('Ctrl Pts',(-0.22412801473866,0.00673863242070432,
-0.0107413514946879));
#33136=CARTESIAN_POINT('Ctrl Pts',(-0.224111008867221,0.00650134479792787,
-0.0107179940224818));
#33137=CARTESIAN_POINT('Ctrl Pts',(-0.224094430592809,0.0062402098664611,
-0.0106849790050444));
#33138=CARTESIAN_POINT('Ctrl Pts',(-0.224072172068249,0.00582632754687287,
-0.0106209007979213));
#33139=CARTESIAN_POINT('Ctrl Pts',(-0.224058310898166,0.00517837148533668,
-0.0104791024854185));
#33140=CARTESIAN_POINT('Ctrl Pts',(-0.224068978285216,0.00468250947702801,
-0.0103259955728961));
#33141=CARTESIAN_POINT('Ctrl Pts',(-0.224080543674127,0.00442370045670947,
-0.0102317785325732));
#33142=CARTESIAN_POINT('Ctrl Pts',(-0.224080576473508,0.00442296681989542,
-0.0102315114221622));
#33143=CARTESIAN_POINT('Ctrl Pts',(-0.224092164582625,0.00416389245189672,
-0.01013717187508));
#33144=CARTESIAN_POINT('Ctrl Pts',(-0.224118916883511,0.0037587335085994,
-0.00996905170028294));
#33145=CARTESIAN_POINT('Ctrl Pts',(-0.22417075519572,0.00330687307078908,
-0.00974336361782637));
#33146=CARTESIAN_POINT('Ctrl Pts',(-0.224215944808682,0.00300301955498354,
-0.00957745415886877));
#33147=CARTESIAN_POINT('Ctrl Pts',(-0.224266694586266,0.00273933256641242,
-0.0094197813232676));
#33148=CARTESIAN_POINT('Ctrl Pts',(-0.224313605043636,0.00252528923250781,
-0.00928311801791386));
#33149=CARTESIAN_POINT('Ctrl Pts',(-0.224360139565172,0.00233246415434654,
-0.00915264520743171));
#33150=CARTESIAN_POINT('Ctrl Pts',(-0.224383537818016,0.00224151895518211,
-0.00908844952425034));
#33151=CARTESIAN_POINT('Ctrl Pts',(-0.224435538741471,0.00204291078658062,
-0.00894477273158201));
#33152=CARTESIAN_POINT('Ctrl Pts',(-0.224483417379835,0.00186891392296787,
-0.00881022807967479));
#33153=CARTESIAN_POINT('Ctrl Pts',(-0.224520891120564,0.00173723890051058,
-0.00870172018785915));
#33154=CARTESIAN_POINT('',(-0.212297190745867,0.00261509365239396,-0.00909973957363974));
#33155=CARTESIAN_POINT('',(-0.211094978475873,0.0026144378598994,-0.00907540326291864));
#33156=CARTESIAN_POINT('',(-0.212297189692149,0.00261509491117278,-0.00909973513226721));
#33157=CARTESIAN_POINT('',(-0.210993897433281,0.00750003962408243,-0.0104762800771199));
#33158=CARTESIAN_POINT('Ctrl Pts',(-0.211094976956083,0.00261443904769588,
-0.00907540097906681));
#33159=CARTESIAN_POINT('Ctrl Pts',(-0.211076902605002,0.00273164864698635,
-0.00914838755433385));
#33160=CARTESIAN_POINT('Ctrl Pts',(-0.211053454528153,0.00288716843060544,
-0.00924010842643544));
#33161=CARTESIAN_POINT('Ctrl Pts',(-0.211027284102128,0.00306711239604655,
-0.00933999693310741));
#33162=CARTESIAN_POINT('Ctrl Pts',(-0.21101466974253,0.00315522153342331,
-0.00938771508920937));
#33163=CARTESIAN_POINT('Ctrl Pts',(-0.210991202323522,0.00332631582695644,
-0.00947684014530071));
#33164=CARTESIAN_POINT('Ctrl Pts',(-0.210966529056182,0.00351877420073698,
-0.00957165595315125));
#33165=CARTESIAN_POINT('Ctrl Pts',(-0.210940630339799,0.00373561938964548,
-0.00967286496974557));
#33166=CARTESIAN_POINT('Ctrl Pts',(-0.21090882306288,0.00405724803395585,
-0.00980902641083227));
#33167=CARTESIAN_POINT('Ctrl Pts',(-0.210880468868142,0.00443154685424827,
-0.00995193760637929));
#33168=CARTESIAN_POINT('Ctrl Pts',(-0.210860080553832,0.00496167972118646,
-0.0101244790534111));
#33169=CARTESIAN_POINT('Ctrl Pts',(-0.210862937430638,0.00545949645723989,
-0.0102482570737715));
#33170=CARTESIAN_POINT('Ctrl Pts',(-0.210876138533289,0.00588408926952714,
-0.0103325668728133));
#33171=CARTESIAN_POINT('Ctrl Pts',(-0.210893327512164,0.0062282183878831,
-0.010387245267968));
#33172=CARTESIAN_POINT('Ctrl Pts',(-0.210908799693423,0.00646418655898334,
-0.010416504326486));
#33173=CARTESIAN_POINT('Ctrl Pts',(-0.210924391642302,0.00667919920548634,
-0.0104384931741096));
#33174=CARTESIAN_POINT('Ctrl Pts',(-0.210939543408632,0.00687173172318124,
-0.0104538539003637));
#33175=CARTESIAN_POINT('Ctrl Pts',(-0.210948449678075,0.00697902885001758,
-0.0104606407092845));
#33176=CARTESIAN_POINT('Ctrl Pts',(-0.210966087921597,0.00718683343980474,
-0.010471448835588));
#33177=CARTESIAN_POINT('Ctrl Pts',(-0.210981837268104,0.00736539084021717,
-0.0104760080954136));
#33178=CARTESIAN_POINT('Ctrl Pts',(-0.210993897433281,0.00750003962408243,
-0.0104762800771199));
#33179=CARTESIAN_POINT('',(-0.211094250162357,0.0123877779842441,-0.00907399873728111));
#33180=CARTESIAN_POINT('Ctrl Pts',(-0.210993897632963,0.00750004185348807,
-0.0104762800816229));
#33181=CARTESIAN_POINT('Ctrl Pts',(-0.210981890216983,0.00763468789296296,
-0.0104760080851524));
#33182=CARTESIAN_POINT('Ctrl Pts',(-0.210966199980559,0.00781332793409896,
-0.0104714488088166));
#33183=CARTESIAN_POINT('Ctrl Pts',(-0.210948602845398,0.00802143287698861,
-0.0104606187649496));
#33184=CARTESIAN_POINT('Ctrl Pts',(-0.210939703774113,0.00812901655090803,
-0.0104538083326638));
#33185=CARTESIAN_POINT('Ctrl Pts',(-0.210924554722707,0.00832203008104696,
-0.0104383893943833));
#33186=CARTESIAN_POINT('Ctrl Pts',(-0.210908948238448,0.00853754616492999,
-0.0104163157338736));
#33187=CARTESIAN_POINT('Ctrl Pts',(-0.210893432115795,0.00877414459232575,
-0.0103869227932625));
#33188=CARTESIAN_POINT('Ctrl Pts',(-0.210876133572762,0.00911857566127197,
-0.0103320979866237));
#33189=CARTESIAN_POINT('Ctrl Pts',(-0.210862740048901,0.00954314440249559,
-0.0102476263108843));
#33190=CARTESIAN_POINT('Ctrl Pts',(-0.210859479042776,0.0100378417967945,
-0.0101245951266467));
#33191=CARTESIAN_POINT('Ctrl Pts',(-0.210879522352077,0.010570553837214,
-0.0099512065487221));
#33192=CARTESIAN_POINT('Ctrl Pts',(-0.210907788954054,0.0109453488756747,
-0.0098079652419107));
#33193=CARTESIAN_POINT('Ctrl Pts',(-0.210939669417399,0.011267837985318,
-0.00967129752156446));
#33194=CARTESIAN_POINT('Ctrl Pts',(-0.210965530369932,0.0114839680748931,
-0.00957031370016262));
#33195=CARTESIAN_POINT('Ctrl Pts',(-0.210990215655556,0.0116761440659366,
-0.0094755657339967));
#33196=CARTESIAN_POINT('Ctrl Pts',(-0.211013692363919,0.0118468850488585,
-0.00938656527404313));
#33197=CARTESIAN_POINT('Ctrl Pts',(-0.211026338937093,0.0119349808819548,
-0.00933882751891443));
#33198=CARTESIAN_POINT('Ctrl Pts',(-0.211052578045645,0.0121148872431664,
-0.00923890045957065));
#33199=CARTESIAN_POINT('Ctrl Pts',(-0.211076107929383,0.0122704862945661,
-0.00914708137410498));
#33200=CARTESIAN_POINT('Ctrl Pts',(-0.211094250162357,0.0123877779842441,
-0.00907399873728111));
#33201=CARTESIAN_POINT('',(-0.212296026124715,0.0123861564107362,-0.00909893835561097));
#33202=CARTESIAN_POINT('',(-0.21109425028115,0.0123877742504626,-0.00907399277386768));
#33203=CARTESIAN_POINT('',(-0.212194328822827,0.00750004200959953,-0.0105034107997523));
#33204=CARTESIAN_POINT('Ctrl Pts',(-0.212296025195952,0.012386155034837,
-0.00909893592235296));
#33205=CARTESIAN_POINT('Ctrl Pts',(-0.212277771181288,0.0122681537068886,
-0.00917262789174738));
#33206=CARTESIAN_POINT('Ctrl Pts',(-0.212262026617893,0.0121640536793492,
-0.00923406794799332));
#33207=CARTESIAN_POINT('Ctrl Pts',(-0.212248015826452,0.012069474226596,
-0.00928799208719917));
#33208=CARTESIAN_POINT('Ctrl Pts',(-0.212241010396515,0.0120221842692378,
-0.00931495428849542));
#33209=CARTESIAN_POINT('Ctrl Pts',(-0.212234439427194,0.0119772443834241,
-0.00933998720033867));
#33210=CARTESIAN_POINT('Ctrl Pts',(-0.212229075568991,0.0119402994511595,
-0.00936027144983805));
#33211=CARTESIAN_POINT('Ctrl Pts',(-0.212223711710787,0.0119033545188948,
-0.00938055569933742));
#33212=CARTESIAN_POINT('Ctrl Pts',(-0.212219552489172,0.0118744719849607,
-0.00939621227379056));
#33213=CARTESIAN_POINT('Ctrl Pts',(-0.212213511685548,0.0118314285085296,
-0.00941909943121386));
#33214=CARTESIAN_POINT('Ctrl Pts',(-0.212207470881924,0.0117883850320986,
-0.00944198658863716));
#33215=CARTESIAN_POINT('Ctrl Pts',(-0.212199552919732,0.0117310655767387,
-0.0094718896685894));
#33216=CARTESIAN_POINT('Ctrl Pts',(-0.212192484407939,0.0116783235343651,
-0.00949868046344015));
#33217=CARTESIAN_POINT('Ctrl Pts',(-0.212185415896147,0.0116255814919915,
-0.00952547125829089));
#33218=CARTESIAN_POINT('Ctrl Pts',(-0.212179193892156,0.0115774868294401,
-0.00954929070656413));
#33219=CARTESIAN_POINT('Ctrl Pts',(-0.212173309502402,0.0115310109034,-0.00957186554182796));
#33220=CARTESIAN_POINT('Ctrl Pts',(-0.212161540722894,0.0114380590513197,
-0.00961701521235564));
#33221=CARTESIAN_POINT('Ctrl Pts',(-0.212151120316311,0.0113516431713247,
-0.00965728933529618));
#33222=CARTESIAN_POINT('Ctrl Pts',(-0.212140516807543,0.0112547003042211,
-0.00970048125207246));
#33223=CARTESIAN_POINT('Ctrl Pts',(-0.212129913298776,0.0111577574371174,
-0.00974367316884873));
#33224=CARTESIAN_POINT('Ctrl Pts',(-0.212119135175636,0.0110501002630214,
-0.00978938029664853));
#33225=CARTESIAN_POINT('Ctrl Pts',(-0.212110169288513,0.0109496173505987,
-0.00982987977422684));
#33226=CARTESIAN_POINT('Ctrl Pts',(-0.212105030416407,0.0108920247411125,
-0.0098530923836181));
#33227=CARTESIAN_POINT('Ctrl Pts',(-0.212100484409045,0.0108368243355517,
-0.00987468061069946));
#33228=CARTESIAN_POINT('Ctrl Pts',(-0.212096381915708,0.0107818522688614,
-0.00989559572584027));
#33229=CARTESIAN_POINT('Ctrl Pts',(-0.212093326711515,0.0107409135335892,
-0.00991117160671009));
#33230=CARTESIAN_POINT('Ctrl Pts',(-0.212090517482946,0.0107000997302077,
-0.00992637045413619));
#33231=CARTESIAN_POINT('Ctrl Pts',(-0.212087892544318,0.010658492958655,
-0.00994152400292711));
#33232=CARTESIAN_POINT('Ctrl Pts',(-0.212075593191774,0.0104635412191762,
-0.0100125271253955));
#33233=CARTESIAN_POINT('Ctrl Pts',(-0.212067363419537,0.0102509499324125,
-0.0100818754945736));
#33234=CARTESIAN_POINT('Ctrl Pts',(-0.212063884862461,0.0100453926460674,
-0.0101409198863523));
#33235=CARTESIAN_POINT('Ctrl Pts',(-0.212060406305386,0.00983983535972219,
-0.0101999642781311));
#33236=CARTESIAN_POINT('Ctrl Pts',(-0.212061657359005,0.00964157027834746,
-0.0102496821449324));
#33237=CARTESIAN_POINT('Ctrl Pts',(-0.212066560809478,0.00943377986916841,
-0.0102944520101106));
#33238=CARTESIAN_POINT('Ctrl Pts',(-0.212069012534715,0.00932988466457889,
-0.0103168369426997));
#33239=CARTESIAN_POINT('Ctrl Pts',(-0.2120723790939,0.00922360061547029,
-0.0103379082944401));
#33240=CARTESIAN_POINT('Ctrl Pts',(-0.212076974896308,0.00911290057028226,
-0.0103577387941635));
#33241=CARTESIAN_POINT('Ctrl Pts',(-0.212081570698716,0.00900220052509422,
-0.010377569293887));
#33242=CARTESIAN_POINT('Ctrl Pts',(-0.212087400244757,0.00888704309246514,
-0.0103959570783915));
#33243=CARTESIAN_POINT('Ctrl Pts',(-0.212093439725352,0.00878228104010102,
-0.0104108722877212));
#33244=CARTESIAN_POINT('Ctrl Pts',(-0.212099479205947,0.00867751898773691,
-0.0104257874970509));
#33245=CARTESIAN_POINT('Ctrl Pts',(-0.212105719912849,0.00858320444963351,
-0.0104376177616694));
#33246=CARTESIAN_POINT('Ctrl Pts',(-0.212113035079603,0.00848009932947122,
-0.0104488749494349));
#33247=CARTESIAN_POINT('Ctrl Pts',(-0.21211669266298,0.00842854676939008,
-0.0104545035433176));
#33248=CARTESIAN_POINT('Ctrl Pts',(-0.212120619623256,0.00837479494961345,
-0.0104599551726937));
#33249=CARTESIAN_POINT('Ctrl Pts',(-0.212125126833372,0.00831578408466029,
-0.0104653377458155));
#33250=CARTESIAN_POINT('Ctrl Pts',(-0.212129634043488,0.00825677321970713,
-0.0104707203189373));
#33251=CARTESIAN_POINT('Ctrl Pts',(-0.212134724759161,0.00819248868025532,
-0.0104758892980401));
#33252=CARTESIAN_POINT('Ctrl Pts',(-0.21213874797157,0.00814265720978303,
-0.0104794924998593));
#33253=CARTESIAN_POINT('Ctrl Pts',(-0.212142771183979,0.00809282573931075,
-0.0104830957016785));
#33254=CARTESIAN_POINT('Ctrl Pts',(-0.212145721744291,0.00805746323684213,
-0.0104853613080341));
#33255=CARTESIAN_POINT('Ctrl Pts',(-0.212149407167978,0.00801383089916331,
-0.0104879038888235));
#33256=CARTESIAN_POINT('Ctrl Pts',(-0.212153092591665,0.00797019856148449,
-0.0104904464696128));
#33257=CARTESIAN_POINT('Ctrl Pts',(-0.212157515838839,0.00791828959182719,
-0.0104931349412913));
#33258=CARTESIAN_POINT('Ctrl Pts',(-0.212162223711799,0.00786378802432783,
-0.0104954173976478));
#33259=CARTESIAN_POINT('Ctrl Pts',(-0.212171639457718,0.00775478488932911,
-0.0104999823103607));
#33260=CARTESIAN_POINT('Ctrl Pts',(-0.212182188900109,0.00763541561494652,
-0.010503135815364));
#33261=CARTESIAN_POINT('Ctrl Pts',(-0.212194328841677,0.00750004244211601,
-0.0105034108204182));
#33262=CARTESIAN_POINT('Ctrl Pts',(-0.212194328802889,0.00750004201135476,
-0.0105034108195435));
#33263=CARTESIAN_POINT('Ctrl Pts',(-0.212182123539449,0.00736450040649182,
-0.0105031355974154));
#33264=CARTESIAN_POINT('Ctrl Pts',(-0.212171528626418,0.00724509368721271,
-0.0104999761795604));
#33265=CARTESIAN_POINT('Ctrl Pts',(-0.212162080336148,0.00713610960086918,
-0.0104954100708588));
#33266=CARTESIAN_POINT('Ctrl Pts',(-0.212157356186009,0.00708161749997084,
-0.0104931270140894));
#33267=CARTESIAN_POINT('Ctrl Pts',(-0.21215291990874,0.00702973214041256,
-0.010490438460955));
#33268=CARTESIAN_POINT('Ctrl Pts',(-0.212149231583743,0.00698621172109704,
-0.010487902327003));
#33269=CARTESIAN_POINT('Ctrl Pts',(-0.212145543258746,0.00694269130178152,
-0.010485366193051));
#33270=CARTESIAN_POINT('Ctrl Pts',(-0.212142599894812,0.0069075289581561,
-0.0104831149386858));
#33271=CARTESIAN_POINT('Ctrl Pts',(-0.212138566498245,0.00685768893969642,
-0.0104795127975055));
#33272=CARTESIAN_POINT('Ctrl Pts',(-0.212134533101678,0.00680784892123675,
-0.0104759106563253));
#33273=CARTESIAN_POINT('Ctrl Pts',(-0.212129414893486,0.00674334732119604,
-0.0104707262493208));
#33274=CARTESIAN_POINT('Ctrl Pts',(-0.212124891557789,0.00668420290603628,
-0.010465331278609));
#33275=CARTESIAN_POINT('Ctrl Pts',(-0.212120368222091,0.00662505849087652,
-0.0104599363078971));
#33276=CARTESIAN_POINT('Ctrl Pts',(-0.212116436438123,0.00657125637734932,
-0.0104544781964647));
#33277=CARTESIAN_POINT('Ctrl Pts',(-0.212112775599472,0.00651961866839045,
-0.0104488387645201));
#33278=CARTESIAN_POINT('Ctrl Pts',(-0.21210545392217,0.00641634325047269,
-0.0104375599006309));
#33279=CARTESIAN_POINT('Ctrl Pts',(-0.212099213203322,0.00632171996357587,
-0.010425680554823));
#33280=CARTESIAN_POINT('Ctrl Pts',(-0.212093220629257,0.00621716805955512,
-0.0104107896322911));
#33281=CARTESIAN_POINT('Ctrl Pts',(-0.212087228055191,0.00611261615553437,
-0.0103958987097591));
#33282=CARTESIAN_POINT('Ctrl Pts',(-0.212081491953092,0.00599818549761978,
-0.0103776255386813));
#33283=CARTESIAN_POINT('Ctrl Pts',(-0.212076978793602,0.00588796000678455,
-0.0103578922018477));
#33284=CARTESIAN_POINT('Ctrl Pts',(-0.212072465634112,0.00577773451594932,
-0.0103381588650141));
#33285=CARTESIAN_POINT('Ctrl Pts',(-0.212069171194045,0.00567167514409762,
-0.0103171548169983));
#33286=CARTESIAN_POINT('Ctrl Pts',(-0.212066792035586,0.00556794849651943,
-0.0102948284638349));
#33287=CARTESIAN_POINT('Ctrl Pts',(-0.212062033718667,0.00536049520136305,
-0.0102501757575081));
#33288=CARTESIAN_POINT('Ctrl Pts',(-0.212060929276825,0.00516233987027589,
-0.0102005541469401));
#33289=CARTESIAN_POINT('Ctrl Pts',(-0.212064583752465,0.00495647680610926,
-0.0101414727213551));
#33290=CARTESIAN_POINT('Ctrl Pts',(-0.212068238228106,0.00475061374194264,
-0.0100823912957701));
#33291=CARTESIAN_POINT('Ctrl Pts',(-0.212076673891627,0.00453730905366078,
-0.0100128424971044));
#33292=CARTESIAN_POINT('Ctrl Pts',(-0.212089098860114,0.00434224089645113,
-0.00994181834806706));
#33293=CARTESIAN_POINT('Ctrl Pts',(-0.212091765988984,0.00430036779920021,
-0.0099265723892066));
#33294=CARTESIAN_POINT('Ctrl Pts',(-0.212094615809571,0.00425932394153444,
-0.00991129019538823));
#33295=CARTESIAN_POINT('Ctrl Pts',(-0.212097714097661,0.00421814204450483,
-0.00989562226672202));
#33296=CARTESIAN_POINT('Ctrl Pts',(-0.21210183258344,0.00416339986030607,
-0.00987479523594094));
#33297=CARTESIAN_POINT('Ctrl Pts',(-0.212106390106241,0.00410841068640518,
-0.00985329330232126));
#33298=CARTESIAN_POINT('Ctrl Pts',(-0.212111541160687,0.00405096246581216,
-0.00983014395607332));
#33299=CARTESIAN_POINT('Ctrl Pts',(-0.212120567292405,0.00395029662904939,
-0.00978957963072948));
#33300=CARTESIAN_POINT('Ctrl Pts',(-0.212131423698469,0.00384219210363941,
-0.00974368374009559));
#33301=CARTESIAN_POINT('Ctrl Pts',(-0.212142046213562,0.00374522463100718,
-0.0097004800320845));
#33302=CARTESIAN_POINT('Ctrl Pts',(-0.212152668728655,0.00364825715837495,
-0.0096572763240734));
#33303=CARTESIAN_POINT('Ctrl Pts',(-0.212163048553079,0.00356223260132983,
-0.00961718215571804));
#33304=CARTESIAN_POINT('Ctrl Pts',(-0.21217478537429,0.00346950464697697,
-0.00957214819609432));
#33305=CARTESIAN_POINT('Ctrl Pts',(-0.212180653784895,0.00342314066980054,
-0.00954963121628245));
#33306=CARTESIAN_POINT('Ctrl Pts',(-0.212186862003761,0.00337511703119302,
-0.00952585173312588));
#33307=CARTESIAN_POINT('Ctrl Pts',(-0.212193910295831,0.00332246376500242,
-0.00949911215485694));
#33308=CARTESIAN_POINT('Ctrl Pts',(-0.2122009585879,0.00326981049881182,
-0.00947237257658799));
#33309=CARTESIAN_POINT('Ctrl Pts',(-0.212208849875716,0.0032125970416991,
-0.00944253293996776));
#33310=CARTESIAN_POINT('Ctrl Pts',(-0.21221487211149,0.00316961435383794,
-0.00941968492124474));
#33311=CARTESIAN_POINT('Ctrl Pts',(-0.212220894347265,0.00312663166597678,
-0.00939683690252173));
#33312=CARTESIAN_POINT('Ctrl Pts',(-0.212225043125917,0.00309776524461444,
-0.00938119425465462));
#33313=CARTESIAN_POINT('Ctrl Pts',(-0.212230393485056,0.00306084166967678,
-0.00936092826695534));
#33314=CARTESIAN_POINT('Ctrl Pts',(-0.212235743844195,0.00302391809473912,
-0.00934066227925607));
#33315=CARTESIAN_POINT('Ctrl Pts',(-0.212242298250575,0.00297900456721415,
-0.00931565235421951));
#33316=CARTESIAN_POINT('Ctrl Pts',(-0.212249286853305,0.00293173364208715,
-0.00928871011573586));
#33317=CARTESIAN_POINT('Ctrl Pts',(-0.212263264021031,0.00283719204706346,
-0.00923482578423803));
#33318=CARTESIAN_POINT('Ctrl Pts',(-0.212278973919057,0.00273310083018332,
-0.0091734129978045));
#33319=CARTESIAN_POINT('Ctrl Pts',(-0.212297189426323,0.00261509213602985,
-0.00909974167633009));
#33320=CARTESIAN_POINT('',(-0.20229073069173,0.00260802819594702,-0.00889711922744007));
#33321=CARTESIAN_POINT('',(-0.201088519916106,0.00260697650863716,-0.00887281289522955));
#33322=CARTESIAN_POINT('',(-0.202290729582105,0.00260802964547657,-0.0088971142446013));
#33323=CARTESIAN_POINT('',(-0.200997253167062,0.00750071976884877,-0.0102503476155925));
#33324=CARTESIAN_POINT('Ctrl Pts',(-0.201088517234415,0.00260697768703412,
-0.00887281028342328));
#33325=CARTESIAN_POINT('Ctrl Pts',(-0.201070231378405,0.00272574422538841,
-0.00894517065855103));
#33326=CARTESIAN_POINT('Ctrl Pts',(-0.20104660700157,0.00288268449617453,
-0.00903571755969753));
#33327=CARTESIAN_POINT('Ctrl Pts',(-0.201020428886199,0.00306324011348402,
-0.00913380586456596));
#33328=CARTESIAN_POINT('Ctrl Pts',(-0.201008031521991,0.00315009960764293,
-0.00917988033017122));
#33329=CARTESIAN_POINT('Ctrl Pts',(-0.200984567569492,0.00332254158062,
-0.00926785663333399));
#33330=CARTESIAN_POINT('Ctrl Pts',(-0.200960305513351,0.00351465179944262,
-0.00936066460635266));
#33331=CARTESIAN_POINT('Ctrl Pts',(-0.200923777451925,0.00382954798428417,
-0.00950417474699339));
#33332=CARTESIAN_POINT('Ctrl Pts',(-0.200882155475116,0.00433605979405848,
-0.00970630389687771));
#33333=CARTESIAN_POINT('Ctrl Pts',(-0.200862761315044,0.00496362486152777,
-0.00990440070219615));
#33334=CARTESIAN_POINT('Ctrl Pts',(-0.200867614140204,0.00544563190383476,
-0.0100236066604576));
#33335=CARTESIAN_POINT('Ctrl Pts',(-0.200881077294953,0.005828723981634,
-0.0100982028485135));
#33336=CARTESIAN_POINT('Ctrl Pts',(-0.200891145223225,0.00604404165042094,
-0.010134424351333));
#33337=CARTESIAN_POINT('Ctrl Pts',(-0.200901663721965,0.00623413010597689,
-0.0101623574414713));
#33338=CARTESIAN_POINT('Ctrl Pts',(-0.200907769791474,0.00633199116033011,
-0.0101751201838898));
#33339=CARTESIAN_POINT('Ctrl Pts',(-0.200919720793469,0.00651408529372874,
-0.010197196127569));
#33340=CARTESIAN_POINT('Ctrl Pts',(-0.200944415623066,0.00685633873757801,
-0.0102308035714179));
#33341=CARTESIAN_POINT('Ctrl Pts',(-0.200974002174022,0.00722536468550294,
-0.0102498434994338));
#33342=CARTESIAN_POINT('Ctrl Pts',(-0.200997253167062,0.00750071976884877,
-0.0102503476155925));
#33343=CARTESIAN_POINT('',(-0.201091338207746,0.0123976804872637,-0.00887001172820126));
#33344=CARTESIAN_POINT('Ctrl Pts',(-0.200997253189733,0.00750072003734376,
-0.0102503476160841));
#33345=CARTESIAN_POINT('Ctrl Pts',(-0.200974226058333,0.00777622966032588,
-0.0102498057883578));
#33346=CARTESIAN_POINT('Ctrl Pts',(-0.200944926608782,0.00814550668245003,
-0.0102306939411073));
#33347=CARTESIAN_POINT('Ctrl Pts',(-0.200920475693722,0.00848807026377426,
-0.0101969861106214));
#33348=CARTESIAN_POINT('Ctrl Pts',(-0.200908644715003,0.00867036462369381,
-0.0101748434138683));
#33349=CARTESIAN_POINT('Ctrl Pts',(-0.200902600687783,0.00876833805227905,
-0.010162042409973));
#33350=CARTESIAN_POINT('Ctrl Pts',(-0.200892191101917,0.00895870315128538,
-0.0101340170690275));
#33351=CARTESIAN_POINT('Ctrl Pts',(-0.200882239017754,0.00917425974551143,
-0.010097690760335));
#33352=CARTESIAN_POINT('Ctrl Pts',(-0.200868964749715,0.00955773818742233,
-0.0100228808043527));
#33353=CARTESIAN_POINT('Ctrl Pts',(-0.200864271521825,0.0100393106820076,
-0.00990363217018893));
#33354=CARTESIAN_POINT('Ctrl Pts',(-0.200883875554183,0.0106684281424501,
-0.00970474543934178));
#33355=CARTESIAN_POINT('Ctrl Pts',(-0.200925612659579,0.0111740766689703,
-0.00950266590494921));
#33356=CARTESIAN_POINT('Ctrl Pts',(-0.200962341330629,0.0114892663409321,
-0.00935886602107145));
#33357=CARTESIAN_POINT('Ctrl Pts',(-0.200986739504071,0.0116814829294643,
-0.00926589566588928));
#33358=CARTESIAN_POINT('Ctrl Pts',(-0.201010344072047,0.0118540654419843,
-0.00917774291603716));
#33359=CARTESIAN_POINT('Ctrl Pts',(-0.201022808712449,0.0119409346873194,
-0.00913160785205659));
#33360=CARTESIAN_POINT('Ctrl Pts',(-0.201049148976313,0.0121216430743756,
-0.00903331926895959));
#33361=CARTESIAN_POINT('Ctrl Pts',(-0.201072928578555,0.0122787618858155,
-0.00894255830868901));
#33362=CARTESIAN_POINT('Ctrl Pts',(-0.201091338207746,0.0123976804872637,
-0.00887001172820126));
#33363=CARTESIAN_POINT('',(-0.202293074116991,0.0123964300494642,-0.00889443311216738));
#33364=CARTESIAN_POINT('',(-0.201091338329048,0.0123976767118359,-0.00887000556980743));
#33365=CARTESIAN_POINT('',(-0.202197548254198,0.00750045600863564,-0.0102774753127245));
#33366=CARTESIAN_POINT('Ctrl Pts',(-0.202293072280915,0.0123964287538336,
-0.00889443052768938));
#33367=CARTESIAN_POINT('Ctrl Pts',(-0.202274494498572,0.0122768166966399,
-0.00896759163493234));
#33368=CARTESIAN_POINT('Ctrl Pts',(-0.202258537883566,0.012171743084332,
-0.00902831707970255));
#33369=CARTESIAN_POINT('Ctrl Pts',(-0.202244401605263,0.0120766332932925,
-0.00908143808158457));
#33370=CARTESIAN_POINT('Ctrl Pts',(-0.202237333434346,0.0120290781840582,
-0.00910799870189006));
#33371=CARTESIAN_POINT('Ctrl Pts',(-0.20223072137725,0.0119839839266795,
-0.00913260678336198));
#33372=CARTESIAN_POINT('Ctrl Pts',(-0.202225363198743,0.0119471877968328,
-0.00915240392969132));
#33373=CARTESIAN_POINT('Ctrl Pts',(-0.202220005020236,0.0119103916669861,
-0.00917220107602065));
#33374=CARTESIAN_POINT('Ctrl Pts',(-0.202215898250785,0.0118819602340639,
-0.0091873091097473));
#33375=CARTESIAN_POINT('Ctrl Pts',(-0.202209856163251,0.0118388980500071,
-0.00920975838000546));
#33376=CARTESIAN_POINT('Ctrl Pts',(-0.202203814075716,0.0117958358659502,
-0.00923220765026362));
#33377=CARTESIAN_POINT('Ctrl Pts',(-0.202195841123907,0.0117380282236051,
-0.00926178017206805));
#33378=CARTESIAN_POINT('Ctrl Pts',(-0.202188777096842,0.0116850814160394,
-0.00928815591228989));
#33379=CARTESIAN_POINT('Ctrl Pts',(-0.202181713069777,0.0116321346084737,
-0.00931453165251173));
#33380=CARTESIAN_POINT('Ctrl Pts',(-0.202175554902053,0.0115841212056271,
-0.00933785864569768));
#33381=CARTESIAN_POINT('Ctrl Pts',(-0.202169685062092,0.0115371577243816,
-0.00936023633717544));
#33382=CARTESIAN_POINT('Ctrl Pts',(-0.202157945382171,0.0114432307618907,
-0.00940499172013097));
#33383=CARTESIAN_POINT('Ctrl Pts',(-0.202147359312351,0.011353504796092,
-0.0094459379756937));
#33384=CARTESIAN_POINT('Ctrl Pts',(-0.202137462087568,0.011259896757467,
-0.00948687411303633));
#33385=CARTESIAN_POINT('Ctrl Pts',(-0.202120092033886,0.0110956106377205,
-0.00955871878856009));
#33386=CARTESIAN_POINT('Ctrl Pts',(-0.202104854053046,0.0109191718891678,
-0.00963009428879758));
#33387=CARTESIAN_POINT('Ctrl Pts',(-0.202093387924333,0.0107391546369728,
-0.00969630675200009));
#33388=CARTESIAN_POINT('Ctrl Pts',(-0.202091787558797,0.0107140290332449,
-0.00970554824464586));
#33389=CARTESIAN_POINT('Ctrl Pts',(-0.202090260671614,0.0106888351820918,
-0.00971469236466777));
#33390=CARTESIAN_POINT('Ctrl Pts',(-0.202088811721322,0.0106635979043288,
-0.00972372989803367));
#33391=CARTESIAN_POINT('Ctrl Pts',(-0.202076981486153,0.0104575432641258,
-0.00979751858885518));
#33392=CARTESIAN_POINT('Ctrl Pts',(-0.20207034465538,0.0102484667046851,
-0.00986398925107306));
#33393=CARTESIAN_POINT('Ctrl Pts',(-0.202067972793861,0.0100475507252513,
-0.00992073131987059));
#33394=CARTESIAN_POINT('Ctrl Pts',(-0.202065600932341,0.00984663474581746,
-0.00997747338866811));
#33395=CARTESIAN_POINT('Ctrl Pts',(-0.202067476359534,0.00965412391713009,
-0.0100252955433957));
#33396=CARTESIAN_POINT('Ctrl Pts',(-0.202073202188225,0.00944386085916814,
-0.0100700604354503));
#33397=CARTESIAN_POINT('Ctrl Pts',(-0.20207606510257,0.00933872933018716,
-0.0100924428814776));
#33398=CARTESIAN_POINT('Ctrl Pts',(-0.202079895387504,0.00922911533405485,
-0.0101138466780218));
#33399=CARTESIAN_POINT('Ctrl Pts',(-0.202084523624796,0.00912069371656406,
-0.010133028299003));
#33400=CARTESIAN_POINT('Ctrl Pts',(-0.202086837743442,0.00906648290781867,
-0.0101426191094935));
#33401=CARTESIAN_POINT('Ctrl Pts',(-0.202089350290228,0.00901257874257112,
-0.0101517018283888));
#33402=CARTESIAN_POINT('Ctrl Pts',(-0.202092361027929,0.00895383404463594,
-0.0101610201059614));
#33403=CARTESIAN_POINT('Ctrl Pts',(-0.20209537176563,0.00889508934670077,
-0.010170338383534));
#33404=CARTESIAN_POINT('Ctrl Pts',(-0.202098884187202,0.00883147883691273,
-0.0101797361479915));
#33405=CARTESIAN_POINT('Ctrl Pts',(-0.202101649554293,0.00878349099574898,
-0.0101864567721823));
#33406=CARTESIAN_POINT('Ctrl Pts',(-0.202104414921384,0.00873550315458523,
-0.0101931773963731));
#33407=CARTESIAN_POINT('Ctrl Pts',(-0.202106428339549,0.00870316764003492,
-0.0101974389521304));
#33408=CARTESIAN_POINT('Ctrl Pts',(-0.202108920491588,0.00866427834590321,
-0.0102023845624647));
#33409=CARTESIAN_POINT('Ctrl Pts',(-0.202111412643626,0.00862538905177151,
-0.0102073301727989));
#33410=CARTESIAN_POINT('Ctrl Pts',(-0.20211438615768,0.00857993192696311,
-0.0102128429215111));
#33411=CARTESIAN_POINT('Ctrl Pts',(-0.20211753897259,0.00853333627651013,
-0.0102181086866933));
#33412=CARTESIAN_POINT('Ctrl Pts',(-0.20212384460241,0.00844014497560417,
-0.0102286402170578));
#33413=CARTESIAN_POINT('Ctrl Pts',(-0.202130864181834,0.00834241335367361,
-0.0102383282389047));
#33414=CARTESIAN_POINT('Ctrl Pts',(-0.202138818565719,0.00823614458621563,
-0.0102469384026684));
#33415=CARTESIAN_POINT('Ctrl Pts',(-0.20215472733349,0.00802360705129966,
-0.0102641587301959));
#33416=CARTESIAN_POINT('Ctrl Pts',(-0.202174378256334,0.00777691961388399,
-0.0102769379987594));
#33417=CARTESIAN_POINT('Ctrl Pts',(-0.202197548276474,0.00750045623478144,
-0.010277475295121));
#33418=CARTESIAN_POINT('Ctrl Pts',(-0.202197548257345,0.00750045600840331,
-0.0102774752946998));
#33419=CARTESIAN_POINT('Ctrl Pts',(-0.202174203175516,0.00722418787536874,
-0.0102769612949105));
#33420=CARTESIAN_POINT('Ctrl Pts',(-0.202154402182172,0.00697769519644182,
-0.0102642204595934));
#33421=CARTESIAN_POINT('Ctrl Pts',(-0.202138370075718,0.0067653447285158,
-0.010247046325628));
#33422=CARTESIAN_POINT('Ctrl Pts',(-0.202130354020302,0.0066591694655523,
-0.0102384592562998));
#33423=CARTESIAN_POINT('Ctrl Pts',(-0.202123279456543,0.00656152943931938,
-0.0102287961037126));
#33424=CARTESIAN_POINT('Ctrl Pts',(-0.202116923777592,0.0064684343667805,
-0.0102182920830441));
#33425=CARTESIAN_POINT('Ctrl Pts',(-0.202113745938117,0.00642188683051106,
-0.0102130400727099));
#33426=CARTESIAN_POINT('Ctrl Pts',(-0.202110748631194,0.00637647896299386,
-0.0102075418327333));
#33427=CARTESIAN_POINT('Ctrl Pts',(-0.202108236329092,0.00633763121108928,
-0.010202609085463));
#33428=CARTESIAN_POINT('Ctrl Pts',(-0.202105724026989,0.0062987834591847,
-0.0101976763381926));
#33429=CARTESIAN_POINT('Ctrl Pts',(-0.202103694108944,0.00626648183425165,
-0.010193425669544));
#33430=CARTESIAN_POINT('Ctrl Pts',(-0.2021009060143,0.00621855639123403,
-0.010186723946201));
#33431=CARTESIAN_POINT('Ctrl Pts',(-0.202098117919657,0.00617063094821641,
-0.010180022222858));
#33432=CARTESIAN_POINT('Ctrl Pts',(-0.202094576527078,0.00610711120290014,
-0.0101706520808344));
#33433=CARTESIAN_POINT('Ctrl Pts',(-0.202091539695686,0.00604844186568722,
-0.0101613598309362));
#33434=CARTESIAN_POINT('Ctrl Pts',(-0.202088502864294,0.0059897725284743,
-0.0101520675810381));
#33435=CARTESIAN_POINT('Ctrl Pts',(-0.202085967113789,0.00593592844766217,
-0.0101430087253429));
#33436=CARTESIAN_POINT('Ctrl Pts',(-0.202083630277739,0.00588177702189636,
-0.0101334427620972));
#33437=CARTESIAN_POINT('Ctrl Pts',(-0.202078956605641,0.00577347417036475,
-0.0101143108356057));
#33438=CARTESIAN_POINT('Ctrl Pts',(-0.202075082802893,0.00566397593382631,
-0.0100929619309007));
#33439=CARTESIAN_POINT('Ctrl Pts',(-0.202072182143848,0.00555889914283848,
-0.0100706232669665));
#33440=CARTESIAN_POINT('Ctrl Pts',(-0.202066380825758,0.00534874556086281,
-0.0100259459390981));
#33441=CARTESIAN_POINT('Ctrl Pts',(-0.202064453366962,0.00515610306662607,
-0.00997815057565958));
#33442=CARTESIAN_POINT('Ctrl Pts',(-0.202066768684074,0.00495539428595943,
-0.00992153686344134));
#33443=CARTESIAN_POINT('Ctrl Pts',(-0.202069084001186,0.00475468550529279,
-0.0098649231512231));
#33444=CARTESIAN_POINT('Ctrl Pts',(-0.202075659074073,0.00454614650373027,
-0.00979871421367979));
#33445=CARTESIAN_POINT('Ctrl Pts',(-0.202087442152237,0.00434017468158449,
-0.00972505509448496));
#33446=CARTESIAN_POINT('Ctrl Pts',(-0.202088957696926,0.00431368249535475,
-0.00971558102622213));
#33447=CARTESIAN_POINT('Ctrl Pts',(-0.202090559446696,0.00428723079419437,
-0.00970598690689844));
#33448=CARTESIAN_POINT('Ctrl Pts',(-0.202092242088241,0.00426085025377553,
-0.00969628392349822));
#33449=CARTESIAN_POINT('Ctrl Pts',(-0.202103641671852,0.00408212699746957,
-0.00963054801507335));
#33450=CARTESIAN_POINT('Ctrl Pts',(-0.202118754034746,0.00390674732751332,
-0.00955964449039378));
#33451=CARTESIAN_POINT('Ctrl Pts',(-0.20213592699882,0.00374367671188409,
-0.00948841157134542));
#33452=CARTESIAN_POINT('Ctrl Pts',(-0.202145780893062,0.0036501063419974,
-0.00944753792554636));
#33453=CARTESIAN_POINT('Ctrl Pts',(-0.202156309756316,0.00356052315313633,
-0.00940670249336416));
#33454=CARTESIAN_POINT('Ctrl Pts',(-0.20216799037999,0.00346667879554435,
-0.00936203806939491));
#33455=CARTESIAN_POINT('Ctrl Pts',(-0.202173830691827,0.00341975661674836,
-0.00933970585741029));
#33456=CARTESIAN_POINT('Ctrl Pts',(-0.202179958877149,0.00337176970234555,
-0.00931641897443527));
#33457=CARTESIAN_POINT('Ctrl Pts',(-0.202186990410553,0.00331883357972307,
-0.00929007896089968));
#33458=CARTESIAN_POINT('Ctrl Pts',(-0.202194021943957,0.0032658974571006,
-0.00926373894736408));
#33459=CARTESIAN_POINT('Ctrl Pts',(-0.202201959897997,0.00320808475490152,
-0.00923419745669377));
#33460=CARTESIAN_POINT('Ctrl Pts',(-0.202207969334436,0.0031650605155377,
-0.00921179363609146));
#33461=CARTESIAN_POINT('Ctrl Pts',(-0.202213978770875,0.00312203627617388,
-0.00918938981548915));
#33462=CARTESIAN_POINT('Ctrl Pts',(-0.202218055227422,0.00309368573465424,
-0.00917434201417049));
#33463=CARTESIAN_POINT('Ctrl Pts',(-0.202223379993947,0.00305695144231377,
-0.00915460154150268));
#33464=CARTESIAN_POINT('Ctrl Pts',(-0.202228704760472,0.00302021714997329,
-0.00913486106883488));
#33465=CARTESIAN_POINT('Ctrl Pts',(-0.202235280308945,0.00297516564357389,
-0.0091103060139232));
#33466=CARTESIAN_POINT('Ctrl Pts',(-0.202242310233515,0.00292764956256295,
-0.00908379936175299));
#33467=CARTESIAN_POINT('Ctrl Pts',(-0.202256370042748,0.00283261767028968,
-0.00903078620789074));
#33468=CARTESIAN_POINT('Ctrl Pts',(-0.202272243236238,0.00272760700184593,
-0.00897017266924841));
#33469=CARTESIAN_POINT('Ctrl Pts',(-0.202290729295407,0.00260802662900566,
-0.00889712143907862));
#33470=CARTESIAN_POINT('',(-0.200288489608108,0.00260606627767471,-0.0088565175084996));
#33471=CARTESIAN_POINT('',(-0.199085603811712,0.00260467847622167,-0.00883205133599132));
#33472=CARTESIAN_POINT('',(-0.200288488520405,0.00260606784889207,-0.0088565123499802));
#33473=CARTESIAN_POINT('',(-0.198998268035306,0.00750170158931661,-0.0102051687696475));
#33474=CARTESIAN_POINT('Ctrl Pts',(-0.199085601119488,0.00260467972009568,
-0.00883204861089906));
#33475=CARTESIAN_POINT('Ctrl Pts',(-0.199067506452137,0.00272371785988628,
-0.00890426028999085));
#33476=CARTESIAN_POINT('Ctrl Pts',(-0.199044131665411,0.00288099175507442,
-0.00899460795740418));
#33477=CARTESIAN_POINT('Ctrl Pts',(-0.199018239202327,0.00306188063533018,
-0.00909245634302826));
#33478=CARTESIAN_POINT('Ctrl Pts',(-0.199005978008815,0.00314889853402773,
-0.00913841719159824));
#33479=CARTESIAN_POINT('Ctrl Pts',(-0.198982790163463,0.00332156603532327,
-0.00922613374755011));
#33480=CARTESIAN_POINT('Ctrl Pts',(-0.198958825555564,0.0035139176367545,
-0.00931866793364172));
#33481=CARTESIAN_POINT('Ctrl Pts',(-0.198922764022766,0.003829290069547,
-0.00946178592376709));
#33482=CARTESIAN_POINT('Ctrl Pts',(-0.198881879694765,0.00433562257220421,
-0.00966303763238278));
#33483=CARTESIAN_POINT('Ctrl Pts',(-0.198863131383457,0.00496409099012789,
-0.00986064921761845));
#33484=CARTESIAN_POINT('Ctrl Pts',(-0.198868335412294,0.00544577509415154,
-0.00997929788943944));
#33485=CARTESIAN_POINT('Ctrl Pts',(-0.198881970765267,0.00582907039941651,
-0.010053649419941));
#33486=CARTESIAN_POINT('Ctrl Pts',(-0.198892111562041,0.00604451891685977,
-0.0100897483235882));
#33487=CARTESIAN_POINT('Ctrl Pts',(-0.198902678405336,0.0062347615700293,
-0.0101175891596819));
#33488=CARTESIAN_POINT('Ctrl Pts',(-0.19890880151892,0.00633269713647193,
-0.0101303069565454));
#33489=CARTESIAN_POINT('Ctrl Pts',(-0.198920775760608,0.00651489848546796,
-0.0101522995605522));
#33490=CARTESIAN_POINT('Ctrl Pts',(-0.198945485503522,0.00685728554587353,
-0.0101857637123629));
#33491=CARTESIAN_POINT('Ctrl Pts',(-0.198975049131093,0.00722635221066761,
-0.010204694340746));
#33492=CARTESIAN_POINT('Ctrl Pts',(-0.198998268035306,0.00750170158931661,
-0.0102051687696475));
#33493=CARTESIAN_POINT('',(-0.199090547585037,0.0123998542045573,-0.00882937998736431));
#33494=CARTESIAN_POINT('Ctrl Pts',(-0.198998268042099,0.0075017016698774,
-0.0102051687697863));
#33495=CARTESIAN_POINT('Ctrl Pts',(-0.198975262697197,0.00777716699517044,
-0.0102045984688354));
#33496=CARTESIAN_POINT('Ctrl Pts',(-0.19894598350055,0.00814639028559267,
-0.0101855245739562));
#33497=CARTESIAN_POINT('Ctrl Pts',(-0.198921535655541,0.00848891979571509,
-0.0101519135771396));
#33498=CARTESIAN_POINT('Ctrl Pts',(-0.198909699198878,0.00867120867347047,
-0.0101298369351647));
#33499=CARTESIAN_POINT('Ctrl Pts',(-0.198903651182801,0.0087691668271986,
-0.010117076818613));
#33500=CARTESIAN_POINT('Ctrl Pts',(-0.198893222445148,0.0089595786910395,
-0.0100891311615914));
#33501=CARTESIAN_POINT('Ctrl Pts',(-0.198883240814823,0.00917515726562705,
-0.0100529157275236));
#33502=CARTESIAN_POINT('Ctrl Pts',(-0.198869893334788,0.00955867496945718,
-0.00997833705459149));
#33503=CARTESIAN_POINT('Ctrl Pts',(-0.198865044854715,0.0100400285423306,
-0.00985955619907535));
#33504=CARTESIAN_POINT('Ctrl Pts',(-0.198884354860069,0.0106695831171145,
-0.00966124188583534));
#33505=CARTESIAN_POINT('Ctrl Pts',(-0.198925753482806,0.0111752154117488,
-0.00945993219594404));
#33506=CARTESIAN_POINT('Ctrl Pts',(-0.198962259694651,0.011490639491165,
-0.00931660497153037));
#33507=CARTESIAN_POINT('Ctrl Pts',(-0.198986515375409,0.0116829856636076,
-0.00922395071753861));
#33508=CARTESIAN_POINT('Ctrl Pts',(-0.199009988182743,0.011855702949848,
-0.0091360949988362));
#33509=CARTESIAN_POINT('Ctrl Pts',(-0.199022383731062,0.0119426366934164,
-0.00909011953258369));
#33510=CARTESIAN_POINT('Ctrl Pts',(-0.199048581320397,0.0121235063356898,
-0.00899215974570331));
#33511=CARTESIAN_POINT('Ctrl Pts',(-0.19907223476441,0.0122807914137443,
-0.00890169526387644));
#33512=CARTESIAN_POINT('Ctrl Pts',(-0.199090547585037,0.0123998542045573,
-0.00882937998736431));
#33513=CARTESIAN_POINT('',(-0.200292338257129,0.0123986218814099,-0.00885373242023577));
#33514=CARTESIAN_POINT('',(-0.1990905477074,0.0123998504040343,-0.00882937376053058));
#33515=CARTESIAN_POINT('',(-0.200198408071207,0.00750103329744417,-0.0102322930460279));
#33516=CARTESIAN_POINT('Ctrl Pts',(-0.200292336411079,0.0123986205739213,
-0.00885372980557329));
#33517=CARTESIAN_POINT('Ctrl Pts',(-0.200273857423805,0.0122788598610061,
-0.00892666423347511));
#33518=CARTESIAN_POINT('Ctrl Pts',(-0.200257986138083,0.0121736699411429,
-0.00898719795378537));
#33519=CARTESIAN_POINT('Ctrl Pts',(-0.2002439262477,0.0120784622944802,
-0.00904014962650077));
#33520=CARTESIAN_POINT('Ctrl Pts',(-0.20023689627133,0.0120308582600157,
-0.00906662558028448));
#33521=CARTESIAN_POINT('Ctrl Pts',(-0.200230320168875,0.0119857198874726,
-0.00909115471047935));
#33522=CARTESIAN_POINT('Ctrl Pts',(-0.200224991193952,0.0119488887897826,
-0.0091108881514725));
#33523=CARTESIAN_POINT('Ctrl Pts',(-0.200219662219028,0.0119120576920926,
-0.00913062159246565));
#33524=CARTESIAN_POINT('Ctrl Pts',(-0.20021557791321,0.0118835999835593,
-0.00914568084411158));
#33525=CARTESIAN_POINT('Ctrl Pts',(-0.200209569574122,0.0118404999931127,
-0.00916805714683687));
#33526=CARTESIAN_POINT('Ctrl Pts',(-0.200203561235034,0.0117974000026662,
-0.00919043344956217));
#33527=CARTESIAN_POINT('Ctrl Pts',(-0.200195633296685,0.0117395438100094,
-0.00921990941307956));
#33528=CARTESIAN_POINT('Ctrl Pts',(-0.200188609958376,0.0116865548788483,
-0.00924619873884898));
#33529=CARTESIAN_POINT('Ctrl Pts',(-0.200181586620067,0.0116335659476873,
-0.0092724880646184));
#33530=CARTESIAN_POINT('Ctrl Pts',(-0.200175464829421,0.0115855163576409,
-0.00929573837995581));
#33531=CARTESIAN_POINT('Ctrl Pts',(-0.200169630008592,0.0115385156030165,
-0.00931804389564718));
#33532=CARTESIAN_POINT('Ctrl Pts',(-0.200157960366936,0.0114445140937676,
-0.00936265492702992));
#33533=CARTESIAN_POINT('Ctrl Pts',(-0.200147438913252,0.0113547089314509,
-0.00940347437178023));
#33534=CARTESIAN_POINT('Ctrl Pts',(-0.200137609106914,0.0112610547873119,
-0.00944427013630663));
#33535=CARTESIAN_POINT('Ctrl Pts',(-0.200120051269694,0.0110937713067034,
-0.00951713885500349));
#33536=CARTESIAN_POINT('Ctrl Pts',(-0.200104710590186,0.0109140070200952,
-0.0095894788353709));
#33537=CARTESIAN_POINT('Ctrl Pts',(-0.200093291444196,0.0107306172547326,
-0.0096564589648824));
#33538=CARTESIAN_POINT('Ctrl Pts',(-0.200091924505863,0.0107086644308998,
-0.00966447687679018));
#33539=CARTESIAN_POINT('Ctrl Pts',(-0.200090613761087,0.010686660781902,
-0.00967242046945206));
#33540=CARTESIAN_POINT('Ctrl Pts',(-0.200089362133423,0.0106646224704097,
-0.00968028375905126));
#33541=CARTESIAN_POINT('Ctrl Pts',(-0.200077654643436,0.010458480245711,
-0.00975383549244965));
#33542=CARTESIAN_POINT('Ctrl Pts',(-0.200071117844305,0.010249176179895,
-0.00982014029840789));
#33543=CARTESIAN_POINT('Ctrl Pts',(-0.200068825516657,0.0100482127987205,
-0.00987669426350142));
#33544=CARTESIAN_POINT('Ctrl Pts',(-0.20006653318901,0.00984724941754597,
-0.00993324822859494));
#33545=CARTESIAN_POINT('Ctrl Pts',(-0.200068467409846,0.00965487328195331,
-0.00998087145327418));
#33546=CARTESIAN_POINT('Ctrl Pts',(-0.200074230964292,0.00944461437737611,
-0.0100254863843596));
#33547=CARTESIAN_POINT('Ctrl Pts',(-0.200077112741515,0.00933948492508751,
-0.0100477938499023));
#33548=CARTESIAN_POINT('Ctrl Pts',(-0.200080956650382,0.00922984032252973,
-0.0100691336047581));
#33549=CARTESIAN_POINT('Ctrl Pts',(-0.200085593257487,0.00912138630961319,
-0.0100882582187389));
#33550=CARTESIAN_POINT('Ctrl Pts',(-0.20008791156104,0.00906715930315493,
-0.0100978205257293));
#33551=CARTESIAN_POINT('Ctrl Pts',(-0.200090426979645,0.00901323845330599,
-0.0101068764881864));
#33552=CARTESIAN_POINT('Ctrl Pts',(-0.200093439296429,0.00895446814128281,
-0.0101161684714052));
#33553=CARTESIAN_POINT('Ctrl Pts',(-0.200096451613213,0.00889569782925962,
-0.0101254604546241));
#33554=CARTESIAN_POINT('Ctrl Pts',(-0.20009996431432,0.00883205290627755,
-0.0101348326651809));
#33555=CARTESIAN_POINT('Ctrl Pts',(-0.200102728596934,0.00878404736045819,
-0.0101415338671528));
#33556=CARTESIAN_POINT('Ctrl Pts',(-0.200105492879549,0.00873604181463882,
-0.0101482350691247));
#33557=CARTESIAN_POINT('Ctrl Pts',(-0.200107503860301,0.00870370514200726,
-0.0101524828667423));
#33558=CARTESIAN_POINT('Ctrl Pts',(-0.200109992697036,0.00866481179141373,
-0.0101574129882443));
#33559=CARTESIAN_POINT('Ctrl Pts',(-0.200112481533771,0.0086259184408202,
-0.0101623431097463));
#33560=CARTESIAN_POINT('Ctrl Pts',(-0.200115450847707,0.008580454442893,
-0.0101678389360936));
#33561=CARTESIAN_POINT('Ctrl Pts',(-0.200118598464806,0.00853385386382148,
-0.010173088425976));
#33562=CARTESIAN_POINT('Ctrl Pts',(-0.200124893699004,0.00844065270567845,
-0.0101835874057408));
#33563=CARTESIAN_POINT('Ctrl Pts',(-0.200131898901286,0.0083429189224858,
-0.010193245062841));
#33564=CARTESIAN_POINT('Ctrl Pts',(-0.20013983500335,0.00823665261474254,
-0.0102018289916747));
#33565=CARTESIAN_POINT('Ctrl Pts',(-0.200155707207479,0.00802411999925601,
-0.0102189968493419));
#33566=CARTESIAN_POINT('Ctrl Pts',(-0.200175305948972,0.00777745593880945,
-0.0102317401265822));
#33567=CARTESIAN_POINT('Ctrl Pts',(-0.200198408092455,0.00750103375755189,
-0.0102322930261764));
#33568=CARTESIAN_POINT('Ctrl Pts',(-0.200198408053672,0.00750103329896434,
-0.0102322930253509));
#33569=CARTESIAN_POINT('Ctrl Pts',(-0.2001750414276,0.00722473781003592,
-0.0102317956646293));
#33570=CARTESIAN_POINT('Ctrl Pts',(-0.200155217020202,0.00697821917512664,
-0.0102191136148449));
#33571=CARTESIAN_POINT('Ctrl Pts',(-0.200139160143905,0.00676583736411692,
-0.0102020103849557));
#33572=CARTESIAN_POINT('Ctrl Pts',(-0.200131131701314,0.00665964639986116,
-0.0101934587652799));
#33573=CARTESIAN_POINT('Ctrl Pts',(-0.200124044414963,0.00656198933436801,
-0.0101838339575191));
#33574=CARTESIAN_POINT('Ctrl Pts',(-0.200117675154785,0.00646887989036955,
-0.0101733710542036));
#33575=CARTESIAN_POINT('Ctrl Pts',(-0.200114490524696,0.00642232516837032,
-0.0101681396025458));
#33576=CARTESIAN_POINT('Ctrl Pts',(-0.200111486208921,0.00637691075266694,
-0.0101626627715528));
#33577=CARTESIAN_POINT('Ctrl Pts',(-0.200108967406514,0.00633805215836633,
-0.0101577484283255));
#33578=CARTESIAN_POINT('Ctrl Pts',(-0.200106448604107,0.00629919356406571,
-0.0101528340850982));
#33579=CARTESIAN_POINT('Ctrl Pts',(-0.200104412705854,0.00626687691983241,
-0.0101485983115396));
#33580=CARTESIAN_POINT('Ctrl Pts',(-0.200101616155769,0.00621895242659197,
-0.0101419232912671));
#33581=CARTESIAN_POINT('Ctrl Pts',(-0.200098819605684,0.00617102793335153,
-0.0101352482709947));
#33582=CARTESIAN_POINT('Ctrl Pts',(-0.200095267259168,0.00610752485173003,
-0.0101259176528732));
#33583=CARTESIAN_POINT('Ctrl Pts',(-0.200092218919278,0.00604886456963942,
-0.0101166636401912));
#33584=CARTESIAN_POINT('Ctrl Pts',(-0.200089170579389,0.0059902042875488,
-0.0101074096275093));
#33585=CARTESIAN_POINT('Ctrl Pts',(-0.200086622783407,0.00593636187616354,
-0.0100983869607788));
#33586=CARTESIAN_POINT('Ctrl Pts',(-0.200084272753936,0.00588221105991508,
-0.0100888589275013));
#33587=CARTESIAN_POINT('Ctrl Pts',(-0.200079572694994,0.00577390942741817,
-0.0100698028609464));
#33588=CARTESIAN_POINT('Ctrl Pts',(-0.20007566789051,0.00566440786363879,
-0.0100485377791556));
#33589=CARTESIAN_POINT('Ctrl Pts',(-0.200072733636695,0.00555930929747007,
-0.0100262824238011));
#33590=CARTESIAN_POINT('Ctrl Pts',(-0.200066865129066,0.00534911216513262,
-0.00998177171309202));
#33591=CARTESIAN_POINT('Ctrl Pts',(-0.200064860248902,0.00515635425120098,
-0.0099341348136642));
#33592=CARTESIAN_POINT('Ctrl Pts',(-0.200067068255993,0.00495556995531808,
-0.00987772033772398));
#33593=CARTESIAN_POINT('Ctrl Pts',(-0.200069276263084,0.00475478565943518,
-0.00982130586178375));
#33594=CARTESIAN_POINT('Ctrl Pts',(-0.200075713987207,0.004546208178983,
-0.00975534338054551));
#33595=CARTESIAN_POINT('Ctrl Pts',(-0.200087321533276,0.00434016439324928,
-0.00968195214074013));
#33596=CARTESIAN_POINT('Ctrl Pts',(-0.2000886527572,0.00431653403973075,
-0.00967353518734554));
#33597=CARTESIAN_POINT('Ctrl Pts',(-0.200090052016831,0.00429293545299616,
-0.00966502305895532));
#33598=CARTESIAN_POINT('Ctrl Pts',(-0.200091515596528,0.00426939032521055,
-0.00965642358470294));
#33599=CARTESIAN_POINT('Ctrl Pts',(-0.200102813632993,0.00408763478913916,
-0.009590040336886));
#33600=CARTESIAN_POINT('Ctrl Pts',(-0.200117944500455,0.00390914660919813,
-0.00951826971542129));
#33601=CARTESIAN_POINT('Ctrl Pts',(-0.200135198996426,0.00374331233281143,
-0.00944613006251162));
#33602=CARTESIAN_POINT('Ctrl Pts',(-0.200144943842591,0.00364965387329946,
-0.00940538764840724));
#33603=CARTESIAN_POINT('Ctrl Pts',(-0.200155362599063,0.00355996581759564,
-0.00936467522534425));
#33604=CARTESIAN_POINT('Ctrl Pts',(-0.200166923307577,0.00346601444258958,
-0.00932014774930243));
#33605=CARTESIAN_POINT('Ctrl Pts',(-0.200172703661834,0.00341903875508654,
-0.00929788401128153));
#33606=CARTESIAN_POINT('Ctrl Pts',(-0.200178769436932,0.0033709977718656,
-0.00927466910998229));
#33607=CARTESIAN_POINT('Ctrl Pts',(-0.200185729564161,0.00331800612595654,
-0.00924841316153132));
#33608=CARTESIAN_POINT('Ctrl Pts',(-0.200192689691389,0.00326501448004748,
-0.00922215721308034));
#33609=CARTESIAN_POINT('Ctrl Pts',(-0.20020054722797,0.00320714423423817,
-0.00919271239613813));
#33610=CARTESIAN_POINT('Ctrl Pts',(-0.200206498554751,0.0031640587926023,
-0.00917037262902342));
#33611=CARTESIAN_POINT('Ctrl Pts',(-0.200212449881531,0.00312097335096644,
-0.00914803286190872));
#33612=CARTESIAN_POINT('Ctrl Pts',(-0.200216490557461,0.00309255879840688,
-0.00913301582033758));
#33613=CARTESIAN_POINT('Ctrl Pts',(-0.200221766654028,0.00305575582272453,
-0.00911332320001298));
#33614=CARTESIAN_POINT('Ctrl Pts',(-0.200227042750594,0.00301895284704218,
-0.00909363057968837));
#33615=CARTESIAN_POINT('Ctrl Pts',(-0.200233556728865,0.00297382752400723,
-0.00906914078631249));
#33616=CARTESIAN_POINT('Ctrl Pts',(-0.200240520992314,0.0029262323204959,
-0.00904270432387586));
#33617=CARTESIAN_POINT('Ctrl Pts',(-0.200254449480275,0.00283104217957486,
-0.00898983154680711));
#33618=CARTESIAN_POINT('Ctrl Pts',(-0.200270175007452,0.00272585285310391,
-0.00892937760645072));
#33619=CARTESIAN_POINT('Ctrl Pts',(-0.20028848823233,0.00260606466462287,
-0.00885651981476795));
#33620=CARTESIAN_POINT('',(-0.198286049999512,0.00260395535089921,-0.00881591880117876));
#33621=CARTESIAN_POINT('',(-0.197087022945346,0.00260284474309971,-0.00879175610761492));
#33622=CARTESIAN_POINT('',(-0.198286048907163,0.00260395688255514,-0.00881591368481554));
#33623=CARTESIAN_POINT('',(-0.196999277771019,0.00750268308291533,-0.0101599897056429));
#33624=CARTESIAN_POINT('Ctrl Pts',(-0.19708702016317,0.00260284594471271,
-0.00879175341490894));
#33625=CARTESIAN_POINT('Ctrl Pts',(-0.197068834773877,0.00272208793814125,
-0.00886375452525914));
#33626=CARTESIAN_POINT('Ctrl Pts',(-0.197045347018576,0.00287958672224235,
-0.00895381700776416));
#33627=CARTESIAN_POINT('Ctrl Pts',(-0.197019337786194,0.0030606704278004,
-0.00905132901012702));
#33628=CARTESIAN_POINT('Ctrl Pts',(-0.197007030683302,0.00314771264160573,
-0.00909709763797359));
#33629=CARTESIAN_POINT('Ctrl Pts',(-0.196983739637954,0.00332057904228507,
-0.00918452681865033));
#33630=CARTESIAN_POINT('Ctrl Pts',(-0.196959681604442,0.00351309773812326,
-0.00927673815620894));
#33631=CARTESIAN_POINT('Ctrl Pts',(-0.196923484098549,0.00382889007914085,
-0.0094194146781178));
#33632=CARTESIAN_POINT('Ctrl Pts',(-0.196882627187949,0.00433458182040128,
-0.00961962280043831));
#33633=CARTESIAN_POINT('Ctrl Pts',(-0.196864021895861,0.00496479377443585,
-0.00981699691993611));
#33634=CARTESIAN_POINT('Ctrl Pts',(-0.196869394342641,0.00544543475974735,
-0.00993489940569601));
#33635=CARTESIAN_POINT('Ctrl Pts',(-0.196883099379931,0.00582913403511029,
-0.0100090605613923));
#33636=CARTESIAN_POINT('Ctrl Pts',(-0.196893270946229,0.00604484605787118,
-0.0100450608561695));
#33637=CARTESIAN_POINT('Ctrl Pts',(-0.196903863329604,0.00623549696952723,
-0.0100728439930441));
#33638=CARTESIAN_POINT('Ctrl Pts',(-0.196909981015821,0.00633340968562837,
-0.0100855011664594));
#33639=CARTESIAN_POINT('Ctrl Pts',(-0.196921948697463,0.0065157190270304,
-0.0101074090344271));
#33640=CARTESIAN_POINT('Ctrl Pts',(-0.196946621808918,0.00685819946467974,
-0.0101407227075091));
#33641=CARTESIAN_POINT('Ctrl Pts',(-0.196976119313645,0.00722732122593311,
-0.0101595453695121));
#33642=CARTESIAN_POINT('Ctrl Pts',(-0.196999277771019,0.00750268308291533,
-0.0101599897056429));
#33643=CARTESIAN_POINT('',(-0.19708967999411,0.0124019686593504,-0.00878888197156201));
#33644=CARTESIAN_POINT('Ctrl Pts',(-0.196999277761509,0.00750268319688206,
-0.0101599897053952));
#33645=CARTESIAN_POINT('Ctrl Pts',(-0.19697629483056,0.00777809536223536,
-0.010159391190194));
#33646=CARTESIAN_POINT('Ctrl Pts',(-0.196947035992263,0.00814725538564192,
-0.0101403577789055));
#33647=CARTESIAN_POINT('Ctrl Pts',(-0.196922590041325,0.00848974553611497,
-0.0101068472176815));
#33648=CARTESIAN_POINT('Ctrl Pts',(-0.196910746879266,0.00867202861783065,
-0.0100848385512457));
#33649=CARTESIAN_POINT('Ctrl Pts',(-0.196904694182073,0.00876996963382525,
-0.0100721206783229));
#33650=CARTESIAN_POINT('Ctrl Pts',(-0.196894243760702,0.00896043688002101,
-0.0100442557114248));
#33651=CARTESIAN_POINT('Ctrl Pts',(-0.196884229454297,0.00917604072854748,
-0.0100081532861656));
#33652=CARTESIAN_POINT('Ctrl Pts',(-0.196870802252705,0.00955960072650904,
-0.00993381012963068));
#33653=CARTESIAN_POINT('Ctrl Pts',(-0.196865786671437,0.0100406836425149,
-0.00981551941099423));
#33654=CARTESIAN_POINT('Ctrl Pts',(-0.196884786269139,0.0106707171059872,
-0.00961778134897869));
#33655=CARTESIAN_POINT('Ctrl Pts',(-0.196925832894908,0.0111762928595007,
-0.00941727326247245));
#33656=CARTESIAN_POINT('Ctrl Pts',(-0.196962111865516,0.0114919544302138,
-0.00927443101340539));
#33657=CARTESIAN_POINT('Ctrl Pts',(-0.196986222319099,0.0116844289439496,
-0.00918210195977756));
#33658=CARTESIAN_POINT('Ctrl Pts',(-0.197009561269637,0.0118572808422539,
-0.00909455157396046));
#33659=CARTESIAN_POINT('Ctrl Pts',(-0.197021886668872,0.0119442782511614,
-0.00904874043222638));
#33660=CARTESIAN_POINT('Ctrl Pts',(-0.197047939559998,0.0121253088794259,
-0.0089511188934817));
#33661=CARTESIAN_POINT('Ctrl Pts',(-0.197071465199352,0.0122827607284905,
-0.00886095937504394));
#33662=CARTESIAN_POINT('Ctrl Pts',(-0.19708967999411,0.0124019686593504,
-0.00878888197156201));
#33663=CARTESIAN_POINT('',(-0.198291539773098,0.0124007197494604,-0.00881318649061618));
#33664=CARTESIAN_POINT('',(-0.197089680117917,0.0124019648222841,-0.00878887565627935));
#33665=CARTESIAN_POINT('',(-0.198199421594319,0.00750212679056316,-0.0101871141141493));
#33666=CARTESIAN_POINT('Ctrl Pts',(-0.19829153792328,0.0124007184247131,
-0.00881318383781034));
#33667=CARTESIAN_POINT('Ctrl Pts',(-0.198273154963815,0.0122808214712712,
-0.00888587603724278));
#33668=CARTESIAN_POINT('Ctrl Pts',(-0.198257366571701,0.0121755265252124,
-0.008946205391425));
#33669=CARTESIAN_POINT('Ctrl Pts',(-0.19824338083647,0.0120802313201533,
-0.00899897686821169));
#33670=CARTESIAN_POINT('Ctrl Pts',(-0.198236387938163,0.0120325835084961,
-0.00902536272241327));
#33671=CARTESIAN_POINT('Ctrl Pts',(-0.19822984672429,0.0119874059341052,
-0.0090498079275906));
#33672=CARTESIAN_POINT('Ctrl Pts',(-0.198224546066974,0.0119505437898245,
-0.00906947374403427));
#33673=CARTESIAN_POINT('Ctrl Pts',(-0.198219245409658,0.0119136816455438,
-0.00908913956047794));
#33674=CARTESIAN_POINT('Ctrl Pts',(-0.198215182862346,0.0118852005663994,
-0.0091041471282794));
#33675=CARTESIAN_POINT('Ctrl Pts',(-0.198209207227433,0.0118420675052475,
-0.00912644603588376));
#33676=CARTESIAN_POINT('Ctrl Pts',(-0.198203231592519,0.0117989344440956,
-0.00914874494348811));
#33677=CARTESIAN_POINT('Ctrl Pts',(-0.198195347282797,0.0117410363097808,
-0.00917811846332321));
#33678=CARTESIAN_POINT('Ctrl Pts',(-0.198188363332505,0.0116880111449667,
-0.00920431629631211));
#33679=CARTESIAN_POINT('Ctrl Pts',(-0.198181379382213,0.0116349859801525,
-0.00923051412930102));
#33680=CARTESIAN_POINT('Ctrl Pts',(-0.198175292753102,0.0115869053439776,
-0.00925368344306097));
#33681=CARTESIAN_POINT('Ctrl Pts',(-0.198169491817117,0.0115398731891329,
-0.00927591228520045));
#33682=CARTESIAN_POINT('Ctrl Pts',(-0.198157889945145,0.0114458088794436,
-0.0093203699694794));
#33683=CARTESIAN_POINT('Ctrl Pts',(-0.19814743116075,0.0113559392858479,
-0.00936105307203295));
#33684=CARTESIAN_POINT('Ctrl Pts',(-0.198137665924961,0.0112622449179336,
-0.00940170329857409));
#33685=CARTESIAN_POINT('Ctrl Pts',(-0.198119918429903,0.0110919632813885,
-0.00947558166773796));
#33686=CARTESIAN_POINT('Ctrl Pts',(-0.198104472435404,0.0109088411223429,
-0.00954888130057903));
#33687=CARTESIAN_POINT('Ctrl Pts',(-0.198093103285736,0.0107220794811649,
-0.00961660935126367));
#33688=CARTESIAN_POINT('Ctrl Pts',(-0.198091961100495,0.0107033167419592,
-0.00962341355229707));
#33689=CARTESIAN_POINT('Ctrl Pts',(-0.19809086006255,0.0106845181021202,
-0.00963016337228091));
#33690=CARTESIAN_POINT('Ctrl Pts',(-0.198089801972049,0.0106656934819478,
-0.00963685515692382));
#33691=CARTESIAN_POINT('Ctrl Pts',(-0.198078211798985,0.0104594912662437,
-0.00971015601546697));
#33692=CARTESIAN_POINT('Ctrl Pts',(-0.198071773321818,0.0102500417112847,
-0.00977626718318716));
#33693=CARTESIAN_POINT('Ctrl Pts',(-0.198069561648013,0.0100490540489262,
-0.00983262714102995));
#33694=CARTESIAN_POINT('Ctrl Pts',(-0.198067349974208,0.00984806638656765,
-0.00988898709887274));
#33695=CARTESIAN_POINT('Ctrl Pts',(-0.198069347056296,0.00965578772279335,
-0.00993642202513691));
#33696=CARTESIAN_POINT('Ctrl Pts',(-0.198075160204693,0.00944555197793135,
-0.00998088478378631));
#33697=CARTESIAN_POINT('Ctrl Pts',(-0.198078066778892,0.00934043410550035,
-0.010003116163111));
#33698=CARTESIAN_POINT('Ctrl Pts',(-0.198081932177224,0.00923078260354119,
-0.0100243883948405));
#33699=CARTESIAN_POINT('Ctrl Pts',(-0.19808658619968,0.00912232210711473,
-0.0100434533383869));
#33700=CARTESIAN_POINT('Ctrl Pts',(-0.198088913210908,0.00906809185890151,
-0.0100529858101601));
#33701=CARTESIAN_POINT('Ctrl Pts',(-0.198091436320725,0.0090141678228968,
-0.0100620138170739));
#33702=CARTESIAN_POINT('Ctrl Pts',(-0.198094455876335,0.00895538944683462,
-0.0100712781216205));
#33703=CARTESIAN_POINT('Ctrl Pts',(-0.198097475431945,0.00889661107077245,
-0.0100805424261671));
#33704=CARTESIAN_POINT('Ctrl Pts',(-0.198100994909325,0.00883295335593808,
-0.0100898876623028));
#33705=CARTESIAN_POINT('Ctrl Pts',(-0.198103763339097,0.00878494462583791,
-0.0100965688979994));
#33706=CARTESIAN_POINT('Ctrl Pts',(-0.198106531768869,0.00873693589573774,
-0.0101032501336961));
#33707=CARTESIAN_POINT('Ctrl Pts',(-0.198108544282875,0.00870460546688416,
-0.0101074843223612));
#33708=CARTESIAN_POINT('Ctrl Pts',(-0.198111034743449,0.00866571681355967,
-0.0101123992216654));
#33709=CARTESIAN_POINT('Ctrl Pts',(-0.198113525204022,0.00862682816023517,
-0.0101173141209696));
#33710=CARTESIAN_POINT('Ctrl Pts',(-0.198116496223594,0.00858136740023335,
-0.0101227934913069));
#33711=CARTESIAN_POINT('Ctrl Pts',(-0.198119644971167,0.00853477128033713,
-0.0101280274800034));
#33712=CARTESIAN_POINT('Ctrl Pts',(-0.198125942466314,0.00844157904054469,
-0.0101384954573962));
#33713=CARTESIAN_POINT('Ctrl Pts',(-0.198132947640148,0.0083438589764961,
-0.0101481254404693));
#33714=CARTESIAN_POINT('Ctrl Pts',(-0.198140881896705,0.00823760956696105,
-0.0101566869216774));
#33715=CARTESIAN_POINT('Ctrl Pts',(-0.198156750409818,0.00802511074789094,
-0.0101738098840936));
#33716=CARTESIAN_POINT('Ctrl Pts',(-0.198176338188712,0.00777849317508189,
-0.0101865293230802));
#33717=CARTESIAN_POINT('Ctrl Pts',(-0.198199421628184,0.00750212729749527,
-0.0101871140925375));
#33718=CARTESIAN_POINT('Ctrl Pts',(-0.198199421585483,0.00750212679134634,
-0.0101871140916879));
#33719=CARTESIAN_POINT('Ctrl Pts',(-0.19817611086679,0.00722581833102842,
-0.0101866502867765));
#33720=CARTESIAN_POINT('Ctrl Pts',(-0.198156325937573,0.00697926626484938,
-0.0101740436271574));
#33721=CARTESIAN_POINT('Ctrl Pts',(-0.198140292280466,0.00676682765207862,
-0.0101570226512735));
#33722=CARTESIAN_POINT('Ctrl Pts',(-0.198132275447017,0.00666060828083482,
-0.010148512158135));
#33723=CARTESIAN_POINT('Ctrl Pts',(-0.198125195705892,0.0065629169676353,
-0.0101389301595227));
#33724=CARTESIAN_POINT('Ctrl Pts',(-0.19811882975459,0.00646976830575511,
-0.0101285110517695));
#33725=CARTESIAN_POINT('Ctrl Pts',(-0.198115646778939,0.00642319397481502,
-0.0101233014978929));
#33726=CARTESIAN_POINT('Ctrl Pts',(-0.198112643055707,0.00637775867941244,
-0.0101178469343614));
#33727=CARTESIAN_POINT('Ctrl Pts',(-0.198110124028647,0.00633887748420828,
-0.0101129516600973));
#33728=CARTESIAN_POINT('Ctrl Pts',(-0.198107605001588,0.00629999628900412,
-0.0101080563858333));
#33729=CARTESIAN_POINT('Ctrl Pts',(-0.198105568069999,0.00626765542999263,
-0.0101038361134122));
#33730=CARTESIAN_POINT('Ctrl Pts',(-0.198102768660702,0.00621970700526403,
-0.0100971867469011));
#33731=CARTESIAN_POINT('Ctrl Pts',(-0.198099969251406,0.00617175858053543,
-0.0100905373803899));
#33732=CARTESIAN_POINT('Ctrl Pts',(-0.198096412203787,0.00610823162866769,
-0.0100812432595164));
#33733=CARTESIAN_POINT('Ctrl Pts',(-0.198093357310053,0.00604954828080428,
-0.0100720247747581));
#33734=CARTESIAN_POINT('Ctrl Pts',(-0.198090302416319,0.00599086493294086,
-0.0100628062899997));
#33735=CARTESIAN_POINT('Ctrl Pts',(-0.198087746225221,0.00593700044571326,
-0.0100538176925686));
#33736=CARTESIAN_POINT('Ctrl Pts',(-0.198085385863729,0.00588282738046454,
-0.0100443253007111));
#33737=CARTESIAN_POINT('Ctrl Pts',(-0.198080665140746,0.0057744812499671,
-0.0100253405169961));
#33738=CARTESIAN_POINT('Ctrl Pts',(-0.198076731913763,0.00566493425632279,
-0.0100041534600163));
#33739=CARTESIAN_POINT('Ctrl Pts',(-0.198073762684054,0.0055598002853358,
-0.0099819807918791));
#33740=CARTESIAN_POINT('Ctrl Pts',(-0.198067824224635,0.00534953234336182,
-0.00993763545560475));
#33741=CARTESIAN_POINT('Ctrl Pts',(-0.198065723172711,0.00515674447587092,
-0.0098901830470329));
#33742=CARTESIAN_POINT('Ctrl Pts',(-0.198067795176596,0.00495584284339765,
-0.00983396133677063));
#33743=CARTESIAN_POINT('Ctrl Pts',(-0.19806986718048,0.00475494121092437,
-0.00977773962650836));
#33744=CARTESIAN_POINT('Ctrl Pts',(-0.198076129141512,0.00454615886947251,
-0.00971197455341941));
#33745=CARTESIAN_POINT('Ctrl Pts',(-0.19808751697505,0.00433996447480952,
-0.00963882206161961));
#33746=CARTESIAN_POINT('Ctrl Pts',(-0.1980886606595,0.00431925629338696,
-0.0096314753290657));
#33747=CARTESIAN_POINT('Ctrl Pts',(-0.198089856071713,0.00429857301439935,
-0.00962405606956587));
#33748=CARTESIAN_POINT('Ctrl Pts',(-0.198091100757126,0.00427792906636229,
-0.00961656945493562));
#33749=CARTESIAN_POINT('Ctrl Pts',(-0.19810224958662,0.00409301820096132,
-0.0095495107514493));
#33750=CARTESIAN_POINT('Ctrl Pts',(-0.198117351628113,0.00391134860607491,
-0.00947685497202321));
#33751=CARTESIAN_POINT('Ctrl Pts',(-0.198134642942845,0.0037426810059623,
-0.00940378604143685));
#33752=CARTESIAN_POINT('Ctrl Pts',(-0.198144253824731,0.00364893195287393,
-0.00936317276984185));
#33753=CARTESIAN_POINT('Ctrl Pts',(-0.19815453763596,0.00355913397483952,
-0.00932258020023471));
#33754=CARTESIAN_POINT('Ctrl Pts',(-0.198165951518634,0.0034650713667194,
-0.00927818672101255));
#33755=CARTESIAN_POINT('Ctrl Pts',(-0.19817165845997,0.00341804006265935,
-0.00925598998140148));
#33756=CARTESIAN_POINT('Ctrl Pts',(-0.198177647851039,0.00336994309909578,
-0.00923284565855996));
#33757=CARTESIAN_POINT('Ctrl Pts',(-0.198184521108951,0.00331689198911531,
-0.00920667124833827));
#33758=CARTESIAN_POINT('Ctrl Pts',(-0.198191394366863,0.00326384087913483,
-0.00918049683811658));
#33759=CARTESIAN_POINT('Ctrl Pts',(-0.19819915453481,0.00320590715697485,
-0.00915114497768505));
#33760=CARTESIAN_POINT('Ctrl Pts',(-0.198205034234217,0.00316276107666219,
-0.00912886912670075));
#33761=CARTESIAN_POINT('Ctrl Pts',(-0.198210913933625,0.00311961499634954,
-0.00910659327571644));
#33762=CARTESIAN_POINT('Ctrl Pts',(-0.198214908743702,0.00309114345848673,
-0.00909161049026879));
#33763=CARTESIAN_POINT('Ctrl Pts',(-0.198220123131444,0.00305428016161934,
-0.00907197000303025));
#33764=CARTESIAN_POINT('Ctrl Pts',(-0.198225337519186,0.00301741686475196,
-0.00905232951579172));
#33765=CARTESIAN_POINT('Ctrl Pts',(-0.198231773934725,0.00297222742744097,
-0.00902791004712459));
#33766=CARTESIAN_POINT('Ctrl Pts',(-0.198238655187191,0.00292456530403474,
-0.00900155052998051));
#33767=CARTESIAN_POINT('Ctrl Pts',(-0.198252417653548,0.00282924132440047,
-0.00894883164345515));
#33768=CARTESIAN_POINT('Ctrl Pts',(-0.198267955385782,0.00272390777960448,
-0.00888855753184361));
#33769=CARTESIAN_POINT('Ctrl Pts',(-0.19828604862211,0.00260395376029585,
-0.00881592108484782));
#33770=CARTESIAN_POINT('',(-0.196289740186323,0.00260194423827529,-0.00877559941110405));
#33771=CARTESIAN_POINT('',(-0.195088737224831,0.00260009358768204,-0.00875100653258347));
#33772=CARTESIAN_POINT('',(-0.196289739083861,0.00260194595557777,-0.00877559392180319));
#33773=CARTESIAN_POINT('',(-0.195000274942555,0.00750353096665004,-0.0101148103080916));
#33774=CARTESIAN_POINT('Ctrl Pts',(-0.195088731428378,0.00260009275075466,
-0.00875100644688389));
#33775=CARTESIAN_POINT('Ctrl Pts',(-0.19507056550841,0.00271953784598169,
-0.00882281095420666));
#33776=CARTESIAN_POINT('Ctrl Pts',(-0.195047104552263,0.00287727544354604,
-0.00891261530507464));
#33777=CARTESIAN_POINT('Ctrl Pts',(-0.19502112831294,0.0030585954650411,
-0.00900983362472126));
#33778=CARTESIAN_POINT('Ctrl Pts',(-0.195008840275359,0.00314572278523736,
-0.00905545099263045));
#33779=CARTESIAN_POINT('Ctrl Pts',(-0.194985579883127,0.0033188059569336,
-0.00914261832470328));
#33780=CARTESIAN_POINT('Ctrl Pts',(-0.194961558956498,0.00351153316062807,
-0.00923454340707606));
#33781=CARTESIAN_POINT('Ctrl Pts',(-0.194925419797059,0.00382775789515487,
-0.00937681516219749));
#33782=CARTESIAN_POINT('Ctrl Pts',(-0.194884704941291,0.0043332136886723,
-0.00957614800626863));
#33783=CARTESIAN_POINT('Ctrl Pts',(-0.194866033057843,0.00496456833265218,
-0.00977314711040076));
#33784=CARTESIAN_POINT('Ctrl Pts',(-0.194871276563153,0.00544563633208474,
-0.00989065977731558));
#33785=CARTESIAN_POINT('Ctrl Pts',(-0.194884841613502,0.00582946020051222,
-0.00996453896154419));
#33786=CARTESIAN_POINT('Ctrl Pts',(-0.194894925268009,0.00604519454255553,
-0.0100003920022963));
#33787=CARTESIAN_POINT('Ctrl Pts',(-0.194905432082424,0.00623580302069773,
-0.0100280526202424));
#33788=CARTESIAN_POINT('Ctrl Pts',(-0.194911508299211,0.00633376414709155,
-0.0100406629644592));
#33789=CARTESIAN_POINT('Ctrl Pts',(-0.194923395497329,0.00651612336821955,
-0.0100624828569292));
#33790=CARTESIAN_POINT('Ctrl Pts',(-0.194947915530162,0.0068587387170376,
-0.0100956620679014));
#33791=CARTESIAN_POINT('Ctrl Pts',(-0.194977244056656,0.00722802825436263,
-0.0101143934759757));
#33792=CARTESIAN_POINT('Ctrl Pts',(-0.195000274942555,0.00750353096665004,
-0.0101148103080916));
#33793=CARTESIAN_POINT('',(-0.195088829404437,0.0124036829985792,-0.00874872615458748));
#33794=CARTESIAN_POINT('Ctrl Pts',(-0.195000274941086,0.00750353098422301,
-0.0101148103080518));
#33795=CARTESIAN_POINT('Ctrl Pts',(-0.19497724729087,0.00777891435449093,
-0.0101141862235937));
#33796=CARTESIAN_POINT('Ctrl Pts',(-0.194947927290943,0.00814801528533906,
-0.0100951955251351));
#33797=CARTESIAN_POINT('Ctrl Pts',(-0.19492342235388,0.00849042376455305,
-0.0100617947839754));
#33798=CARTESIAN_POINT('Ctrl Pts',(-0.194911546715732,0.0086726534583307,
-0.0100398642542001));
#33799=CARTESIAN_POINT('Ctrl Pts',(-0.194905476612654,0.00877055768838091,
-0.010027193464408));
#33800=CARTESIAN_POINT('Ctrl Pts',(-0.194894989814472,0.00896096337319932,
-0.00999943328655211));
#33801=CARTESIAN_POINT('Ctrl Pts',(-0.194884930759344,0.00917651379624448,
-0.00996346768226511));
#33802=CARTESIAN_POINT('Ctrl Pts',(-0.194871414892465,0.00956001074350432,
-0.00988940804155719));
#33803=CARTESIAN_POINT('Ctrl Pts',(-0.194866267314259,0.0100411730412217,
-0.00977154454516943));
#33804=CARTESIAN_POINT('Ctrl Pts',(-0.194885029757862,0.010671297796436,
-0.00957454608000461));
#33805=CARTESIAN_POINT('Ctrl Pts',(-0.194925805250576,0.0111770444460619,
-0.00937480202317456));
#33806=CARTESIAN_POINT('Ctrl Pts',(-0.19496188907685,0.0114928984561674,
-0.00923248932403923));
#33807=CARTESIAN_POINT('Ctrl Pts',(-0.19498587479727,0.0116854970829846,
-0.00914050560741373));
#33808=CARTESIAN_POINT('Ctrl Pts',(-0.195009096984921,0.0118584739142889,
-0.00905328224883865));
#33809=CARTESIAN_POINT('Ctrl Pts',(-0.195021362145538,0.0119455411324728,
-0.00900764103933122));
#33810=CARTESIAN_POINT('Ctrl Pts',(-0.195047288504676,0.0121267277435333,
-0.00891037903369575));
#33811=CARTESIAN_POINT('Ctrl Pts',(-0.195070701448721,0.0122843379937074,
-0.0088205465890419));
#33812=CARTESIAN_POINT('Ctrl Pts',(-0.195088829404437,0.0124036829985792,
-0.00874872615458748));
#33813=CARTESIAN_POINT('',(-0.196290666237131,0.012402736317308,-0.00877278749374763));
#33814=CARTESIAN_POINT('',(-0.195088829525986,0.0124036792402707,-0.0087487199395675));
#33815=CARTESIAN_POINT('',(-0.196200542036419,0.00750313725781679,-0.0101419374936355));
#33816=CARTESIAN_POINT('Ctrl Pts',(-0.196290664392037,0.0124027350217015,
-0.00877278488125371));
#33817=CARTESIAN_POINT('Ctrl Pts',(-0.19627237848276,0.0122827028385748,
-0.00884522665494427));
#33818=CARTESIAN_POINT('Ctrl Pts',(-0.196256673581162,0.0121773026599296,
-0.00890534564544836));
#33819=CARTESIAN_POINT('Ctrl Pts',(-0.196242762233673,0.0120819185796832,
-0.00895793228268215));
#33820=CARTESIAN_POINT('Ctrl Pts',(-0.196235806530618,0.0120342263385952,
-0.00898422571209386));
#33821=CARTESIAN_POINT('Ctrl Pts',(-0.196229300231151,0.0119890086386769,
-0.0090085850142568));
#33822=CARTESIAN_POINT('Ctrl Pts',(-0.196224027764951,0.0119521137132335,
-0.00902818212269904));
#33823=CARTESIAN_POINT('Ctrl Pts',(-0.19621875529875,0.0119152187877902,
-0.00904777923114128));
#33824=CARTESIAN_POINT('Ctrl Pts',(-0.196214714231417,0.0118867117807409,
-0.00906273491264468));
#33825=CARTESIAN_POINT('Ctrl Pts',(-0.196208771113589,0.0118435442940514,
-0.00908495482459714));
#33826=CARTESIAN_POINT('Ctrl Pts',(-0.19620282799576,0.0118003768073619,
-0.00910717473654961));
#33827=CARTESIAN_POINT('Ctrl Pts',(-0.196194987218421,0.0117424366024625,
-0.00913644284299786));
#33828=CARTESIAN_POINT('Ctrl Pts',(-0.196188042371249,0.0116893745499815,
-0.00916254679872934));
#33829=CARTESIAN_POINT('Ctrl Pts',(-0.196181097524077,0.0116363124975004,
-0.00918865075446083));
#33830=CARTESIAN_POINT('Ctrl Pts',(-0.196175045583579,0.0115881996144841,
-0.00921173723675161));
#33831=CARTESIAN_POINT('Ctrl Pts',(-0.196169278080669,0.0115411361970223,
-0.00923388702235407));
#33832=CARTESIAN_POINT('Ctrl Pts',(-0.196157743074849,0.0114470093620985,
-0.009278186593559));
#33833=CARTESIAN_POINT('Ctrl Pts',(-0.196147346135914,0.0113570811040665,
-0.00931872661950712));
#33834=CARTESIAN_POINT('Ctrl Pts',(-0.196137642854787,0.0112633381126882,
-0.00935923068811809));
#33835=CARTESIAN_POINT('Ctrl Pts',(-0.196119711067213,0.0110900998661695,
-0.00943408272473305));
#33836=CARTESIAN_POINT('Ctrl Pts',(-0.196104159211111,0.010903618744401,
-0.00950832225153081));
#33837=CARTESIAN_POINT('Ctrl Pts',(-0.196092840715868,0.0107135413899731,
-0.00957675825515148));
#33838=CARTESIAN_POINT('Ctrl Pts',(-0.196091909842126,0.0106979087449592,
-0.00958238667813743));
#33839=CARTESIAN_POINT('Ctrl Pts',(-0.196091007602874,0.0106822523640472,
-0.00958797717070507));
#33840=CARTESIAN_POINT('Ctrl Pts',(-0.19609013502917,0.0106665779486784,
-0.00959352765109829));
#33841=CARTESIAN_POINT('Ctrl Pts',(-0.19607865283047,0.0104603182930727,
-0.00966656643100897));
#33842=CARTESIAN_POINT('Ctrl Pts',(-0.196072306157994,0.0102508063682596,
-0.00973244927437508));
#33843=CARTESIAN_POINT('Ctrl Pts',(-0.196070171014414,0.0100497920320044,
-0.00978860958523751));
#33844=CARTESIAN_POINT('Ctrl Pts',(-0.196068035870834,0.00984877769574926,
-0.00984476989609994));
#33845=CARTESIAN_POINT('Ctrl Pts',(-0.196070094248627,0.00965650659372004,
-0.00989203246707846));
#33846=CARTESIAN_POINT('Ctrl Pts',(-0.196075963871027,0.00944628266376169,
-0.00993633782451496));
#33847=CARTESIAN_POINT('Ctrl Pts',(-0.196078898682228,0.00934117069878252,
-0.00995849050323321));
#33848=CARTESIAN_POINT('Ctrl Pts',(-0.196082791096299,0.00923152646979285,
-0.0099796884291423));
#33849=CARTESIAN_POINT('Ctrl Pts',(-0.196087469396512,0.00912307680290144,
-0.00999868741761622));
#33850=CARTESIAN_POINT('Ctrl Pts',(-0.196089808546619,0.00906885196945574,
-0.0100081869118532));
#33851=CARTESIAN_POINT('Ctrl Pts',(-0.196092343114862,0.00901493417674492,
-0.0100171838575576));
#33852=CARTESIAN_POINT('Ctrl Pts',(-0.196095374433549,0.00895616243316652,
-0.0100264167229923));
#33853=CARTESIAN_POINT('Ctrl Pts',(-0.196098405752237,0.00889739068958812,
-0.010035649588427));
#33854=CARTESIAN_POINT('Ctrl Pts',(-0.196101937283514,0.00883374017538179,
-0.0100449635987899));
#33855=CARTESIAN_POINT('Ctrl Pts',(-0.196104714320117,0.00878573972656593,
-0.0100516224160801));
#33856=CARTESIAN_POINT('Ctrl Pts',(-0.196107491356719,0.00873773927775008,
-0.0100582812333704));
#33857=CARTESIAN_POINT('Ctrl Pts',(-0.19610950904998,0.00870541800268859,
-0.0100625009696805));
#33858=CARTESIAN_POINT('Ctrl Pts',(-0.196112005669307,0.00866653822219212,
-0.0100673995537587));
#33859=CARTESIAN_POINT('Ctrl Pts',(-0.196114502288634,0.00862765844169564,
-0.010072298137837));
#33860=CARTESIAN_POINT('Ctrl Pts',(-0.196117480435931,0.00858220637125886,
-0.0100777597870329));
#33861=CARTESIAN_POINT('Ctrl Pts',(-0.196120636207888,0.00853561902876165,
-0.0100829772314099));
#33862=CARTESIAN_POINT('Ctrl Pts',(-0.196126947751801,0.00844244434376721,
-0.0100934121201638));
#33863=CARTESIAN_POINT('Ctrl Pts',(-0.196133966574071,0.00834474209293421,
-0.0101030131519277));
#33864=CARTESIAN_POINT('Ctrl Pts',(-0.196141914853224,0.00823851085581078,
-0.0101115512170876));
#33865=CARTESIAN_POINT('Ctrl Pts',(-0.196157811408511,0.00802604842191928,
-0.0101286273441639));
#33866=CARTESIAN_POINT('Ctrl Pts',(-0.196177428716306,0.00777946867134234,
-0.0101413224703218));
#33867=CARTESIAN_POINT('Ctrl Pts',(-0.196200542403418,0.00750313728849443,
-0.0101419374846836));
#33868=CARTESIAN_POINT('Ctrl Pts',(-0.196200542416589,0.00750313713103434,
-0.0101419374850341));
#33869=CARTESIAN_POINT('Ctrl Pts',(-0.196177284241936,0.00722677170552974,
-0.010141504463779));
#33870=CARTESIAN_POINT('Ctrl Pts',(-0.196157539522526,0.00698015070048215,
-0.0101289673247935));
#33871=CARTESIAN_POINT('Ctrl Pts',(-0.196141534742996,0.00676764915535907,
-0.0101120253286253));
#33872=CARTESIAN_POINT('Ctrl Pts',(-0.196133532353232,0.00666139838279753,
-0.0101035543305412));
#33873=CARTESIAN_POINT('Ctrl Pts',(-0.196126464215432,0.00656367714880856,
-0.0100940144642487));
#33874=CARTESIAN_POINT('Ctrl Pts',(-0.196120106043974,0.00647047985556275,
-0.0100836370516775));
#33875=CARTESIAN_POINT('Ctrl Pts',(-0.196116926958245,0.00642388120893984,
-0.0100784483453919));
#33876=CARTESIAN_POINT('Ctrl Pts',(-0.19611392617026,0.00637841690895378,
-0.0100730144654881));
#33877=CARTESIAN_POINT('Ctrl Pts',(-0.196111410478906,0.00633953041564724,
-0.010068140055752));
#33878=CARTESIAN_POINT('Ctrl Pts',(-0.196108894787553,0.0063006439223407,
-0.0100632656460158));
#33879=CARTESIAN_POINT('Ctrl Pts',(-0.196106861587228,0.00626832150873382,
-0.0100590666463675));
#33880=CARTESIAN_POINT('Ctrl Pts',(-0.196104060770134,0.00622029929122412,
-0.0100524357044143));
#33881=CARTESIAN_POINT('Ctrl Pts',(-0.19610125995304,0.00617227707371441,
-0.0100458047624611));
#33882=CARTESIAN_POINT('Ctrl Pts',(-0.196097696376481,0.00610858406790501,
-0.0100365253965468));
#33883=CARTESIAN_POINT('Ctrl Pts',(-0.196094636239161,0.00604977851394286,
-0.0100273247247253));
#33884=CARTESIAN_POINT('Ctrl Pts',(-0.19609157610184,0.00599097295998071,
-0.0100181240529037));
#33885=CARTESIAN_POINT('Ctrl Pts',(-0.196089015934455,0.00593703009000086,
-0.0100091571569817));
#33886=CARTESIAN_POINT('Ctrl Pts',(-0.196086651610151,0.00588278080726641,
-0.00999968780876252));
#33887=CARTESIAN_POINT('Ctrl Pts',(-0.196081922961544,0.00577428224179751,
-0.00998074911232417));
#33888=CARTESIAN_POINT('Ctrl Pts',(-0.196077981909559,0.00566459157770989,
-0.00995961140281356));
#33889=CARTESIAN_POINT('Ctrl Pts',(-0.19607500205802,0.00555945248426065,
-0.00993751976640365));
#33890=CARTESIAN_POINT('Ctrl Pts',(-0.196069042354942,0.00534917429736217,
-0.00989333649358383));
#33891=CARTESIAN_POINT('Ctrl Pts',(-0.196066908198774,0.00515692595402839,
-0.00984620317386021));
#33892=CARTESIAN_POINT('Ctrl Pts',(-0.196068981777312,0.00495587356963853,
-0.00979016583001711));
#33893=CARTESIAN_POINT('Ctrl Pts',(-0.196071055355851,0.00475482118524867,
-0.00973412848617402));
#33894=CARTESIAN_POINT('Ctrl Pts',(-0.196077354771034,0.00454521109940807,
-0.00966835812863127));
#33895=CARTESIAN_POINT('Ctrl Pts',(-0.196088821024484,0.00433885181007513,
-0.00959542674868746));
#33896=CARTESIAN_POINT('Ctrl Pts',(-0.196089792739332,0.00432136376253628,
-0.00958924613310358));
#33897=CARTESIAN_POINT('Ctrl Pts',(-0.196090801571326,0.00430389812924055,
-0.00958301572777096));
#33898=CARTESIAN_POINT('Ctrl Pts',(-0.196091846079231,0.0042864628553818,
-0.00957673843898767));
#33899=CARTESIAN_POINT('Ctrl Pts',(-0.196103126784216,0.00409816157032374,
-0.00950894360225902));
#33900=CARTESIAN_POINT('Ctrl Pts',(-0.196118568741884,0.00391348555761878,
-0.00943549127838421));
#33901=CARTESIAN_POINT('Ctrl Pts',(-0.196136356400838,0.00374185548860918,
-0.00936145714508957));
#33902=CARTESIAN_POINT('Ctrl Pts',(-0.196146073731612,0.00364809463139091,
-0.00932101257823032));
#33903=CARTESIAN_POINT('Ctrl Pts',(-0.196156487876551,0.00355816449055205,
-0.00928053745040833));
#33904=CARTESIAN_POINT('Ctrl Pts',(-0.196168046508536,0.00346400760203785,
-0.00923629354441179));
#33905=CARTESIAN_POINT('Ctrl Pts',(-0.196173825824529,0.00341692915778075,
-0.00921417159141352));
#33906=CARTESIAN_POINT('Ctrl Pts',(-0.196179891183077,0.0033687942155918,
-0.00919111063395478));
#33907=CARTESIAN_POINT('Ctrl Pts',(-0.196186854858822,0.00331568620136784,
-0.00916502378152004));
#33908=CARTESIAN_POINT('Ctrl Pts',(-0.196193818534566,0.00326257818714388,
-0.00913893692908531));
#33909=CARTESIAN_POINT('Ctrl Pts',(-0.196201683566926,0.00320456836380365,
-0.00910967677303251));
#33910=CARTESIAN_POINT('Ctrl Pts',(-0.196207638740065,0.00316139558869042,
-0.00908748652539309));
#33911=CARTESIAN_POINT('Ctrl Pts',(-0.196213593913204,0.0031182228135772,
-0.00906529627775366));
#33912=CARTESIAN_POINT('Ctrl Pts',(-0.196217634816342,0.00308977453463767,
-0.00905039288359229));
#33913=CARTESIAN_POINT('Ctrl Pts',(-0.196222914850236,0.00305290139557111,
-0.00903083600740598));
#33914=CARTESIAN_POINT('Ctrl Pts',(-0.196228194884131,0.00301602825650455,
-0.00901127913121967));
#33915=CARTESIAN_POINT('Ctrl Pts',(-0.196234716492052,0.00297079552253433,
-0.00898694760628085));
#33916=CARTESIAN_POINT('Ctrl Pts',(-0.196241690253741,0.00292307688435604,
-0.00896067750775797));
#33917=CARTESIAN_POINT('Ctrl Pts',(-0.196255637737435,0.00282763987953676,
-0.00890813746019911));
#33918=CARTESIAN_POINT('Ctrl Pts',(-0.196271389759889,0.00272214090200285,
-0.00884804823129562));
#33919=CARTESIAN_POINT('Ctrl Pts',(-0.196289738784128,0.00260194254294682,
-0.00877560186874003));
#33920=CARTESIAN_POINT('',(-0.22252089691926,0.00173296344499172,-0.0086607489990303));
#33921=CARTESIAN_POINT('',(-0.22131752266871,0.001732003051347,-0.00863750155434712));
#33922=CARTESIAN_POINT('',(-0.221317522515984,0.00173199629815866,-0.00863750974697598));
#33923=CARTESIAN_POINT('',(-0.220881156857209,0.0044216146108216,-0.0101613899799023));
#33924=CARTESIAN_POINT('Ctrl Pts',(-0.22131752266871,0.001732003051347,
-0.00863750155434712));
#33925=CARTESIAN_POINT('Ctrl Pts',(-0.221280608098474,0.00186237282555748,
-0.00874426915938514));
#33926=CARTESIAN_POINT('Ctrl Pts',(-0.221233212581849,0.00203562110891459,
-0.00887756445341166));
#33927=CARTESIAN_POINT('Ctrl Pts',(-0.221181445914481,0.00223503566955665,
-0.00902112143140114));
#33928=CARTESIAN_POINT('Ctrl Pts',(-0.221157385236667,0.002329669593433,
-0.00908751775139101));
#33929=CARTESIAN_POINT('Ctrl Pts',(-0.221111886300313,0.00252077303573938,
-0.00921607714287932));
#33930=CARTESIAN_POINT('Ctrl Pts',(-0.221065558612416,0.0027351991985903,
-0.00935230474791183));
#33931=CARTESIAN_POINT('Ctrl Pts',(-0.221015381104576,0.00300050906695994,
-0.00951012073222565));
#33932=CARTESIAN_POINT('Ctrl Pts',(-0.220970549456544,0.00330668853965943,
-0.00967636498042947));
#33933=CARTESIAN_POINT('Ctrl Pts',(-0.220919173025872,0.00375989492422517,
-0.00990132539660816));
#33934=CARTESIAN_POINT('Ctrl Pts',(-0.220892662923779,0.00416326457627243,
-0.0100677775881752));
#33935=CARTESIAN_POINT('Ctrl Pts',(-0.220881156857209,0.0044216146108216,
-0.0101613899799023));
#33936=CARTESIAN_POINT('',(-0.220990770344514,0.00750289496288283,-0.0107022172106033));
#33937=CARTESIAN_POINT('Ctrl Pts',(-0.220881156857209,0.0044216146108216,
-0.0101613899799023));
#33938=CARTESIAN_POINT('Ctrl Pts',(-0.220869650790639,0.00467996464537077,
-0.0102550023716294));
#33939=CARTESIAN_POINT('Ctrl Pts',(-0.22085897332715,0.00517553858083778,
-0.0104075156831151));
#33940=CARTESIAN_POINT('Ctrl Pts',(-0.220872746753963,0.00582497912567758,
-0.0105490747109447));
#33941=CARTESIAN_POINT('Ctrl Pts',(-0.220894825643282,0.00623887119176755,
-0.0106129012161888));
#33942=CARTESIAN_POINT('Ctrl Pts',(-0.220911316471387,0.00650002679818652,
-0.010645792840235));
#33943=CARTESIAN_POINT('Ctrl Pts',(-0.220928204267902,0.00673675762205502,
-0.0106690295622062));
#33944=CARTESIAN_POINT('Ctrl Pts',(-0.220938207005333,0.00686646402018735,
-0.0106790684180989));
#33945=CARTESIAN_POINT('Ctrl Pts',(-0.220958367107639,0.00712002666152971,
-0.0106952223995177));
#33946=CARTESIAN_POINT('Ctrl Pts',(-0.220976662293923,0.00733816544666396,
-0.0107019515992283));
#33947=CARTESIAN_POINT('Ctrl Pts',(-0.220990770344514,0.00750289496288283,
-0.0107022172106033));
#33948=CARTESIAN_POINT('',(-0.220878076795315,0.0105847978297417,-0.0101590210697871));
#33949=CARTESIAN_POINT('Ctrl Pts',(-0.220990765990492,0.00750294549844078,
-0.0107022170957316));
#33950=CARTESIAN_POINT('Ctrl Pts',(-0.22097656165945,0.00766781034107023,
-0.0107018419086198));
#33951=CARTESIAN_POINT('Ctrl Pts',(-0.220958128570126,0.00788622176558849,
-0.010694956094636));
#33952=CARTESIAN_POINT('Ctrl Pts',(-0.220937788273734,0.00814023517284528,
-0.0106785867159598));
#33953=CARTESIAN_POINT('Ctrl Pts',(-0.220927673950829,0.00827039995690873,
-0.0106684092823677));
#33954=CARTESIAN_POINT('Ctrl Pts',(-0.2209106107512,0.0085074164570001,
-0.0106449487005366));
#33955=CARTESIAN_POINT('Ctrl Pts',(-0.220893897670049,0.00876904348654153,
-0.0106117657537804));
#33956=CARTESIAN_POINT('Ctrl Pts',(-0.220871431947319,0.00918327907519644,
-0.0105475333080408));
#33957=CARTESIAN_POINT('Ctrl Pts',(-0.220856863313028,0.00983530374811943,
-0.0104046120531604));
#33958=CARTESIAN_POINT('Ctrl Pts',(-0.220866936794483,0.0103285626661751,
-0.0102520979581623));
#33959=CARTESIAN_POINT('Ctrl Pts',(-0.220878076795315,0.0105847978297417,
-0.0101590210697871));
#33960=CARTESIAN_POINT('',(-0.221311657438852,0.0132815265142635,-0.00862621316345587));
#33961=CARTESIAN_POINT('Ctrl Pts',(-0.220878076795315,0.0105847978297417,
-0.0101590210697871));
#33962=CARTESIAN_POINT('Ctrl Pts',(-0.220878137729977,0.0105861994097892,
-0.0101585119487601));
#33963=CARTESIAN_POINT('Ctrl Pts',(-0.22088943342552,0.0108452945702086,
-0.0100643226589043));
#33964=CARTESIAN_POINT('Ctrl Pts',(-0.220915712841839,0.0112491091634393,
-0.00989717402810534));
#33965=CARTESIAN_POINT('Ctrl Pts',(-0.220966901565007,0.0117033824356887,
-0.00967107301525563));
#33966=CARTESIAN_POINT('Ctrl Pts',(-0.221011958082026,0.0120124705433347,
-0.00950263684076823));
#33967=CARTESIAN_POINT('Ctrl Pts',(-0.221061649944544,0.0122768352979043,
-0.00934477849302234));
#33968=CARTESIAN_POINT('Ctrl Pts',(-0.221107694057363,0.0124917040509188,
-0.009207793630019));
#33969=CARTESIAN_POINT('Ctrl Pts',(-0.221152929443628,0.0126833989489049,
-0.0090783511460067));
#33970=CARTESIAN_POINT('Ctrl Pts',(-0.221176784331268,0.0127781205930578,
-0.00901163571788361));
#33971=CARTESIAN_POINT('Ctrl Pts',(-0.221228121535475,0.0129777814119194,
-0.008867344763671));
#33972=CARTESIAN_POINT('Ctrl Pts',(-0.221275085769101,0.013151123064894,
-0.00873344581796572));
#33973=CARTESIAN_POINT('Ctrl Pts',(-0.221311657037594,0.0132815289113517,
-0.00862621670222814));
#33974=CARTESIAN_POINT('',(-0.222515321099814,0.0132803985666653,-0.00864958405725804));
#33975=CARTESIAN_POINT('',(-0.222515320943395,0.013280405523687,-0.00864959244197508));
#33976=CARTESIAN_POINT('',(-0.222078175707026,0.010589795154743,-0.010183304001148));
#33977=CARTESIAN_POINT('Ctrl Pts',(-0.222515321099814,0.0132803985666653,
-0.00864958405725804));
#33978=CARTESIAN_POINT('Ctrl Pts',(-0.22247838679018,0.0131487451657634,
-0.00875812340870462));
#33979=CARTESIAN_POINT('Ctrl Pts',(-0.222431140247769,0.012974593196174,
-0.00889287803634793));
#33980=CARTESIAN_POINT('Ctrl Pts',(-0.222379701242625,0.0127754092376983,
-0.00903706435333658));
#33981=CARTESIAN_POINT('Ctrl Pts',(-0.222356407099826,0.0126836110770626,
-0.0091018905341631));
#33982=CARTESIAN_POINT('Ctrl Pts',(-0.222310370393322,0.012490449153673,
-0.00923264820054545));
#33983=CARTESIAN_POINT('Ctrl Pts',(-0.222263835967482,0.0122757574562573,
-0.0093697752596197));
#33984=CARTESIAN_POINT('Ctrl Pts',(-0.222213597622187,0.0120127350671868,
-0.0095271791305912));
#33985=CARTESIAN_POINT('Ctrl Pts',(-0.222167895914748,0.0117045189932484,
-0.00969555561414337));
#33986=CARTESIAN_POINT('Ctrl Pts',(-0.222116057296822,0.0112509721833174,
-0.00992190901452015));
#33987=CARTESIAN_POINT('Ctrl Pts',(-0.222089558267121,0.0108477787632884,
-0.0100892171625672));
#33988=CARTESIAN_POINT('Ctrl Pts',(-0.222078175707026,0.010589795154743,
-0.010183304001148));
#33989=CARTESIAN_POINT('',(-0.222191222341661,0.00750354856662756,-0.010729348089511));
#33990=CARTESIAN_POINT('Ctrl Pts',(-0.222078175707026,0.010589795154743,
-0.010183304001148));
#33991=CARTESIAN_POINT('Ctrl Pts',(-0.22206679314693,0.0103318115461975,
-0.0102773908397288));
#33992=CARTESIAN_POINT('Ctrl Pts',(-0.222056594946149,0.00983746833872088,
-0.0104306606633226));
#33993=CARTESIAN_POINT('Ctrl Pts',(-0.2220713925672,0.0091839301427948,
-0.0105742538518266));
#33994=CARTESIAN_POINT('Ctrl Pts',(-0.222094064925071,0.00876980798679073,
-0.0106386169255547));
#33995=CARTESIAN_POINT('Ctrl Pts',(-0.222110874185597,0.00850825014440612,
-0.0106718828955474));
#33996=CARTESIAN_POINT('Ctrl Pts',(-0.222128052876237,0.00827084237768706,
-0.0106954393284925));
#33997=CARTESIAN_POINT('Ctrl Pts',(-0.222138118385459,0.00814180097829653,
-0.0107055572231305));
#33998=CARTESIAN_POINT('Ctrl Pts',(-0.222158491389853,0.00788794183207559,
-0.0107220001061996));
#33999=CARTESIAN_POINT('Ctrl Pts',(-0.222176969724701,0.00766907929165035,
-0.010728960325345));
#34000=CARTESIAN_POINT('Ctrl Pts',(-0.22219122384913,0.00750355041477949,
-0.0107293482161627));
#34001=CARTESIAN_POINT('',(-0.222081204604315,0.00442193154451798,-0.0101876159050024));
#34002=CARTESIAN_POINT('Ctrl Pts',(-0.22219122368108,0.00750354845177293,
-0.010729348213144));
#34003=CARTESIAN_POINT('Ctrl Pts',(-0.222177054476964,0.00733803644934816,
-0.0107290936725269));
#34004=CARTESIAN_POINT('Ctrl Pts',(-0.222158703787922,0.00711934029188453,
-0.0107223125470692));
#34005=CARTESIAN_POINT('Ctrl Pts',(-0.222138508319268,0.0068658863078884,
-0.0107061095911713));
#34006=CARTESIAN_POINT('Ctrl Pts',(-0.222128566128202,0.00673744809951971,
-0.0106961575846219));
#34007=CARTESIAN_POINT('Ctrl Pts',(-0.222111554921162,0.00650011441462726,
-0.0106728327203371));
#34008=CARTESIAN_POINT('Ctrl Pts',(-0.222094975466172,0.00623895487711817,
-0.0106398758531691));
#34009=CARTESIAN_POINT('Ctrl Pts',(-0.222072719549722,0.00582501305167259,
-0.0105759182598013));
#34010=CARTESIAN_POINT('Ctrl Pts',(-0.222058883145086,0.00517694615728237,
-0.0104344345821352));
#34011=CARTESIAN_POINT('Ctrl Pts',(-0.22206961077245,0.00468075083121768,
-0.0102815841682815));
#34012=CARTESIAN_POINT('Ctrl Pts',(-0.222081204604315,0.00442193154451798,
-0.0101876159050024));
#34013=CARTESIAN_POINT('Ctrl Pts',(-0.222081236730105,0.00442121470034128,
-0.0101873556089765));
#34014=CARTESIAN_POINT('Ctrl Pts',(-0.222092852784074,0.00416213643488008,
-0.0100932681026557));
#34015=CARTESIAN_POINT('Ctrl Pts',(-0.222119643967736,0.0037572121452274,
-0.00992571002071133));
#34016=CARTESIAN_POINT('Ctrl Pts',(-0.222171540892955,0.00330489363448679,
-0.0097005072347765));
#34017=CARTESIAN_POINT('Ctrl Pts',(-0.222216824087379,0.00300031071146108,
-0.00953470605702957));
#34018=CARTESIAN_POINT('Ctrl Pts',(-0.22226751910141,0.00273651678297638,
-0.00937745944238771));
#34019=CARTESIAN_POINT('Ctrl Pts',(-0.22231438217505,0.00252220880427444,
-0.00924106999805114));
#34020=CARTESIAN_POINT('Ctrl Pts',(-0.222360856121196,0.00232912295519028,
-0.0091108494752828));
#34021=CARTESIAN_POINT('Ctrl Pts',(-0.222384218798713,0.00223804757091996,
-0.00904677611111708));
#34022=CARTESIAN_POINT('Ctrl Pts',(-0.222436134874479,0.00203916205828335,
-0.00890338236979424));
#34023=CARTESIAN_POINT('Ctrl Pts',(-0.222483927643371,0.0018649090272055,
-0.00876910508506613));
#34024=CARTESIAN_POINT('Ctrl Pts',(-0.222521332224266,0.00173302259371186,
-0.00866080956817125));
#34025=CARTESIAN_POINT('',(-0.220521369425964,0.00173331988493514,-0.00862374985263368));
#34026=CARTESIAN_POINT('',(-0.219242026281106,0.00197737824222187,-0.00879310176875613));
#34027=CARTESIAN_POINT('Ctrl Pts',(-0.220521098969949,0.00173330778007932,
-0.00862373486994674));
#34028=CARTESIAN_POINT('Ctrl Pts',(-0.220437463496804,0.00173270302656685,
-0.00862167993463741));
#34029=CARTESIAN_POINT('Ctrl Pts',(-0.220369227103567,0.00173229065597507,
-0.00862007045367697));
#34030=CARTESIAN_POINT('Ctrl Pts',(-0.220311184555208,0.00173215324673003,
-0.00861887697602086));
#34031=CARTESIAN_POINT('Ctrl Pts',(-0.220282122230284,0.00173208444492447,
-0.00861827939310259));
#34032=CARTESIAN_POINT('Ctrl Pts',(-0.220255615581277,0.00173208457694698,
-0.00861778610679002));
#34033=CARTESIAN_POINT('Ctrl Pts',(-0.220236891963046,0.00173207055296993,
-0.00861742606792021));
#34034=CARTESIAN_POINT('Ctrl Pts',(-0.220218168344816,0.00173205652899288,
-0.00861706602905041));
#34035=CARTESIAN_POINT('Ctrl Pts',(-0.220207227757186,0.00173202834123672,
-0.00861683924709774));
#34036=CARTESIAN_POINT('Ctrl Pts',(-0.220183160781322,0.00173231835779415,
-0.00861662965552147));
#34037=CARTESIAN_POINT('Ctrl Pts',(-0.220159093805458,0.00173260837435157,
-0.00861642006394521));
#34038=CARTESIAN_POINT('Ctrl Pts',(-0.220121900441102,0.00173321658367137,
-0.00861622767665298));
#34039=CARTESIAN_POINT('Ctrl Pts',(-0.220089219607307,0.00173419131657759,
-0.00861641983989896));
#34040=CARTESIAN_POINT('Ctrl Pts',(-0.220056538773513,0.00173516604948381,
-0.00861661200314494));
#34041=CARTESIAN_POINT('Ctrl Pts',(-0.22002837047154,0.00173650736236591,
-0.00861718864907257));
#34042=CARTESIAN_POINT('Ctrl Pts',(-0.220001719326565,0.00173796383479279,
-0.00861788694802301));
#34043=CARTESIAN_POINT('Ctrl Pts',(-0.219948417036616,0.00174087677964655,
-0.00861928354592391));
#34044=CARTESIAN_POINT('Ctrl Pts',(-0.219901183321191,0.00174424799001159,
-0.00862116963247801));
#34045=CARTESIAN_POINT('Ctrl Pts',(-0.219846041444898,0.00175121840781084,
-0.00862583421971319));
#34046=CARTESIAN_POINT('Ctrl Pts',(-0.219790899568604,0.0017581888256101,
-0.00863049880694838));
#34047=CARTESIAN_POINT('Ctrl Pts',(-0.219727849628244,0.00176876278295717,
-0.0086379366743074));
#34048=CARTESIAN_POINT('Ctrl Pts',(-0.219672835763088,0.001780783273963,
-0.00864663676002183));
#34049=CARTESIAN_POINT('Ctrl Pts',(-0.219617821897932,0.00179280376496883,
-0.00865533684573626));
#34050=CARTESIAN_POINT('Ctrl Pts',(-0.219570843848114,0.00180625926555738,
-0.00866531313618264));
#34051=CARTESIAN_POINT('Ctrl Pts',(-0.2195205738428,0.00182568220387981,
-0.00867987985899917));
#34052=CARTESIAN_POINT('Ctrl Pts',(-0.219470303837487,0.00184510514220223,
-0.0086944465818157));
#34053=CARTESIAN_POINT('Ctrl Pts',(-0.219416742624575,0.00187052796332885,
-0.00871356370743997));
#34054=CARTESIAN_POINT('Ctrl Pts',(-0.219375354713411,0.00189334849853141,
-0.00873064671564717));
#34055=CARTESIAN_POINT('Ctrl Pts',(-0.219333967134904,0.00191616885031262,
-0.00874772958654872));
#34056=CARTESIAN_POINT('Ctrl Pts',(-0.219304750253871,0.00193628767794186,
-0.00876290562638991));
#34057=CARTESIAN_POINT('Ctrl Pts',(-0.219242026281106,0.00197737824222187,
-0.00879310176875613));
#34058=CARTESIAN_POINT('',(-0.218875283101098,0.004581383707407,-0.0101734940573489));
#34059=CARTESIAN_POINT('Ctrl Pts',(-0.219242024743306,0.00197737933473877,
-0.00879310257408756));
#34060=CARTESIAN_POINT('Ctrl Pts',(-0.219210397264156,0.00210431985748318,
-0.00888947722217451));
#34061=CARTESIAN_POINT('Ctrl Pts',(-0.219169695880014,0.00227317409004623,
-0.009010265597418));
#34062=CARTESIAN_POINT('Ctrl Pts',(-0.219125114125995,0.00246844791056431,
-0.00914120233515241));
#34063=CARTESIAN_POINT('Ctrl Pts',(-0.219104107029856,0.00256264491586247,
-0.0092027760354157));
#34064=CARTESIAN_POINT('Ctrl Pts',(-0.219065185789401,0.0027495795362576,
-0.00932001390846926));
#34065=CARTESIAN_POINT('Ctrl Pts',(-0.219025709089311,0.00295899128206887,
-0.00944417732113124));
#34066=CARTESIAN_POINT('Ctrl Pts',(-0.218983512591821,0.00321686005853762,
-0.00958744196166714));
#34067=CARTESIAN_POINT('Ctrl Pts',(-0.218946533756309,0.00351210751955368,
-0.00973738318907154));
#34068=CARTESIAN_POINT('Ctrl Pts',(-0.21890460182961,0.00394769638303296,
-0.0099397871903584));
#34069=CARTESIAN_POINT('Ctrl Pts',(-0.218883863192036,0.00433227617929637,
-0.0100887511287044));
#34070=CARTESIAN_POINT('Ctrl Pts',(-0.218875329342033,0.00458003691306957,
-0.0101730362524699));
#34071=CARTESIAN_POINT('Ctrl Pts',(-0.218875283101098,0.004581383707407,
-0.0101734940573489));
#34072=CARTESIAN_POINT('',(-0.218991324367386,0.0075019122725732,-0.0106570283411247));
#34073=CARTESIAN_POINT('Ctrl Pts',(-0.218875283101098,0.004581383707407,
-0.0101734940573489));
#34074=CARTESIAN_POINT('Ctrl Pts',(-0.218866870630764,0.00482640183843447,
-0.0102567810839603));
#34075=CARTESIAN_POINT('Ctrl Pts',(-0.218860428272785,0.00530009638128035,
-0.010394044359322));
#34076=CARTESIAN_POINT('Ctrl Pts',(-0.21887680296636,0.00591647553201763,
-0.0105204386808791));
#34077=CARTESIAN_POINT('Ctrl Pts',(-0.218898906555435,0.00630803933518748,
-0.0105773429465142));
#34078=CARTESIAN_POINT('Ctrl Pts',(-0.218915046210659,0.00655448980943694,
-0.0106066073820039));
#34079=CARTESIAN_POINT('Ctrl Pts',(-0.218931315724247,0.00677698709341947,
-0.0106272402886752));
#34080=CARTESIAN_POINT('Ctrl Pts',(-0.218940988343653,0.00690018648445271,
-0.0106362673398873));
#34081=CARTESIAN_POINT('Ctrl Pts',(-0.218960350606911,0.00713991109271049,
-0.0106507120235621));
#34082=CARTESIAN_POINT('Ctrl Pts',(-0.218977853687112,0.00734620133041628,
-0.0106567570334487));
#34083=CARTESIAN_POINT('Ctrl Pts',(-0.218991324367386,0.0075019122725732,
-0.0106570283411247));
#34084=CARTESIAN_POINT('',(-0.218873033347197,0.0104354629346669,-0.0101677297475496));
#34085=CARTESIAN_POINT('Ctrl Pts',(-0.218991324487739,0.00750191366376445,
-0.0106570283435486));
#34086=CARTESIAN_POINT('Ctrl Pts',(-0.218977714066313,0.00765844874886421,
-0.0106566873977884));
#34087=CARTESIAN_POINT('Ctrl Pts',(-0.218960026395843,0.00786583414945123,
-0.010650493139574));
#34088=CARTESIAN_POINT('Ctrl Pts',(-0.218940437271565,0.00810702606773746,
-0.0106357748472563));
#34089=CARTESIAN_POINT('Ctrl Pts',(-0.218930665620513,0.00823074935764031,
-0.0106266120296459));
#34090=CARTESIAN_POINT('Ctrl Pts',(-0.218914122265686,0.00845551885065929,
-0.0106055490032873));
#34091=CARTESIAN_POINT('Ctrl Pts',(-0.218897729797661,0.00870399621762634,
-0.010575730408042));
#34092=CARTESIAN_POINT('Ctrl Pts',(-0.218875282033582,0.009098281554932,
-0.0105178852734934));
#34093=CARTESIAN_POINT('Ctrl Pts',(-0.218858574729261,0.00971840699337653,
-0.0103892973309567));
#34094=CARTESIAN_POINT('Ctrl Pts',(-0.218864545490841,0.0101899590796915,
-0.010251929948102));
#34095=CARTESIAN_POINT('Ctrl Pts',(-0.218873033347197,0.0104354629346669,
-0.0101677297475496));
#34096=CARTESIAN_POINT('',(-0.219239360238103,0.0130430516485843,-0.00877739741392787));
#34097=CARTESIAN_POINT('Ctrl Pts',(-0.218873033347197,0.0104354629346669,
-0.0101677297475496));
#34098=CARTESIAN_POINT('Ctrl Pts',(-0.218873073881679,0.0104366353592755,
-0.010167327642307));
#34099=CARTESIAN_POINT('Ctrl Pts',(-0.218881669369809,0.0106845336709657,
-0.0100822476343057));
#34100=CARTESIAN_POINT('Ctrl Pts',(-0.218910030592733,0.0112002405915132,
-0.00988053471852809));
#34101=CARTESIAN_POINT('Ctrl Pts',(-0.218966215343186,0.0117059336228815,
-0.00963087579587884));
#34102=CARTESIAN_POINT('Ctrl Pts',(-0.219024577480456,0.0120623302121355,
-0.00943183626992845));
#34103=CARTESIAN_POINT('Ctrl Pts',(-0.219063926983141,0.0122714635384721,
-0.00930705603696086));
#34104=CARTESIAN_POINT('Ctrl Pts',(-0.219102562059971,0.0124578218778547,
-0.00918947672058609));
#34105=CARTESIAN_POINT('Ctrl Pts',(-0.219123412166533,0.0125519183301058,
-0.00912760747078243));
#34106=CARTESIAN_POINT('Ctrl Pts',(-0.219167638695722,0.0127470745854724,
-0.00899597806498157));
#34107=CARTESIAN_POINT('Ctrl Pts',(-0.219207998992883,0.0129160142680807,
-0.00887442197202375));
#34108=CARTESIAN_POINT('Ctrl Pts',(-0.219239355956135,0.0130430487440735,
-0.00877739980923923));
#34109=CARTESIAN_POINT('',(-0.220511173800118,0.0132638184474622,-0.00862591209587123));
#34110=CARTESIAN_POINT('Ctrl Pts',(-0.219239360856092,0.0130430506754479,
-0.00877739805133272));
#34111=CARTESIAN_POINT('Ctrl Pts',(-0.219298950996701,0.0130687144123312,
-0.00875880433339075));
#34112=CARTESIAN_POINT('Ctrl Pts',(-0.219358531392433,0.0130945392596808,
-0.00873977229127666));
#34113=CARTESIAN_POINT('Ctrl Pts',(-0.219411335221623,0.0131167513828459,
-0.00872328489173723));
#34114=CARTESIAN_POINT('Ctrl Pts',(-0.219464140496835,0.013138964114286,
-0.00870679704069332));
#34115=CARTESIAN_POINT('Ctrl Pts',(-0.219500760265905,0.013153861192503,
-0.00869564715063633));
#34116=CARTESIAN_POINT('Ctrl Pts',(-0.219546226692826,0.0131713559086997,
-0.0086825393609088));
#34117=CARTESIAN_POINT('Ctrl Pts',(-0.219591693119748,0.0131888506248964,
-0.00866943157118127));
#34118=CARTESIAN_POINT('Ctrl Pts',(-0.21964621378914,0.0132085111685916,
-0.00865465912376249));
#34119=CARTESIAN_POINT('Ctrl Pts',(-0.219698198990407,0.0132250723510747,
-0.00864224352548852));
#34120=CARTESIAN_POINT('Ctrl Pts',(-0.219750184191674,0.0132416335335577,
-0.00862982792721455));
#34121=CARTESIAN_POINT('Ctrl Pts',(-0.219799465343604,0.0132554691542827,
-0.00861948547653094));
#34122=CARTESIAN_POINT('Ctrl Pts',(-0.219852540605556,0.0132676479975295,
-0.00861050659516199));
#34123=CARTESIAN_POINT('Ctrl Pts',(-0.219905615867508,0.0132798268407764,
-0.00860152771379304));
#34124=CARTESIAN_POINT('Ctrl Pts',(-0.219962601807985,0.0132900276350841,
-0.00859416917716125));
#34125=CARTESIAN_POINT('Ctrl Pts',(-0.22001809697308,0.0132963990632951,
-0.00858991670627559));
#34126=CARTESIAN_POINT('Ctrl Pts',(-0.220073592138176,0.0133027704915062,
-0.00858566423538993));
#34127=CARTESIAN_POINT('Ctrl Pts',(-0.220127543994927,0.0133055155736895,
-0.00858435336394495));
#34128=CARTESIAN_POINT('Ctrl Pts',(-0.220180503294847,0.0133043243406397,
-0.00858630552910945));
#34129=CARTESIAN_POINT('Ctrl Pts',(-0.220206982944806,0.0133037287241147,
-0.0085872816116917));
#34130=CARTESIAN_POINT('Ctrl Pts',(-0.220232730829742,0.0133021797482245,
-0.00858903927174345));
#34131=CARTESIAN_POINT('Ctrl Pts',(-0.22026032775548,0.013299662179195,
-0.00859163540799559));
#34132=CARTESIAN_POINT('Ctrl Pts',(-0.220287924681219,0.0132971446101655,
-0.00859423154424774));
#34133=CARTESIAN_POINT('Ctrl Pts',(-0.22031735564104,0.0132935272221941,
-0.00859777443096918));
#34134=CARTESIAN_POINT('Ctrl Pts',(-0.220343331894914,0.0132899564633698,
-0.00860121291144217));
#34135=CARTESIAN_POINT('Ctrl Pts',(-0.220369308148789,0.0132863857045454,
-0.00860465139191516));
#34136=CARTESIAN_POINT('Ctrl Pts',(-0.22037830388446,0.0132847864229076,
-0.00860614092202279));
#34137=CARTESIAN_POINT('Ctrl Pts',(-0.22040632557493,0.0132804512126285,
-0.00861024553754777));
#34138=CARTESIAN_POINT('Ctrl Pts',(-0.220434276772263,0.0132761269082787,
-0.00861433982724225));
#34139=CARTESIAN_POINT('Ctrl Pts',(-0.220465993395677,0.0132709838364459,
-0.00861918120032084));
#34140=CARTESIAN_POINT('Ctrl Pts',(-0.220510858531432,0.0132638681299273,
-0.00862586523173163));
#34141=CARTESIAN_POINT('',(-0.220090131945959,0.0108157693199988,-0.0100543335553095));
#34142=CARTESIAN_POINT('Ctrl Pts',(-0.220511198231108,0.0132638143311653,
-0.00862591593995484));
#34143=CARTESIAN_POINT('Ctrl Pts',(-0.220474612184434,0.013132908947053,
-0.00873278603088295));
#34144=CARTESIAN_POINT('Ctrl Pts',(-0.220427708291213,0.0129593513417706,
-0.00886587344975926));
#34145=CARTESIAN_POINT('Ctrl Pts',(-0.220376512267889,0.0127601128577709,
-0.00900883800189919));
#34146=CARTESIAN_POINT('Ctrl Pts',(-0.220353002206104,0.0126668690042777,
-0.00907408224202567));
#34147=CARTESIAN_POINT('Ctrl Pts',(-0.220307516279135,0.0124745968776834,
-0.00920306768613607));
#34148=CARTESIAN_POINT('Ctrl Pts',(-0.220261403766907,0.0122600991432045,
-0.009338899311862));
#34149=CARTESIAN_POINT('Ctrl Pts',(-0.220211695130772,0.0119970268718438,
-0.00949498790625071));
#34150=CARTESIAN_POINT('Ctrl Pts',(-0.220166577384904,0.0116890499212551,
-0.009661813304815));
#34151=CARTESIAN_POINT('Ctrl Pts',(-0.220123247623221,0.011305666268294,
-0.00985154441700039));
#34152=CARTESIAN_POINT('Ctrl Pts',(-0.220100481153719,0.0109961152750341,
-0.00998355150383413));
#34153=CARTESIAN_POINT('Ctrl Pts',(-0.220090131945959,0.0108157693199988,
-0.0100543335553095));
#34154=CARTESIAN_POINT('',(-0.22019175144594,0.00750243957431793,-0.010684158764387));
#34155=CARTESIAN_POINT('Ctrl Pts',(-0.220090131945959,0.0108157693199988,
-0.0100543335553095));
#34156=CARTESIAN_POINT('Ctrl Pts',(-0.220085557370637,0.0107360524784264,
-0.0100856207642881));
#34157=CARTESIAN_POINT('Ctrl Pts',(-0.22006845689036,0.0103958729688586,
-0.0102140461491421));
#34158=CARTESIAN_POINT('Ctrl Pts',(-0.220057020156484,0.00982779650229385,
-0.0103888558048875));
#34159=CARTESIAN_POINT('Ctrl Pts',(-0.220072085364924,0.00917638566997734,
-0.0105309147603936));
#34160=CARTESIAN_POINT('Ctrl Pts',(-0.220094819050192,0.00876357564947826,
-0.0105945725520012));
#34161=CARTESIAN_POINT('Ctrl Pts',(-0.220111615632777,0.00850307729270115,
-0.0106274384754032));
#34162=CARTESIAN_POINT('Ctrl Pts',(-0.220128755043961,0.00826671083837223,
-0.0106507003321801));
#34163=CARTESIAN_POINT('Ctrl Pts',(-0.220138784930233,0.00813832419183378,
-0.010660684037487));
#34164=CARTESIAN_POINT('Ctrl Pts',(-0.22015910220265,0.00788550868615409,
-0.0106769231726282));
#34165=CARTESIAN_POINT('Ctrl Pts',(-0.220177533161667,0.00766742881797243,
-0.0106837925977353));
#34166=CARTESIAN_POINT('Ctrl Pts',(-0.22019175281392,0.00750244141589442,
-0.0106841588886674));
#34167=CARTESIAN_POINT('',(-0.220081376539163,0.00442299110476343,-0.0101444921821041));
#34168=CARTESIAN_POINT('Ctrl Pts',(-0.220191752647251,0.00750243947116139,
-0.0106841588854298));
#34169=CARTESIAN_POINT('Ctrl Pts',(-0.220177578180119,0.00733704887202067,
-0.0106838835219745));
#34170=CARTESIAN_POINT('Ctrl Pts',(-0.22015922048139,0.00711852767169112,
-0.0106771046134885));
#34171=CARTESIAN_POINT('Ctrl Pts',(-0.220139015624589,0.00686530054035368,
-0.0106609453039589));
#34172=CARTESIAN_POINT('Ctrl Pts',(-0.220129069993647,0.00673700584535355,
-0.010651026291088));
#34173=CARTESIAN_POINT('Ctrl Pts',(-0.220112044459368,0.00649988309557624,
-0.0106277828308853));
#34174=CARTESIAN_POINT('Ctrl Pts',(-0.220095442997511,0.00623893652743939,
-0.0105949464252065));
#34175=CARTESIAN_POINT('Ctrl Pts',(-0.220073138675426,0.00582541150882776,
-0.0105312604256392));
#34176=CARTESIAN_POINT('Ctrl Pts',(-0.220059160562007,0.00517687267843841,
-0.0103901109544776));
#34177=CARTESIAN_POINT('Ctrl Pts',(-0.220069811611103,0.00468149176814678,
-0.010238002757777));
#34178=CARTESIAN_POINT('Ctrl Pts',(-0.220081376539163,0.00442299110476343,
-0.0101444921821041));
#34179=CARTESIAN_POINT('Ctrl Pts',(-0.22008140790703,0.00442229028145444,
-0.0101442386316291));
#34180=CARTESIAN_POINT('Ctrl Pts',(-0.220092994577836,0.00416353624782033,
-0.010050611906748));
#34181=CARTESIAN_POINT('Ctrl Pts',(-0.22011975529717,0.00375896969551987,
-0.00988387768562756));
#34182=CARTESIAN_POINT('Ctrl Pts',(-0.220171662014429,0.00330655391001369,
-0.0096595890396178));
#34183=CARTESIAN_POINT('Ctrl Pts',(-0.220217007334562,0.00300150929740094,
-0.00949424527209877));
#34184=CARTESIAN_POINT('Ctrl Pts',(-0.220267680085307,0.00273767985326313,
-0.00933766032672383));
#34185=CARTESIAN_POINT('Ctrl Pts',(-0.220314530683991,0.00252326153527256,
-0.00920181247202401));
#34186=CARTESIAN_POINT('Ctrl Pts',(-0.220360978000976,0.00233010820899768,
-0.0090721446842305));
#34187=CARTESIAN_POINT('Ctrl Pts',(-0.220384350015444,0.00223890246433455,
-0.00900828010102458));
#34188=CARTESIAN_POINT('Ctrl Pts',(-0.220436257236716,0.00203984277084597,
-0.00886543629554137));
#34189=CARTESIAN_POINT('Ctrl Pts',(-0.220484038290209,0.00186542210487714,
-0.00873168119613634));
#34190=CARTESIAN_POINT('Ctrl Pts',(-0.2205214329925,0.00173338441996231,
-0.00862380411186018));
#34191=CARTESIAN_POINT('',(-0.218374793789608,0.00221918351113939,-0.0089535596216209));
#34192=CARTESIAN_POINT('',(-0.217726229879918,0.00223894560702424,-0.00895610833897201));
#34193=CARTESIAN_POINT('Ctrl Pts',(-0.218375409693209,0.00221079122986865,
-0.00894874908347634));
#34194=CARTESIAN_POINT('Ctrl Pts',(-0.218295547237171,0.00221203449658772,
-0.00894808355786149));
#34195=CARTESIAN_POINT('Ctrl Pts',(-0.218197262847863,0.00221365986816565,
-0.00894733157532527));
#34196=CARTESIAN_POINT('Ctrl Pts',(-0.218095525843496,0.00221584476839926,
-0.00894690951729281));
#34197=CARTESIAN_POINT('Ctrl Pts',(-0.21806412726539,0.00221644786389076,
-0.00894672852039272));
#34198=CARTESIAN_POINT('Ctrl Pts',(-0.217956617159952,0.00222021619904336,
-0.00894731928771769));
#34199=CARTESIAN_POINT('Ctrl Pts',(-0.217848140139888,0.0022267806586541,
-0.00894987064576114));
#34200=CARTESIAN_POINT('Ctrl Pts',(-0.217779211918502,0.00223241879127506,
-0.00895252955645527));
#34201=CARTESIAN_POINT('Ctrl Pts',(-0.217726229879918,0.00223894560702424,
-0.00895610833897201));
#34202=CARTESIAN_POINT('',(-0.217123286376409,0.00243485131310274,-0.00907883473156682));
#34203=CARTESIAN_POINT('Ctrl Pts',(-0.217725491044994,0.0022390367465584,
-0.00895615833124103));
#34204=CARTESIAN_POINT('Ctrl Pts',(-0.217672196328649,0.00224561982685404,
-0.00895977065528357));
#34205=CARTESIAN_POINT('Ctrl Pts',(-0.217551154797832,0.00226440842063028,
-0.00897066068600668));
#34206=CARTESIAN_POINT('Ctrl Pts',(-0.217408393547704,0.00230150415104225,
-0.00899375480814277));
#34207=CARTESIAN_POINT('Ctrl Pts',(-0.217285693066462,0.00234646807569697,
-0.00902240631599514));
#34208=CARTESIAN_POINT('Ctrl Pts',(-0.217185031478673,0.00239905726908142,
-0.00905606193974296));
#34209=CARTESIAN_POINT('Ctrl Pts',(-0.217158224898363,0.00241473880623142,
-0.00906610084421658));
#34210=CARTESIAN_POINT('Ctrl Pts',(-0.217123288446565,0.00243483964324871,
-0.00907882698336438));
#34211=CARTESIAN_POINT('',(-0.216865219429701,0.00485302928795331,-0.0102164733809617));
#34212=CARTESIAN_POINT('Ctrl Pts',(-0.217123286376409,0.00243485131310274,
-0.00907883473156682));
#34213=CARTESIAN_POINT('Ctrl Pts',(-0.217102113171765,0.00255420866614419,
-0.00915808195356356));
#34214=CARTESIAN_POINT('Ctrl Pts',(-0.21708380628641,0.00266021556918632,
-0.0092245717761884));
#34215=CARTESIAN_POINT('Ctrl Pts',(-0.217067506905344,0.00275710066248676,
-0.009283221761031));
#34216=CARTESIAN_POINT('Ctrl Pts',(-0.217059356949207,0.00280554478791243,
-0.00931254770917369));
#34217=CARTESIAN_POINT('Ctrl Pts',(-0.217051709940288,0.00285174138298016,
-0.00933986164713557));
#34218=CARTESIAN_POINT('Ctrl Pts',(-0.217045421662262,0.00289008361015183,
-0.00936219529050879));
#34219=CARTESIAN_POINT('Ctrl Pts',(-0.217039133384235,0.0029284258373235,
-0.009384528933882));
#34220=CARTESIAN_POINT('Ctrl Pts',(-0.21703420124665,0.00295883822773935,
-0.00940200972756825));
#34221=CARTESIAN_POINT('Ctrl Pts',(-0.217027206770864,0.00300335905250413,
-0.00942710119986508));
#34222=CARTESIAN_POINT('Ctrl Pts',(-0.217020212295079,0.00304787987726892,
-0.0094521926721619));
#34223=CARTESIAN_POINT('Ctrl Pts',(-0.217011160118175,0.00310663789704563,
-0.00948466851452673));
#34224=CARTESIAN_POINT('Ctrl Pts',(-0.217003118562495,0.00316070130514153,
-0.00951375775303658));
#34225=CARTESIAN_POINT('Ctrl Pts',(-0.216995077006816,0.00321476471323742,
-0.00954284699154643));
#34226=CARTESIAN_POINT('Ctrl Pts',(-0.216988042899663,0.00326405254348306,
-0.00956870246583691));
#34227=CARTESIAN_POINT('Ctrl Pts',(-0.216981348057688,0.00331234769037973,
-0.00959353732849681));
#34228=CARTESIAN_POINT('Ctrl Pts',(-0.216967958373738,0.00340893798417307,
-0.0096432070538166));
#34229=CARTESIAN_POINT('Ctrl Pts',(-0.21695592618917,0.00350156050347066,
-0.00968877543301438));
#34230=CARTESIAN_POINT('Ctrl Pts',(-0.216944760158758,0.00359749171350427,
-0.00973398076094292));
#34231=CARTESIAN_POINT('Ctrl Pts',(-0.216922771495283,0.0037864038887724,
-0.00982300118328198));
#34232=CARTESIAN_POINT('Ctrl Pts',(-0.21690415162039,0.00398835918519624,
-0.00991015012701886));
#34233=CARTESIAN_POINT('Ctrl Pts',(-0.216890742090616,0.00419768307541563,
-0.00999111343977628));
#34234=CARTESIAN_POINT('Ctrl Pts',(-0.216890532673751,0.00420095209032992,
-0.00999237784527073));
#34235=CARTESIAN_POINT('Ctrl Pts',(-0.216890324527644,0.00420422288475571,
-0.00999364077261011));
#34236=CARTESIAN_POINT('Ctrl Pts',(-0.216890117659308,0.0042074954350809,
-0.00999490220917792));
#34237=CARTESIAN_POINT('Ctrl Pts',(-0.216876664450443,0.00442031825757234,
-0.010076936850079));
#34238=CARTESIAN_POINT('Ctrl Pts',(-0.216868621236676,0.00464079347560287,
-0.0101522452372161));
#34239=CARTESIAN_POINT('Ctrl Pts',(-0.216865269537596,0.00484988229780852,
-0.010215521621625));
#34240=CARTESIAN_POINT('Ctrl Pts',(-0.216865252717512,0.00485093158400454,
-0.0102158391662741));
#34241=CARTESIAN_POINT('Ctrl Pts',(-0.21686523601491,0.00485198057392772,
-0.0102161564384166));
#34242=CARTESIAN_POINT('Ctrl Pts',(-0.216865219429701,0.00485302928795331,
-0.0102164733809617));
#34243=CARTESIAN_POINT('',(-0.216992039098873,0.00750111755777987,-0.0106118430505361));
#34244=CARTESIAN_POINT('Ctrl Pts',(-0.216865219429701,0.00485302928795331,
-0.0102164733809617));
#34245=CARTESIAN_POINT('Ctrl Pts',(-0.216861931118884,0.0050609521426977,
-0.0102793244231641));
#34246=CARTESIAN_POINT('Ctrl Pts',(-0.216863257542664,0.0052573906192139,
-0.0103315033714261));
#34247=CARTESIAN_POINT('Ctrl Pts',(-0.216868505685461,0.00547448632452407,
-0.0103809849429286));
#34248=CARTESIAN_POINT('Ctrl Pts',(-0.216871142991853,0.00558358165851651,
-0.0104058505134466));
#34249=CARTESIAN_POINT('Ctrl Pts',(-0.216874776812353,0.00569795300210121,
-0.0104297581638601));
#34250=CARTESIAN_POINT('Ctrl Pts',(-0.216879266843606,0.00581122729905882,
-0.0104511884062416));
#34251=CARTESIAN_POINT('Ctrl Pts',(-0.216881511859233,0.00586786444753763,
-0.0104619035274324));
#34252=CARTESIAN_POINT('Ctrl Pts',(-0.216883969709047,0.00592421706211528,
-0.01047205379377));
#34253=CARTESIAN_POINT('Ctrl Pts',(-0.216886933193732,0.00598565404839195,
-0.0104824658612332));
#34254=CARTESIAN_POINT('Ctrl Pts',(-0.216889896678417,0.00604709103466862,
-0.0104928779286964));
#34255=CARTESIAN_POINT('Ctrl Pts',(-0.216893369691221,0.00611364246361058,
-0.0105033779096584));
#34256=CARTESIAN_POINT('Ctrl Pts',(-0.216896123391226,0.00616408061379814,
-0.0105109157434318));
#34257=CARTESIAN_POINT('Ctrl Pts',(-0.216898877091231,0.00621451876398571,
-0.0105184535772053));
#34258=CARTESIAN_POINT('Ctrl Pts',(-0.216900906026196,0.00624880836994755,
-0.0105232721194047));
#34259=CARTESIAN_POINT('Ctrl Pts',(-0.216903405858141,0.00628979497340091,
-0.0105288248191684));
#34260=CARTESIAN_POINT('Ctrl Pts',(-0.216905905690085,0.00633078157685427,
-0.010534377518932));
#34261=CARTESIAN_POINT('Ctrl Pts',(-0.216908879346214,0.00637848184697154,
-0.0105405341876129));
#34262=CARTESIAN_POINT('Ctrl Pts',(-0.216912033183608,0.00642730938192668,
-0.0105464029380313));
#34263=CARTESIAN_POINT('Ctrl Pts',(-0.216918340858396,0.00652496445183697,
-0.010558140438868));
#34264=CARTESIAN_POINT('Ctrl Pts',(-0.216925365659119,0.00662711239577533,
-0.0105688859918395));
#34265=CARTESIAN_POINT('Ctrl Pts',(-0.2169333224102,0.00673786809107805,
-0.0105783972974196));
#34266=CARTESIAN_POINT('Ctrl Pts',(-0.216949235882187,0.00695937906166578,
-0.0105974198725104));
#34267=CARTESIAN_POINT('Ctrl Pts',(-0.216968880550106,0.00721532289054462,
-0.0106113550043929));
#34268=CARTESIAN_POINT('Ctrl Pts',(-0.21699203903428,0.00750111756314772,
-0.0106118429721946));
#34269=CARTESIAN_POINT('',(-0.216863263875865,0.0101606619361279,-0.010212275920378));
#34270=CARTESIAN_POINT('Ctrl Pts',(-0.216992039166016,0.00750111918887558,
-0.0106118429749703));
#34271=CARTESIAN_POINT('Ctrl Pts',(-0.216968632225441,0.00778826296106311,
-0.0106112783068527));
#34272=CARTESIAN_POINT('Ctrl Pts',(-0.216948771168368,0.00804539121894196,
-0.0105971483131848));
#34273=CARTESIAN_POINT('Ctrl Pts',(-0.216932675029404,0.00826792612051201,
-0.0105778926417949));
#34274=CARTESIAN_POINT('Ctrl Pts',(-0.216924626959922,0.00837919357129703,
-0.0105682648061));
#34275=CARTESIAN_POINT('Ctrl Pts',(-0.216917519271334,0.00848181317185611,
-0.0105573930115986));
#34276=CARTESIAN_POINT('Ctrl Pts',(-0.216911135474933,0.00857989135437507,
-0.0105455248340113));
#34277=CARTESIAN_POINT('Ctrl Pts',(-0.216907943576732,0.00862893044563455,
-0.0105395907452177));
#34278=CARTESIAN_POINT('Ctrl Pts',(-0.21690493355368,0.00867683009665796,
-0.010533367524606));
#34279=CARTESIAN_POINT('Ctrl Pts',(-0.216902401326156,0.00871801683620453,
-0.0105277512234802));
#34280=CARTESIAN_POINT('Ctrl Pts',(-0.216899869098632,0.00875920357575109,
-0.0105221349223544));
#34281=CARTESIAN_POINT('Ctrl Pts',(-0.216897811733291,0.00879369422056019,
-0.0105172560114583));
#34282=CARTESIAN_POINT('Ctrl Pts',(-0.216895024263018,0.00884428163387125,
-0.0105096476733168));
#34283=CARTESIAN_POINT('Ctrl Pts',(-0.216892236792745,0.00889486904718231,
-0.0105020393351752));
#34284=CARTESIAN_POINT('Ctrl Pts',(-0.21688872467329,0.00896151771075859,
-0.0104914585369431));
#34285=CARTESIAN_POINT('Ctrl Pts',(-0.216885723173758,0.00902305138276646,
-0.0104809685050821));
#34286=CARTESIAN_POINT('Ctrl Pts',(-0.216882721674225,0.00908458505477434,
-0.0104704784732212));
#34287=CARTESIAN_POINT('Ctrl Pts',(-0.216880226901671,0.00914103396809379,
-0.0104602530991236));
#34288=CARTESIAN_POINT('Ctrl Pts',(-0.216877944706416,0.00919776531074823,
-0.0104494608864153));
#34289=CARTESIAN_POINT('Ctrl Pts',(-0.216873380315907,0.0093112279960571,
-0.0104278764609987));
#34290=CARTESIAN_POINT('Ctrl Pts',(-0.216869671153504,0.00942577893288784,
-0.0104038046864359));
#34291=CARTESIAN_POINT('Ctrl Pts',(-0.216866955637489,0.00953491448523924,
-0.0103788076593657));
#34292=CARTESIAN_POINT('Ctrl Pts',(-0.216861524605459,0.00975318558994206,
-0.0103288136052253));
#34293=CARTESIAN_POINT('Ctrl Pts',(-0.21686004247206,0.00995004301390614,
-0.0102762708499468));
#34294=CARTESIAN_POINT('Ctrl Pts',(-0.216863248962655,0.0101596890081031,
-0.0102125715953075));
#34295=CARTESIAN_POINT('Ctrl Pts',(-0.216863253922439,0.0101600132874919,
-0.0102124730656149));
#34296=CARTESIAN_POINT('Ctrl Pts',(-0.216863258893508,0.0101603375965186,
-0.0102123745061583));
#34297=CARTESIAN_POINT('Ctrl Pts',(-0.216863263875865,0.0101606619361279,
-0.010212275920378));
#34298=CARTESIAN_POINT('',(-0.217121128085406,0.012579797101843,-0.00906899462937275));
#34299=CARTESIAN_POINT('Ctrl Pts',(-0.216863263875865,0.0101606619361279,
-0.010212275920378));
#34300=CARTESIAN_POINT('Ctrl Pts',(-0.21686647997781,0.0103700218636815,
-0.0101486367803184));
#34301=CARTESIAN_POINT('Ctrl Pts',(-0.21687439950964,0.010591699526372,
-0.0100726047017749));
#34302=CARTESIAN_POINT('Ctrl Pts',(-0.216887811284844,0.01080539853155,
-0.00998985337042852));
#34303=CARTESIAN_POINT('Ctrl Pts',(-0.216901243837455,0.0110194285973771,
-0.00990697384143589));
#34304=CARTESIAN_POINT('Ctrl Pts',(-0.216920179082265,0.0112256173796445,
-0.00981766775388043));
#34305=CARTESIAN_POINT('Ctrl Pts',(-0.216942545157854,0.0114176480916229,
-0.00972674550743857));
#34306=CARTESIAN_POINT('Ctrl Pts',(-0.216953728195649,0.0115136634476121,
-0.00968128438421765));
#34307=CARTESIAN_POINT('Ctrl Pts',(-0.216965766307836,0.011606196353727,
-0.00963554356500761));
#34308=CARTESIAN_POINT('Ctrl Pts',(-0.216979152369634,0.0117026516621678,
-0.00958571758408353));
#34309=CARTESIAN_POINT('Ctrl Pts',(-0.216985845400533,0.0117508793163882,
-0.0095608045936215));
#34310=CARTESIAN_POINT('Ctrl Pts',(-0.21699287531768,0.0118000881067751,
-0.00953487462933585));
#34311=CARTESIAN_POINT('Ctrl Pts',(-0.217000911950288,0.0118540545891475,
-0.00950570975585976));
#34312=CARTESIAN_POINT('Ctrl Pts',(-0.217008948582896,0.0119080210715199,
-0.00947654488238367));
#34313=CARTESIAN_POINT('Ctrl Pts',(-0.217017995097714,0.0119666640174066,
-0.00944399243305965));
#34314=CARTESIAN_POINT('Ctrl Pts',(-0.21702497551412,0.0120110411913712,
-0.00941887608284972));
#34315=CARTESIAN_POINT('Ctrl Pts',(-0.217031955930525,0.0120554183653357,
-0.00939375973263978));
#34316=CARTESIAN_POINT('Ctrl Pts',(-0.217036865614439,0.012085659087643,
-0.00937630582863259));
#34317=CARTESIAN_POINT('Ctrl Pts',(-0.217043142812678,0.0121239056967825,
-0.00935393704026712));
#34318=CARTESIAN_POINT('Ctrl Pts',(-0.217049420010916,0.012162152305922,
-0.00933156825190165));
#34319=CARTESIAN_POINT('Ctrl Pts',(-0.21705706731629,0.0122083289073836,
-0.00930415691288176));
#34320=CARTESIAN_POINT('Ctrl Pts',(-0.217065224007411,0.0122568003427244,
-0.0092746964595612));
#34321=CARTESIAN_POINT('Ctrl Pts',(-0.217081537389652,0.0123537432134059,
-0.00921577555292007));
#34322=CARTESIAN_POINT('Ctrl Pts',(-0.217099884128624,0.0124599993389447,
-0.00914886769251459));
#34323=CARTESIAN_POINT('Ctrl Pts',(-0.217121128085406,0.012579797101843,
-0.00906899462937275));
#34324=CARTESIAN_POINT('',(-0.218370318086279,0.0127783343977889,-0.00895639519171424));
#34325=CARTESIAN_POINT('Ctrl Pts',(-0.217121134551835,0.0125797994500258,
-0.00906899318316964));
#34326=CARTESIAN_POINT('Ctrl Pts',(-0.217191804233479,0.0126054620271479,
-0.00905318806274778));
#34327=CARTESIAN_POINT('Ctrl Pts',(-0.217256223599339,0.0126283520543175,
-0.00903890986338815));
#34328=CARTESIAN_POINT('Ctrl Pts',(-0.217302115212182,0.0126446977363176,
-0.0090286476961318));
#34329=CARTESIAN_POINT('Ctrl Pts',(-0.217348008224749,0.0126610439168714,
-0.00901838521587279));
#34330=CARTESIAN_POINT('Ctrl Pts',(-0.217375371780285,0.0126708651259043,
-0.00901216817068204));
#34331=CARTESIAN_POINT('Ctrl Pts',(-0.217421043282157,0.0126856582776629,
-0.00900283837934702));
#34332=CARTESIAN_POINT('Ctrl Pts',(-0.217466714784029,0.0127004514294214,
-0.008993508588012));
#34333=CARTESIAN_POINT('Ctrl Pts',(-0.217530695084449,0.0127201865022325,
-0.00898102254617446));
#34334=CARTESIAN_POINT('Ctrl Pts',(-0.217583564792478,0.0127352872287596,
-0.00897146523766335));
#34335=CARTESIAN_POINT('Ctrl Pts',(-0.217636434500507,0.0127503879552868,
-0.00896190792915224));
#34336=CARTESIAN_POINT('Ctrl Pts',(-0.217678193008114,0.0127608763428775,
-0.00895531057012255));
#34337=CARTESIAN_POINT('Ctrl Pts',(-0.217729528732368,0.0127712441764474,
-0.0089489621938623));
#34338=CARTESIAN_POINT('Ctrl Pts',(-0.217780864456622,0.0127816120100172,
-0.00894261381760204));
#34339=CARTESIAN_POINT('Ctrl Pts',(-0.217841777631961,0.0127918506441235,
-0.00893650234048543));
#34340=CARTESIAN_POINT('Ctrl Pts',(-0.217895152298986,0.0127988050770367,
-0.00893256964675583));
#34341=CARTESIAN_POINT('Ctrl Pts',(-0.217948526966011,0.0128057595099498,
-0.00892863695302623));
#34342=CARTESIAN_POINT('Ctrl Pts',(-0.217994363019984,0.012809433646628,
-0.00892688845320798));
#34343=CARTESIAN_POINT('Ctrl Pts',(-0.21805055697462,0.0128092199536068,
-0.0089281316531678));
#34344=CARTESIAN_POINT('Ctrl Pts',(-0.218106750929257,0.0128090062605855,
-0.00892937485312762));
#34345=CARTESIAN_POINT('Ctrl Pts',(-0.218173302827974,0.0128049031209714,
-0.00893360751126326));
#34346=CARTESIAN_POINT('Ctrl Pts',(-0.218210920925695,0.0128010511373276,
-0.00893709374166423));
#34347=CARTESIAN_POINT('Ctrl Pts',(-0.218229729974556,0.0127991251455056,
-0.00893883685686471));
#34348=CARTESIAN_POINT('Ctrl Pts',(-0.218241305558444,0.0127972624849013,
-0.00894039412328682));
#34349=CARTESIAN_POINT('Ctrl Pts',(-0.218265649751042,0.0127936761158908,
-0.00894342788658745));
#34350=CARTESIAN_POINT('Ctrl Pts',(-0.218289993402882,0.0127900898265444,
-0.0089464615824991));
#34351=CARTESIAN_POINT('Ctrl Pts',(-0.218327105109004,0.0127847794349534,
-0.00895097104991555));
#34352=CARTESIAN_POINT('Ctrl Pts',(-0.218370317942987,0.0127783336174386,
-0.00895639540594475));
#34353=CARTESIAN_POINT('',(-0.218192328823198,0.00750145352954351,-0.0106389704498565));
#34354=CARTESIAN_POINT('Ctrl Pts',(-0.21837032082272,0.0127783331878846,
-0.00895639576742774));
#34355=CARTESIAN_POINT('Ctrl Pts',(-0.2183439323543,0.012652728887447,-0.00904519967598788));
#34356=CARTESIAN_POINT('Ctrl Pts',(-0.218310137320484,0.012487227094208,
-0.00915553509374897));
#34357=CARTESIAN_POINT('Ctrl Pts',(-0.218273310798793,0.0122983058782609,
-0.00927380836242531));
#34358=CARTESIAN_POINT('Ctrl Pts',(-0.218256491297685,0.0122105314035711,
-0.00932747218006369));
#34359=CARTESIAN_POINT('Ctrl Pts',(-0.218223737672891,0.0120283826649878,
-0.00943442067100643));
#34360=CARTESIAN_POINT('Ctrl Pts',(-0.218190747060741,0.011826330921257,
-0.00954666467228927));
#34361=CARTESIAN_POINT('Ctrl Pts',(-0.218141804676599,0.011482855228234,
-0.00972545966649745));
#34362=CARTESIAN_POINT('Ctrl Pts',(-0.218096132925033,0.0110017408951039,
-0.00994723586626805));
#34363=CARTESIAN_POINT('Ctrl Pts',(-0.21806416032289,0.0102673499403875,
-0.0102164366774509));
#34364=CARTESIAN_POINT('Ctrl Pts',(-0.218060939651304,0.00959120948818163,
-0.0104014795600675));
#34365=CARTESIAN_POINT('Ctrl Pts',(-0.218079867987217,0.00900424255639963,
-0.0105156946566394));
#34366=CARTESIAN_POINT('Ctrl Pts',(-0.218102229010278,0.0086333641300724,
-0.0105668629736167));
#34367=CARTESIAN_POINT('Ctrl Pts',(-0.218118265007893,0.00839965564503378,
-0.0105932637896215));
#34368=CARTESIAN_POINT('Ctrl Pts',(-0.218134302478235,0.00818786903454358,
-0.010611949873552));
#34369=CARTESIAN_POINT('Ctrl Pts',(-0.218143594577732,0.00807273732045675,
-0.0106199877322447));
#34370=CARTESIAN_POINT('Ctrl Pts',(-0.218162363505145,0.007845797986924,
-0.0106330829467462));
#34371=CARTESIAN_POINT('Ctrl Pts',(-0.218179293357208,0.00764982103741828,
-0.0106386516765767));
#34372=CARTESIAN_POINT('Ctrl Pts',(-0.218192328410096,0.00750146607432276,
-0.0106389704552747));
#34373=CARTESIAN_POINT('',(-0.218168819694483,0.00722390949581899,-0.0106342099373409));
#34374=CARTESIAN_POINT('Ctrl Pts',(-0.218168819694483,0.00722390949581899,
-0.0106342099373409));
#34375=CARTESIAN_POINT('Ctrl Pts',(-0.218176520975478,0.00731811245431353,
-0.0106372886165177));
#34376=CARTESIAN_POINT('Ctrl Pts',(-0.218184399517934,0.00741054312879059,
-0.0106388058153284));
#34377=CARTESIAN_POINT('Ctrl Pts',(-0.218192384061994,0.00750144032682139,
-0.0106389717172126));
#34378=CARTESIAN_POINT('',(-0.218067226304046,0.00503956785288683,-0.0102972720892691));
#34379=CARTESIAN_POINT('Ctrl Pts',(-0.218067226304046,0.00503956785288683,
-0.0102972720892691));
#34380=CARTESIAN_POINT('Ctrl Pts',(-0.218067185525726,0.00505809304800469,
-0.0103024611533192));
#34381=CARTESIAN_POINT('Ctrl Pts',(-0.218067177931978,0.00507743493358728,
-0.0103078133779122));
#34382=CARTESIAN_POINT('Ctrl Pts',(-0.218067213740286,0.00509763683519755,
-0.0103133285534128));
#34383=CARTESIAN_POINT('Ctrl Pts',(-0.218067323085079,0.0051593256681294,
-0.0103301697769081));
#34384=CARTESIAN_POINT('Ctrl Pts',(-0.218067839272296,0.00522906185989146,
-0.0103484334274165));
#34385=CARTESIAN_POINT('Ctrl Pts',(-0.218068679804542,0.00529559666923563,
-0.0103650231422464));
#34386=CARTESIAN_POINT('Ctrl Pts',(-0.218070360869035,0.00542866628792398,
-0.0103982025719062));
#34387=CARTESIAN_POINT('Ctrl Pts',(-0.218073329595319,0.00554881996646211,
-0.0104251247091534));
#34388=CARTESIAN_POINT('Ctrl Pts',(-0.218076908899421,0.00566137842301226,
-0.0104483888337291));
#34389=CARTESIAN_POINT('Ctrl Pts',(-0.218078698551471,0.00571765765128734,
-0.0104600208960169));
#34390=CARTESIAN_POINT('Ctrl Pts',(-0.218080642275032,0.00577205172292444,
-0.0104706744407793));
#34391=CARTESIAN_POINT('Ctrl Pts',(-0.218082316864294,0.00581688288328235,
-0.0104791407821068));
#34392=CARTESIAN_POINT('Ctrl Pts',(-0.218083991453555,0.00586171404364027,
-0.0104876071234344));
#34393=CARTESIAN_POINT('Ctrl Pts',(-0.218085392599717,0.00589694463862414,
-0.0104940791762582));
#34394=CARTESIAN_POINT('Ctrl Pts',(-0.218087902510866,0.00595381709000237,
-0.0105039369644601));
#34395=CARTESIAN_POINT('Ctrl Pts',(-0.218090412422016,0.0060106895413806,
-0.010513794752662));
#34396=CARTESIAN_POINT('Ctrl Pts',(-0.218094039354121,0.00608926915687774,
-0.0105266693991204));
#34397=CARTESIAN_POINT('Ctrl Pts',(-0.218097647768551,0.00616140852413473,
-0.0105374851630196));
#34398=CARTESIAN_POINT('Ctrl Pts',(-0.21810125618298,0.00623354789139173,
-0.0105483009269187));
#34399=CARTESIAN_POINT('Ctrl Pts',(-0.218104840027185,0.00629920841664498,
-0.0105573273134242));
#34400=CARTESIAN_POINT('Ctrl Pts',(-0.21810864713066,0.00636524535728989,
-0.0105657273357896));
#34401=CARTESIAN_POINT('Ctrl Pts',(-0.21811626133761,0.0064973192385797,
-0.0105825273805204));
#34402=CARTESIAN_POINT('Ctrl Pts',(-0.218124774963466,0.00663092686543204,
-0.010596538903368));
#34403=CARTESIAN_POINT('Ctrl Pts',(-0.21813377702416,0.00676090874178825,
-0.0106073825650924));
#34404=CARTESIAN_POINT('Ctrl Pts',(-0.218144821541264,0.00692038190082795,
-0.0106206865197607));
#34405=CARTESIAN_POINT('Ctrl Pts',(-0.218156597381377,0.00707438379641082,
-0.0106293941026331));
#34406=CARTESIAN_POINT('Ctrl Pts',(-0.218168819694483,0.00722390949581899,
-0.0106342099373409));
#34407=CARTESIAN_POINT('',(-0.218239365786335,0.00292191358914088,-0.00940513443333053));
#34408=CARTESIAN_POINT('Ctrl Pts',(-0.218239365786335,0.00292191358914088,
-0.00940513443333053));
#34409=CARTESIAN_POINT('Ctrl Pts',(-0.218238792806652,0.0029251222736152,
-0.00940698975198401));
#34410=CARTESIAN_POINT('Ctrl Pts',(-0.218238445755819,0.00292708854324504,
-0.00940812657818748));
#34411=CARTESIAN_POINT('Ctrl Pts',(-0.21823756891017,0.00293204686566356,
-0.0094109852334095));
#34412=CARTESIAN_POINT('Ctrl Pts',(-0.218235815218872,0.0029419635105006,
-0.00941670254385354));
#34413=CARTESIAN_POINT('Ctrl Pts',(-0.218231942760466,0.0029638601938198,
-0.00942928697033889));
#34414=CARTESIAN_POINT('Ctrl Pts',(-0.21822787405026,0.00298719841881205,
-0.00944252702285582));
#34415=CARTESIAN_POINT('Ctrl Pts',(-0.218223805340055,0.00301053664380429,
-0.00945576707537276));
#34416=CARTESIAN_POINT('Ctrl Pts',(-0.218219539291199,0.00303528553849307,
-0.00946971592895734));
#34417=CARTESIAN_POINT('Ctrl Pts',(-0.218213751414185,0.0030701619301952,
-0.0094890281096133));
#34418=CARTESIAN_POINT('Ctrl Pts',(-0.218207963537172,0.00310503832189734,
-0.00950834029026926));
#34419=CARTESIAN_POINT('Ctrl Pts',(-0.218200656891965,0.00315012600620321,
-0.00953286696427101));
#34420=CARTESIAN_POINT('Ctrl Pts',(-0.218195678764406,0.00318147339027357,
-0.00954966258126009));
#34421=CARTESIAN_POINT('Ctrl Pts',(-0.218190700636847,0.00321282077434394,
-0.00956645819824917));
#34422=CARTESIAN_POINT('Ctrl Pts',(-0.218188047637253,0.0032303403141343,
-0.00957568617622878));
#34423=CARTESIAN_POINT('Ctrl Pts',(-0.218185146908979,0.00324971646011447,
-0.00958586023691622));
#34424=CARTESIAN_POINT('Ctrl Pts',(-0.218182246180705,0.00326909260609464,
-0.00959603429760365));
#34425=CARTESIAN_POINT('Ctrl Pts',(-0.218179098878308,0.00329035409754875,
-0.00960709906973049));
#34426=CARTESIAN_POINT('Ctrl Pts',(-0.218176253632057,0.00331011660456465,
-0.00961729005975538));
#34427=CARTESIAN_POINT('Ctrl Pts',(-0.218170563139556,0.00334964161859643,
-0.00963767203980516));
#34428=CARTESIAN_POINT('Ctrl Pts',(-0.218166080234634,0.00338315645788068,
-0.00965458901309295));
#34429=CARTESIAN_POINT('Ctrl Pts',(-0.218162997197411,0.00340695588194977,
-0.00966651052277642));
#34430=CARTESIAN_POINT('Ctrl Pts',(-0.218159914160189,0.00343075530601885,
-0.00967843203245989));
#34431=CARTESIAN_POINT('Ctrl Pts',(-0.218158229993477,0.00344481455338721,
-0.00968540588559376));
#34432=CARTESIAN_POINT('Ctrl Pts',(-0.218155623561165,0.00346732892055049,
-0.0096964817580923));
#34433=CARTESIAN_POINT('Ctrl Pts',(-0.218153017128853,0.00348984328771378,
-0.00970755763059083));
#34434=CARTESIAN_POINT('Ctrl Pts',(-0.218149489538936,0.00352083904218928,
-0.00972268272617012));
#34435=CARTESIAN_POINT('Ctrl Pts',(-0.218145698752299,0.00355603855260194,
-0.00973953220309792));
#34436=CARTESIAN_POINT('Ctrl Pts',(-0.218138117179025,0.00362643757342724,
-0.00977323115695354));
#34437=CARTESIAN_POINT('Ctrl Pts',(-0.218129480285224,0.00371359685156356,
-0.00981394704659143));
#34438=CARTESIAN_POINT('Ctrl Pts',(-0.218120327490645,0.00382045082663618,
-0.0098609864964249));
#34439=CARTESIAN_POINT('Ctrl Pts',(-0.218111430575817,0.0039243175426439,
-0.00990671088967925));
#34440=CARTESIAN_POINT('Ctrl Pts',(-0.218102045208114,0.00404676564641263,
-0.00995845054893569));
#34441=CARTESIAN_POINT('Ctrl Pts',(-0.218093488760285,0.00419254916904724,
-0.0100150756804606));
#34442=CARTESIAN_POINT('Ctrl Pts',(-0.218093242672536,0.00419674197658215,
-0.0100167042477625));
#34443=CARTESIAN_POINT('Ctrl Pts',(-0.218092997270442,0.00420095411548004,
-0.0100183367377336));
#34444=CARTESIAN_POINT('Ctrl Pts',(-0.218092752585342,0.00420518570318234,
-0.0100199731032982));
#34445=CARTESIAN_POINT('Ctrl Pts',(-0.218088376403874,0.00428086744973251,
-0.0100492394242707));
#34446=CARTESIAN_POINT('Ctrl Pts',(-0.218084231623577,0.00436280105608194,
-0.0100796894394523));
#34447=CARTESIAN_POINT('Ctrl Pts',(-0.218080684506125,0.00444451868101746,
-0.0101086817016788));
#34448=CARTESIAN_POINT('Ctrl Pts',(-0.218078910947399,0.00448537749348523,
-0.0101231778327921));
#34449=CARTESIAN_POINT('Ctrl Pts',(-0.218077285414237,0.00452615834643487,
-0.0101373736765752));
#34450=CARTESIAN_POINT('Ctrl Pts',(-0.218075624279617,0.00457624654385498,
-0.0101542910449909));
#34451=CARTESIAN_POINT('Ctrl Pts',(-0.218073963144998,0.0046263347412751,
-0.0101712084134067));
#34452=CARTESIAN_POINT('Ctrl Pts',(-0.218072272056151,0.00468581839975855,
-0.0101905884528484));
#34453=CARTESIAN_POINT('Ctrl Pts',(-0.218071447583993,0.00471612569496449,
-0.0102002835390278));
#34454=CARTESIAN_POINT('Ctrl Pts',(-0.218070623111836,0.00474643299017044,
-0.0102099786252072));
#34455=CARTESIAN_POINT('Ctrl Pts',(-0.218070659325998,0.00474747926921614,
-0.0102102591521145));
#34456=CARTESIAN_POINT('Ctrl Pts',(-0.218070464943007,0.0047579619995227,
-0.0102135587519226));
#34457=CARTESIAN_POINT('Ctrl Pts',(-0.218070270560016,0.00476844472982926,
-0.0102168583517308));
#34458=CARTESIAN_POINT('Ctrl Pts',(-0.218069847248265,0.00478838736452002,
-0.0102231010164984));
#34459=CARTESIAN_POINT('Ctrl Pts',(-0.218069478328105,0.00480837573778782,
-0.0102292653606357));
#34460=CARTESIAN_POINT('Ctrl Pts',(-0.218068740487783,0.00484835248432341,
-0.0102415940489103));
#34461=CARTESIAN_POINT('Ctrl Pts',(-0.218068218029874,0.00488848284454727,
-0.010253708712889));
#34462=CARTESIAN_POINT('Ctrl Pts',(-0.218067808892948,0.00493538064483942,
-0.0102674371328632));
#34463=CARTESIAN_POINT('Ctrl Pts',(-0.218067533740465,0.00496692032110471,
-0.0102766697603835));
#34464=CARTESIAN_POINT('Ctrl Pts',(-0.218067310047023,0.00500152274259813,
-0.0102866230349954));
#34465=CARTESIAN_POINT('Ctrl Pts',(-0.218067226304046,0.00503956785288683,
-0.0102972720892691));
#34466=CARTESIAN_POINT('Ctrl Pts',(-0.218376761434817,0.00221897027385242,
-0.00895460279999876));
#34467=CARTESIAN_POINT('Ctrl Pts',(-0.218355952991769,0.00231749375230912,
-0.00902431860700982));
#34468=CARTESIAN_POINT('Ctrl Pts',(-0.218334517744941,0.00242125175277667,
-0.00909488120513588));
#34469=CARTESIAN_POINT('Ctrl Pts',(-0.218312034443821,0.00253513217699072,
-0.00916849870701569));
#34470=CARTESIAN_POINT('Ctrl Pts',(-0.21830047926189,0.00259366046041081,
-0.00920633405970635));
#34471=CARTESIAN_POINT('Ctrl Pts',(-0.218288648360434,0.00265490126580173,
-0.00924491974098864));
#34472=CARTESIAN_POINT('Ctrl Pts',(-0.218277484656516,0.00271395923175535,
-0.00928118760704619));
#34473=CARTESIAN_POINT('Ctrl Pts',(-0.218271902804557,0.00274348821473217,
-0.00929932154007497));
#34474=CARTESIAN_POINT('Ctrl Pts',(-0.218266487013573,0.00277244827579136,
-0.0093169127990102));
#34475=CARTESIAN_POINT('Ctrl Pts',(-0.218260030845217,0.00280768393378573,
-0.00933797457472041));
#34476=CARTESIAN_POINT('Ctrl Pts',(-0.218253574676861,0.00284291959178011,
-0.00935903635043062));
#34477=CARTESIAN_POINT('Ctrl Pts',(-0.218246081021776,0.00288451657071139,
-0.00938342616520849));
#34478=CARTESIAN_POINT('Ctrl Pts',(-0.218242518753658,0.00290434037807777,
-0.00939494737615413));
#34479=CARTESIAN_POINT('Ctrl Pts',(-0.218240737619598,0.00291425228176096,
-0.00940070798162694));
#34480=CARTESIAN_POINT('Ctrl Pts',(-0.218239938766018,0.00291870490466656,
-0.00940327911467706));
#34481=CARTESIAN_POINT('Ctrl Pts',(-0.218239365786335,0.00292191358914088,
-0.00940513443333053));
#34482=CARTESIAN_POINT('',(-0.216308829828652,0.00249826452155856,-0.00910474619664736));
#34483=CARTESIAN_POINT('',(-0.21509802079524,0.00254314437078809,-0.00910972203361875));
#34484=CARTESIAN_POINT('',(-0.215098016915191,0.0025432095719676,-0.00910961934179909));
#34485=CARTESIAN_POINT('',(-0.21499263029402,0.00750051042987691,-0.0105666547348202));
#34486=CARTESIAN_POINT('Ctrl Pts',(-0.215098014875374,0.00254314350555366,
-0.00910972191547035));
#34487=CARTESIAN_POINT('Ctrl Pts',(-0.215078880714392,0.00266192639885594,
-0.00918587769076132));
#34488=CARTESIAN_POINT('Ctrl Pts',(-0.215054137693622,0.00281927250189698,
-0.00928133661873205));
#34489=CARTESIAN_POINT('Ctrl Pts',(-0.215026681725501,0.00300083501512849,
-0.0093849589510143));
#34490=CARTESIAN_POINT('Ctrl Pts',(-0.215013620542869,0.00308864591147306,
-0.00943387030120433));
#34491=CARTESIAN_POINT('Ctrl Pts',(-0.214989036432337,0.0032621192389327,
-0.00952675263777239));
#34492=CARTESIAN_POINT('Ctrl Pts',(-0.214963579756326,0.00345572023067802,
-0.00962485021407883));
#34493=CARTESIAN_POINT('Ctrl Pts',(-0.214925234692333,0.00377343520887324,
-0.00977659470988523));
#34494=CARTESIAN_POINT('Ctrl Pts',(-0.214881440536056,0.00428400451155548,
-0.00998993632116904));
#34495=CARTESIAN_POINT('Ctrl Pts',(-0.214860207112644,0.0049215028701946,
-0.0102002226568554));
#34496=CARTESIAN_POINT('Ctrl Pts',(-0.214864229236519,0.0054097933709423,
-0.0103262195562019));
#34497=CARTESIAN_POINT('Ctrl Pts',(-0.214877231587741,0.00579919116479696,
-0.0104053314765542));
#34498=CARTESIAN_POINT('Ctrl Pts',(-0.2148871035798,0.00601821428182061,
-0.0104437537652626));
#34499=CARTESIAN_POINT('Ctrl Pts',(-0.214897480943101,0.00621158765416454,
-0.010473381553683));
#34500=CARTESIAN_POINT('Ctrl Pts',(-0.214903550546303,0.00631154295636838,
-0.0104869694861788));
#34501=CARTESIAN_POINT('Ctrl Pts',(-0.214915416994173,0.00649705465937709,
-0.01051040061382));
#34502=CARTESIAN_POINT('Ctrl Pts',(-0.214939982118418,0.00684552155670783,
-0.0105460281812664));
#34503=CARTESIAN_POINT('Ctrl Pts',(-0.21496945372088,0.00722074018422242,
-0.0105661467154913));
#34504=CARTESIAN_POINT('Ctrl Pts',(-0.21499263029402,0.00750051042987691,
-0.0105666547348202));
#34505=CARTESIAN_POINT('',(-0.215095414441432,0.0124591460413101,-0.00910819331956975));
#34506=CARTESIAN_POINT('Ctrl Pts',(-0.214992630415778,0.00750051189965118,
-0.010566654737489));
#34507=CARTESIAN_POINT('Ctrl Pts',(-0.214969342612911,0.00778055055796294,
-0.0105661125628055));
#34508=CARTESIAN_POINT('Ctrl Pts',(-0.214939714956889,0.00815615289366023,
-0.0105459126315921));
#34509=CARTESIAN_POINT('Ctrl Pts',(-0.214914988096678,0.00850509262545842,
-0.0105101549770463));
#34510=CARTESIAN_POINT('Ctrl Pts',(-0.214903033354419,0.00869081285498103,
-0.0104866497375707));
#34511=CARTESIAN_POINT('Ctrl Pts',(-0.214896904227771,0.00879108378126653,
-0.0104729875780705));
#34512=CARTESIAN_POINT('Ctrl Pts',(-0.214886455051281,0.00898415541890412,
-0.0104433475154732));
#34513=CARTESIAN_POINT('Ctrl Pts',(-0.214876476790143,0.00920293166221906,
-0.0104049125080223));
#34514=CARTESIAN_POINT('Ctrl Pts',(-0.214863260859888,0.00959187816631272,
-0.0103257769396539));
#34515=CARTESIAN_POINT('Ctrl Pts',(-0.214858821715445,0.0100779610425055,
-0.0102003615124657));
#34516=CARTESIAN_POINT('Ctrl Pts',(-0.214879534188101,0.0107186135739898,
-0.00998899566147673));
#34517=CARTESIAN_POINT('Ctrl Pts',(-0.214923072812692,0.0112295676181993,
-0.00977519129368386));
#34518=CARTESIAN_POINT('Ctrl Pts',(-0.214961205141803,0.0115466288585745,
-0.0096236389989249));
#34519=CARTESIAN_POINT('Ctrl Pts',(-0.214986555872579,0.0117399447159114,
-0.00952561889921954));
#34520=CARTESIAN_POINT('Ctrl Pts',(-0.215011037359278,0.0119130572004991,
-0.00943287805535147));
#34521=CARTESIAN_POINT('Ctrl Pts',(-0.215024090110732,0.0120009612740028,
-0.0093838919409602));
#34522=CARTESIAN_POINT('Ctrl Pts',(-0.215051519974409,0.0121826213746208,
-0.00928015774996104));
#34523=CARTESIAN_POINT('Ctrl Pts',(-0.215076266198542,0.0123401831812057,
-0.00918451547138759));
#34524=CARTESIAN_POINT('Ctrl Pts',(-0.215095408231139,0.0124591472231019,
-0.00910819364212774));
#34525=CARTESIAN_POINT('',(-0.216305506198624,0.0125054790081327,-0.00910194677041158));
#34526=CARTESIAN_POINT('',(-0.216305506198628,0.0125054790081358,-0.00910194677040962));
#34527=CARTESIAN_POINT('',(-0.21606291203367,0.0101163502415278,-0.0102080466013605));
#34528=CARTESIAN_POINT('Ctrl Pts',(-0.216305504030195,0.0125055507042171,
-0.00910205625925057));
#34529=CARTESIAN_POINT('Ctrl Pts',(-0.216285573012244,0.0123847852099932,
-0.00918076999389213));
#34530=CARTESIAN_POINT('Ctrl Pts',(-0.216268459633762,0.0122785427758774,
-0.00924611596648593));
#34531=CARTESIAN_POINT('Ctrl Pts',(-0.216253300799397,0.0121823096002432,
-0.00930328007396658));
#34532=CARTESIAN_POINT('Ctrl Pts',(-0.216245721382214,0.0121341930124262,
-0.0093318621277069));
#34533=CARTESIAN_POINT('Ctrl Pts',(-0.21623863170164,0.0120885445419686,
-0.00935834388998212));
#34534=CARTESIAN_POINT('Ctrl Pts',(-0.216232891551287,0.012051317695906,
-0.00937963114515802));
#34535=CARTESIAN_POINT('Ctrl Pts',(-0.216227151400934,0.0120140908498435,
-0.00940091840033392));
#34536=CARTESIAN_POINT('Ctrl Pts',(-0.216222758129353,0.0119853611814783,
-0.00941714121196255));
#34537=CARTESIAN_POINT('Ctrl Pts',(-0.216216277214704,0.0119417188391278,
-0.00944131001650295));
#34538=CARTESIAN_POINT('Ctrl Pts',(-0.216209796300054,0.0118980764967773,
-0.00946547882104336));
#34539=CARTESIAN_POINT('Ctrl Pts',(-0.216201232533199,0.0118393910761824,
-0.00949736036638175));
#34540=CARTESIAN_POINT('Ctrl Pts',(-0.216193646182268,0.0117856311521386,
-0.00952578762890845));
#34541=CARTESIAN_POINT('Ctrl Pts',(-0.216186059831338,0.0117318712280949,
-0.00955421489143515));
#34542=CARTESIAN_POINT('Ctrl Pts',(-0.216179447590711,0.0116831194740222,
-0.00957934676861737));
#34543=CARTESIAN_POINT('Ctrl Pts',(-0.216173143906361,0.0116354147837649,
-0.00960345893009553));
#34544=CARTESIAN_POINT('Ctrl Pts',(-0.216160536537661,0.0115400054032504,
-0.00965168325305186));
#34545=CARTESIAN_POINT('Ctrl Pts',(-0.216149163753679,0.011448784674882,
-0.0096958139505624));
#34546=CARTESIAN_POINT('Ctrl Pts',(-0.216138525624132,0.0113536345020631,
-0.0097399040558179));
#34547=CARTESIAN_POINT('Ctrl Pts',(-0.216119015322928,0.0111791293390033,
-0.00982076519121042));
#34548=CARTESIAN_POINT('Ctrl Pts',(-0.216101987621509,0.0109911688732712,
-0.00990098102958284));
#34549=CARTESIAN_POINT('Ctrl Pts',(-0.216089376752195,0.0107988963082568,
-0.00997514789234148));
#34550=CARTESIAN_POINT('Ctrl Pts',(-0.216088235290362,0.0107814929247929,
-0.00998186104121329));
#34551=CARTESIAN_POINT('Ctrl Pts',(-0.216087130014783,0.010764054992567,
-0.0099885262252447));
#34552=CARTESIAN_POINT('Ctrl Pts',(-0.216086062359817,0.0107465897968397,
-0.00999514054140734));
#34553=CARTESIAN_POINT('Ctrl Pts',(-0.216073208630083,0.0105363225168689,
-0.0100747717284893));
#34554=CARTESIAN_POINT('Ctrl Pts',(-0.216065806914254,0.0103219438699067,
-0.0101467674241031));
#34555=CARTESIAN_POINT('Ctrl Pts',(-0.21606291203367,0.0101163502415278,
-0.0102080466013605));
#34556=CARTESIAN_POINT('',(-0.216192971496085,0.00750084397878958,-0.0105937835194403));
#34557=CARTESIAN_POINT('Ctrl Pts',(-0.216062905705723,0.0101159003354215,
-0.0102081806868227));
#34558=CARTESIAN_POINT('Ctrl Pts',(-0.216060015292875,0.00991016956652308,
-0.0102694889169385));
#34559=CARTESIAN_POINT('Ctrl Pts',(-0.216061617126363,0.00971354178683412,
-0.0103209970309253));
#34560=CARTESIAN_POINT('Ctrl Pts',(-0.21606719175661,0.00949795270790532,
-0.0103693828238878));
#34561=CARTESIAN_POINT('Ctrl Pts',(-0.216069979071733,0.00939015816844091,
-0.0103935757203691));
#34562=CARTESIAN_POINT('Ctrl Pts',(-0.216073764939323,0.00927757116026392,
-0.0104167477640333));
#34563=CARTESIAN_POINT('Ctrl Pts',(-0.21607838814934,0.0091661349877902,
-0.0104375189787289));
#34564=CARTESIAN_POINT('Ctrl Pts',(-0.216080699754349,0.00911041690155334,
-0.0104479045860768));
#34565=CARTESIAN_POINT('Ctrl Pts',(-0.216083219538258,0.00905499630344108,
-0.0104577417300695));
#34566=CARTESIAN_POINT('Ctrl Pts',(-0.216086249687527,0.00899457404370174,
-0.0104678359117436));
#34567=CARTESIAN_POINT('Ctrl Pts',(-0.216089279836797,0.0089341517839624,
-0.0104779300934177));
#34568=CARTESIAN_POINT('Ctrl Pts',(-0.216092824138265,0.00886869900919264,
-0.010488112205039));
#34569=CARTESIAN_POINT('Ctrl Pts',(-0.216095620120263,0.00881928313990659,
-0.0104953976695696));
#34570=CARTESIAN_POINT('Ctrl Pts',(-0.216098416102261,0.00876986727062052,
-0.0105026831341002));
#34571=CARTESIAN_POINT('Ctrl Pts',(-0.21610045846058,0.00873652214479988,
-0.0105073081857298));
#34572=CARTESIAN_POINT('Ctrl Pts',(-0.216102985135538,0.00869646623545131,
-0.0105126682511252));
#34573=CARTESIAN_POINT('Ctrl Pts',(-0.216105511810496,0.00865641032610275,
-0.0105180283165205));
#34574=CARTESIAN_POINT('Ctrl Pts',(-0.21610852564855,0.0086096276180213,
-0.0105239968074858));
#34575=CARTESIAN_POINT('Ctrl Pts',(-0.216111722711867,0.00856168836907106,
-0.0105296950506111));
#34576=CARTESIAN_POINT('Ctrl Pts',(-0.216118116838502,0.00846580987117058,
-0.0105410915368618));
#34577=CARTESIAN_POINT('Ctrl Pts',(-0.216125240347082,0.00836532088670505,
-0.010551563202669));
#34578=CARTESIAN_POINT('Ctrl Pts',(-0.216133315547689,0.00825611658081511,
-0.0105608620487624));
#34579=CARTESIAN_POINT('Ctrl Pts',(-0.216149465933751,0.00803770817395129,
-0.0105794597235006));
#34580=CARTESIAN_POINT('Ctrl Pts',(-0.21616942628362,0.00778443696992211,
-0.0105932247541572));
#34581=CARTESIAN_POINT('Ctrl Pts',(-0.216192971885712,0.00750084401094905,
-0.0105937834231419));
#34582=CARTESIAN_POINT('',(-0.216064562234792,0.00488811599144484,-0.0102094142070321));
#34583=CARTESIAN_POINT('Ctrl Pts',(-0.216192971951985,0.00750084321272765,
-0.0105937834247143));
#34584=CARTESIAN_POINT('Ctrl Pts',(-0.216169508654091,0.00721699231932673,
-0.0105932796528161));
#34585=CARTESIAN_POINT('Ctrl Pts',(-0.216149636727297,0.0069635594796243,
-0.010579541065668));
#34586=CARTESIAN_POINT('Ctrl Pts',(-0.216133576495944,0.00674505389894682,
-0.0105609655730863));
#34587=CARTESIAN_POINT('Ctrl Pts',(-0.216125546380267,0.00663580110860809,
-0.0105516778267954));
#34588=CARTESIAN_POINT('Ctrl Pts',(-0.216118468404311,0.00653527978127621,
-0.0105412154642067));
#34589=CARTESIAN_POINT('Ctrl Pts',(-0.216112124596152,0.00643941830546403,
-0.0105298339080441));
#34590=CARTESIAN_POINT('Ctrl Pts',(-0.216108952692073,0.00639148756755795,
-0.0105241431299627));
#34591=CARTESIAN_POINT('Ctrl Pts',(-0.216105965202961,0.00634472567739711,
-0.0105181838109217));
#34592=CARTESIAN_POINT('Ctrl Pts',(-0.216103460103315,0.00630465700703719,
-0.0105128275687491));
#34593=CARTESIAN_POINT('Ctrl Pts',(-0.216100955003668,0.00626458833667726,
-0.0105074713265765));
#34594=CARTESIAN_POINT('Ctrl Pts',(-0.216098929471675,0.00623119702191735,
-0.0105028436523896));
#34595=CARTESIAN_POINT('Ctrl Pts',(-0.216096169915181,0.00618188883829889,
-0.0104955812314442));
#34596=CARTESIAN_POINT('Ctrl Pts',(-0.216093410358688,0.00613258065468043,
-0.0104883188104988));
#34597=CARTESIAN_POINT('Ctrl Pts',(-0.216089922022156,0.00606738903619435,
-0.0104781880715125));
#34598=CARTESIAN_POINT('Ctrl Pts',(-0.216086942406758,0.00600717401362571,
-0.0104681413248275));
#34599=CARTESIAN_POINT('Ctrl Pts',(-0.216083962791361,0.00594695899105708,
-0.0104580945781425));
#34600=CARTESIAN_POINT('Ctrl Pts',(-0.216081488159746,0.00589169212150471,
-0.010448298718238));
#34601=CARTESIAN_POINT('Ctrl Pts',(-0.216079222483585,0.00583612546404543,
-0.0104379565789868));
#34602=CARTESIAN_POINT('Ctrl Pts',(-0.216074691131264,0.00572499214912688,
-0.0104172723004846));
#34603=CARTESIAN_POINT('Ctrl Pts',(-0.21607100017286,0.00561269828959701,
-0.0103941983821629));
#34604=CARTESIAN_POINT('Ctrl Pts',(-0.216068305392988,0.00550514230539665,
-0.01037009988483));
#34605=CARTESIAN_POINT('Ctrl Pts',(-0.216062915833244,0.00529003033699593,
-0.0103219028901643));
#34606=CARTESIAN_POINT('Ctrl Pts',(-0.21606148974563,0.00509366268594511,
-0.010270561045398));
#34607=CARTESIAN_POINT('Ctrl Pts',(-0.216064562234792,0.00488811599144484,
-0.0102094142070321));
#34608=CARTESIAN_POINT('Ctrl Pts',(-0.216064562234792,0.00488811599144484,
-0.0102094142070321));
#34609=CARTESIAN_POINT('Ctrl Pts',(-0.216067634723955,0.00468256929694457,
-0.0101482673686662));
#34610=CARTESIAN_POINT('Ctrl Pts',(-0.21607522582377,0.00446813446215115,
-0.0100764011159303));
#34611=CARTESIAN_POINT('Ctrl Pts',(-0.216088338924692,0.00425716728514312,
-0.00999661661287887));
#34612=CARTESIAN_POINT('Ctrl Pts',(-0.216089502570561,0.00423844623011241,
-0.00998953660122299));
#34613=CARTESIAN_POINT('Ctrl Pts',(-0.216090709717795,0.00421975125104769,
-0.00998239617590539));
#34614=CARTESIAN_POINT('Ctrl Pts',(-0.21609195844297,0.00420109267159996,
-0.00997519932710212));
#34615=CARTESIAN_POINT('Ctrl Pts',(-0.216104781575639,0.00400948811007565,
-0.0099012950374873));
#34616=CARTESIAN_POINT('Ctrl Pts',(-0.216121989182533,0.00382182884714497,
-0.00982121910009571));
#34617=CARTESIAN_POINT('Ctrl Pts',(-0.216141498420156,0.00364853401298664,
-0.00974097652987249));
#34618=CARTESIAN_POINT('Ctrl Pts',(-0.216152202950225,0.00355344881288889,
-0.00969694820737177));
#34619=CARTESIAN_POINT('Ctrl Pts',(-0.216163596637211,0.00346261072515542,
-0.00965303427445999));
#34620=CARTESIAN_POINT('Ctrl Pts',(-0.216176231034628,0.00336745049549093,
-0.00960497891364581));
#34621=CARTESIAN_POINT('Ctrl Pts',(-0.216182548233336,0.00331987038065869,
-0.00958095123323872));
#34622=CARTESIAN_POINT('Ctrl Pts',(-0.21618917555074,0.0032712106596776,
-0.00955589038338166));
#34623=CARTESIAN_POINT('Ctrl Pts',(-0.216196774500355,0.0032175566238911,
-0.00952754662918728));
#34624=CARTESIAN_POINT('Ctrl Pts',(-0.21620437344997,0.0031639025881046,
-0.0094992028749929));
#34625=CARTESIAN_POINT('Ctrl Pts',(-0.21621294731804,0.00310533630168092,
-0.00946741828469016));
#34626=CARTESIAN_POINT('Ctrl Pts',(-0.216219436071743,0.00306177318974593,
-0.00944331847681517));
#34627=CARTESIAN_POINT('Ctrl Pts',(-0.216225924825445,0.00301821007781095,
-0.00941921866894019));
#34628=CARTESIAN_POINT('Ctrl Pts',(-0.216230323693065,0.00298952042971264,
-0.00940303591356076));
#34629=CARTESIAN_POINT('Ctrl Pts',(-0.216236072810317,0.00295233499613605,
-0.00938179523158231));
#34630=CARTESIAN_POINT('Ctrl Pts',(-0.21624182192757,0.00291514956255945,
-0.00936055454960386));
#34631=CARTESIAN_POINT('Ctrl Pts',(-0.216248923937414,0.00286954355307472,
-0.009334126324145));
#34632=CARTESIAN_POINT('Ctrl Pts',(-0.216256517647776,0.00282146039342472,
-0.00930559553315848));
#34633=CARTESIAN_POINT('Ctrl Pts',(-0.216271705068501,0.00272529407412471,
-0.00924853395118545));
#34634=CARTESIAN_POINT('Ctrl Pts',(-0.216288854896236,0.00261908279258283,
-0.0091832809841745));
#34635=CARTESIAN_POINT('Ctrl Pts',(-0.216308831619352,0.00249832230384034,
-0.0091046579272641));
#34636=CARTESIAN_POINT('',(-0.191002128727803,0.00750279694962982,-0.0100254048439417));
#34637=CARTESIAN_POINT('',(-0.190954131521021,0.0114757689203866,-0.00915712253688136));
#34638=CARTESIAN_POINT('Ctrl Pts',(-0.190954094375179,0.0114755956741647,
-0.00915648079316597));
#34639=CARTESIAN_POINT('Ctrl Pts',(-0.190949712020098,0.0114114603137452,
-0.00918577312088179));
#34640=CARTESIAN_POINT('Ctrl Pts',(-0.190945071320235,0.0113437322707912,
-0.00921585170663403));
#34641=CARTESIAN_POINT('Ctrl Pts',(-0.190940278164648,0.0112720433793392,
-0.00924659321808342));
#34642=CARTESIAN_POINT('Ctrl Pts',(-0.190935484712584,0.0112003500536294,
-0.00927733663102393));
#34643=CARTESIAN_POINT('Ctrl Pts',(-0.190930538969924,0.0111246908651552,
-0.00930873403932449));
#34644=CARTESIAN_POINT('Ctrl Pts',(-0.190925612592709,0.0110457932672867,
-0.00934019431223972));
#34645=CARTESIAN_POINT('Ctrl Pts',(-0.190920686215494,0.0109668956694181,
-0.00937165458515496));
#34646=CARTESIAN_POINT('Ctrl Pts',(-0.190915778457101,0.0108847753427232,
-0.00940321350242323));
#34647=CARTESIAN_POINT('Ctrl Pts',(-0.190910892877424,0.0107962805502497,
-0.00943565448019979));
#34648=CARTESIAN_POINT('Ctrl Pts',(-0.190908982581279,0.0107616784616149,
-0.00944833913154536));
#34649=CARTESIAN_POINT('Ctrl Pts',(-0.19090707603451,0.0107260969951283,
-0.00946114643072369));
#34650=CARTESIAN_POINT('Ctrl Pts',(-0.190905267900651,0.0106913983121456,
-0.00947340659224363));
#34651=CARTESIAN_POINT('Ctrl Pts',(-0.190904763884623,0.0106817260789378,
-0.0094768241035493));
#34652=CARTESIAN_POINT('Ctrl Pts',(-0.190904267515394,0.0106721226257211,
-0.00948019962700674));
#34653=CARTESIAN_POINT('Ctrl Pts',(-0.190903780843293,0.0106626287092986,
-0.00948351987320058));
#34654=CARTESIAN_POINT('Ctrl Pts',(-0.190902664550575,0.0106408522611478,
-0.00949113561004409));
#34655=CARTESIAN_POINT('Ctrl Pts',(-0.190901598866219,0.010619657350123,
-0.0094984750067754));
#34656=CARTESIAN_POINT('Ctrl Pts',(-0.190900336275497,0.0105935509108808,
-0.00950738083319582));
#34657=CARTESIAN_POINT('Ctrl Pts',(-0.190899073684775,0.0105674444716387,
-0.00951628665961624));
#34658=CARTESIAN_POINT('Ctrl Pts',(-0.190897615764644,0.0105364013707763,
-0.00952668559938698));
#34659=CARTESIAN_POINT('Ctrl Pts',(-0.190896985542716,0.0105229623294542,
-0.00953115285039524));
#34660=CARTESIAN_POINT('Ctrl Pts',(-0.190896670431751,0.0105162428087932,
-0.00953338647589937));
#34661=CARTESIAN_POINT('Ctrl Pts',(-0.190896561953082,0.0105139287668234,
-0.00953415071739028));
#34662=CARTESIAN_POINT('Ctrl Pts',(-0.190896511796388,0.0105128545877792,
-0.00953450644811207));
#34663=CARTESIAN_POINT('Ctrl Pts',(-0.190896486718041,0.0105123174982571,
-0.00953468431347296));
#34664=CARTESIAN_POINT('Ctrl Pts',(-0.190896476230896,0.010512090212176,
-0.00953475955545459));
#34665=CARTESIAN_POINT('Ctrl Pts',(-0.19089646182634,0.0105117765703442,
-0.00953486338619688));
#34666=CARTESIAN_POINT('Ctrl Pts',(-0.190896447421783,0.0105114629285123,
-0.00953496721693918));
#34667=CARTESIAN_POINT('Ctrl Pts',(-0.190896429099489,0.0105110629359991,
-0.00953509965162892));
#34668=CARTESIAN_POINT('Ctrl Pts',(-0.19089638835623,0.0105101803497181,
-0.00953539165248889));
#34669=CARTESIAN_POINT('Ctrl Pts',(-0.190896225383196,0.0105066500045945,
-0.00953655965592877));
#34670=CARTESIAN_POINT('Ctrl Pts',(-0.190895703714802,0.0104953975208178,
-0.00954027885553927));
#34671=CARTESIAN_POINT('Ctrl Pts',(-0.190895127071901,0.0104827302132629,
-0.00954442716706281));
#34672=CARTESIAN_POINT('Ctrl Pts',(-0.190893973786097,0.0104573955981532,
-0.00955272379010988));
#34673=CARTESIAN_POINT('Ctrl Pts',(-0.19089259953884,0.0104264180483005,
-0.00956278615109603));
#34674=CARTESIAN_POINT('Ctrl Pts',(-0.190890902985786,0.0103836168892928,
-0.00957629011243121));
#34675=CARTESIAN_POINT('Ctrl Pts',(-0.190889206432731,0.010340815730285,
-0.0095897940737664));
#34676=CARTESIAN_POINT('Ctrl Pts',(-0.190887188717151,0.0102861734770876,
-0.00960668668092587));
#34677=CARTESIAN_POINT('Ctrl Pts',(-0.190885238302781,0.0102249868586566,
-0.00962483435560046));
#34678=CARTESIAN_POINT('Ctrl Pts',(-0.190884263095595,0.0101943935494411,
-0.00963390819293776));
#34679=CARTESIAN_POINT('Ctrl Pts',(-0.190883304145586,0.0101621723310017,
-0.00964332198835475));
#34680=CARTESIAN_POINT('Ctrl Pts',(-0.190882305478128,0.010123072861922,
-0.00965445185984557));
#34681=CARTESIAN_POINT('Ctrl Pts',(-0.190881306810671,0.0100839733928422,
-0.0096655817313364));
#34682=CARTESIAN_POINT('Ctrl Pts',(-0.190880270863819,0.0100379635616817,
-0.00967831595867959));
#34683=CARTESIAN_POINT('Ctrl Pts',(-0.190879609294718,0.0100059172322142,
-0.00968700170894241));
#34684=CARTESIAN_POINT('Ctrl Pts',(-0.190878947725618,0.00997387090274672,
-0.00969568745920523));
#34685=CARTESIAN_POINT('Ctrl Pts',(-0.190878657565483,0.00995582424085349,
-0.00970046013451214));
#34686=CARTESIAN_POINT('Ctrl Pts',(-0.190878343369803,0.00993486250300072,
-0.00970597129447378));
#34687=CARTESIAN_POINT('Ctrl Pts',(-0.190878029174123,0.00991390076514795,
-0.00971148245443542));
#34688=CARTESIAN_POINT('Ctrl Pts',(-0.190877692134822,0.00989001008289119,
-0.00971767787286489));
#34689=CARTESIAN_POINT('Ctrl Pts',(-0.190877422907681,0.0098672072748013,
-0.00972349682048002));
#34690=CARTESIAN_POINT('Ctrl Pts',(-0.1908768844534,0.00982160165862154,
-0.00973513471571027));
#34691=CARTESIAN_POINT('Ctrl Pts',(-0.190876616187465,0.00978035869652348,
-0.00974531472603288));
#34692=CARTESIAN_POINT('Ctrl Pts',(-0.190876473111491,0.00974219455184456,
-0.00975451522161448));
#34693=CARTESIAN_POINT('Ctrl Pts',(-0.190876330035517,0.00970403040716564,
-0.00976371571719607));
#34694=CARTESIAN_POINT('Ctrl Pts',(-0.190876311814032,0.00966894964395492,
-0.00977195208813503));
#34695=CARTESIAN_POINT('Ctrl Pts',(-0.190876488385096,0.00963105439853278,
-0.00978061835509751));
#34696=CARTESIAN_POINT('Ctrl Pts',(-0.190876664956159,0.00959315915311064,
-0.00978928462205999));
#34697=CARTESIAN_POINT('Ctrl Pts',(-0.19087703863711,0.00955242519301168,
-0.00979827588427239));
#34698=CARTESIAN_POINT('Ctrl Pts',(-0.190877227802085,0.00953392878073028,
-0.00980230657795196));
#34699=CARTESIAN_POINT('Ctrl Pts',(-0.190877322384573,0.00952468057458957,
-0.00980432192479174));
#34700=CARTESIAN_POINT('Ctrl Pts',(-0.190877370417995,0.00952099580690186,
-0.00980511608364548));
#34701=CARTESIAN_POINT('Ctrl Pts',(-0.190877416245437,0.00951868580370159,
-0.00980561603274182));
#34702=CARTESIAN_POINT('Ctrl Pts',(-0.190877462072879,0.00951637580050133,
-0.00980611598183816));
#34703=CARTESIAN_POINT('Ctrl Pts',(-0.190877505748922,0.009515440046279,
-0.00980631926023749));
#34704=CARTESIAN_POINT('Ctrl Pts',(-0.190877592138407,0.00951168488289209,
-0.00980712931189838));
#34705=CARTESIAN_POINT('Ctrl Pts',(-0.190877764917375,0.00950417455611826,
-0.00980874941522017));
#34706=CARTESIAN_POINT('Ctrl Pts',(-0.190878108686614,0.00948538517546544,
-0.00981279043480945));
#34707=CARTESIAN_POINT('Ctrl Pts',(-0.190878570724653,0.00946280542795435,
-0.00981753707052625));
#34708=CARTESIAN_POINT('Ctrl Pts',(-0.190879494800731,0.00941764593293216,
-0.00982703034195985));
#34709=CARTESIAN_POINT('Ctrl Pts',(-0.190880889082616,0.00935735369003375,
-0.00983947571397337));
#34710=CARTESIAN_POINT('Ctrl Pts',(-0.190883526254305,0.00927378471309401,
-0.00985531897787881));
#34711=CARTESIAN_POINT('Ctrl Pts',(-0.190886163425994,0.00919021573615428,
-0.00987116224178425));
#34712=CARTESIAN_POINT('Ctrl Pts',(-0.190890046919921,0.00908333562718222,
-0.0098902484430308));
#34713=CARTESIAN_POINT('Ctrl Pts',(-0.19089556723871,0.00896203269271428,
-0.00990916826768047));
#34714=CARTESIAN_POINT('Ctrl Pts',(-0.190898327398105,0.00890138122548031,
-0.00991862818000531));
#34715=CARTESIAN_POINT('Ctrl Pts',(-0.190901494806612,0.00883714055904416,
-0.00992813433623493));
#34716=CARTESIAN_POINT('Ctrl Pts',(-0.190905913041937,0.00875970557271916,
-0.0099385485861674));
#34717=CARTESIAN_POINT('Ctrl Pts',(-0.190910331277262,0.00868227058639415,
-0.00994896283609988));
#34718=CARTESIAN_POINT('Ctrl Pts',(-0.190916009238766,0.00859158540031464,
-0.0099598880920389));
#34719=CARTESIAN_POINT('Ctrl Pts',(-0.190920299492141,0.00852624126001904,
-0.00996706295173374));
#34720=CARTESIAN_POINT('Ctrl Pts',(-0.190924589745517,0.00846089711972344,
-0.00997423781142858));
#34721=CARTESIAN_POINT('Ctrl Pts',(-0.190927481335499,0.00842094452761956,
-0.0099781492331332));
#34722=CARTESIAN_POINT('Ctrl Pts',(-0.190930754362073,0.00837603777468225,
-0.00998237237824975));
#34723=CARTESIAN_POINT('Ctrl Pts',(-0.190934027388647,0.00833113102174495,
-0.0099865955233663));
#34724=CARTESIAN_POINT('Ctrl Pts',(-0.190937686315205,0.00828125394742464,
-0.00999093235948039));
#34725=CARTESIAN_POINT('Ctrl Pts',(-0.190941295904069,0.00823342278523267,
-0.00999471241801912));
#34726=CARTESIAN_POINT('Ctrl Pts',(-0.190948515081796,0.00813776046084873,
-0.0100022725350966));
#34727=CARTESIAN_POINT('Ctrl Pts',(-0.190955532508425,0.00805029181322841,
-0.010007800356196));
#34728=CARTESIAN_POINT('Ctrl Pts',(-0.190962490680233,0.00796595757437065,
-0.0100121008424296));
#34729=CARTESIAN_POINT('Ctrl Pts',(-0.19097640702385,0.00779728909665514,
-0.010020701814897));
#34730=CARTESIAN_POINT('Ctrl Pts',(-0.190990092174909,0.00764116175118779,
-0.0100241361536859));
#34731=CARTESIAN_POINT('Ctrl Pts',(-0.191002150316979,0.00750280017557725,
-0.0100244496327049));
#34732=CARTESIAN_POINT('',(-0.191550785002591,0.0118950229056552,-0.00896386114240554));
#34733=CARTESIAN_POINT('Ctrl Pts',(-0.190954112929703,0.0114756574972142,
-0.00915645285326651));
#34734=CARTESIAN_POINT('Ctrl Pts',(-0.190982008539415,0.0115054322583542,
-0.00914338889688701));
#34735=CARTESIAN_POINT('Ctrl Pts',(-0.19101287342955,0.0115380979044843,
-0.00912884832062592));
#34736=CARTESIAN_POINT('Ctrl Pts',(-0.191106704839325,0.0116251376084165,
-0.00908978613440817));
#34737=CARTESIAN_POINT('Ctrl Pts',(-0.191229718411826,0.0117176478910505,
-0.00904729586658412));
#34738=CARTESIAN_POINT('Ctrl Pts',(-0.191370919388666,0.0118051770272004,
-0.00900648410289972));
#34739=CARTESIAN_POINT('Ctrl Pts',(-0.191495260460881,0.0118685913453507,
-0.00897644371887849));
#34740=CARTESIAN_POINT('Ctrl Pts',(-0.191550246290606,0.0118947665274591,
-0.00896398319195776));
#34741=CARTESIAN_POINT('',(-0.19224419201362,0.0121632767044805,-0.00883255225498704));
#34742=CARTESIAN_POINT('Ctrl Pts',(-0.191550785002591,0.0118950229056552,
-0.00896386114240554));
#34743=CARTESIAN_POINT('Ctrl Pts',(-0.191605544537764,0.0119210766204984,
-0.00895145795873606));
#34744=CARTESIAN_POINT('Ctrl Pts',(-0.191677122179383,0.0119519839958818,
-0.00893663396839678));
#34745=CARTESIAN_POINT('Ctrl Pts',(-0.19179224763391,0.0119993353150033,
-0.00891377444744784));
#34746=CARTESIAN_POINT('Ctrl Pts',(-0.191909096678037,0.012044435087274,
-0.00889178266758456));
#34747=CARTESIAN_POINT('Ctrl Pts',(-0.191939931439879,0.0120558519308887,
-0.00888617858607348));
#34748=CARTESIAN_POINT('Ctrl Pts',(-0.19204879387273,0.0120964762074764,
-0.00886617854625054));
#34749=CARTESIAN_POINT('Ctrl Pts',(-0.192155333347995,0.0121356773845727,
-0.00884660375394572));
#34750=CARTESIAN_POINT('Ctrl Pts',(-0.192242639246286,0.0121676311322629,
-0.00883037490798918));
#34751=CARTESIAN_POINT('',(-0.192083217793351,0.0103603962460601,-0.00960945776125992));
#34752=CARTESIAN_POINT('Ctrl Pts',(-0.192083217793351,0.0103603962460601,
-0.00960945776125992));
#34753=CARTESIAN_POINT('Ctrl Pts',(-0.192085199140223,0.0104074107317101,
-0.00959475205438907));
#34754=CARTESIAN_POINT('Ctrl Pts',(-0.192087605796192,0.0104586710651692,
-0.00957826631006171));
#34755=CARTESIAN_POINT('Ctrl Pts',(-0.192090621658018,0.0105149888983772,
-0.00955956027685326));
#34756=CARTESIAN_POINT('Ctrl Pts',(-0.19209365489289,0.0105716311537188,
-0.00954074648645924));
#34757=CARTESIAN_POINT('Ctrl Pts',(-0.192097307609679,0.0106333734291636,
-0.00951962630166627));
#34758=CARTESIAN_POINT('Ctrl Pts',(-0.192101334370423,0.0106965037041797,
-0.00949723574375678));
#34759=CARTESIAN_POINT('Ctrl Pts',(-0.192105873419757,0.0107676654768694,
-0.0094719966363405));
#34760=CARTESIAN_POINT('Ctrl Pts',(-0.19211088773952,0.0108405851111344,
-0.00944513150529008));
#34761=CARTESIAN_POINT('Ctrl Pts',(-0.192116025794393,0.0109101028658402,
-0.0094185854425774));
#34762=CARTESIAN_POINT('Ctrl Pts',(-0.192135418226145,0.0111724819853732,
-0.0093183933033018));
#34763=CARTESIAN_POINT('Ctrl Pts',(-0.192156505092465,0.0113871237995003,
-0.00922445471737479));
#34764=CARTESIAN_POINT('Ctrl Pts',(-0.192178577024194,0.0115925865308087,
-0.00912711081785286));
#34765=CARTESIAN_POINT('Ctrl Pts',(-0.192200229318518,0.0117941429503239,
-0.00903161764629643));
#34766=CARTESIAN_POINT('Ctrl Pts',(-0.192222852910695,0.0119862268713765,
-0.00893168204109561));
#34767=CARTESIAN_POINT('Ctrl Pts',(-0.192244557816236,0.0121587843232118,
-0.00883537905873995));
#34768=CARTESIAN_POINT('',(-0.192075076622818,0.00956760145971055,-0.00982142515813679));
#34769=CARTESIAN_POINT('Ctrl Pts',(-0.192075076622818,0.00956760145971055,
-0.00982142515813679));
#34770=CARTESIAN_POINT('Ctrl Pts',(-0.192073708408936,0.00962478404706063,
-0.00980871295728778));
#34771=CARTESIAN_POINT('Ctrl Pts',(-0.192072762001713,0.00967780303936765,
-0.00979636424425594));
#34772=CARTESIAN_POINT('Ctrl Pts',(-0.192072138417696,0.00972752489408203,
-0.00978441260142664));
#34773=CARTESIAN_POINT('Ctrl Pts',(-0.1920711088619,0.00980961715801607,
-0.00976468008293502));
#34774=CARTESIAN_POINT('Ctrl Pts',(-0.192070963831367,0.00988266913471998,
-0.00974582350900616));
#34775=CARTESIAN_POINT('Ctrl Pts',(-0.192071049839845,0.00991534567965813,
-0.0097372756757167));
#34776=CARTESIAN_POINT('Ctrl Pts',(-0.192071092844084,0.00993168395212721,
-0.00973300175907198));
#34777=CARTESIAN_POINT('Ctrl Pts',(-0.192071192640264,0.00993794032390922,
-0.00973134918095328));
#34778=CARTESIAN_POINT('Ctrl Pts',(-0.192071408671919,0.00995217223025025,
-0.0097275694112986));
#34779=CARTESIAN_POINT('Ctrl Pts',(-0.192071624703575,0.00996640413659128,
-0.00972378964164391));
#34780=CARTESIAN_POINT('Ctrl Pts',(-0.192071957564754,0.00998860428775286,
-0.00971785558555461));
#34781=CARTESIAN_POINT('Ctrl Pts',(-0.19207246071673,0.0100145240014813,
-0.00971078580027881));
#34782=CARTESIAN_POINT('Ctrl Pts',(-0.192073467020682,0.010066363428938,
-0.00969664622972721));
#34783=CARTESIAN_POINT('Ctrl Pts',(-0.192075153115435,0.0101331011051023,
-0.00967802702342739));
#34784=CARTESIAN_POINT('Ctrl Pts',(-0.192077829300968,0.0102151293872966,
-0.00965373321717447));
#34785=CARTESIAN_POINT('Ctrl Pts',(-0.19207925462564,0.0102588172904748,
-0.00964079444255896));
#34786=CARTESIAN_POINT('Ctrl Pts',(-0.192080960098135,0.010306848665772,
-0.00962627732697882));
#34787=CARTESIAN_POINT('Ctrl Pts',(-0.192083217793351,0.0103603962460601,
-0.00960945776125992));
#34788=CARTESIAN_POINT('',(-0.192177608446634,0.00780160333064341,-0.010046203453906));
#34789=CARTESIAN_POINT('Ctrl Pts',(-0.192177608446634,0.00780160333064341,
-0.010046203453906));
#34790=CARTESIAN_POINT('Ctrl Pts',(-0.192167966362081,0.00792071951974089,
-0.0100422162115806));
#34791=CARTESIAN_POINT('Ctrl Pts',(-0.192158463911435,0.00804293334057657,
-0.0100358383462041));
#34792=CARTESIAN_POINT('Ctrl Pts',(-0.192149221874634,0.00816902089203289,
-0.0100267146508605));
#34793=CARTESIAN_POINT('Ctrl Pts',(-0.192140658477299,0.00828584987955978,
-0.0100182609052117));
#34794=CARTESIAN_POINT('Ctrl Pts',(-0.192132320993025,0.00840599740158487,
-0.0100073464338714));
#34795=CARTESIAN_POINT('Ctrl Pts',(-0.192124643137378,0.00852403942360911,
-0.00999438297314338));
#34796=CARTESIAN_POINT('Ctrl Pts',(-0.192120804209555,0.00858306043462123,
-0.00998790124277939));
#34797=CARTESIAN_POINT('Ctrl Pts',(-0.192117128736142,0.00864156067840806,
-0.00998097171308127));
#34798=CARTESIAN_POINT('Ctrl Pts',(-0.192113255424149,0.00870685231601164,
-0.00997253562426482));
#34799=CARTESIAN_POINT('Ctrl Pts',(-0.192109382112156,0.00877214395361522,
-0.00996409953544838));
#34800=CARTESIAN_POINT('Ctrl Pts',(-0.192105316501578,0.00884419624784911,
-0.00995391015699222));
#34801=CARTESIAN_POINT('Ctrl Pts',(-0.192102640615622,0.00889274882880993,
-0.0099466716761585));
#34802=CARTESIAN_POINT('Ctrl Pts',(-0.192099964729666,0.00894130140977075,
-0.00993943319532478));
#34803=CARTESIAN_POINT('Ctrl Pts',(-0.192098671392472,0.00896640363023614,
-0.00993546631412305));
#34804=CARTESIAN_POINT('Ctrl Pts',(-0.192096901885914,0.0090014033603828,
-0.00992984074869916));
#34805=CARTESIAN_POINT('Ctrl Pts',(-0.192095132379357,0.00903640309052946,
-0.00992421518327526));
#34806=CARTESIAN_POINT('Ctrl Pts',(-0.192092889846057,0.00908127598741976,
-0.00991679012291164));
#34807=CARTESIAN_POINT('Ctrl Pts',(-0.192090632228416,0.00913068544408291,
-0.0099081590733559));
#34808=CARTESIAN_POINT('Ctrl Pts',(-0.192086116993135,0.00922950435740919,
-0.00989089697424441));
#34809=CARTESIAN_POINT('Ctrl Pts',(-0.192081547517015,0.00934643028253622,
-0.00986853887825808));
#34810=CARTESIAN_POINT('Ctrl Pts',(-0.192078312514945,0.00945039149167174,
-0.00984674944504866));
#34811=CARTESIAN_POINT('Ctrl Pts',(-0.192077036897294,0.00949138520680904,
-0.00983815749209412));
#34812=CARTESIAN_POINT('Ctrl Pts',(-0.19207596737083,0.00953037606040437,
-0.00982971706688361));
#34813=CARTESIAN_POINT('Ctrl Pts',(-0.192075076622818,0.00956760145971055,
-0.00982142515813679));
#34814=CARTESIAN_POINT('',(-0.192202406927022,0.00750306323134365,-0.0100515763887981));
#34815=CARTESIAN_POINT('Ctrl Pts',(-0.192202513508821,0.00750308895613145,
-0.010051578743107));
#34816=CARTESIAN_POINT('Ctrl Pts',(-0.19219416019488,0.00760065611110659,
-0.0100513580199758));
#34817=CARTESIAN_POINT('Ctrl Pts',(-0.192185833516719,0.00770000348444694,
-0.0100496541681167));
#34818=CARTESIAN_POINT('Ctrl Pts',(-0.192177608446634,0.00780160333064341,
-0.010046203453906));
#34819=CARTESIAN_POINT('',(-0.192248325555084,0.00283771562762635,-0.00883349052758685));
#34820=CARTESIAN_POINT('Ctrl Pts',(-0.192202406132311,0.0075030381940905,
-0.0100515763327894));
#34821=CARTESIAN_POINT('Ctrl Pts',(-0.192180243642943,0.00724060161082699,
-0.0100511599388438));
#34822=CARTESIAN_POINT('Ctrl Pts',(-0.192161403564018,0.00700671406050332,
-0.010039924073732));
#34823=CARTESIAN_POINT('Ctrl Pts',(-0.192146104291984,0.00680544197489901,
-0.010024804214849));
#34824=CARTESIAN_POINT('Ctrl Pts',(-0.192138454655968,0.00670480593209685,
-0.0100172442854074));
#34825=CARTESIAN_POINT('Ctrl Pts',(-0.192131689594209,0.00661232353382941,
-0.0100087410484208));
#34826=CARTESIAN_POINT('Ctrl Pts',(-0.192125592592653,0.00652423194571237,
-0.0099995109234971));
#34827=CARTESIAN_POINT('Ctrl Pts',(-0.192122544091875,0.00648018615165385,
-0.00999489586103524));
#34828=CARTESIAN_POINT('Ctrl Pts',(-0.192119663317349,0.00643724085037231,
-0.00999006751205205));
#34829=CARTESIAN_POINT('Ctrl Pts',(-0.192117246548196,0.00640051459612932,
-0.00998573832613764));
#34830=CARTESIAN_POINT('Ctrl Pts',(-0.192114829779043,0.00636378834188632,
-0.00998140914022324));
#34831=CARTESIAN_POINT('Ctrl Pts',(-0.192112874722809,0.00633326978455562,
-0.00997768108228416));
#34832=CARTESIAN_POINT('Ctrl Pts',(-0.192110173707211,0.00628802258600407,
-0.00997180968673719));
#34833=CARTESIAN_POINT('Ctrl Pts',(-0.192107472691613,0.00624277538745251,
-0.00996593829119022));
#34834=CARTESIAN_POINT('Ctrl Pts',(-0.192104029975276,0.00618282343766615,
-0.00995773385839349));
#34835=CARTESIAN_POINT('Ctrl Pts',(-0.192101053261483,0.00612740831063799,
-0.00994959447270961));
#34836=CARTESIAN_POINT('Ctrl Pts',(-0.192098076547689,0.00607199318360983,
-0.00994145508702573));
#34837=CARTESIAN_POINT('Ctrl Pts',(-0.192095562803207,0.00602109455563342,
-0.0099335162360786));
#34838=CARTESIAN_POINT('Ctrl Pts',(-0.192093220004145,0.00596989500140285,
-0.00992513296170256));
#34839=CARTESIAN_POINT('Ctrl Pts',(-0.192088534406023,0.0058674958929417,
-0.00990836641295047));
#34840=CARTESIAN_POINT('Ctrl Pts',(-0.192084536208433,0.005763920479537,
-0.00988966016638157));
#34841=CARTESIAN_POINT('Ctrl Pts',(-0.192081415054645,0.00566425619301311,
-0.00987003838255628));
#34842=CARTESIAN_POINT('Ctrl Pts',(-0.192075172747069,0.00546492761996531,
-0.00983079481490569));
#34843=CARTESIAN_POINT('Ctrl Pts',(-0.192072423513269,0.00528110931116734,
-0.0097885680268741));
#34844=CARTESIAN_POINT('Ctrl Pts',(-0.192073251416343,0.00509090909543717,
-0.00973895831064353));
#34845=CARTESIAN_POINT('Ctrl Pts',(-0.192074079319417,0.00490070887970699,
-0.00968934859441295));
#34846=CARTESIAN_POINT('Ctrl Pts',(-0.192078496030296,0.00470428524458125,
-0.00963182068569001));
#34847=CARTESIAN_POINT('Ctrl Pts',(-0.192087498668996,0.00450687929544704,
-0.00956675209872605));
#34848=CARTESIAN_POINT('Ctrl Pts',(-0.192090597557793,0.0044389282085873,
-0.00954435418607945));
#34849=CARTESIAN_POINT('Ctrl Pts',(-0.192094240798635,0.00437085466656924,
-0.00952106564267644));
#34850=CARTESIAN_POINT('Ctrl Pts',(-0.192098321240294,0.00430350915708436,
-0.00949717571328445));
#34851=CARTESIAN_POINT('Ctrl Pts',(-0.192106094964564,0.00417520799137725,
-0.00945166257049145));
#34852=CARTESIAN_POINT('Ctrl Pts',(-0.192115455498677,0.00404957328148242,
-0.00940391344723426));
#34853=CARTESIAN_POINT('Ctrl Pts',(-0.192125661936788,0.00393218901364697,
-0.0093566959282813));
#34854=CARTESIAN_POINT('Ctrl Pts',(-0.192133443844579,0.00384268927451646,
-0.00932069488907387));
#34855=CARTESIAN_POINT('Ctrl Pts',(-0.192141713192645,0.00375792550577707,
-0.00928514457643751));
#34856=CARTESIAN_POINT('Ctrl Pts',(-0.192150961541251,0.00366809730207177,
-0.00924584842708775));
#34857=CARTESIAN_POINT('Ctrl Pts',(-0.192155585715555,0.00362318320021912,
-0.00922620035241287));
#34858=CARTESIAN_POINT('Ctrl Pts',(-0.192160454647697,0.00357700519549584,
-0.00920561480746488));
#34859=CARTESIAN_POINT('Ctrl Pts',(-0.192166084452628,0.00352564880435533,
-0.00918214278170644));
#34860=CARTESIAN_POINT('Ctrl Pts',(-0.192171714257559,0.00347429241321481,
-0.009158670755948));
#34861=CARTESIAN_POINT('Ctrl Pts',(-0.192178107904039,0.00341782177126255,
-0.00913216947701166));
#34862=CARTESIAN_POINT('Ctrl Pts',(-0.192182856103435,0.00337653518451095,
-0.00911243306662588));
#34863=CARTESIAN_POINT('Ctrl Pts',(-0.192187604302832,0.00333524859775935,
-0.0090926966562401));
#34864=CARTESIAN_POINT('Ctrl Pts',(-0.192190702779538,0.00330904560688187,
-0.00907993339924628));
#34865=CARTESIAN_POINT('Ctrl Pts',(-0.192194848209666,0.00327420029768371,
-0.00906276405503103));
#34866=CARTESIAN_POINT('Ctrl Pts',(-0.192198993639795,0.00323935498848554,
-0.00904559471081578));
#34867=CARTESIAN_POINT('Ctrl Pts',(-0.192204188357678,0.00319592462016647,
-0.00902390474551468));
#34868=CARTESIAN_POINT('Ctrl Pts',(-0.192209757191958,0.00314991669976397,
-0.00900039555100338));
#34869=CARTESIAN_POINT('Ctrl Pts',(-0.192220894802916,0.00305790133484018,
-0.00895337740514728));
#34870=CARTESIAN_POINT('Ctrl Pts',(-0.192233524872454,0.00295546957808864,
-0.00889928118286497));
#34871=CARTESIAN_POINT('Ctrl Pts',(-0.192248325555084,0.00283771562762635,
-0.00883349052758685));
#34872=CARTESIAN_POINT('',(-0.191553952154239,0.00311173424349743,-0.00896743066851387));
#34873=CARTESIAN_POINT('Ctrl Pts',(-0.192248325784721,0.00283771380064023,
-0.00883348950682583));
#34874=CARTESIAN_POINT('Ctrl Pts',(-0.192159559175055,0.00287026003210736,
-0.00884999395305135));
#34875=CARTESIAN_POINT('Ctrl Pts',(-0.192051952701296,0.002909925198048,
-0.00886976448652076));
#34876=CARTESIAN_POINT('Ctrl Pts',(-0.191942427586231,0.00295087481736943,
-0.00888988564171143));
#34877=CARTESIAN_POINT('Ctrl Pts',(-0.191911532237965,0.00296233637983365,
-0.0088955006447997));
#34878=CARTESIAN_POINT('Ctrl Pts',(-0.191794791792164,0.00300748343666059,
-0.00891747224580303));
#34879=CARTESIAN_POINT('Ctrl Pts',(-0.19167990500933,0.00305483718076373,
-0.00894028783858838));
#34880=CARTESIAN_POINT('Ctrl Pts',(-0.191608493575298,0.00308573597984556,
-0.00895507813941301));
#34881=CARTESIAN_POINT('Ctrl Pts',(-0.191553952154239,0.00311173424349743,
-0.00896743066851387));
#34882=CARTESIAN_POINT('',(-0.190960920351713,0.00353164358673204,-0.00915988485915696));
#34883=CARTESIAN_POINT('Ctrl Pts',(-0.191553952154239,0.00311173424349743,
-0.00896743066851387));
#34884=CARTESIAN_POINT('Ctrl Pts',(-0.19155359586138,0.00311190407764358,
-0.00896751136164249));
#34885=CARTESIAN_POINT('Ctrl Pts',(-0.191498295283096,0.00313827803607244,
-0.00898004191267913));
#34886=CARTESIAN_POINT('Ctrl Pts',(-0.191373471881798,0.0032020936917313,
-0.00901021252823672));
#34887=CARTESIAN_POINT('Ctrl Pts',(-0.191231596802177,0.00329042310218504,
-0.00905130621942784));
#34888=CARTESIAN_POINT('Ctrl Pts',(-0.191109723337658,0.0033824962913484,
-0.0090935043810653));
#34889=CARTESIAN_POINT('Ctrl Pts',(-0.191016448616462,0.00346942958168849,
-0.0091324314801918));
#34890=CARTESIAN_POINT('Ctrl Pts',(-0.190985875275939,0.00350190193797071,
-0.00914685397494124));
#34891=CARTESIAN_POINT('Ctrl Pts',(-0.190959572667231,0.0035301458997474,
-0.00915922254898372));
#34892=CARTESIAN_POINT('Ctrl Pts',(-0.191002127391188,0.00750278968961046,
-0.0100244491176612));
#34893=CARTESIAN_POINT('Ctrl Pts',(-0.190990221104079,0.00736450438490425,
-0.0100242208049121));
#34894=CARTESIAN_POINT('Ctrl Pts',(-0.190976714774398,0.00720855534636783,
-0.01002089006384));
#34895=CARTESIAN_POINT('Ctrl Pts',(-0.19096297251905,0.00703989889402128,
-0.0100123976464476));
#34896=CARTESIAN_POINT('Ctrl Pts',(-0.190956101391376,0.006955570667848,
-0.0100081514377514));
#34897=CARTESIAN_POINT('Ctrl Pts',(-0.190949169912125,0.00686806652701917,
-0.0100026753145071));
#34898=CARTESIAN_POINT('Ctrl Pts',(-0.190942056597734,0.0067725971625629,
-0.00999519316408741));
#34899=CARTESIAN_POINT('Ctrl Pts',(-0.190938499940539,0.00672486248033477,
-0.00999145208887758));
#34900=CARTESIAN_POINT('Ctrl Pts',(-0.190934898866426,0.00667513881342257,
-0.00998716338353452));
#34901=CARTESIAN_POINT('Ctrl Pts',(-0.190931658652001,0.00663007179450303,
-0.00998295529844936));
#34902=CARTESIAN_POINT('Ctrl Pts',(-0.190928418437576,0.00658500477558349,
-0.0099787472133642));
#34903=CARTESIAN_POINT('Ctrl Pts',(-0.190925534780746,0.00654457897619451,
-0.00997481061464137));
#34904=CARTESIAN_POINT('Ctrl Pts',(-0.19092132251379,0.00647953294953688,
-0.00996770967567637));
#34905=CARTESIAN_POINT('Ctrl Pts',(-0.190917110246834,0.00641448692287925,
-0.00996060873671137));
#34906=CARTESIAN_POINT('Ctrl Pts',(-0.190911579923794,0.00632486907082429,
-0.00994987435196803));
#34907=CARTESIAN_POINT('Ctrl Pts',(-0.190907267674604,0.00624812638706539,
-0.00993961898765824));
#34908=CARTESIAN_POINT('Ctrl Pts',(-0.190902955425414,0.00617138370330648,
-0.00992936362334845));
#34909=CARTESIAN_POINT('Ctrl Pts',(-0.190899852732142,0.0061074629321523,
-0.00991996732482893));
#34910=CARTESIAN_POINT('Ctrl Pts',(-0.19089715233397,0.00604732256013647,
-0.00991064863510685));
#34911=CARTESIAN_POINT('Ctrl Pts',(-0.190891751537625,0.00592704181610479,
-0.00989201125566268));
#34912=CARTESIAN_POINT('Ctrl Pts',(-0.190887966444545,0.00582194003441517,
-0.00987339125729909));
#34913=CARTESIAN_POINT('Ctrl Pts',(-0.190885369196734,0.0057370259760568,
-0.00985739551877355));
#34914=CARTESIAN_POINT('Ctrl Pts',(-0.190882771948922,0.00565211191769842,
-0.00984139978024802));
#34915=CARTESIAN_POINT('Ctrl Pts',(-0.190881361562531,0.00558737163844979,
-0.00982807330323891));
#34916=CARTESIAN_POINT('Ctrl Pts',(-0.190880516547924,0.00554736685038776,
-0.00981970824679295));
#34917=CARTESIAN_POINT('Ctrl Pts',(-0.190879671533318,0.00550736206232573,
-0.00981134319034699));
#34918=CARTESIAN_POINT('Ctrl Pts',(-0.190879390734427,0.00549208313057967,
-0.00980799146704673));
#34919=CARTESIAN_POINT('Ctrl Pts',(-0.190879230051964,0.0054773044431616,
-0.00980478925362853));
#34920=CARTESIAN_POINT('Ctrl Pts',(-0.190879069369502,0.00546252575574354,
-0.00980158704021034));
#34921=CARTESIAN_POINT('Ctrl Pts',(-0.190879028737872,0.0054482467302615,
-0.00979853728640441));
#34922=CARTESIAN_POINT('Ctrl Pts',(-0.190878983617291,0.00540844431622106,
-0.00978961469117975));
#34923=CARTESIAN_POINT('Ctrl Pts',(-0.19087893849671,0.00536864190218062,
-0.00978069209595509));
#34924=CARTESIAN_POINT('Ctrl Pts',(-0.190878890080572,0.0053033293280606,
-0.00976584248435005));
#34925=CARTESIAN_POINT('Ctrl Pts',(-0.190879598832768,0.00521811957514347,
-0.00974492384284556));
#34926=CARTESIAN_POINT('Ctrl Pts',(-0.190880307584965,0.00513290982222635,
-0.00972400520134109));
#34927=CARTESIAN_POINT('Ctrl Pts',(-0.190881774469879,0.00502780711904499,
-0.00969697509695359));
#34928=CARTESIAN_POINT('Ctrl Pts',(-0.190884578999687,0.00490824705285926,
-0.00966337665691388));
#34929=CARTESIAN_POINT('Ctrl Pts',(-0.19088598126459,0.00484846701976639,
-0.00964657743689403));
#34930=CARTESIAN_POINT('Ctrl Pts',(-0.190887716330757,0.00478505569684817,
-0.00962820893403036));
#34931=CARTESIAN_POINT('Ctrl Pts',(-0.190890410878822,0.00470957227208617,
-0.00960523613729057));
#34932=CARTESIAN_POINT('Ctrl Pts',(-0.190893105426888,0.00463408884732416,
-0.00958226334055077));
#34933=CARTESIAN_POINT('Ctrl Pts',(-0.190896767981085,0.0045466489712431,
-0.00955429495332745));
#34934=CARTESIAN_POINT('Ctrl Pts',(-0.190899553155149,0.00448481957625672,
-0.00953379913870298));
#34935=CARTESIAN_POINT('Ctrl Pts',(-0.190902338329213,0.00442299018127034,
-0.0095133033240785));
#34936=CARTESIAN_POINT('Ctrl Pts',(-0.190904235759669,0.00438660942184642,
-0.00950076099502019));
#34937=CARTESIAN_POINT('Ctrl Pts',(-0.190906434316899,0.00434482368852979,
-0.00948618781464346));
#34938=CARTESIAN_POINT('Ctrl Pts',(-0.190907050637439,0.00433310991307086,
-0.00948210252167129));
#34939=CARTESIAN_POINT('Ctrl Pts',(-0.190907690955913,0.0043209760970172,
-0.00947784468285007));
#34940=CARTESIAN_POINT('Ctrl Pts',(-0.190908348288388,0.00430858853902742,
-0.00947346796251659));
#34941=CARTESIAN_POINT('Ctrl Pts',(-0.190910035812157,0.00427678682632307,
-0.00946223191399535));
#34942=CARTESIAN_POINT('Ctrl Pts',(-0.190911835469614,0.00424331587844342,
-0.00945020363068093));
#34943=CARTESIAN_POINT('Ctrl Pts',(-0.190913629094266,0.00421096117813992,
-0.00943837282589162));
#34944=CARTESIAN_POINT('Ctrl Pts',(-0.190918613666388,0.00412104585670863,
-0.00940549443093067));
#34945=CARTESIAN_POINT('Ctrl Pts',(-0.190923547291744,0.00403969563693671,
-0.00937427513158476));
#34946=CARTESIAN_POINT('Ctrl Pts',(-0.190928497783178,0.00396137688375242,
-0.00934312046999013));
#34947=CARTESIAN_POINT('Ctrl Pts',(-0.190938398766047,0.00380473937738384,
-0.00928081114680089));
#34948=CARTESIAN_POINT('Ctrl Pts',(-0.190948372721054,0.00366035364625716,
-0.00921849341705995));
#34949=CARTESIAN_POINT('Ctrl Pts',(-0.190957165817421,0.00353276917114798,
-0.00916037178863552));
#34950=CARTESIAN_POINT('Ctrl Pts',(-0.227150244243996,0.0164740029315869,
0.00232534147293063));
#34951=CARTESIAN_POINT('Ctrl Pts',(-0.237845216608682,0.0163630583331681,
0.00229659353481578));
#34952=CARTESIAN_POINT('Ctrl Pts',(-0.227150244243996,0.0164948323843597,
0.00192393728845175));
#34953=CARTESIAN_POINT('Ctrl Pts',(-0.237845216608682,0.0163665512368261,
0.0018892790127829));
#34954=CARTESIAN_POINT('Ctrl Pts',(-0.227150244243996,0.0165287121322363,
0.00114598487796074));
#34955=CARTESIAN_POINT('Ctrl Pts',(-0.237845216608682,0.0163722325524412,
0.00111537528026272));
#34956=CARTESIAN_POINT('Ctrl Pts',(-0.227150244243996,0.0165470707859482,
-9.63426955345028E-15));
#34957=CARTESIAN_POINT('Ctrl Pts',(-0.237845216608682,0.0163753111262956,
-3.20734770353177E-16));
#34958=CARTESIAN_POINT('Ctrl Pts',(-0.227150244243997,0.0165287121322335,
-0.00114598487798004));
#34959=CARTESIAN_POINT('Ctrl Pts',(-0.237845216608682,0.0163722325524407,
-0.00111537528026388));
#34960=CARTESIAN_POINT('Ctrl Pts',(-0.227150244243996,0.0164948323843552,
-0.00192393728847136));
#34961=CARTESIAN_POINT('Ctrl Pts',(-0.237845216608682,0.0163665512368254,
-0.00188927901278524));
#34962=CARTESIAN_POINT('Ctrl Pts',(-0.227150244243996,0.0164156764744566,
-0.00344935006783133));
#34963=CARTESIAN_POINT('Ctrl Pts',(-0.237845216608682,0.0163532775339462,
-0.0034371522067016));
#34964=CARTESIAN_POINT('Ctrl Pts',(-0.227150244243997,0.0158708078188047,
-0.00568348814190198));
#34965=CARTESIAN_POINT('Ctrl Pts',(-0.237845216608683,0.0158878089324482,
-0.00572426400319885));
#34966=CARTESIAN_POINT('Ctrl Pts',(-0.227150244243996,0.0138592003117079,
-0.00851222286772063));
#34967=CARTESIAN_POINT('Ctrl Pts',(-0.237845216608682,0.0139254525795067,
-0.00865325189315152));
#34968=CARTESIAN_POINT('Ctrl Pts',(-0.227150244243997,0.0109293641084061,
-0.0103996324725637));
#34969=CARTESIAN_POINT('Ctrl Pts',(-0.237845216608683,0.0109812780384655,
-0.0106210180177305));
#34970=CARTESIAN_POINT('Ctrl Pts',(-0.227150244243996,0.0074999999998714,
-0.0110623240930123));
#34971=CARTESIAN_POINT('Ctrl Pts',(-0.237845216608682,0.00749999999987136,
-0.01131420416039));
#34972=CARTESIAN_POINT('Ctrl Pts',(-0.227150244243997,0.00407063589135525,
-0.0103996324724683));
#34973=CARTESIAN_POINT('Ctrl Pts',(-0.237845216608683,0.00401872196129691,
-0.0106210180176321));
#34974=CARTESIAN_POINT('Ctrl Pts',(-0.227150244243996,0.00114079968810594,
-0.00851222286754358));
#34975=CARTESIAN_POINT('Ctrl Pts',(-0.237845216608682,0.00107454742031117,
-0.00865325189296982));
#34976=CARTESIAN_POINT('Ctrl Pts',(-0.227150244243997,-0.000870807818911773,
-0.00568348814166902));
#34977=CARTESIAN_POINT('Ctrl Pts',(-0.237845216608682,-0.00088780893254747,
-0.00572426400296157));
#34978=CARTESIAN_POINT('Ctrl Pts',(-0.227150244243996,-0.00141567647450146,
-0.00344935006758328));
#34979=CARTESIAN_POINT('Ctrl Pts',(-0.237845216608682,-0.00135327753398082,
-0.00343715220645101));
#34980=CARTESIAN_POINT('Ctrl Pts',(-0.227150244243996,-0.00149483238436559,
-0.00192393728824214));
#34981=CARTESIAN_POINT('Ctrl Pts',(-0.237845216608682,-0.00136655123682709,
-0.00188927901255543));
#34982=CARTESIAN_POINT('Ctrl Pts',(-0.227150244243996,-0.0015287121322383,
-0.00114598487779204));
#34983=CARTESIAN_POINT('Ctrl Pts',(-0.237845216608682,-0.00137223255244152,
-0.0011153752800763));
#34984=CARTESIAN_POINT('Ctrl Pts',(-0.227150244243997,-0.00154707078594764,
1.16062262795529E-13));
#34985=CARTESIAN_POINT('Ctrl Pts',(-0.237845216608682,-0.00137531112629545,
1.24505090562086E-13));
#34986=CARTESIAN_POINT('Ctrl Pts',(-0.227150244243996,-0.00152871213223388,
0.00114598487802365));
#34987=CARTESIAN_POINT('Ctrl Pts',(-0.237845216608682,-0.00137223255244077,
0.00111537528032471));
#34988=CARTESIAN_POINT('Ctrl Pts',(-0.227150244243996,-0.0014948323843583,
0.00192393728847254));
#34989=CARTESIAN_POINT('Ctrl Pts',(-0.237845216608682,-0.00136655123682587,
0.00188927901280252));
#34990=CARTESIAN_POINT('Ctrl Pts',(-0.227150244243996,-0.00141567647446389,
0.00344935006836688));
#34991=CARTESIAN_POINT('Ctrl Pts',(-0.237845216608682,-0.00135327753394768,
0.00343715220737864));
#34992=CARTESIAN_POINT('Ctrl Pts',(-0.227150244243997,-0.000870821762961343,
0.00568349039573915));
#34993=CARTESIAN_POINT('Ctrl Pts',(-0.237845216608682,-0.000887826039510656,
0.00572426676828764));
#34994=CARTESIAN_POINT('Ctrl Pts',(-0.227150244243997,0.00114085439618864,
0.00851222287679413));
#34995=CARTESIAN_POINT('Ctrl Pts',(-0.237845216608682,0.0010746145376654,
0.00865325190429854));
#34996=CARTESIAN_POINT('Ctrl Pts',(-0.227150244243996,0.00407062011024736,
0.0103996408584618));
#34997=CARTESIAN_POINT('Ctrl Pts',(-0.237845216608682,0.00401870260056976,
0.0106210283057897));
#34998=CARTESIAN_POINT('Ctrl Pts',(-0.227150244243997,0.00750000000000013,
0.0110623211795783));
#34999=CARTESIAN_POINT('Ctrl Pts',(-0.237845216608683,0.00749999999999948,
0.0113142005861093));
#35000=CARTESIAN_POINT('Ctrl Pts',(-0.227150244243996,0.0109293798897529,
0.0103996408584618));
#35001=CARTESIAN_POINT('Ctrl Pts',(-0.237845216608681,0.0109812973994292,
0.0106210283057901));
#35002=CARTESIAN_POINT('Ctrl Pts',(-0.227150244243997,0.0138591456038116,
0.00851222287679417));
#35003=CARTESIAN_POINT('Ctrl Pts',(-0.237845216608683,0.0139253854623337,
0.00865325190429944));
#35004=CARTESIAN_POINT('Ctrl Pts',(-0.227150244243997,0.0158708217629616,
0.00568349039573924));
#35005=CARTESIAN_POINT('Ctrl Pts',(-0.237845216608682,0.0158878260395101,
0.00572426676828895));
#35006=CARTESIAN_POINT('Ctrl Pts',(-0.227150244243996,0.0164156764744642,
0.00344935006836702));
#35007=CARTESIAN_POINT('Ctrl Pts',(-0.237845216608682,0.0163532775339475,
0.00343715220738017));
#35008=CARTESIAN_POINT('Ctrl Pts',(-0.227150244243996,0.0164740029315869,
0.00232534147293065));
#35009=CARTESIAN_POINT('Ctrl Pts',(-0.237845216608682,0.0163630583331681,
0.0022965935348158));
#35010=CARTESIAN_POINT('Ctrl Pts',(-0.228219847986792,0.016461711610013,
0.00232234304728456));
#35011=CARTESIAN_POINT('Ctrl Pts',(-0.228197323008168,0.016464402919773,
0.00228169207879242));
#35012=CARTESIAN_POINT('Ctrl Pts',(-0.228079010729088,0.0164779108194991,
0.00206553236692686));
#35013=CARTESIAN_POINT('Ctrl Pts',(-0.227880678619148,0.0164952290445269,
0.00167731055896527));
#35014=CARTESIAN_POINT('Ctrl Pts',(-0.227674259713159,0.0165145714831501,
0.00121095180943624));
#35015=CARTESIAN_POINT('Ctrl Pts',(-0.227539125616474,0.0165251767327821,
0.000875323514963339));
#35016=CARTESIAN_POINT('Ctrl Pts',(-0.227433352259856,0.0165318672222558,
0.000599149205354619));
#35017=CARTESIAN_POINT('Ctrl Pts',(-0.227387103565297,0.0165342612366672,
0.000474629663494434));
#35018=CARTESIAN_POINT('Ctrl Pts',(-0.227320232205383,0.0165373421710725,
0.000293417962783554));
#35019=CARTESIAN_POINT('Ctrl Pts',(-0.227259872684817,0.0165392417731146,
0.00012778562427802));
#35020=CARTESIAN_POINT('Ctrl Pts',(-0.22721365317106,0.0165399630933673,
2.96878969900656E-7));
#35021=CARTESIAN_POINT('Ctrl Pts',(-0.230613689225592,0.0164370167296803,
0.00231666183293795));
#35022=CARTESIAN_POINT('Ctrl Pts',(-0.230153199896009,0.0164750623910427,
0.00163855477769135));
#35023=CARTESIAN_POINT('Ctrl Pts',(-0.229898110941495,0.0164961381222382,
0.000819433299928898));
#35024=CARTESIAN_POINT('Ctrl Pts',(-0.22989804971791,0.016496143666697,
2.94875754180074E-7));
#35025=CARTESIAN_POINT('Ctrl Pts',(-0.228031317757249,0.0074842289792918,
0.0108613267143847));
#35026=CARTESIAN_POINT('Ctrl Pts',(-0.227896128234583,0.00732271517640735,
0.0108579839540074));
#35027=CARTESIAN_POINT('Ctrl Pts',(-0.227765076018135,0.00716310491063475,
0.010850325819301));
#35028=CARTESIAN_POINT('Ctrl Pts',(-0.227510609193765,0.00684731467260396,
0.0108270338085957));
#35029=CARTESIAN_POINT('Ctrl Pts',(-0.227389668743883,0.00669440562499774,
0.010811585495654));
#35030=CARTESIAN_POINT('Ctrl Pts',(-0.227162362130326,0.00640136431994779,
0.0107751132274823));
#35031=CARTESIAN_POINT('Ctrl Pts',(-0.227055775511969,0.00626093688400325,
0.0107540679242784));
#35032=CARTESIAN_POINT('Ctrl Pts',(-0.226906495617072,0.0060594832359516,
0.010719534205083));
#35033=CARTESIAN_POINT('Ctrl Pts',(-0.226858502324212,0.00599386222138074,
0.0107075273154425));
#35034=CARTESIAN_POINT('Ctrl Pts',(-0.226766049082705,0.00586567726531639,
0.0106827143943246));
#35035=CARTESIAN_POINT('Ctrl Pts',(-0.226722124661603,0.00580387778100626,
0.010670098269507));
#35036=CARTESIAN_POINT('Ctrl Pts',(-0.226585218374531,0.00560808410484936,
0.0106279534125427));
#35037=CARTESIAN_POINT('Ctrl Pts',(-0.22649022366447,0.00546820172234809,
0.0105949410804036));
#35038=CARTESIAN_POINT('Ctrl Pts',(-0.226366825461877,0.00528228167215783,
0.010545833840231));
#35039=CARTESIAN_POINT('Ctrl Pts',(-0.226342874294171,0.00524602651289862,
0.0105360458953431));
#35040=CARTESIAN_POINT('Ctrl Pts',(-0.226286724768651,0.0051604222146116,
0.0105122439934791));
#35041=CARTESIAN_POINT('Ctrl Pts',(-0.226255147092778,0.00511204014714452,
0.0104984660406559));
#35042=CARTESIAN_POINT('Ctrl Pts',(-0.22614990532583,0.00495042207797637,
0.0104506682428966));
#35043=CARTESIAN_POINT('Ctrl Pts',(-0.226065736316993,0.00482068030019097,
0.0104102462744603));
#35044=CARTESIAN_POINT('Ctrl Pts',(-0.22596754801256,0.00467004487225661,
0.0103583034518151));
#35045=CARTESIAN_POINT('Ctrl Pts',(-0.228033577259197,0.00748440686309183,
0.0107613524026377));
#35046=CARTESIAN_POINT('Ctrl Pts',(-0.227898387621481,0.00732471444696238,
0.0107580128797965));
#35047=CARTESIAN_POINT('Ctrl Pts',(-0.227767333526622,0.00716689330363822,
0.0107504075964718));
#35048=CARTESIAN_POINT('Ctrl Pts',(-0.227512859749499,0.00685462755823802,
0.0107273112564122));
#35049=CARTESIAN_POINT('Ctrl Pts',(-0.227391914277135,0.00670341734486022,
0.0107120043085084));
#35050=CARTESIAN_POINT('Ctrl Pts',(-0.227164595337582,0.00641362330544489,
0.0106758791788512));
#35051=CARTESIAN_POINT('Ctrl Pts',(-0.227058001408668,0.0062747475907083,
0.0106550398501494));
#35052=CARTESIAN_POINT('Ctrl Pts',(-0.226908709318108,0.00607551732420086,
0.0106208500119865));
#35053=CARTESIAN_POINT('Ctrl Pts',(-0.226860711754346,0.00601062006567001,
0.0106089635890604));
#35054=CARTESIAN_POINT('Ctrl Pts',(-0.226768249633801,0.00588384843464617,
0.0105844012148158));
#35055=CARTESIAN_POINT('Ctrl Pts',(-0.226724320673869,0.00582273009633135,
0.0105719132109536));
#35056=CARTESIAN_POINT('Ctrl Pts',(-0.226587399145727,0.00562909428433601,
0.01053019877818));
#35057=CARTESIAN_POINT('Ctrl Pts',(-0.226492392400433,0.00549075322107965,
0.0104975265728443));
#35058=CARTESIAN_POINT('Ctrl Pts',(-0.226368976136859,0.00530688423445996,
0.0104489304488435));
#35059=CARTESIAN_POINT('Ctrl Pts',(-0.226345021363545,0.00527102914326667,
0.0104392445660052));
#35060=CARTESIAN_POINT('Ctrl Pts',(-0.226288863050377,0.00518636992476106,
0.0104156915057688));
#35061=CARTESIAN_POINT('Ctrl Pts',(-0.226257280279058,0.00513852220521404,
0.0104020578835452));
#35062=CARTESIAN_POINT('Ctrl Pts',(-0.22615202079073,0.00497869053802895,
0.0103547623018));
#35063=CARTESIAN_POINT('Ctrl Pts',(-0.226067836783359,0.00485038433404092,
0.0103147666318135));
#35064=CARTESIAN_POINT('Ctrl Pts',(-0.225969628990936,0.00470142166790477,
0.0102633762890857));
#35065=CARTESIAN_POINT('Ctrl Pts',(-0.228033588556707,0.00748440775251083,
0.010760852531079));
#35066=CARTESIAN_POINT('Ctrl Pts',(-0.227898398918416,0.00732472444331515,
0.0107575130244254));
#35067=CARTESIAN_POINT('Ctrl Pts',(-0.227767344814165,0.00716691224560324,
0.0107499080053577));
#35068=CARTESIAN_POINT('Ctrl Pts',(-0.227512871002277,0.00685466412266619,
0.0107268126436513));
#35069=CARTESIAN_POINT('Ctrl Pts',(-0.227391925504801,0.00670346240345954,
0.0107115064025727));
#35070=CARTESIAN_POINT('Ctrl Pts',(-0.227164606503619,0.00641368460037238,
0.010675383008608));
#35071=CARTESIAN_POINT('Ctrl Pts',(-0.227058012538152,0.00627481664424182,
0.0106545447097788));
#35072=CARTESIAN_POINT('Ctrl Pts',(-0.226908720386613,0.00607559749464211,
0.010620356591021));
#35073=CARTESIAN_POINT('Ctrl Pts',(-0.226860722801496,0.00601070385489146,
0.0106084707704285));
#35074=CARTESIAN_POINT('Ctrl Pts',(-0.226768260636557,0.00588393929049282,
0.0105839096489183));
#35075=CARTESIAN_POINT('Ctrl Pts',(-0.226724331653931,0.00582282435790797,
0.0105714222856609));
#35076=CARTESIAN_POINT('Ctrl Pts',(-0.226587410049583,0.00562919933523344,
0.0105297100050082));
#35077=CARTESIAN_POINT('Ctrl Pts',(-0.226492403244113,0.00549086597857331,
0.0104970395003065));
#35078=CARTESIAN_POINT('Ctrl Pts',(-0.226368986890234,0.00530700724727147,
0.0104484459318865));
#35079=CARTESIAN_POINT('Ctrl Pts',(-0.226345032098891,0.00527115415641851,
0.0104387605593585));
#35080=CARTESIAN_POINT('Ctrl Pts',(-0.226288873741786,0.00518649966331181,
0.0104152087433303));
#35081=CARTESIAN_POINT('Ctrl Pts',(-0.22625729094499,0.00513865461550439,
0.0104015758427596));
#35082=CARTESIAN_POINT('Ctrl Pts',(-0.226152031368055,0.00497883188032922,
0.0103542827720945));
#35083=CARTESIAN_POINT('Ctrl Pts',(-0.226067847285692,0.00485053285421017,
0.0103142892336002));
#35084=CARTESIAN_POINT('Ctrl Pts',(-0.225969639395827,0.00470157855188301,
0.0102629016532721));
#35085=CARTESIAN_POINT('',(-0.228033577259201,0.00748440686309334,0.0107613524025277));
#35086=CARTESIAN_POINT('',(-0.225967548079419,0.0046700458803542,0.0103583004019229));
#35087=CARTESIAN_POINT('Ctrl Pts',(-0.228074264635775,0.00750982551816477,
-0.0108453770253309));
#35088=CARTESIAN_POINT('Ctrl Pts',(-0.228010676434541,0.00740838976828053,
-0.0105824436407257));
#35089=CARTESIAN_POINT('Ctrl Pts',(-0.2279824250062,0.00743349469607835,
-0.0102960204663357));
#35090=CARTESIAN_POINT('Ctrl Pts',(-0.227032943648517,0.00632417137993069,
-0.0115546191985225));
#35091=CARTESIAN_POINT('Ctrl Pts',(-0.226887473210818,0.00609211727794893,
-0.0109531076947852));
#35092=CARTESIAN_POINT('Ctrl Pts',(-0.226822842547162,0.0061495497066744,
-0.0102978587061822));
#35093=CARTESIAN_POINT('Ctrl Pts',(-0.226297317381162,0.00493120265784604,
-0.0122699105575636));
#35094=CARTESIAN_POINT('Ctrl Pts',(-0.226063698082153,0.00455853369847132,
-0.0113039088181618));
#35095=CARTESIAN_POINT('Ctrl Pts',(-0.225959904001537,0.00465076772176458,
-0.0102516069772177));
#35096=CARTESIAN_POINT('',(-0.228051045268546,0.00748331776699234,-0.0108612187236825));
#35097=CARTESIAN_POINT('Ctrl Pts',(-0.228054819889729,0.00748068141629659,
-0.0107604444270582));
#35098=CARTESIAN_POINT('Ctrl Pts',(-0.228053849738522,0.00748110294260517,
-0.0107931625663296));
#35099=CARTESIAN_POINT('Ctrl Pts',(-0.228052595462817,0.00748196696929443,
-0.0108267367625979));
#35100=CARTESIAN_POINT('Ctrl Pts',(-0.228051045268536,0.00748331776753071,
-0.0108612187236609));
#35101=CARTESIAN_POINT('',(-0.225969776335003,0.0046444390782959,-0.010349214474902));
#35102=CARTESIAN_POINT('Ctrl Pts',(-0.225970412829803,0.00464426457540287,
-0.010349129960529));
#35103=CARTESIAN_POINT('Ctrl Pts',(-0.22636217413668,0.00527485403368463,
-0.0105691174221872));
#35104=CARTESIAN_POINT('Ctrl Pts',(-0.226793102923008,0.00589537795378531,
-0.0107098724323669));
#35105=CARTESIAN_POINT('Ctrl Pts',(-0.227558354882916,0.00688782458229315,
-0.0108376974244079));
#35106=CARTESIAN_POINT('Ctrl Pts',(-0.227831875264664,0.00721793479916253,
-0.0108558255878856));
#35107=CARTESIAN_POINT('Ctrl Pts',(-0.228051045268268,0.007483317767219,
-0.0108612187237897));
#35108=CARTESIAN_POINT('Ctrl Pts',(-0.225969808834085,0.00464327366247554,
-0.0103488652066219));
#35109=CARTESIAN_POINT('Ctrl Pts',(-0.225970621228311,0.00465291285345407,
-0.0103160414183464));
#35110=CARTESIAN_POINT('Ctrl Pts',(-0.225971427024039,0.00466253501940138,
-0.0102838463488178));
#35111=CARTESIAN_POINT('Ctrl Pts',(-0.225972227593275,0.00467213421594552,
-0.0102522642048503));
#35112=CARTESIAN_POINT('Origin',(-0.226575103310132,0.00449228442477202,
-0.00733395845215797));
#35113=CARTESIAN_POINT('',(-0.226088434634005,0.00750609353843923,-0.010817348945422));
#35114=CARTESIAN_POINT('Ctrl Pts',(-0.226088397422881,0.00750571596719848,
-0.0108173527010167));
#35115=CARTESIAN_POINT('Ctrl Pts',(-0.226046795568232,0.00707975121101806,
-0.0108166967955858));
#35116=CARTESIAN_POINT('Ctrl Pts',(-0.226012355211352,0.00663228020961852,
-0.0107848740755647));
#35117=CARTESIAN_POINT('Ctrl Pts',(-0.225963781900347,0.00565398292249233,
-0.0106396516049241));
#35118=CARTESIAN_POINT('Ctrl Pts',(-0.225955904863431,0.00512512163672698,
-0.0105097994417222));
#35119=CARTESIAN_POINT('Ctrl Pts',(-0.225969743835921,0.00464560449411625,
-0.0103495637431821));
#35120=CARTESIAN_POINT('Ctrl Pts',(-0.226088471845129,0.00750647110967997,
-0.0108173451898272));
#35121=CARTESIAN_POINT('Ctrl Pts',(-0.226091014474231,0.00750607256368142,
-0.010783628416141));
#35122=CARTESIAN_POINT('Ctrl Pts',(-0.226093586961953,0.00750568099604601,
-0.0107499136549416));
#35123=CARTESIAN_POINT('Ctrl Pts',(-0.226096189362409,0.00750529647355148,
-0.0107162198524223));
#35124=CARTESIAN_POINT('Origin',(-0.215,-0.00247776328493882,0.0055));
#35125=CARTESIAN_POINT('',(-0.215000000652701,-0.000412667879180649,0.0055002646485004));
#35126=CARTESIAN_POINT('',(-0.192200819587666,-0.000325482083450908,0.0055001426619674));
#35127=CARTESIAN_POINT('Ctrl Pts',(-0.215000000137371,-0.000412703772444445,
0.00550080483265447));
#35128=CARTESIAN_POINT('Ctrl Pts',(-0.207400273519179,-0.000383662849035535,
0.00550259700144263));
#35129=CARTESIAN_POINT('Ctrl Pts',(-0.199800545652181,-0.000354576027343994,
0.005502376420274));
#35130=CARTESIAN_POINT('Ctrl Pts',(-0.192200819587666,-0.000325482083450908,
0.0055001426619674));
#35131=CARTESIAN_POINT('',(-0.192768810477056,-0.000446740227034733,0.00549999916447762));
#35132=CARTESIAN_POINT('Origin',(-0.194168411395185,0.0075,0.0055));
#35133=CARTESIAN_POINT('',(-0.203737790159114,-0.000488441743501772,0.00550001369129769));
#35134=CARTESIAN_POINT('Ctrl Pts',(-0.192768810477182,-0.000446740193101186,
0.00549999665791052));
#35135=CARTESIAN_POINT('Ctrl Pts',(-0.196360853593688,-0.000461346127092089,
0.00549997224869372));
#35136=CARTESIAN_POINT('Ctrl Pts',(-0.200017180154384,-0.000475246610178321,
0.00550000407222806));
#35137=CARTESIAN_POINT('Ctrl Pts',(-0.203737790159114,-0.000488441743501772,
0.00550001369129769));
#35138=CARTESIAN_POINT('',(-0.214999999997124,-0.000525629251200218,0.0055000000000044));
#35139=CARTESIAN_POINT('Ctrl Pts',(-0.203737790159114,-0.000488441743501772,
0.00550001369129769));
#35140=CARTESIAN_POINT('Ctrl Pts',(-0.207428602217097,-0.000501531198487641,
0.00550002323332928));
#35141=CARTESIAN_POINT('Ctrl Pts',(-0.211182672164629,-0.000513926566459491,
0.00550001115861136));
#35142=CARTESIAN_POINT('Ctrl Pts',(-0.214999999996537,-0.000525629250696233,
0.00550005330994453));
#35143=CARTESIAN_POINT('',(-0.215,-0.00247776328493882,0.0055));
#35144=CARTESIAN_POINT('Origin',(-0.215,-0.00247776328493882,0.0055));
#35145=CARTESIAN_POINT('',(-0.215000000652833,0.0154126678792567,0.00550026464927285));
#35146=CARTESIAN_POINT('',(-0.214999999997124,0.0155256292511986,0.0055000000000044));
#35147=CARTESIAN_POINT('',(-0.215,-0.00247776328493882,0.0055));
#35148=CARTESIAN_POINT('',(-0.20373779012803,0.015488441743392,0.00550001369129815));
#35149=CARTESIAN_POINT('Ctrl Pts',(-0.214999999996537,0.0155256292506966,
0.0055000533099388));
#35150=CARTESIAN_POINT('Ctrl Pts',(-0.211182672153911,0.0155139265664271,
0.00550001115860741));
#35151=CARTESIAN_POINT('Ctrl Pts',(-0.207428602197274,0.0155015308720983,
0.00549998488159998));
#35152=CARTESIAN_POINT('Ctrl Pts',(-0.20373779012803,0.015488441743392,
0.00550001369129815));
#35153=CARTESIAN_POINT('',(-0.192768810477057,0.0154467402270351,0.00549999916447917));
#35154=CARTESIAN_POINT('Ctrl Pts',(-0.20373779012803,0.015488441743392,
0.00550001369129815));
#35155=CARTESIAN_POINT('Ctrl Pts',(-0.200017180135304,0.0154752462761579,
0.00549996529271644));
#35156=CARTESIAN_POINT('Ctrl Pts',(-0.196360853583685,0.0154613461270517,
0.00549997224869849));
#35157=CARTESIAN_POINT('Ctrl Pts',(-0.192768810477184,0.0154467401931016,
0.00549999665791672));
#35158=CARTESIAN_POINT('',(-0.192200819587632,0.0153254820834438,0.00550014266023027));
#35159=CARTESIAN_POINT('Origin',(-0.194168411395185,0.0075,0.0055));
#35160=CARTESIAN_POINT('Ctrl Pts',(-0.192200819587632,0.0153254820834438,
0.00550014266023027));
#35161=CARTESIAN_POINT('Ctrl Pts',(-0.199800545652162,0.0153545760275143,
0.00550237641958232));
#35162=CARTESIAN_POINT('Ctrl Pts',(-0.207400273519175,0.0153836628489491,
0.00550259700179216));
#35163=CARTESIAN_POINT('Ctrl Pts',(-0.215000000137363,0.0154127037724312,
0.00550080483406418));
#35164=CARTESIAN_POINT('Origin',(-0.215,-0.00247776328493882,-0.0055));
#35165=CARTESIAN_POINT('',(-0.21499999999666,-0.00052563024928965,-0.00550000000000594));
#35166=CARTESIAN_POINT('',(-0.215000000652509,-0.000412669026508687,-0.00550026458441123));
#35167=CARTESIAN_POINT('',(-0.215,-0.00247776328493882,-0.0055));
#35168=CARTESIAN_POINT('',(-0.203436374848878,-0.000487371363831537,-0.00550001526954719));
#35169=CARTESIAN_POINT('Ctrl Pts',(-0.214999999995963,-0.000525630248646836,
-0.0055000585798767));
#35170=CARTESIAN_POINT('Ctrl Pts',(-0.211078734069006,-0.000513608696396548,
-0.00550001184318302));
#35171=CARTESIAN_POINT('Ctrl Pts',(-0.207224192351256,-0.000500856290275313,
-0.00550002560630164));
#35172=CARTESIAN_POINT('Ctrl Pts',(-0.203436374848878,-0.000487371363831537,
-0.00550001526954719));
#35173=CARTESIAN_POINT('',(-0.192317997805077,-0.000444941992647508,-0.0054999973805848));
#35174=CARTESIAN_POINT('Ctrl Pts',(-0.203436374848878,-0.000487371363831537,
-0.00550001526954719));
#35175=CARTESIAN_POINT('Ctrl Pts',(-0.19966407605156,-0.000473941685191043,
-0.00550000497514246));
#35176=CARTESIAN_POINT('Ctrl Pts',(-0.19595795585078,-0.000459785480996097,
-0.00549997085736725));
#35177=CARTESIAN_POINT('Ctrl Pts',(-0.192318014246932,-0.000444902576975657,
-0.00549999627590324));
#35178=CARTESIAN_POINT('',(-0.192182752978689,-0.00032540324872727,-0.00550013765774565));
#35179=CARTESIAN_POINT('Ctrl Pts',(-0.192317958818237,-0.000445035454884037,
-0.00549999999999998));
#35180=CARTESIAN_POINT('Ctrl Pts',(-0.192281469524508,-0.000429789928121892,
-0.00549999999999998));
#35181=CARTESIAN_POINT('Ctrl Pts',(-0.192251227013467,-0.000413059060916608,
-0.00549999999897596));
#35182=CARTESIAN_POINT('Ctrl Pts',(-0.192217246193221,-0.000387604767502657,
-0.00549999999897596));
#35183=CARTESIAN_POINT('Ctrl Pts',(-0.192201562270466,-0.000374406090242385,
-0.00550000000001939));
#35184=CARTESIAN_POINT('Ctrl Pts',(-0.192187769696388,-0.000353338816389856,
-0.00550000000001939));
#35185=CARTESIAN_POINT('Ctrl Pts',(-0.192184706735899,-0.000347322586940135,
-0.00549999999999998));
#35186=CARTESIAN_POINT('Ctrl Pts',(-0.192182140916727,-0.0003382625628242,
-0.00549999999999998));
#35187=CARTESIAN_POINT('Ctrl Pts',(-0.192181602954142,-0.000335449050862324,
-0.00549999999999998));
#35188=CARTESIAN_POINT('Ctrl Pts',(-0.192181177992225,-0.000330149245389187,
-0.00549999999999998));
#35189=CARTESIAN_POINT('Ctrl Pts',(-0.192181212347043,-0.00032770017804238,
-0.00549999999999998));
#35190=CARTESIAN_POINT('Ctrl Pts',(-0.192181505015942,-0.000325264067446612,
-0.00549999999999998));
#35191=CARTESIAN_POINT('Ctrl Pts',(-0.192182752978689,-0.00032540324872727,
-0.00550013765774565));
#35192=CARTESIAN_POINT('Ctrl Pts',(-0.199788501242498,-0.00035452409238897,
-0.00550237637378411));
#35193=CARTESIAN_POINT('Ctrl Pts',(-0.207394251315731,-0.000383637427213978,
-0.0055025986106267));
#35194=CARTESIAN_POINT('Ctrl Pts',(-0.215000000137357,-0.000412704938748334,
-0.00550080479377357));
#35195=CARTESIAN_POINT('Origin',(-0.215,-0.00247776328493882,-0.0055));
#35196=CARTESIAN_POINT('',(-0.215000000653156,0.0154126690265686,-0.00550026455391182));
#35197=CARTESIAN_POINT('',(-0.192200822396014,0.0153254827916868,-0.00550014285674479));
#35198=CARTESIAN_POINT('Ctrl Pts',(-0.215000000137355,0.0154127049387179,
-0.005500804798221));
#35199=CARTESIAN_POINT('Ctrl Pts',(-0.207400274455338,0.0153836638777327,
-0.0055025971330885));
#35200=CARTESIAN_POINT('Ctrl Pts',(-0.199800547524418,0.0153545768886244,
-0.00550237662849891));
#35201=CARTESIAN_POINT('Ctrl Pts',(-0.192200822396014,0.0153254827916868,
-0.00550014285674479));
#35202=CARTESIAN_POINT('',(-0.192768813717413,0.0154467407873535,-0.00549999832876385));
#35203=CARTESIAN_POINT('Origin',(-0.194168411395185,0.0075,-0.0055));
#35204=CARTESIAN_POINT('',(-0.203737786417006,0.0154884425231616,-0.00550001369217832));
#35205=CARTESIAN_POINT('Ctrl Pts',(-0.1927688137175,0.0154467407637849,
-0.0054999966575277));
#35206=CARTESIAN_POINT('Ctrl Pts',(-0.196360852334629,0.0154613467899902,
-0.00549997224670963));
#35207=CARTESIAN_POINT('Ctrl Pts',(-0.200017176569134,0.0154752470087536,
-0.00549996529032058));
#35208=CARTESIAN_POINT('Ctrl Pts',(-0.203737786417006,0.0154884425231616,
-0.00550001369217832));
#35209=CARTESIAN_POINT('',(-0.214999999997124,0.0155256300978718,-0.0055000000000044));
#35210=CARTESIAN_POINT('Ctrl Pts',(-0.203737786417006,0.0154884425231616,
-0.00550001369217832));
#35211=CARTESIAN_POINT('Ctrl Pts',(-0.207428597610741,0.0155015316960027,
-0.00549998488064372));
#35212=CARTESIAN_POINT('Ctrl Pts',(-0.211182668804386,0.0155139274126174,
-0.00550001115947315));
#35213=CARTESIAN_POINT('Ctrl Pts',(-0.214999999996537,0.0155256300973698,
-0.0055000533136723));
#35214=CARTESIAN_POINT('',(-0.215,-0.00247776328493882,-0.0055));
#35215=CARTESIAN_POINT('Origin',(-0.227003760671838,0.00749996257915086,
-0.00184311590365041));
#35216=CARTESIAN_POINT('',(-0.225965850681397,0.0102943062435013,-0.0103692862560009));
#35217=CARTESIAN_POINT('Ctrl Pts',(-0.228051045268804,0.00748331776721652,
-0.0108612187238017));
#35218=CARTESIAN_POINT('Ctrl Pts',(-0.228046268562556,0.0074888841515757,
-0.0108611222719965));
#35219=CARTESIAN_POINT('Ctrl Pts',(-0.228041495105673,0.00749445191188697,
-0.0108610207252172));
#35220=CARTESIAN_POINT('Ctrl Pts',(-0.227530170041864,0.0080914144788298,
-0.0108495888326834));
#35221=CARTESIAN_POINT('Ctrl Pts',(-0.227035276032252,0.00872930600873977,
-0.0107790866609926));
#35222=CARTESIAN_POINT('Ctrl Pts',(-0.226365419755937,0.0096839489506607,
-0.0105596857066268));
#35223=CARTESIAN_POINT('Ctrl Pts',(-0.226161417598064,0.00998868739612624,
-0.0104735785805751));
#35224=CARTESIAN_POINT('Ctrl Pts',(-0.225966633299167,0.0102930893843531,
-0.0103697246588685));
#35225=CARTESIAN_POINT('Ctrl Pts',(-0.225965034805744,0.0102941399146425,
-0.0103693454509162));
#35226=CARTESIAN_POINT('Ctrl Pts',(-0.225943934273099,0.00937798607974839,
-0.010668449685717));
#35227=CARTESIAN_POINT('Ctrl Pts',(-0.225999253113111,0.00841521474472878,
-0.0108147357619121));
#35228=CARTESIAN_POINT('Ctrl Pts',(-0.226088508031683,0.00750609596646259,
-0.0108173549212978));
#35229=CARTESIAN_POINT('Ctrl Pts',(-0.185819463593633,0.0166104930553049,
0.00236863820262676));
#35230=CARTESIAN_POINT('Ctrl Pts',(-0.203223508587672,0.0164247592890707,
0.00234416866113263));
#35231=CARTESIAN_POINT('Ctrl Pts',(-0.220627582451438,0.0162418056983084,
0.00231971009381821));
#35232=CARTESIAN_POINT('Ctrl Pts',(-0.238031675744303,0.0160611171225611,
0.00229373846137714));
#35233=CARTESIAN_POINT('Ctrl Pts',(-0.18581926440362,0.0166461165277183,
0.00221607060080922));
#35234=CARTESIAN_POINT('Ctrl Pts',(-0.203223313044138,0.0164497831264032,
0.00218726310900855));
#35235=CARTESIAN_POINT('Ctrl Pts',(-0.220627389279833,0.0162559154123599,
0.00215868502272393));
#35236=CARTESIAN_POINT('Ctrl Pts',(-0.238031485810861,0.0160641905057161,
0.0021289558365353));
#35237=CARTESIAN_POINT('Ctrl Pts',(-0.185818880874426,0.0167106984888996,
0.00190682671781972));
#35238=CARTESIAN_POINT('Ctrl Pts',(-0.203222934036142,0.0164938099422013,
0.00186885154579339));
#35239=CARTESIAN_POINT('Ctrl Pts',(-0.220627006269502,0.016278128585195,
0.00183193650018925));
#35240=CARTESIAN_POINT('Ctrl Pts',(-0.238031099947329,0.0160640878015832,
0.00179531454904686));
#35241=CARTESIAN_POINT('Ctrl Pts',(-0.185818335405062,0.0168157482814852,
0.00126613919744405));
#35242=CARTESIAN_POINT('Ctrl Pts',(-0.203222383696577,0.0165663597906042,
0.00122992539721983));
#35243=CARTESIAN_POINT('Ctrl Pts',(-0.220626440719063,0.016317358802535,
0.00119476376827596));
#35244=CARTESIAN_POINT('Ctrl Pts',(-0.238030512988197,0.0160691276034975,
0.00116079870997399));
#35245=CARTESIAN_POINT('Ctrl Pts',(-0.185817827209109,0.0169242355148058,
9.8641936611403E-5));
#35246=CARTESIAN_POINT('Ctrl Pts',(-0.203221858920215,0.0166409437466787,
9.11218039920294E-5));
#35247=CARTESIAN_POINT('Ctrl Pts',(-0.220625885580743,0.0163575362327447,
8.39196676156386E-5));
#35248=CARTESIAN_POINT('Ctrl Pts',(-0.238029902001653,0.0160736640759679,
7.73368998092213E-5));
#35249=CARTESIAN_POINT('Ctrl Pts',(-0.185818130580629,0.0168405937503755,
-0.00127155898818726));
#35250=CARTESIAN_POINT('Ctrl Pts',(-0.20322218710562,0.0165814424082619,
-0.00122048351610829));
#35251=CARTESIAN_POINT('Ctrl Pts',(-0.220626248932598,0.0163217805675101,
-0.0011714081373514));
#35252=CARTESIAN_POINT('Ctrl Pts',(-0.238030331796423,0.0160627645050436,
-0.00112492380137579));
#35253=CARTESIAN_POINT('Ctrl Pts',(-0.185819629874682,0.0165908497836556,
-0.00251327778772927));
#35254=CARTESIAN_POINT('Ctrl Pts',(-0.203223673996629,0.0164148787644927,
-0.00249147144795656));
#35255=CARTESIAN_POINT('Ctrl Pts',(-0.220627751907747,0.0162423115134214,
-0.00246930645840148));
#35256=CARTESIAN_POINT('Ctrl Pts',(-0.238031849291733,0.0160723190230807,
-0.00244485415145052));
#35257=CARTESIAN_POINT('Ctrl Pts',(-0.185821321884765,0.016234179304769,
-0.00369798898814236));
#35258=CARTESIAN_POINT('Ctrl Pts',(-0.203225319480993,0.0161450945583953,
-0.00371151425360031));
#35259=CARTESIAN_POINT('Ctrl Pts',(-0.220629323053567,0.0160579626760164,
-0.0037253545768972));
#35260=CARTESIAN_POINT('Ctrl Pts',(-0.238033334942443,0.0159726607261184,
-0.00373864195256771));
#35261=CARTESIAN_POINT('Ctrl Pts',(-0.185823245401148,0.0155679236134438,
-0.00510694903431088));
#35262=CARTESIAN_POINT('Ctrl Pts',(-0.203227224653483,0.0155630775790093,
-0.00518221799309441));
#35263=CARTESIAN_POINT('Ctrl Pts',(-0.220631203569159,0.0155602580016752,
-0.00525755181874107));
#35264=CARTESIAN_POINT('Ctrl Pts',(-0.238035184380882,0.0155591988240479,
-0.00533210507472633));
#35265=CARTESIAN_POINT('Ctrl Pts',(-0.185825309557818,0.0144549166529026,
-0.00659829769408909));
#35266=CARTESIAN_POINT('Ctrl Pts',(-0.203229286524981,0.0145155596341981,
-0.00676015088892623));
#35267=CARTESIAN_POINT('Ctrl Pts',(-0.22063325576454,0.0145775956365756,
-0.00692214625038456));
#35268=CARTESIAN_POINT('Ctrl Pts',(-0.238037222353744,0.0146408934228599,
-0.00708388886226514));
#35269=CARTESIAN_POINT('Ctrl Pts',(-0.185827024933535,0.0130736100782548,
-0.00784141832828519));
#35270=CARTESIAN_POINT('Ctrl Pts',(-0.203231018325486,0.0131627927804585,
-0.00809004931086922));
#35271=CARTESIAN_POINT('Ctrl Pts',(-0.220635004750871,0.0132529981228345,
-0.00833876091410667));
#35272=CARTESIAN_POINT('Ctrl Pts',(-0.238038987871232,0.0133440928006999,
-0.00858734922546909));
#35273=CARTESIAN_POINT('Ctrl Pts',(-0.18582832438757,0.0114765605098063,
-0.00878674958056091));
#35274=CARTESIAN_POINT('Ctrl Pts',(-0.203232338232321,0.0115609317972438,
-0.00910975493295771));
#35275=CARTESIAN_POINT('Ctrl Pts',(-0.220636347717917,0.011645972461393,
-0.00943280869850027));
#35276=CARTESIAN_POINT('Ctrl Pts',(-0.238040354954934,0.011731574352546,
-0.00975583575545302));
#35277=CARTESIAN_POINT('Ctrl Pts',(-0.185829453345315,0.0091451966229997,
-0.0096057242773119));
#35278=CARTESIAN_POINT('Ctrl Pts',(-0.203233491880005,0.00919013323193661,
-0.00999827176177371));
#35279=CARTESIAN_POINT('Ctrl Pts',(-0.220637530309762,0.00923531471374497,
-0.010390817424762));
#35280=CARTESIAN_POINT('Ctrl Pts',(-0.23804156864792,0.00928068353228921,
-0.0107833654056958));
#35281=CARTESIAN_POINT('Ctrl Pts',(-0.185829632293992,0.00601552622584051,
-0.00973743542872093));
#35282=CARTESIAN_POINT('Ctrl Pts',(-0.203233675322875,0.00597352188698778,
-0.0101422781507738));
#35283=CARTESIAN_POINT('Ctrl Pts',(-0.220637719137517,0.00593129183613322,
-0.0105471134497117));
#35284=CARTESIAN_POINT('Ctrl Pts',(-0.238041763362071,0.00588889329790392,
-0.0109519477983446));
#35285=CARTESIAN_POINT('Ctrl Pts',(-0.185828144842012,0.0030739290209801,
-0.00865481883805552));
#35286=CARTESIAN_POINT('Ctrl Pts',(-0.203232153522101,0.0029784477533647,
-0.00896475560878426));
#35287=CARTESIAN_POINT('Ctrl Pts',(-0.22063615670017,0.00288224573504626,
-0.00927474912637149));
#35288=CARTESIAN_POINT('Ctrl Pts',(-0.23804015699596,0.00278543581335185,
-0.00958473005637672));
#35289=CARTESIAN_POINT('Ctrl Pts',(-0.185826082022641,0.00110130832095057,
-0.00715935834428723));
#35290=CARTESIAN_POINT('Ctrl Pts',(-0.203230064435315,0.00102431113527,
-0.00735889669894074));
#35291=CARTESIAN_POINT('Ctrl Pts',(-0.220634039193033,0.000946044449726581,
-0.00755853937500263));
#35292=CARTESIAN_POINT('Ctrl Pts',(-0.238038010705833,0.000866655562235164,
-0.00775795997137017));
#35293=CARTESIAN_POINT('Ctrl Pts',(-0.185824164055499,-0.00013244480670859,
-0.0057658502018965));
#35294=CARTESIAN_POINT('Ctrl Pts',(-0.20322813912978,-0.000160334959886128,
-0.00587671276434198));
#35295=CARTESIAN_POINT('Ctrl Pts',(-0.220632108537853,-0.000189837833944718,
-0.0059877445582653));
#35296=CARTESIAN_POINT('Ctrl Pts',(-0.238036077190852,-0.000220820008254192,
-0.00609839080888522));
#35297=CARTESIAN_POINT('Ctrl Pts',(-0.185822299173595,-0.000912009378582172,
-0.00442360049681092));
#35298=CARTESIAN_POINT('Ctrl Pts',(-0.203226287658242,-0.000866786568362782,
-0.00446783414154759));
#35299=CARTESIAN_POINT('Ctrl Pts',(-0.220630281624252,-0.00082387334949089,
-0.00451207377872994));
#35300=CARTESIAN_POINT('Ctrl Pts',(-0.23803428087264,-0.000782904229550054,
-0.00455527877134414));
#35301=CARTESIAN_POINT('Ctrl Pts',(-0.185820718130017,-0.00137009218103609,
-0.00326760896710645));
#35302=CARTESIAN_POINT('Ctrl Pts',(-0.203224730158278,-0.00125053240292857,
-0.00326719962044019));
#35303=CARTESIAN_POINT('Ctrl Pts',(-0.220628754805288,-0.00113312156821255,
-0.00326706607813972));
#35304=CARTESIAN_POINT('Ctrl Pts',(-0.23803279135031,-0.00101767765869665,
-0.00326612878115765));
#35305=CARTESIAN_POINT('Ctrl Pts',(-0.185819647933685,-0.00158153457958364,
-0.00252531449976026));
#35306=CARTESIAN_POINT('Ctrl Pts',(-0.203223692052988,-0.00140575636354931,
-0.00250567473614365));
#35307=CARTESIAN_POINT('Ctrl Pts',(-0.220627772291069,-0.00123370234183487,
-0.00248543365897305));
#35308=CARTESIAN_POINT('Ctrl Pts',(-0.238031871675392,-0.001064293369006,
-0.00246259728183289));
#35309=CARTESIAN_POINT('Ctrl Pts',(-0.185818880874262,-0.00171069848643351,
-0.00190682671492207));
#35310=CARTESIAN_POINT('Ctrl Pts',(-0.203222934035982,-0.0014938099322336,
-0.00186885153402852));
#35311=CARTESIAN_POINT('Ctrl Pts',(-0.220627006269333,-0.00127812856598612,
-0.00183193647922556));
#35312=CARTESIAN_POINT('Ctrl Pts',(-0.238031099947143,-0.00106408777175675,
-0.00179531451994465));
#35313=CARTESIAN_POINT('Ctrl Pts',(-0.185818335405171,-0.0018157482831674,
-0.00126613919912989));
#35314=CARTESIAN_POINT('Ctrl Pts',(-0.203222383696684,-0.00156635979742609,
-0.00122992540382135));
#35315=CARTESIAN_POINT('Ctrl Pts',(-0.220626440719173,-0.00131735881546124,
-0.00119476377996408));
#35316=CARTESIAN_POINT('Ctrl Pts',(-0.238030512988314,-0.00106912762331005,
-0.00116079872610497));
#35317=CARTESIAN_POINT('Ctrl Pts',(-0.185817827208834,-0.00192423551004945,
-9.86419358357781E-5));
#35318=CARTESIAN_POINT('Ctrl Pts',(-0.203221858919953,-0.00164094372766557,
-9.11218007194661E-5));
#35319=CARTESIAN_POINT('Ctrl Pts',(-0.220625885580502,-0.00135753619911081,
-8.39196619480522E-5));
#35320=CARTESIAN_POINT('Ctrl Pts',(-0.238029902001436,-0.00107366402718548,
-7.73368926939811E-5));
#35321=CARTESIAN_POINT('Ctrl Pts',(-0.185818130581901,-0.00184059377323484,
0.00127155899038818));
#35322=CARTESIAN_POINT('Ctrl Pts',(-0.20322218710682,-0.00158144249928501,
0.00122048352511737));
#35323=CARTESIAN_POINT('Ctrl Pts',(-0.220626248933645,-0.00132178072462663,
0.0011714081546043));
#35324=CARTESIAN_POINT('Ctrl Pts',(-0.238030331797288,-0.00106276472807202,
0.00112492383001885));
#35325=CARTESIAN_POINT('Ctrl Pts',(-0.185819629872525,-0.00159084974486086,
0.00251327778358106));
#35326=CARTESIAN_POINT('Ctrl Pts',(-0.203223673994595,-0.00141487860996912,
0.00249147143135548));
#35327=CARTESIAN_POINT('Ctrl Pts',(-0.220627751905974,-0.00124231124688325,
0.00246930642685937));
#35328=CARTESIAN_POINT('Ctrl Pts',(-0.238031849290273,-0.00107231864497727,
0.00244485409969644));
#35329=CARTESIAN_POINT('Ctrl Pts',(-0.185821321898498,-0.00123417951568875,
0.00369798917224086));
#35330=CARTESIAN_POINT('Ctrl Pts',(-0.203225319494204,-0.00114509540859564,
0.003711514992569));
#35331=CARTESIAN_POINT('Ctrl Pts',(-0.22062932306665,-0.00105796426044417,
0.00372535589828007));
#35332=CARTESIAN_POINT('Ctrl Pts',(-0.238033334955726,-0.000972663126262614,
0.00373864380762799));
#35333=CARTESIAN_POINT('Ctrl Pts',(-0.185823245436368,-0.000567924396732498,
0.00510694905821607));
#35334=CARTESIAN_POINT('Ctrl Pts',(-0.203227224690427,-0.000563080693363035,
0.00518221807967137));
#35335=CARTESIAN_POINT('Ctrl Pts',(-0.220631203607128,-0.000560263335972913,
0.00525755189961067));
#35336=CARTESIAN_POINT('Ctrl Pts',(-0.238035184419129,-0.000559206262722732,
0.00533210518716677));
#35337=CARTESIAN_POINT('Ctrl Pts',(-0.185825309451763,0.000545085685742881,
0.00659829745055551));
#35338=CARTESIAN_POINT('Ctrl Pts',(-0.203229286420574,0.000484449699432902,
0.00676014989093362));
#35339=CARTESIAN_POINT('Ctrl Pts',(-0.220633255665466,0.000422420785569872,
0.00692214425104443));
#35340=CARTESIAN_POINT('Ctrl Pts',(-0.238037222262465,0.000359130275923251,
0.00708388576133197));
#35341=CARTESIAN_POINT('Ctrl Pts',(-0.18582702479622,0.00192639486310074,
0.00784141870119505));
#35342=CARTESIAN_POINT('Ctrl Pts',(-0.203231018176613,0.00183722692142162,
0.00809005081566443));
#35343=CARTESIAN_POINT('Ctrl Pts',(-0.22063500458984,0.00174703627304292,
0.00833876365528797));
#35344=CARTESIAN_POINT('Ctrl Pts',(-0.238038987697963,0.00165595618969436,
0.00858735323957588));
#35345=CARTESIAN_POINT('Ctrl Pts',(-0.185828324413572,0.00352344076961579,
0.00878675040966002));
#35346=CARTESIAN_POINT('Ctrl Pts',(-0.203232338254504,0.00343907331273139,
0.00910975824932868));
#35347=CARTESIAN_POINT('Ctrl Pts',(-0.220636347734676,0.00335403651878359,
0.00943281459138894));
#35348=CARTESIAN_POINT('Ctrl Pts',(-0.238040354964937,0.00326843848901562,
0.00975584429234039));
#35349=CARTESIAN_POINT('Ctrl Pts',(-0.185829453384424,0.00585480099283502,
0.00960572462550227));
#35350=CARTESIAN_POINT('Ctrl Pts',(-0.203233491922009,0.00580985725942693,
0.00999827314311295));
#35351=CARTESIAN_POINT('Ctrl Pts',(-0.220637530355488,0.00576466867020715,
0.0103908197967745));
#35352=CARTESIAN_POINT('Ctrl Pts',(-0.238041568698001,0.00571929278241239,
0.01078336873748));
#35353=CARTESIAN_POINT('Ctrl Pts',(-0.185829632324535,0.00898447703279034,
0.00973743551044517));
#35354=CARTESIAN_POINT('Ctrl Pts',(-0.20323367535712,0.00902649110858287,
0.0101422784667701));
#35355=CARTESIAN_POINT('Ctrl Pts',(-0.220637719176512,0.00906873086433049,
0.0105471139309657));
#35356=CARTESIAN_POINT('Ctrl Pts',(-0.238041763406542,0.00911113903768637,
0.0109519484055942));
#35357=CARTESIAN_POINT('Ctrl Pts',(-0.185828144821879,0.0119260676124901,
0.00865481978154805));
#35358=CARTESIAN_POINT('Ctrl Pts',(-0.203232153491178,0.0120215388163693,
0.00896475940006844));
#35359=CARTESIAN_POINT('Ctrl Pts',(-0.220636156655006,0.0121177307814799,
0.00927475599174944));
#35360=CARTESIAN_POINT('Ctrl Pts',(-0.238040156934043,0.0122145307595023,
0.00958474013175701));
#35361=CARTESIAN_POINT('Ctrl Pts',(-0.185826081864447,0.0138986875060143,
0.0071593582727713));
#35362=CARTESIAN_POINT('Ctrl Pts',(-0.203230064272376,0.0139756722252048,
0.00735889640414339));
#35363=CARTESIAN_POINT('Ctrl Pts',(-0.22063403902823,0.0140539264607635,
0.00755853873522353));
#35364=CARTESIAN_POINT('Ctrl Pts',(-0.238038010541502,0.0141333028562059,
0.00775795890451245));
#35365=CARTESIAN_POINT('Ctrl Pts',(-0.185824164045733,0.0151324448001649,
0.00576585000582876));
#35366=CARTESIAN_POINT('Ctrl Pts',(-0.203228139124408,0.0151603349181088,
0.00587671195695743));
#35367=CARTESIAN_POINT('Ctrl Pts',(-0.220632108538343,0.0151898375748212,
0.00598774292639455));
#35368=CARTESIAN_POINT('Ctrl Pts',(-0.238036077197705,0.0152208192897305,
0.00609838833446442));
#35369=CARTESIAN_POINT('Ctrl Pts',(-0.185822299200829,0.01591200987427,
0.00442360064358258));
#35370=CARTESIAN_POINT('Ctrl Pts',(-0.203226287685109,0.0158667885469009,
0.00446783472845091));
#35371=CARTESIAN_POINT('Ctrl Pts',(-0.220630281650178,0.0158238768216512,
0.00451207481602829));
#35372=CARTESIAN_POINT('Ctrl Pts',(-0.238034280897302,0.0157829092105071,
0.00455528026393975));
#35373=CARTESIAN_POINT('Ctrl Pts',(-0.185820718137045,0.0163700922862437,
0.00326760909611432));
#35374=CARTESIAN_POINT('Ctrl Pts',(-0.203224730165169,0.0162505328296095,
0.00326720013800919));
#35375=CARTESIAN_POINT('Ctrl Pts',(-0.220628754812585,0.0161331223929292,
0.00326706699899929));
#35376=CARTESIAN_POINT('Ctrl Pts',(-0.238032791358368,0.016017678941859,
0.00326613005920909));
#35377=CARTESIAN_POINT('Ctrl Pts',(-0.18581986197366,0.0165392461104783,
0.00267377340626184));
#35378=CARTESIAN_POINT('Ctrl Pts',(-0.203223899674741,0.0163747116144059,
0.00265797976538081));
#35379=CARTESIAN_POINT('Ctrl Pts',(-0.220627968794648,0.0162135862702056,
0.00264176023600675));
#35380=CARTESIAN_POINT('Ctrl Pts',(-0.238032055611188,0.016054970356251,
0.00262330371106081));
#35381=CARTESIAN_POINT('Ctrl Pts',(-0.185819463593633,0.0166104930553049,
0.00236863820262676));
#35382=CARTESIAN_POINT('Ctrl Pts',(-0.203223508587672,0.0164247592890707,
0.00234416866113263));
#35383=CARTESIAN_POINT('Ctrl Pts',(-0.220627582451438,0.0162418056983084,
0.00231971009381821));
#35384=CARTESIAN_POINT('Ctrl Pts',(-0.238031675744303,0.0160611171225611,
0.00229373846137714));
#35385=CARTESIAN_POINT('',(-0.230843542066567,0.0161181286545946,-0.00261043832732274));
#35386=CARTESIAN_POINT('Origin',(-0.233966934007412,0.0158592789729621,
3.09238363249698E-10));
#35387=CARTESIAN_POINT('',(-0.237700712870106,0.0075106460066284,-0.0107797928880335));
#35388=CARTESIAN_POINT('Ctrl Pts',(-0.230843549406418,0.0161191164318998,
-0.00261050690091829));
#35389=CARTESIAN_POINT('Ctrl Pts',(-0.231651983552228,0.0160415721496965,
-0.00357365221582349));
#35390=CARTESIAN_POINT('Ctrl Pts',(-0.232444275696972,0.0158161744526218,
-0.00451766730635352));
#35391=CARTESIAN_POINT('Ctrl Pts',(-0.233207651413396,0.0154317497833547,
-0.00542716549495472));
#35392=CARTESIAN_POINT('Ctrl Pts',(-0.233971028171898,0.015047324589313,
-0.00633666492510352));
#35393=CARTESIAN_POINT('Ctrl Pts',(-0.234705524570036,0.0145039610841376,
-0.00721168853739024));
#35394=CARTESIAN_POINT('Ctrl Pts',(-0.235365783247194,0.0137804475678366,
-0.00799824442316078));
#35395=CARTESIAN_POINT('Ctrl Pts',(-0.235367844562095,0.0137781887725434,
-0.00800070003551994));
#35396=CARTESIAN_POINT('Ctrl Pts',(-0.235369905152796,0.0137759282229903,
-0.00800315478243444));
#35397=CARTESIAN_POINT('Ctrl Pts',(-0.235371965017888,0.0137736659185172,
-0.0080056086622658));
#35398=CARTESIAN_POINT('Ctrl Pts',(-0.235699802297696,0.013413609453079,
-0.00839615525278972));
#35399=CARTESIAN_POINT('Ctrl Pts',(-0.236009265872864,0.0130091028997178,
-0.00876475090758743));
#35400=CARTESIAN_POINT('Ctrl Pts',(-0.236288883258456,0.012561367000027,
-0.00909784263196301));
#35401=CARTESIAN_POINT('Ctrl Pts',(-0.236570257534211,0.0121108178890046,
-0.00943302723612366));
#35402=CARTESIAN_POINT('Ctrl Pts',(-0.236821407837358,0.011616490160412,
-0.00973226987547397));
#35403=CARTESIAN_POINT('Ctrl Pts',(-0.237030704738135,0.0110795136094463,
-0.00998162692863499));
#35404=CARTESIAN_POINT('Ctrl Pts',(-0.237240001638912,0.0105425370584806,
-0.010230983981796));
#35405=CARTESIAN_POINT('Ctrl Pts',(-0.237407392556333,0.00996285229092137,
-0.0104303849821952));
#35406=CARTESIAN_POINT('Ctrl Pts',(-0.237522490752224,0.00936122795465865,
-0.0105674930798237));
#35407=CARTESIAN_POINT('Ctrl Pts',(-0.237637588948116,0.00875960361839593,
-0.0107046011774521));
#35408=CARTESIAN_POINT('Ctrl Pts',(-0.237700401438083,0.00813606422858096,
-0.0107794203282436));
#35409=CARTESIAN_POINT('Ctrl Pts',(-0.237700712551084,0.00751133792318635,
-0.0107797925062651));
#35410=CARTESIAN_POINT('',(-0.230843542079837,-0.00111813185800299,-0.00261043853789162));
#35411=CARTESIAN_POINT('Ctrl Pts',(-0.237700712870106,0.0075106460066284,
-0.0107797928880335));
#35412=CARTESIAN_POINT('Ctrl Pts',(-0.237700977736204,0.00688614944423556,
-0.0107801099748839));
#35413=CARTESIAN_POINT('Ctrl Pts',(-0.237638789092914,0.006260444451203,
-0.0107060307146087));
#35414=CARTESIAN_POINT('Ctrl Pts',(-0.237524351321969,0.0056561909426634,
-0.0105697092990888));
#35415=CARTESIAN_POINT('Ctrl Pts',(-0.237409871286876,0.0050517142712691,
-0.0104333375373553));
#35416=CARTESIAN_POINT('Ctrl Pts',(-0.237243099478524,0.00446872868422436,
-0.0102346738447992));
#35417=CARTESIAN_POINT('Ctrl Pts',(-0.23703442323106,0.00392995420914097,
-0.00998606057911376));
#35418=CARTESIAN_POINT('Ctrl Pts',(-0.236825746983597,0.00339117973405756,
-0.0097374473134283));
#35419=CARTESIAN_POINT('Ctrl Pts',(-0.236575219550393,0.00289655692010007,
-0.00943895248021973));
#35420=CARTESIAN_POINT('Ctrl Pts',(-0.236294506432514,0.00244619039703509,
-0.00910455462484356));
#35421=CARTESIAN_POINT('Ctrl Pts',(-0.236015370943784,0.00199835496820744,
-0.0087720361109401));
#35422=CARTESIAN_POINT('Ctrl Pts',(-0.235706389506389,0.00159427631684454,
-0.00840400801450611));
#35423=CARTESIAN_POINT('Ctrl Pts',(-0.235379088265152,0.00123416570953253,
-0.00801409801864759));
#35424=CARTESIAN_POINT('Ctrl Pts',(-0.23537723841087,0.00123213042195969,
-0.00801189430969545));
#35425=CARTESIAN_POINT('Ctrl Pts',(-0.2353753879712,0.00123009653891891,
-0.0080096899013831));
#35426=CARTESIAN_POINT('Ctrl Pts',(-0.235373536947083,0.0012280640599786,
-0.00800748479480728));
#35427=CARTESIAN_POINT('Ctrl Pts',(-0.234714818450409,0.000504771769989926,
-0.00722276001697017));
#35428=CARTESIAN_POINT('Ctrl Pts',(-0.233982182394368,-4.06098583481195E-5,
-0.00634993382838675));
#35429=CARTESIAN_POINT('Ctrl Pts',(-0.233216597089855,-0.00042724483431046,
-0.00543781234703487));
#35430=CARTESIAN_POINT('Ctrl Pts',(-0.232451012812611,-0.00081387929148324,
-0.00452569208957409));
#35431=CARTESIAN_POINT('Ctrl Pts',(-0.231652435772805,-0.0010415287758554,
-0.00357419097857274));
#35432=CARTESIAN_POINT('Ctrl Pts',(-0.230843549351773,-0.00111911643714708,
-0.00261050683581516));
#35433=CARTESIAN_POINT('',(-0.230843542065975,-0.00111812869478135,0.00261043842873682));
#35434=CARTESIAN_POINT('Origin',(-0.23396693400794,-0.000859278972356703,
-2.03117108132922E-10));
#35435=CARTESIAN_POINT('Ctrl Pts',(-0.230843549407105,-0.0011191166041277,
0.0026105070108692));
#35436=CARTESIAN_POINT('Ctrl Pts',(-0.231651983097731,-0.00104157341320291,
0.00357365206993173));
#35437=CARTESIAN_POINT('Ctrl Pts',(-0.232444276388805,-0.000816181869474475,
0.0045176677295523));
#35438=CARTESIAN_POINT('Ctrl Pts',(-0.233207649052068,-0.000431751373454661,
0.00542716208151464));
#35439=CARTESIAN_POINT('Ctrl Pts',(-0.233971022757487,-4.73203526106414E-5,
0.00633665767511794));
#35440=CARTESIAN_POINT('Ctrl Pts',(-0.23470551192207,0.00049606094558371,
0.0072116730703037));
#35441=CARTESIAN_POINT('Ctrl Pts',(-0.235365772451735,0.00121957511810953,
0.00799823141159865));
#35442=CARTESIAN_POINT('Ctrl Pts',(-0.23536783372932,0.00122183386822287,
0.00800068698027997));
#35443=CARTESIAN_POINT('Ctrl Pts',(-0.235369894282823,0.00122409437235532,
0.00800314168365631));
#35444=CARTESIAN_POINT('Ctrl Pts',(-0.235371954110837,0.00122635663116605,
0.00800559552008976));
#35445=CARTESIAN_POINT('Ctrl Pts',(-0.235699792387272,0.00158641340486399,
0.00839614342080721));
#35446=CARTESIAN_POINT('Ctrl Pts',(-0.236009259211335,0.00199091601206364,
0.0087647430201395));
#35447=CARTESIAN_POINT('Ctrl Pts',(-0.236288879915149,0.00243864717211577,
0.00909783876953468));
#35448=CARTESIAN_POINT('Ctrl Pts',(-0.236570257493009,0.00288919145452985,
0.00943302737996994));
#35449=CARTESIAN_POINT('Ctrl Pts',(-0.236821411175091,0.00338351354138113,
0.00973227411776468));
#35450=CARTESIAN_POINT('Ctrl Pts',(-0.237030709359485,0.00392048719339499,
0.00998163270096488));
#35451=CARTESIAN_POINT('Ctrl Pts',(-0.237240007543878,0.00445746084540883,
0.0102309912841651));
#35452=CARTESIAN_POINT('Ctrl Pts',(-0.237407397613687,0.00503714549261125,
0.0104303912055088));
#35453=CARTESIAN_POINT('Ctrl Pts',(-0.237522494588081,0.00563877088560149,
0.0105674977840015));
#35454=CARTESIAN_POINT('Ctrl Pts',(-0.237637591562474,0.00624039627859174,
0.0107046043624942));
#35455=CARTESIAN_POINT('Ctrl Pts',(-0.237700402455248,0.00686393789297539,
0.0107794215577471));
#35456=CARTESIAN_POINT('Ctrl Pts',(-0.237700713436944,0.00748866602213257,
0.010779793575244));
#35457=CARTESIAN_POINT('Ctrl Pts',(-0.237700864903606,0.00779294593887606,
0.0107799747699873));
#35458=CARTESIAN_POINT('Ctrl Pts',(-0.237686190487506,0.00809751515955963,
0.0107624949752251));
#35459=CARTESIAN_POINT('Ctrl Pts',(-0.237657867810474,0.00839975141101414,
0.0107287568273012));
#35460=CARTESIAN_POINT('',(-0.186146181811502,0.00666198522174072,0.00957679076397076));
#35461=CARTESIAN_POINT('Origin',(-0.187938685420677,0.00749971564796731,
0.000572374571681731));
#35462=CARTESIAN_POINT('',(-0.192201188841356,-0.000241557430167074,0.00554550626187204));
#35463=CARTESIAN_POINT('Ctrl Pts',(-0.186146181811502,0.00666198522174072,
0.00957679076397076));
#35464=CARTESIAN_POINT('Ctrl Pts',(-0.186240918660984,0.00577359340919673,
0.00949869141429598));
#35465=CARTESIAN_POINT('Ctrl Pts',(-0.186729216300464,0.00408141660355003,
0.00909746875116488));
#35466=CARTESIAN_POINT('Ctrl Pts',(-0.188122925906735,0.00204059109517293,
0.00799351103237768));
#35467=CARTESIAN_POINT('Ctrl Pts',(-0.189934445945795,0.000579265164406154,
0.00668849997305698));
#35468=CARTESIAN_POINT('Ctrl Pts',(-0.191383442893151,-3.83064418099935E-5,
0.00585331050437291));
#35469=CARTESIAN_POINT('Ctrl Pts',(-0.192201188668274,-0.000241594090485781,
0.00554556725774743));
#35470=CARTESIAN_POINT('',(-0.215000291561739,-0.000324149940950663,0.00555319305328791));
#35471=CARTESIAN_POINT('Ctrl Pts',(-0.215000291205181,-0.0003242242949523,
0.00555305246006235));
#35472=CARTESIAN_POINT('Ctrl Pts',(-0.213932608980925,-0.000320905181478583,
0.00555269239176458));
#35473=CARTESIAN_POINT('Ctrl Pts',(-0.212894399737908,-0.000317606952698171,
0.00555234073581887));
#35474=CARTESIAN_POINT('Ctrl Pts',(-0.211885533644697,-0.000314338717420239,
0.00555199786657978));
#35475=CARTESIAN_POINT('Ctrl Pts',(-0.210876667461984,-0.000311070481852365,
0.00555165499731028));
#35476=CARTESIAN_POINT('Ctrl Pts',(-0.209897144434309,-0.000307832227897103,
0.00555132091066889));
#35477=CARTESIAN_POINT('Ctrl Pts',(-0.208947353979719,-0.000304634161730677,
0.00555099707706335));
#35478=CARTESIAN_POINT('Ctrl Pts',(-0.208472458752424,-0.000303035128647463,
0.00555083516026057));
#35479=CARTESIAN_POINT('Ctrl Pts',(-0.208004996668339,-0.000301446149282922,
0.00555067581488556));
#35480=CARTESIAN_POINT('Ctrl Pts',(-0.207544480927504,-0.000299866555274974,
0.00555051916679648));
#35481=CARTESIAN_POINT('Ctrl Pts',(-0.207083965186669,-0.000298286961267027,
0.00555036251870738));
#35482=CARTESIAN_POINT('Ctrl Pts',(-0.206630395789221,-0.000296716714222072,
0.0055502085465108));
#35483=CARTESIAN_POINT('Ctrl Pts',(-0.206185752375027,-0.000295163842050715,
0.00555005809144));
#35484=CARTESIAN_POINT('Ctrl Pts',(-0.205741108960833,-0.000293610969879358,
0.0055499076363692));
#35485=CARTESIAN_POINT('Ctrl Pts',(-0.205305391529366,-0.000292075614881537,
0.00554976078032587));
#35486=CARTESIAN_POINT('Ctrl Pts',(-0.204871168306577,-0.000290532039648846,
0.00554961555720526));
#35487=CARTESIAN_POINT('Ctrl Pts',(-0.204654056695182,-0.0002897602520325,
0.00554954294564495));
#35488=CARTESIAN_POINT('Ctrl Pts',(-0.204437318636325,-0.000288986311853899,
0.00554947068530159));
#35489=CARTESIAN_POINT('Ctrl Pts',(-0.20423043044895,-0.000288244541876076,
0.00554940183661774));
#35490=CARTESIAN_POINT('Ctrl Pts',(-0.204023542261574,-0.000287502771898252,
0.00554933298793389));
#35491=CARTESIAN_POINT('Ctrl Pts',(-0.203826503944328,-0.000286793520252714,
0.00554926775793827));
#35492=CARTESIAN_POINT('Ctrl Pts',(-0.203600728706342,-0.00028597691500919,
0.00554919348805181));
#35493=CARTESIAN_POINT('Ctrl Pts',(-0.203374953468356,-0.000285160309765666,
0.00554911921816535));
#35494=CARTESIAN_POINT('Ctrl Pts',(-0.20312044131193,-0.00028423576377125,
0.00554903555688988));
#35495=CARTESIAN_POINT('Ctrl Pts',(-0.202874057457924,-0.000283336172872535,
0.00554895461009971));
#35496=CARTESIAN_POINT('Ctrl Pts',(-0.202627673603918,-0.000282436581973819,
0.00554887366330954));
#35497=CARTESIAN_POINT('Ctrl Pts',(-0.202389418050814,-0.000281562329560916,
0.00554879566253169));
#35498=CARTESIAN_POINT('Ctrl Pts',(-0.202150286345955,-0.000280680803074264,
0.0055487175181587));
#35499=CARTESIAN_POINT('Ctrl Pts',(-0.201672022936239,-0.000278917750100961,
0.00554856122941273));
#35500=CARTESIAN_POINT('Ctrl Pts',(-0.201190254921159,-0.000277125193128902,
0.00554840411650478));
#35501=CARTESIAN_POINT('Ctrl Pts',(-0.200711444532909,-0.000275326860415499,
0.00554824832785496));
#35502=CARTESIAN_POINT('Ctrl Pts',(-0.199753823756409,-0.00027173019498869,
0.00554793675055534));
#35503=CARTESIAN_POINT('Ctrl Pts',(-0.198808033484689,-0.000268111032540832,
0.00554763085059868));
#35504=CARTESIAN_POINT('Ctrl Pts',(-0.197868562559789,-0.000264450677025733,
0.00554732800782794));
#35505=CARTESIAN_POINT('Ctrl Pts',(-0.196929091634889,-0.000260790321510633,
0.00554702516505721));
#35506=CARTESIAN_POINT('Ctrl Pts',(-0.195995940054903,-0.0002570891780411,
0.00554672565571742));
#35507=CARTESIAN_POINT('Ctrl Pts',(-0.195051666862503,-0.000253275770992353,
0.00554642287911516));
#35508=CARTESIAN_POINT('Ctrl Pts',(-0.194107393750835,-0.000249462364269639,
0.00554612010253878));
#35509=CARTESIAN_POINT('Ctrl Pts',(-0.193151999033877,-0.000245535583896571,
0.00554581330127274));
#35510=CARTESIAN_POINT('Ctrl Pts',(-0.192201188841356,-0.000241557430167074,
0.00554550626187204));
#35511=CARTESIAN_POINT('',(-0.21500029174882,-0.000324094014707694,-0.00555316364009558));
#35512=CARTESIAN_POINT('Ctrl Pts',(-0.215000291561739,-0.000324149940950663,
0.00555319305328791));
#35513=CARTESIAN_POINT('Ctrl Pts',(-0.215668740091759,-0.000326228214530295,
0.00555341885793155));
#35514=CARTESIAN_POINT('Ctrl Pts',(-0.216324728842753,-0.000393731830372502,
0.00543467425660531));
#35515=CARTESIAN_POINT('Ctrl Pts',(-0.216937359547008,-0.000498389548785778,
0.00521197222380067));
#35516=CARTESIAN_POINT('Ctrl Pts',(-0.217007385782656,-0.000510352360967931,
0.00518651645588009));
#35517=CARTESIAN_POINT('Ctrl Pts',(-0.217076845515466,-0.000522776977352358,
0.00515969404947732));
#35518=CARTESIAN_POINT('Ctrl Pts',(-0.217145692593967,-0.000535604694262252,
0.00513152356702724));
#35519=CARTESIAN_POINT('Ctrl Pts',(-0.217816854468214,-0.000660656834613602,
0.00485690111083667));
#35520=CARTESIAN_POINT('Ctrl Pts',(-0.218429805272727,-0.000824611483592641,
0.00445372704704561));
#35521=CARTESIAN_POINT('Ctrl Pts',(-0.218946402817707,-0.000965073719826547,
0.00394589026024182));
#35522=CARTESIAN_POINT('Ctrl Pts',(-0.21911757141393,-0.00101161425032699,
0.00377762443948319));
#35523=CARTESIAN_POINT('Ctrl Pts',(-0.219278158884941,-0.00105556042755966,
0.00359780043100863));
#35524=CARTESIAN_POINT('Ctrl Pts',(-0.219426704704914,-0.00109449434193882,
0.00340810662225617));
#35525=CARTESIAN_POINT('Ctrl Pts',(-0.219502319179551,-0.00111431292371979,
0.00331154653262599));
#35526=CARTESIAN_POINT('Ctrl Pts',(-0.219574813505332,-0.00113283089738519,
0.00321243800056172));
#35527=CARTESIAN_POINT('Ctrl Pts',(-0.219643995497907,-0.00114993043982612,
0.00311087728876615));
#35528=CARTESIAN_POINT('Ctrl Pts',(-0.219784412586894,-0.0011846369853185,
0.00290474186284185));
#35529=CARTESIAN_POINT('Ctrl Pts',(-0.219911192740882,-0.00121336031308103,
0.00268891197041315));
#35530=CARTESIAN_POINT('Ctrl Pts',(-0.220022736935838,-0.00123594984514704,
0.00246439654593185));
#35531=CARTESIAN_POINT('Ctrl Pts',(-0.220074112524313,-0.00124635424587568,
0.00236098809819431));
#35532=CARTESIAN_POINT('Ctrl Pts',(-0.220122255964863,-0.00125547047269016,
0.00225573024477926));
#35533=CARTESIAN_POINT('Ctrl Pts',(-0.220167013742202,-0.00126354003322303,
0.00214910011923536));
#35534=CARTESIAN_POINT('Ctrl Pts',(-0.220255304274326,-0.00127945829002233,
0.00193875833989861));
#35535=CARTESIAN_POINT('Ctrl Pts',(-0.220330419857194,-0.00129139212065717,
0.00172100899924843));
#35536=CARTESIAN_POINT('Ctrl Pts',(-0.220392020117299,-0.00130178661929758,
0.00150014969597866));
#35537=CARTESIAN_POINT('Ctrl Pts',(-0.220528474000989,-0.00132481200435377,
0.00101091296826799));
#35538=CARTESIAN_POINT('Ctrl Pts',(-0.220598617810777,-0.001340773537683,
0.000507277145745172));
#35539=CARTESIAN_POINT('Ctrl Pts',(-0.220598427190772,-0.00134207975133048,
-7.52537007378193E-7));
#35540=CARTESIAN_POINT('Ctrl Pts',(-0.220598376879732,-0.00134242450511075,
-0.000134838682836322));
#35541=CARTESIAN_POINT('Ctrl Pts',(-0.22059342260227,-0.00134174640947658,
-0.000268914120462707));
#35542=CARTESIAN_POINT('Ctrl Pts',(-0.220583640920972,-0.00133993652035355,
-0.000402703728332918));
#35543=CARTESIAN_POINT('Ctrl Pts',(-0.220560148143331,-0.0013355896886151,
-0.000724027784246587));
#35544=CARTESIAN_POINT('Ctrl Pts',(-0.22050881067424,-0.00132468740862665,
-0.00104372328931524));
#35545=CARTESIAN_POINT('Ctrl Pts',(-0.22043068209847,-0.00130920789017929,
-0.00135493667140239));
#35546=CARTESIAN_POINT('Ctrl Pts',(-0.220390026640352,-0.00130115287435809,
-0.00151688154875802));
#35547=CARTESIAN_POINT('Ctrl Pts',(-0.220342116549357,-0.00129187744466456,
-0.00167656205544119));
#35548=CARTESIAN_POINT('Ctrl Pts',(-0.220287103460061,-0.00128219907898819,
-0.00183469943029004));
#35549=CARTESIAN_POINT('Ctrl Pts',(-0.220249785986982,-0.00127563387504865,
-0.00194197003268941));
#35550=CARTESIAN_POINT('Ctrl Pts',(-0.220209199956055,-0.00126886559305341,
-0.00204849177962379));
#35551=CARTESIAN_POINT('Ctrl Pts',(-0.220165384850271,-0.00126128757747624,
-0.00215277905196633));
#35552=CARTESIAN_POINT('Ctrl Pts',(-0.220141806611008,-0.0012572096171193,
-0.00220889920083847));
#35553=CARTESIAN_POINT('Ctrl Pts',(-0.22011729288104,-0.00125287335201092,
-0.00226472495715461));
#35554=CARTESIAN_POINT('Ctrl Pts',(-0.22009186434136,-0.0012481906745658,
-0.0023200354792529));
#35555=CARTESIAN_POINT('Ctrl Pts',(-0.219964032067859,-0.00122465030176397,
-0.00259808800909705));
#35556=CARTESIAN_POINT('Ctrl Pts',(-0.219813080791229,-0.00119207341516924,
-0.00286323534620003));
#35557=CARTESIAN_POINT('Ctrl Pts',(-0.219641753502741,-0.00114977266145016,
-0.00311424190666308));
#35558=CARTESIAN_POINT('Ctrl Pts',(-0.219606803653757,-0.00114114353431307,
-0.00316544590025774));
#35559=CARTESIAN_POINT('Ctrl Pts',(-0.219571005532134,-0.00113213027555365,
-0.00321601272097191));
#35560=CARTESIAN_POINT('Ctrl Pts',(-0.21953438720127,-0.0011227418846443,
-0.00326596039771834));
#35561=CARTESIAN_POINT('Ctrl Pts',(-0.219355791593764,-0.00107695264907934,
-0.00350956614001746));
#35562=CARTESIAN_POINT('Ctrl Pts',(-0.219157685440798,-0.00102227590413239,
-0.00373830700747762));
#35563=CARTESIAN_POINT('Ctrl Pts',(-0.218943331186757,-0.000963766372682074,
-0.00394877174088596));
#35564=CARTESIAN_POINT('Ctrl Pts',(-0.218858026839138,-0.000940481939012855,
-0.00403252821616926));
#35565=CARTESIAN_POINT('Ctrl Pts',(-0.218770149734348,-0.000916567399260997,
-0.00411347430382928));
#35566=CARTESIAN_POINT('Ctrl Pts',(-0.218679855692286,-0.000892327992985571,
-0.00419142830140832));
#35567=CARTESIAN_POINT('Ctrl Pts',(-0.218223323108185,-0.000769771969006836,
-0.00458556881326656));
#35568=CARTESIAN_POINT('Ctrl Pts',(-0.217705003690594,-0.000639141842020944,
-0.00490281622798988));
#35569=CARTESIAN_POINT('Ctrl Pts',(-0.21714503543376,-0.000535117611044864,
-0.00513162917727141));
#35570=CARTESIAN_POINT('Ctrl Pts',(-0.216474315446649,-0.00041051924317671,
-0.00540569724545193));
#35571=CARTESIAN_POINT('Ctrl Pts',(-0.215743833588139,-0.000326403425118811,
-0.00555341379930925));
#35572=CARTESIAN_POINT('Ctrl Pts',(-0.21500029174882,-0.000324094014707694,
-0.00555316364009558));
#35573=CARTESIAN_POINT('',(-0.192201191756381,-0.000241534711908781,-0.00554549092202007));
#35574=CARTESIAN_POINT('Ctrl Pts',(-0.192201191756381,-0.000241534711908781,
-0.00554549092202007));
#35575=CARTESIAN_POINT('Ctrl Pts',(-0.192678594805748,-0.000243532238599143,
-0.00554564514895133));
#35576=CARTESIAN_POINT('Ctrl Pts',(-0.193156777591037,-0.000245515257083601,
-0.00554579917339835));
#35577=CARTESIAN_POINT('Ctrl Pts',(-0.193630540727713,-0.000247462867484684,
-0.00554595129683631));
#35578=CARTESIAN_POINT('Ctrl Pts',(-0.194104303945115,-0.000249410478217631,
-0.0055461034203002));
#35579=CARTESIAN_POINT('Ctrl Pts',(-0.194573647510702,-0.000251323030553919,
-0.00554625388646444));
#35580=CARTESIAN_POINT('Ctrl Pts',(-0.195054169579703,-0.000253263283285137,
-0.00554640817237499));
#35581=CARTESIAN_POINT('Ctrl Pts',(-0.195294430614203,-0.000254233409650747,
-0.00554648531533026));
#35582=CARTESIAN_POINT('Ctrl Pts',(-0.195537486275633,-0.000255210231968368,
-0.00554656325712504));
#35583=CARTESIAN_POINT('Ctrl Pts',(-0.195763838864246,-0.000256116093067966,
-0.00554663583769404));
#35584=CARTESIAN_POINT('Ctrl Pts',(-0.195990191452859,-0.000257021954167565,
-0.00554670841826303));
#35585=CARTESIAN_POINT('Ctrl Pts',(-0.19619984096725,-0.000257857156228515,
-0.0055467758417085));
#35586=CARTESIAN_POINT('Ctrl Pts',(-0.196410720680054,-0.000258693884580058,
-0.00554684397646886));
#35587=CARTESIAN_POINT('Ctrl Pts',(-0.196832480105662,-0.000260367341283143,
-0.00554698024598957));
#35588=CARTESIAN_POINT('Ctrl Pts',(-0.197259160327546,-0.00026204633453472,
-0.00554711897819944));
#35589=CARTESIAN_POINT('Ctrl Pts',(-0.197689895515706,-0.000263726856300013,
-0.00554725977781399));
#35590=CARTESIAN_POINT('Ctrl Pts',(-0.198551365892026,-0.000267087899830605,
-0.00554754137704308));
#35591=CARTESIAN_POINT('Ctrl Pts',(-0.199429056133176,-0.00027045513768323,
-0.00554783128850645));
#35592=CARTESIAN_POINT('Ctrl Pts',(-0.200323641208812,-0.000273827273659161,
-0.00554812814068451));
#35593=CARTESIAN_POINT('Ctrl Pts',(-0.201218226284448,-0.000277199409635091,
-0.00554842499286257));
#35594=CARTESIAN_POINT('Ctrl Pts',(-0.202129706194687,-0.000280576415406435,
-0.00554872876800488));
#35595=CARTESIAN_POINT('Ctrl Pts',(-0.203057914973526,-0.000283953370692891,
-0.00554903828929629));
#35596=CARTESIAN_POINT('Ctrl Pts',(-0.204914332531203,-0.0002907072812658,
-0.00554965733187913));
#35597=CARTESIAN_POINT('Ctrl Pts',(-0.206837665564307,-0.000297461032084291,
-0.00555029923894105));
#35598=CARTESIAN_POINT('Ctrl Pts',(-0.208828046911259,-0.000304177112489735,
-0.00555096192484518));
#35599=CARTESIAN_POINT('Ctrl Pts',(-0.210818428167034,-0.000310893192587523,
-0.00555162461071896));
#35600=CARTESIAN_POINT('Ctrl Pts',(-0.212875857730999,-0.000317571487539541,
-0.00555230799325907));
#35601=CARTESIAN_POINT('Ctrl Pts',(-0.215000291390742,-0.000324168998365841,
-0.0055530216284886));
#35602=CARTESIAN_POINT('',(-0.186146181862621,0.00666198473330996,-0.00957679047534686));
#35603=CARTESIAN_POINT('Ctrl Pts',(-0.192201191480734,-0.000241594683462822,
-0.00554556743215708));
#35604=CARTESIAN_POINT('Ctrl Pts',(-0.191385432420279,-3.88012107838058E-5,
-0.005852563916371));
#35605=CARTESIAN_POINT('Ctrl Pts',(-0.18992436359119,0.000584077259331637,
-0.00669447323493867));
#35606=CARTESIAN_POINT('Ctrl Pts',(-0.188118589959122,0.00204642926269473,
-0.00799717565551262));
#35607=CARTESIAN_POINT('Ctrl Pts',(-0.186728499584069,0.00408398932516683,
-0.0090979910428183));
#35608=CARTESIAN_POINT('Ctrl Pts',(-0.186240928632579,0.00577350042675652,
-0.00949868268458664));
#35609=CARTESIAN_POINT('Ctrl Pts',(-0.186146181862621,0.00666198473330996,
-0.00957679047534686));
#35610=CARTESIAN_POINT('',(-0.186146181862621,0.0083380152666897,-0.00957679047534678));
#35611=CARTESIAN_POINT('Origin',(-0.187904819949368,0.00750020158743468,
-0.000565738065293699));
#35612=CARTESIAN_POINT('',(-0.192201191653566,0.0152415580820476,-0.00554550644721905));
#35613=CARTESIAN_POINT('Ctrl Pts',(-0.186146181862621,0.0083380152666897,
-0.00957679047534678));
#35614=CARTESIAN_POINT('Ctrl Pts',(-0.186240918786417,0.00922640724122356,
-0.00949869080161241));
#35615=CARTESIAN_POINT('Ctrl Pts',(-0.186729216417846,0.0109185839275611,
-0.00909746664888909));
#35616=CARTESIAN_POINT('Ctrl Pts',(-0.18812292744858,0.0129594111220647,
-0.00799351337395886));
#35617=CARTESIAN_POINT('Ctrl Pts',(-0.189934449608939,0.014420736841963,
-0.006688503795585));
#35618=CARTESIAN_POINT('Ctrl Pts',(-0.191383445765099,0.0150383073386066,
-0.00585331155888567));
#35619=CARTESIAN_POINT('Ctrl Pts',(-0.192201191480731,0.0152415946834622,
-0.00554556743215712));
#35620=CARTESIAN_POINT('',(-0.215000291562328,0.0153241509688053,-0.00555319360107524));
#35621=CARTESIAN_POINT('Ctrl Pts',(-0.215000291205702,0.0153242253442285,
-0.00555305296541064));
#35622=CARTESIAN_POINT('Ctrl Pts',(-0.213932597704458,0.0153209061962902,
-0.00555269287857503));
#35623=CARTESIAN_POINT('Ctrl Pts',(-0.212894379313026,0.0153176079358162,
-0.00555234120479523));
#35624=CARTESIAN_POINT('Ctrl Pts',(-0.211885508359842,0.0153143396802069,
-0.00555199831893506));
#35625=CARTESIAN_POINT('Ctrl Pts',(-0.210876637317151,0.0153110714243076,
-0.00555165543304446));
#35626=CARTESIAN_POINT('Ctrl Pts',(-0.209897113717939,0.0153078331616761,
-0.00555132133114625));
#35627=CARTESIAN_POINT('Ctrl Pts',(-0.208947320500622,0.0153046350773028,
-0.00555099748235955));
#35628=CARTESIAN_POINT('Ctrl Pts',(-0.208472423891963,0.0153030360351161,
-0.0055508355579662));
#35629=CARTESIAN_POINT('Ctrl Pts',(-0.208004959878718,0.0153014470440823,
-0.00555067620492078));
#35630=CARTESIAN_POINT('Ctrl Pts',(-0.207544449760479,0.0152998674643782,
-0.00555051955126661));
#35631=CARTESIAN_POINT('Ctrl Pts',(-0.207083939642239,0.0152982878846741,
-0.00555036289761244));
#35632=CARTESIAN_POINT('Ctrl Pts',(-0.206630383419139,0.0152967176785448,
-0.00555020892231339));
#35633=CARTESIAN_POINT('Ctrl Pts',(-0.206185727792834,0.0152951647572964,
-0.00555005845722071));
#35634=CARTESIAN_POINT('Ctrl Pts',(-0.20574107216653,0.0152936118360481,
-0.00554990799212803));
#35635=CARTESIAN_POINT('Ctrl Pts',(-0.205305317136504,0.0152920763396207,
-0.0055497611177857));
#35636=CARTESIAN_POINT('Ctrl Pts',(-0.204871154582032,0.0152905329744749,
-0.00554961590672052));
#35637=CARTESIAN_POINT('Ctrl Pts',(-0.204654073304796,0.015289761291902,
-0.00554954330118793));
#35638=CARTESIAN_POINT('Ctrl Pts',(-0.204437390146812,0.0152889875462586,
-0.00554947105540806));
#35639=CARTESIAN_POINT('Ctrl Pts',(-0.204230423755464,0.0152882454917763,
-0.00554940217900394));
#35640=CARTESIAN_POINT('Ctrl Pts',(-0.204023457364116,0.0152875034372941,
-0.00554933330259982));
#35641=CARTESIAN_POINT('Ctrl Pts',(-0.203826207738076,0.0152867934163249,
-0.00554926799916205));
#35642=CARTESIAN_POINT('Ctrl Pts',(-0.203600730112181,0.0152859778836302,
-0.00554919382403213));
#35643=CARTESIAN_POINT('Ctrl Pts',(-0.203375252486286,0.0152851623509355,
-0.00554911964890221));
#35644=CARTESIAN_POINT('Ctrl Pts',(-0.203121546862791,0.0152842407307248,
-0.00554903625738765));
#35645=CARTESIAN_POINT('Ctrl Pts',(-0.202875762064915,0.0152833433310473,
-0.00554895552284241));
#35646=CARTESIAN_POINT('Ctrl Pts',(-0.202629977267039,0.0152824459313697,
-0.00554887478829716));
#35647=CARTESIAN_POINT('Ctrl Pts',(-0.202392113293296,0.015281573127183,
-0.0055487969371522));
#35648=CARTESIAN_POINT('Ctrl Pts',(-0.202153351523362,0.0152806929783707,
-0.00554871893697691));
#35649=CARTESIAN_POINT('Ctrl Pts',(-0.201675827983494,0.015278932680746,
-0.00554856293662631));
#35650=CARTESIAN_POINT('Ctrl Pts',(-0.201194713260464,0.0152771426083813,
-0.00554840609743424));
#35651=CARTESIAN_POINT('Ctrl Pts',(-0.200716202959138,0.0152753454496153,
-0.00554825048440849));
#35652=CARTESIAN_POINT('Ctrl Pts',(-0.199759182356486,0.0152717511320833,
-0.005547939258357));
#35653=CARTESIAN_POINT('Ctrl Pts',(-0.198812579438422,0.0152681289979275,
-0.00554763326914996));
#35654=CARTESIAN_POINT('Ctrl Pts',(-0.197872595918786,0.0152644669040492,
-0.005547330085655));
#35655=CARTESIAN_POINT('Ctrl Pts',(-0.19693261239915,0.0152608048101709,
-0.00554702690216004));
#35656=CARTESIAN_POINT('Ctrl Pts',(-0.195999248275822,0.015257103211607,
-0.00554672683230568));
#35657=CARTESIAN_POINT('Ctrl Pts',(-0.195055360270019,0.0152532915881122,
-0.0055464240380698));
#35658=CARTESIAN_POINT('Ctrl Pts',(-0.194111472344545,0.0152494799649418,
-0.00554612124385969));
#35659=CARTESIAN_POINT('Ctrl Pts',(-0.193157060542462,0.0152455574395132,
-0.00554581513217478));
#35660=CARTESIAN_POINT('Ctrl Pts',(-0.192201191653566,0.0152415580820476,
-0.00554550644721905));
#35661=CARTESIAN_POINT('Ctrl Pts',(-0.215000291562328,0.0153241509688053,
-0.00555319360107524));
#35662=CARTESIAN_POINT('Ctrl Pts',(-0.215668740328172,0.0153262292429902,
-0.00555341941485916));
#35663=CARTESIAN_POINT('Ctrl Pts',(-0.216324729447901,0.0153937319339566,
-0.00543467464259903));
#35664=CARTESIAN_POINT('Ctrl Pts',(-0.216937360421232,0.0154983886920181,
-0.00521197223979806));
#35665=CARTESIAN_POINT('Ctrl Pts',(-0.217007386432887,0.0155103513509086,
-0.00518651652219178));
#35666=CARTESIAN_POINT('Ctrl Pts',(-0.217076845944537,0.0155227758123586,
-0.00515969417359937));
#35667=CARTESIAN_POINT('Ctrl Pts',(-0.217145692804874,0.0155356033754558,
-0.00513152375635335));
#35668=CARTESIAN_POINT('Ctrl Pts',(-0.217816854743512,0.015660654424613,
-0.00485690103923239));
#35669=CARTESIAN_POINT('Ctrl Pts',(-0.21842980551494,0.0158246085287311,
-0.00445372675993447));
#35670=CARTESIAN_POINT('Ctrl Pts',(-0.218946402952426,0.0159650714808781,
-0.00394588998612724));
#35671=CARTESIAN_POINT('Ctrl Pts',(-0.219117571675436,0.0160116122927455,
-0.00377762401002606));
#35672=CARTESIAN_POINT('Ctrl Pts',(-0.2192781592448,0.0160555588565627,
-0.00359779983207659));
#35673=CARTESIAN_POINT('Ctrl Pts',(-0.219426705149579,0.0160944931464038,
-0.00340810586555922));
#35674=CARTESIAN_POINT('Ctrl Pts',(-0.219502319454705,0.0161143118635625,
-0.00331154596721636));
#35675=CARTESIAN_POINT('Ctrl Pts',(-0.219574813625008,0.0161328299754327,
-0.00321243764433068));
#35676=CARTESIAN_POINT('Ctrl Pts',(-0.219643995479742,0.0161499296503641,
-0.00311087714745257));
#35677=CARTESIAN_POINT('Ctrl Pts',(-0.219784412581996,0.0161846365371998,
-0.00290474172755338));
#35678=CARTESIAN_POINT('Ctrl Pts',(-0.219911192765131,0.0162133601522874,
-0.00268891185321829));
#35679=CARTESIAN_POINT('Ctrl Pts',(-0.220022736985533,0.0162359498238763,
-0.0024643964070149));
#35680=CARTESIAN_POINT('Ctrl Pts',(-0.220074112549396,0.0162463542815091,
-0.00236098802240206));
#35681=CARTESIAN_POINT('Ctrl Pts',(-0.220122255969117,0.0162554705354734,
-0.00225573022547248));
#35682=CARTESIAN_POINT('Ctrl Pts',(-0.220167013727973,0.0162635401033155,
-0.00214910016136067));
#35683=CARTESIAN_POINT('Ctrl Pts',(-0.220255304272581,0.0162794583833577,
-0.00193875838660007));
#35684=CARTESIAN_POINT('Ctrl Pts',(-0.220330419862705,0.0162913921573094,
-0.00172100901754344));
#35685=CARTESIAN_POINT('Ctrl Pts',(-0.220392020126769,0.0163017866191688,
-0.00150014969593761));
#35686=CARTESIAN_POINT('Ctrl Pts',(-0.220528474005327,0.0163248119204041,
-0.00101091297744705));
#35687=CARTESIAN_POINT('Ctrl Pts',(-0.22059861780742,0.0163407734893559,
-0.000507277223307716));
#35688=CARTESIAN_POINT('Ctrl Pts',(-0.220598427190516,0.0163420797339417,
7.52423205390498E-7));
#35689=CARTESIAN_POINT('Ctrl Pts',(-0.220598376880276,0.0163424244960112,
0.000134838607512327));
#35690=CARTESIAN_POINT('Ctrl Pts',(-0.220593422600694,0.0163417464071427,
0.000268914083012791));
#35691=CARTESIAN_POINT('Ctrl Pts',(-0.220583640914636,0.016339936520452,
0.000402703728358851));
#35692=CARTESIAN_POINT('Ctrl Pts',(-0.220560148132489,0.0163355896958366,
0.000724027779571594));
#35693=CARTESIAN_POINT('Ctrl Pts',(-0.220508810660082,0.0163246874026146,
0.0010437232789448));
#35694=CARTESIAN_POINT('Ctrl Pts',(-0.220430682085685,0.0163092078903576,
0.00135493667144938));
#35695=CARTESIAN_POINT('Ctrl Pts',(-0.220390026628729,0.0163011528778462,
0.00151688155244445));
#35696=CARTESIAN_POINT('Ctrl Pts',(-0.220342116540319,0.0162918774559878,
0.00167656206656788));
#35697=CARTESIAN_POINT('Ctrl Pts',(-0.220287103455273,0.016282199079049,
0.00183469943034553));
#35698=CARTESIAN_POINT('Ctrl Pts',(-0.220249786004752,0.0162756338709311,
0.00194196996868066));
#35699=CARTESIAN_POINT('Ctrl Pts',(-0.220209200000601,0.0162688655768999,
0.00204849164457503));
#35700=CARTESIAN_POINT('Ctrl Pts',(-0.220165384926114,0.0162612875677296,
0.0021527788685016));
#35701=CARTESIAN_POINT('Ctrl Pts',(-0.220141806666224,0.01625720960434,
0.00220889908050186));
#35702=CARTESIAN_POINT('Ctrl Pts',(-0.22011729291399,0.0162528733413081,
0.00226472489623903));
#35703=CARTESIAN_POINT('Ctrl Pts',(-0.220091864350141,0.0162481906744713,
0.00232003547938548));
#35704=CARTESIAN_POINT('Origin',(-0.206561433685686,0.00750002637574172,
0.0135355039474176));
#35705=CARTESIAN_POINT('',(-0.186019881459752,0.00692134436047904,0.00979684421662477));
#35706=CARTESIAN_POINT('Ctrl Pts',(-0.185999364351512,0.00749999962802277,
0.00991138348445803));
#35707=CARTESIAN_POINT('Ctrl Pts',(-0.185999376571189,0.00730961846353397,
0.00991131415321303));
#35708=CARTESIAN_POINT('Ctrl Pts',(-0.186006003246306,0.00711673337435274,
0.00987309615363802));
#35709=CARTESIAN_POINT('Ctrl Pts',(-0.186019881459752,0.00692134436047904,
0.00979684421662477));
#35710=CARTESIAN_POINT('',(-0.186041755315114,0.0066688778475149,0.00967860489999109));
#35711=CARTESIAN_POINT('Ctrl Pts',(-0.186019884049452,0.00692131183731184,
0.00979683157756966));
#35712=CARTESIAN_POINT('Ctrl Pts',(-0.186026050535138,0.00683448131744766,
0.00976295078830858));
#35713=CARTESIAN_POINT('Ctrl Pts',(-0.186033396723478,0.00675056489938151,
0.0097230652955223));
#35714=CARTESIAN_POINT('Ctrl Pts',(-0.186041751476459,0.00666887311730628,
0.00967861576317704));
#35715=CARTESIAN_POINT('',(-0.186045756633599,0.00664877182750347,0.00965739225385244));
#35716=CARTESIAN_POINT('Ctrl Pts',(-0.186045750694262,0.00664885008080394,
0.00965739927776235));
#35717=CARTESIAN_POINT('Ctrl Pts',(-0.186045567569101,0.0066487514075171,
0.00965836803390889));
#35718=CARTESIAN_POINT('Ctrl Pts',(-0.186045385816378,0.00664882388039244,
0.00965932990672161));
#35719=CARTESIAN_POINT('Ctrl Pts',(-0.18604500765403,0.00664928351164828,
0.00966133197577962));
#35720=CARTESIAN_POINT('Ctrl Pts',(-0.186044817391655,0.0066496963288531,
0.00966233970967473));
#35721=CARTESIAN_POINT('Ctrl Pts',(-0.18604420014009,0.00665147479437923,
0.00966561019654977));
#35722=CARTESIAN_POINT('Ctrl Pts',(-0.186043801299601,0.00665343241809817,
0.00966772565168096));
#35723=CARTESIAN_POINT('Ctrl Pts',(-0.186042813488648,0.00665927890134443,
0.00967296823442883));
#35724=CARTESIAN_POINT('Ctrl Pts',(-0.186042225851779,0.00666431391360417,
0.0096760919773268));
#35725=CARTESIAN_POINT('Ctrl Pts',(-0.186041756611168,0.00666888632110605,
0.00967858844524271));
#35726=CARTESIAN_POINT('',(-0.18604575186606,0.00835120658339954,0.0096573930787881));
#35727=CARTESIAN_POINT('Ctrl Pts',(-0.186045752236316,0.00664877185494917,
0.00965739112009325));
#35728=CARTESIAN_POINT('Ctrl Pts',(-0.18603600739274,0.00721625009776599,
0.00970894240247701));
#35729=CARTESIAN_POINT('Ctrl Pts',(-0.186036007269321,0.00778372834058278,
0.00970894305537529));
#35730=CARTESIAN_POINT('Ctrl Pts',(-0.18604575186606,0.00835120658339954,
0.0096573930787881));
#35731=CARTESIAN_POINT('',(-0.186041751490874,0.00833112702364014,0.00967861612727941));
#35732=CARTESIAN_POINT('Ctrl Pts',(-0.186045750325906,0.00835112529557688,
0.0096574012264128));
#35733=CARTESIAN_POINT('Ctrl Pts',(-0.186045605429111,0.00835120318317337,
0.00965816774988358));
#35734=CARTESIAN_POINT('Ctrl Pts',(-0.186045460789224,0.00835117430982953,
0.00965893315000607));
#35735=CARTESIAN_POINT('Ctrl Pts',(-0.186045151109668,0.00835090412616134,
0.00966057240088015));
#35736=CARTESIAN_POINT('Ctrl Pts',(-0.186044990615733,0.0083506354811343,
0.00966142226520882));
#35737=CARTESIAN_POINT('Ctrl Pts',(-0.186044474171132,0.00834944013196887,
0.00966415786011833));
#35738=CARTESIAN_POINT('Ctrl Pts',(-0.18604414023323,0.00834809736249489,
0.00966592822660773));
#35739=CARTESIAN_POINT('Ctrl Pts',(-0.186043057962283,0.0083427181772925,
0.00967166900991584));
#35740=CARTESIAN_POINT('Ctrl Pts',(-0.186042338516759,0.00833676576308223,
0.00967549257825685));
#35741=CARTESIAN_POINT('Ctrl Pts',(-0.186041757634892,0.00833110922485847,
0.00967858299879916));
#35742=CARTESIAN_POINT('',(-0.186019881459749,0.0080786556394931,0.00979684421664208));
#35743=CARTESIAN_POINT('Ctrl Pts',(-0.186041751450861,0.00833112702364026,
0.00967861611975897));
#35744=CARTESIAN_POINT('Ctrl Pts',(-0.186033396707417,0.00824943534841117,
0.00972306560553079));
#35745=CARTESIAN_POINT('Ctrl Pts',(-0.186026050708484,0.00816551734876726,
0.00976294827134343));
#35746=CARTESIAN_POINT('Ctrl Pts',(-0.186019884249235,0.00807868703243332,
0.00979682889022281));
#35747=CARTESIAN_POINT('Ctrl Pts',(-0.186019881459749,0.0080786556394931,
0.00979684421664208));
#35748=CARTESIAN_POINT('Ctrl Pts',(-0.18600600325118,0.00788326669427363,
0.00987309612685917));
#35749=CARTESIAN_POINT('Ctrl Pts',(-0.185999376576045,0.00769038148190397,
0.00991131412647235));
#35750=CARTESIAN_POINT('Ctrl Pts',(-0.185999364351488,0.00750000000238413,
0.00991138348459431));
#35751=CARTESIAN_POINT('Origin',(-0.215,-0.00247776328493882,0.));
#35752=CARTESIAN_POINT('',(-0.217717620464915,-0.000864182492545611,-0.00478156822519172));
#35753=CARTESIAN_POINT('Ctrl Pts',(-0.215000000001386,-0.000525628313080397,
0.0055));
#35754=CARTESIAN_POINT('Ctrl Pts',(-0.215733657093434,-0.000527918025936895,
0.0055));
#35755=CARTESIAN_POINT('Ctrl Pts',(-0.216453796216893,-0.000613506209613022,
0.00535197579258614));
#35756=CARTESIAN_POINT('Ctrl Pts',(-0.217113615428784,-0.000737496304503929,
0.00507765997808475));
#35757=CARTESIAN_POINT('Ctrl Pts',(-0.217773434640674,-0.000861486399394835,
0.00480334416358336));
#35758=CARTESIAN_POINT('Ctrl Pts',(-0.218372957928401,-0.00102387445685327,
0.00440280379788875));
#35759=CARTESIAN_POINT('Ctrl Pts',(-0.218878851239864,-0.00116524793995074,
0.00389929670329421));
#35760=CARTESIAN_POINT('Ctrl Pts',(-0.219131797895595,-0.00123593468149947,
0.00364754315599693));
#35761=CARTESIAN_POINT('Ctrl Pts',(-0.219361326626901,-0.0013013686722475,
0.00337004060674126));
#35762=CARTESIAN_POINT('Ctrl Pts',(-0.219562216703885,-0.00135080819197357,
0.00307183602795968));
#35763=CARTESIAN_POINT('Ctrl Pts',(-0.219763106780869,-0.00140024771169963,
0.0027736314491781));
#35764=CARTESIAN_POINT('Ctrl Pts',(-0.219935355158733,-0.00143367458564157,
0.00245471925505583));
#35765=CARTESIAN_POINT('Ctrl Pts',(-0.220074649373074,-0.00146068274866806,
0.00212083446913069));
#35766=CARTESIAN_POINT('Ctrl Pts',(-0.220353237801756,-0.00151469907472103,
0.00145306489728042));
#35767=CARTESIAN_POINT('Ctrl Pts',(-0.220499995520898,-0.00154301300909184,
0.000725393689757325));
#35768=CARTESIAN_POINT('Ctrl Pts',(-0.220499999832106,-0.00154301573465214,
-1.2615307860019E-6));
#35769=CARTESIAN_POINT('Ctrl Pts',(-0.220500004143313,-0.00154301846021245,
-0.000727916751329329));
#35770=CARTESIAN_POINT('Ctrl Pts',(-0.220353266885017,-0.00151470914363584,
-0.00145355702203918));
#35771=CARTESIAN_POINT('Ctrl Pts',(-0.220074654242848,-0.00146068379631778,
-0.00212082205575858));
#35772=CARTESIAN_POINT('Ctrl Pts',(-0.219935347921764,-0.00143367112265876,
-0.00245445457261828));
#35773=CARTESIAN_POINT('Ctrl Pts',(-0.219763071420699,-0.00140023460347288,
-0.0027734933586571));
#35774=CARTESIAN_POINT('Ctrl Pts',(-0.219562410856384,-0.00135085625104822,
-0.00307154800594128));
#35775=CARTESIAN_POINT('Ctrl Pts',(-0.219361750292068,-0.00130147789862356,
-0.00336960265322547));
#35776=CARTESIAN_POINT('Ctrl Pts',(-0.219132710242754,-0.00123617309737434,
-0.00364667970707124));
#35777=CARTESIAN_POINT('Ctrl Pts',(-0.218879812273829,-0.0011655117256891,
-0.00389834020393884));
#35778=CARTESIAN_POINT('Ctrl Pts',(-0.218533262901617,-0.00106868353010786,
-0.00424319385211476));
#35779=CARTESIAN_POINT('Ctrl Pts',(-0.21814193096314,-0.000961794536041287,
-0.00454033265003914));
#35780=CARTESIAN_POINT('Ctrl Pts',(-0.217717620464915,-0.000864182492545611,
-0.00478156822519172));
#35781=CARTESIAN_POINT('Ctrl Pts',(-0.217717620464915,-0.000864182492545611,
-0.00478156822519172));
#35782=CARTESIAN_POINT('Ctrl Pts',(-0.217522646165287,-0.000819325948101552,
-0.00489243010568115));
#35783=CARTESIAN_POINT('Ctrl Pts',(-0.217320705382708,-0.000776429290875688,
-0.00499148255206137));
#35784=CARTESIAN_POINT('Ctrl Pts',(-0.217112947318933,-0.000737367546107008,
-0.00507793792370663));
#35785=CARTESIAN_POINT('Ctrl Pts',(-0.216453070075793,-0.000613300369209368,
-0.00535253584428553));
#35786=CARTESIAN_POINT('Ctrl Pts',(-0.215734488701503,-0.000527921467098434,
-0.0055));
#35787=CARTESIAN_POINT('Ctrl Pts',(-0.215000000001605,-0.000525629159658772,
-0.0055));
#35788=CARTESIAN_POINT('',(-0.217113535264296,-0.000627890658473149,-0.00507769324464509));
#35789=CARTESIAN_POINT('Ctrl Pts',(-0.215000000458298,-0.000412691216678721,
-0.00549999999999998));
#35790=CARTESIAN_POINT('Ctrl Pts',(-0.215733763662974,-0.000415150006623741,
-0.00549999993833047));
#35791=CARTESIAN_POINT('Ctrl Pts',(-0.216453895571815,-0.000502156767438298,
-0.00535189476124435));
#35792=CARTESIAN_POINT('Ctrl Pts',(-0.217113535264296,-0.000627890658473149,
-0.00507769324464509));
#35793=CARTESIAN_POINT('Ctrl Pts',(-0.217113736162319,-0.00062792895318973,
-0.00507760972992005));
#35794=CARTESIAN_POINT('Ctrl Pts',(-0.21777343067469,-0.000753683498393302,
-0.00480335471430899));
#35795=CARTESIAN_POINT('Ctrl Pts',(-0.218372640661352,-0.000918161231759694,
-0.00440304836193869));
#35796=CARTESIAN_POINT('Ctrl Pts',(-0.218878461318587,-0.00106131402982561,
-0.00389968457354958));
#35797=CARTESIAN_POINT('Ctrl Pts',(-0.219131371647205,-0.00113289042885856,
-0.00364800267935503));
#35798=CARTESIAN_POINT('Ctrl Pts',(-0.219360923803304,-0.00119913785768892,
-0.00337054897752257));
#35799=CARTESIAN_POINT('Ctrl Pts',(-0.219561841261719,-0.00124918487971837,
-0.00307239351550298));
#35800=CARTESIAN_POINT('Ctrl Pts',(-0.219762758720135,-0.00129923190174783,
-0.00277423805348339));
#35801=CARTESIAN_POINT('Ctrl Pts',(-0.219935037411276,-0.00133307753813197,
-0.00245537690118891));
#35802=CARTESIAN_POINT('Ctrl Pts',(-0.220074378299315,-0.00136032636734795,
-0.00212148304035139));
#35803=CARTESIAN_POINT('Ctrl Pts',(-0.220353060075392,-0.0014148240257799,
-0.00145369531867635));
#35804=CARTESIAN_POINT('Ctrl Pts',(-0.220499972439958,-0.00144299794853512,
-0.000725772738476444));
#35805=CARTESIAN_POINT('Ctrl Pts',(-0.220499999860936,-0.00144300315744521,
1.12053422684619E-6));
#35806=CARTESIAN_POINT('Ctrl Pts',(-0.220500027281913,-0.0014430083663553,
0.000728013806930138));
#35807=CARTESIAN_POINT('Ctrl Pts',(-0.220353181889183,-0.00141484823386804,
0.00145387666412653));
#35808=CARTESIAN_POINT('Ctrl Pts',(-0.220074498824012,-0.00136034902137536,
0.00212119392664514));
#35809=CARTESIAN_POINT('Ctrl Pts',(-0.219935157291427,-0.00133309941512902,
0.00245485255790444));
#35810=CARTESIAN_POINT('Ctrl Pts',(-0.219762855704549,-0.00129925229730477,
0.00277387333358092));
#35811=CARTESIAN_POINT('Ctrl Pts',(-0.219562168120678,-0.00124926997129964,
0.00307190851276041));
#35812=CARTESIAN_POINT('Ctrl Pts',(-0.219361480536807,-0.00119928764529451,
0.0033699436919399));
#35813=CARTESIAN_POINT('Ctrl Pts',(-0.219132412388149,-0.00113317179309311,
0.00364699857065988));
#35814=CARTESIAN_POINT('Ctrl Pts',(-0.218879539633775,-0.00106161857632371,
0.00389861154566044));
#35815=CARTESIAN_POINT('Ctrl Pts',(-0.218373794125028,-0.000918512142784899,
0.00440183749566157));
#35816=CARTESIAN_POINT('Ctrl Pts',(-0.217772867004196,-0.000753649502850171,
0.00480332063947502));
#35817=CARTESIAN_POINT('Ctrl Pts',(-0.217113099314996,-0.000627808309406593,
0.00507787468216161));
#35818=CARTESIAN_POINT('Ctrl Pts',(-0.216453331762976,-0.000501967142128145,
0.00535242866776241));
#35819=CARTESIAN_POINT('Ctrl Pts',(-0.215734704272005,-0.000415151996213136,
0.00549999993863343));
#35820=CARTESIAN_POINT('Ctrl Pts',(-0.215000000458283,-0.000412690055633917,
0.00549999999999998));
#35821=CARTESIAN_POINT('Origin',(-0.215,-0.00247776328493882,0.));
#35822=CARTESIAN_POINT('',(-0.21771763199541,0.0158641872473072,0.0047815616735964));
#35823=CARTESIAN_POINT('Ctrl Pts',(-0.215000000001386,0.0155256291596571,
-0.0055));
#35824=CARTESIAN_POINT('Ctrl Pts',(-0.2157336570704,0.0155279188704998,
-0.0055));
#35825=CARTESIAN_POINT('Ctrl Pts',(-0.216453796318392,0.0156135057925174,
-0.00535197578874485));
#35826=CARTESIAN_POINT('Ctrl Pts',(-0.217113615626837,0.0157374949853798,
-0.00507765989564486));
#35827=CARTESIAN_POINT('Ctrl Pts',(-0.217773434935281,0.0158614841782422,
-0.00480334400254486));
#35828=CARTESIAN_POINT('Ctrl Pts',(-0.218372958291692,0.0160238716929941,
-0.00440280348312629));
#35829=CARTESIAN_POINT('Ctrl Pts',(-0.218878851501825,0.0161652458161567,
-0.00389929644268416));
#35830=CARTESIAN_POINT('Ctrl Pts',(-0.219131798106892,0.016235932877738,
-0.0036475429224631));
#35831=CARTESIAN_POINT('Ctrl Pts',(-0.219361326745382,0.0163013674845095,
-0.00337004045270962));
#35832=CARTESIAN_POINT('Ctrl Pts',(-0.219562216772735,0.0163508074239199,
-0.0030718359257235));
#35833=CARTESIAN_POINT('Ctrl Pts',(-0.219763106800088,0.0164002473633304,
-0.00277363139873738));
#35834=CARTESIAN_POINT('Ctrl Pts',(-0.219935355171308,0.0164336744598742,
-0.00245471922851232));
#35835=CARTESIAN_POINT('Ctrl Pts',(-0.220074649381718,0.016460682750153,
-0.0021208344484449));
#35836=CARTESIAN_POINT('Ctrl Pts',(-0.220353237802539,0.0165146993307108,
-0.00145306488831005));
#35837=CARTESIAN_POINT('Ctrl Pts',(-0.220499995524514,0.0165430131365752,
-0.000725393619809854));
#35838=CARTESIAN_POINT('Ctrl Pts',(-0.220499999832085,0.0165430157347685,
1.26162095524048E-6));
#35839=CARTESIAN_POINT('Ctrl Pts',(-0.220500004139655,0.0165430183329617,
0.000727916861720345));
#35840=CARTESIAN_POINT('Ctrl Pts',(-0.22035326687219,0.0165147088896741,
0.00145355711184016));
#35841=CARTESIAN_POINT('Ctrl Pts',(-0.220074654185537,0.0164606837862868,
0.00212082219289029));
#35842=CARTESIAN_POINT('Ctrl Pts',(-0.219935347842211,0.0164336712345932,
0.00245445473341535));
#35843=CARTESIAN_POINT('Ctrl Pts',(-0.219763071310037,0.0164002349297366,
0.00277349355999628));
#35844=CARTESIAN_POINT('Ctrl Pts',(-0.219562410692062,0.0163508569943117,
0.00307154825001662));
#35845=CARTESIAN_POINT('Ctrl Pts',(-0.219361750074086,0.0163014790588868,
0.00336960294003696));
#35846=CARTESIAN_POINT('Ctrl Pts',(-0.219132709948445,0.0162361748768451,
0.00364668003869167));
#35847=CARTESIAN_POINT('Ctrl Pts',(-0.21887981193522,0.0161655138270336,
0.00389834054094438));
#35848=CARTESIAN_POINT('Ctrl Pts',(-0.218533265738991,0.0160686869768679,
0.00424319097564957));
#35849=CARTESIAN_POINT('Ctrl Pts',(-0.218141937873558,0.0159617989582928,
0.00454032737798169));
#35850=CARTESIAN_POINT('Ctrl Pts',(-0.21771763199541,0.0158641872473072,
0.0047815616735964));
#35851=CARTESIAN_POINT('Ctrl Pts',(-0.21771763199541,0.0158641872473072,
0.0047815616735964));
#35852=CARTESIAN_POINT('Ctrl Pts',(-0.217522654035082,0.0158193295250965,
0.00489242625492518));
#35853=CARTESIAN_POINT('Ctrl Pts',(-0.21732070929407,0.0157764316704963,
0.00499148093737223));
#35854=CARTESIAN_POINT('Ctrl Pts',(-0.217112947042309,0.0157373688492824,
0.005077938038811));
#35855=CARTESIAN_POINT('Ctrl Pts',(-0.216453069909373,0.0156133007750843,
0.00535253587232454));
#35856=CARTESIAN_POINT('Ctrl Pts',(-0.215734488715537,0.0155279206225147,
0.0055));
#35857=CARTESIAN_POINT('Ctrl Pts',(-0.215000000001386,0.0155256283130808,
0.0055));
#35858=CARTESIAN_POINT('',(-0.217113535052694,0.0156278918245936,0.00507769333272214));
#35859=CARTESIAN_POINT('Ctrl Pts',(-0.215000000458283,0.0154126900556344,
0.00549999999999998));
#35860=CARTESIAN_POINT('Ctrl Pts',(-0.215733763690548,0.0154151488445598,
0.00549999993833244));
#35861=CARTESIAN_POINT('Ctrl Pts',(-0.216453895466079,0.0155021569505519,
0.00535189476437573));
#35862=CARTESIAN_POINT('Ctrl Pts',(-0.217113535052694,0.0156278918245936,
0.00507769333272214));
#35863=CARTESIAN_POINT('Ctrl Pts',(-0.217113735942853,0.0156279301181165,
0.00507760982127901));
#35864=CARTESIAN_POINT('Ctrl Pts',(-0.217773430347217,0.0157536856455482,
0.00480335489272425));
#35865=CARTESIAN_POINT('Ctrl Pts',(-0.218372640253876,0.0159181639994022,
0.00440304871061857));
#35866=CARTESIAN_POINT('Ctrl Pts',(-0.21887846101466,0.0160613161775311,
0.00389968487584725));
#35867=CARTESIAN_POINT('Ctrl Pts',(-0.219131371395052,0.0161328922665954,
0.00364800295846159));
#35868=CARTESIAN_POINT('Ctrl Pts',(-0.219360923648429,0.0161991390750316,
0.00337054917879593));
#35869=CARTESIAN_POINT('Ctrl Pts',(-0.219561841160825,0.0162491856697833,
0.00307239366528832));
#35870=CARTESIAN_POINT('Ctrl Pts',(-0.219762758673222,0.016299232264535,
0.00277423815178071));
#35871=CARTESIAN_POINT('Ctrl Pts',(-0.21993503737532,0.0163330776666233,
0.00245537697442852));
#35872=CARTESIAN_POINT('Ctrl Pts',(-0.220074378271048,0.0163603263626206,
0.00212148310796454));
#35873=CARTESIAN_POINT('Ctrl Pts',(-0.220353060062505,0.0164148237546151,
0.00145369537503657));
#35874=CARTESIAN_POINT('Ctrl Pts',(-0.220499972429734,0.0164429978133269,
0.00072577286152451));
#35875=CARTESIAN_POINT('Ctrl Pts',(-0.220499999860965,0.0164430031575457,
-1.12038921492091E-6));
#35876=CARTESIAN_POINT('Ctrl Pts',(-0.220500027292196,0.0164430085017644,
-0.000728013639954359));
#35877=CARTESIAN_POINT('Ctrl Pts',(-0.220353181916319,0.0164148485032365,
-0.00145387651991067));
#35878=CARTESIAN_POINT('Ctrl Pts',(-0.220074498903735,0.0163603490352413,
-0.00212119373592478));
#35879=CARTESIAN_POINT('Ctrl Pts',(-0.219935157397444,0.0163330993012436,
-0.00245485234393184));
#35880=CARTESIAN_POINT('Ctrl Pts',(-0.219762855845866,0.0162992519580117,
-0.0027738730790881));
#35881=CARTESIAN_POINT('Ctrl Pts',(-0.219562168320338,0.0162492692075871,
-0.00307190821624611));
#35882=CARTESIAN_POINT('Ctrl Pts',(-0.219361480794809,0.0161992864571625,
-0.00336994335340409));
#35883=CARTESIAN_POINT('Ctrl Pts',(-0.219132412727695,0.0161331699814419,
-0.00364699818864903));
#35884=CARTESIAN_POINT('Ctrl Pts',(-0.218879540019051,0.0160616164528147,
-0.00389861116226235));
#35885=CARTESIAN_POINT('Ctrl Pts',(-0.218373794601764,0.0159185093955602,
-0.00440183710948903));
#35886=CARTESIAN_POINT('Ctrl Pts',(-0.21777286742818,0.0157536473775453,
-0.00480332041750894));
#35887=CARTESIAN_POINT('Ctrl Pts',(-0.217113099616091,0.0156278071611984,
-0.00507787455686463));
#35888=CARTESIAN_POINT('Ctrl Pts',(-0.216453331941187,0.0155019669710174,
-0.00535242863913241));
#35889=CARTESIAN_POINT('Ctrl Pts',(-0.215734704256714,0.0154151531583194,
-0.00549999993863114));
#35890=CARTESIAN_POINT('Ctrl Pts',(-0.2150000004583,0.0154126912166778,
-0.00549999999999998));
#35891=CARTESIAN_POINT('Origin',(-0.206561432239279,0.00749997362422107,
-0.0135355036852295));
#35892=CARTESIAN_POINT('',(-0.186019881496892,0.0080786561625007,-0.00979684401252669));
#35893=CARTESIAN_POINT('Ctrl Pts',(-0.185999364351523,0.00750000038130581,
-0.00991138348445716));
#35894=CARTESIAN_POINT('Ctrl Pts',(-0.185999376571405,0.00769038170948611,
-0.00991131415203012));
#35895=CARTESIAN_POINT('Ctrl Pts',(-0.186006003258135,0.00788326696988442,
-0.00987309608428367));
#35896=CARTESIAN_POINT('Ctrl Pts',(-0.186019881496892,0.0080786561625007,
-0.00979684401252669));
#35897=CARTESIAN_POINT('',(-0.186041755776097,0.00833112667101796,-0.00967861197300846));
#35898=CARTESIAN_POINT('Ctrl Pts',(-0.186019884086589,0.00807868868559217,
-0.00979683137349002));
#35899=CARTESIAN_POINT('Ctrl Pts',(-0.186026050577798,0.0081655192043983,
-0.00976295055579292));
#35900=CARTESIAN_POINT('Ctrl Pts',(-0.186033396771404,0.0082494356206791,
-0.00972306503719262));
#35901=CARTESIAN_POINT('Ctrl Pts',(-0.186041751529428,0.00833112740062736,
-0.00967861548148799));
#35902=CARTESIAN_POINT('',(-0.186045753543968,0.00835130156890068,-0.00965738420265808));
#35903=CARTESIAN_POINT('Ctrl Pts',(-0.186045764689502,0.00835128455723845,
-0.00965738815309785));
#35904=CARTESIAN_POINT('Ctrl Pts',(-0.186043858668127,0.00835231500591592,
-0.00966747326300593));
#35905=CARTESIAN_POINT('Ctrl Pts',(-0.186042683533208,0.00834015517577814,
-0.00967370297361173));
#35906=CARTESIAN_POINT('Ctrl Pts',(-0.186041757888406,0.00833112619861691,
-0.00967861022784464));
#35907=CARTESIAN_POINT('',(-0.186045753664356,0.00664869142106229,-0.00965738356578759));
#35908=CARTESIAN_POINT('Ctrl Pts',(-0.186045753543968,0.00835130156890068,
-0.00965738420265809));
#35909=CARTESIAN_POINT('Ctrl Pts',(-0.186036006823495,0.00778376485295418,
-0.00970894540982141));
#35910=CARTESIAN_POINT('Ctrl Pts',(-0.186036006863625,0.00721622813700805,
-0.00970894519753124));
#35911=CARTESIAN_POINT('Ctrl Pts',(-0.186045753664356,0.00664869142106229,
-0.00965738356578759));
#35912=CARTESIAN_POINT('',(-0.186041751543844,0.00666887245842392,-0.00967861584559627));
#35913=CARTESIAN_POINT('Origin',(-0.185976327015533,0.0109621773062506,
-0.0100140390940224));
#35914=CARTESIAN_POINT('',(-0.186019881496891,0.00692134383750547,-0.00979684401253565));
#35915=CARTESIAN_POINT('Ctrl Pts',(-0.18604175150383,0.00666887245842397,
-0.00967861583807533));
#35916=CARTESIAN_POINT('Ctrl Pts',(-0.186033396755342,0.0067505641315426,
-0.00972306534721564));
#35917=CARTESIAN_POINT('Ctrl Pts',(-0.186026050751142,0.00683448212941961,
-0.00976294803884862));
#35918=CARTESIAN_POINT('Ctrl Pts',(-0.186019884286368,0.00692131244471435,
-0.00979682868616852));
#35919=CARTESIAN_POINT('Ctrl Pts',(-0.186019881496891,0.00692134383750547,
-0.00979684401253565));
#35920=CARTESIAN_POINT('Ctrl Pts',(-0.186006003262742,0.00711673296524612,
-0.00987309605897389));
#35921=CARTESIAN_POINT('Ctrl Pts',(-0.185999376576004,0.00730961835274437,
-0.00991131412676384));
#35922=CARTESIAN_POINT('Ctrl Pts',(-0.185999364351498,0.00750000000000023,
-0.00991138348459597));
#35923=CARTESIAN_POINT('Origin',(-0.238,-0.00203858085746875,-0.0110866403454819));
#35924=CARTESIAN_POINT('',(-0.230921436096816,0.0162188491197267,-0.00255390765181725));
#35925=CARTESIAN_POINT('',(-0.230921436098924,0.0163191149846998,-0.0025539076543603));
#35926=CARTESIAN_POINT('',(-0.2309214360969,-0.00203858085746875,-0.00255390765191895));
#35927=CARTESIAN_POINT('',(-0.235510405486502,0.0139139931904494,-0.0080856016051615));
#35928=CARTESIAN_POINT('Ctrl Pts',(-0.2309214360969,0.0163191144755479,
-0.00255390765191895));
#35929=CARTESIAN_POINT('Ctrl Pts',(-0.23174153328286,0.0162404099789032,
-0.00354247965131538));
#35930=CARTESIAN_POINT('Ctrl Pts',(-0.233359727310792,0.0157744006398884,
-0.00549310371513331));
#35931=CARTESIAN_POINT('Ctrl Pts',(-0.234843981104082,0.0146553646943324,
-0.0072822718346736));
#35932=CARTESIAN_POINT('Ctrl Pts',(-0.235510405486502,0.0139139931904494,
-0.00808560160516149));
#35933=CARTESIAN_POINT('',(-0.237188474496957,0.011147446881013,-0.0101084009333268));
#35934=CARTESIAN_POINT('Ctrl Pts',(-0.235510405486502,0.0139139931904494,
-0.00808560160516149));
#35935=CARTESIAN_POINT('Ctrl Pts',(-0.236176829868922,0.0131726216865665,
-0.00888893137564938));
#35936=CARTESIAN_POINT('Ctrl Pts',(-0.236767551737116,0.0122493966515786,
-0.00960100685685503));
#35937=CARTESIAN_POINT('Ctrl Pts',(-0.237188474496957,0.011147446881013,
-0.0101084009333268));
#35938=CARTESIAN_POINT('',(-0.237859980412293,0.00748903372880752,-0.0109178561499695));
#35939=CARTESIAN_POINT('Ctrl Pts',(-0.237188474496957,0.011147446881013,
-0.0101084009333268));
#35940=CARTESIAN_POINT('Ctrl Pts',(-0.237609397256798,0.0100454971104472,
-0.0106157950097985));
#35941=CARTESIAN_POINT('Ctrl Pts',(-0.237860520908286,0.00876482260430375,
-0.0109185076815363));
#35942=CARTESIAN_POINT('Ctrl Pts',(-0.237859980412293,0.00748903372880752,
-0.0109178561499695));
#35943=CARTESIAN_POINT('',(-0.230921436098932,-0.00131911498648589,-0.00255390765437028));
#35944=CARTESIAN_POINT('Ctrl Pts',(-0.237859980412293,0.00748903372880752,
-0.0109178561499695));
#35945=CARTESIAN_POINT('Ctrl Pts',(-0.2378594399163,0.00621324485331131,
-0.0109172046184027));
#35946=CARTESIAN_POINT('Ctrl Pts',(-0.237355030629353,0.00367143836361342,
-0.0103091731486599));
#35947=CARTESIAN_POINT('Ctrl Pts',(-0.235579072060058,0.000893727961130872,
-0.00816837454119071));
#35948=CARTESIAN_POINT('Ctrl Pts',(-0.233347520676672,-0.00077875050644683,
-0.00547838943869806));
#35949=CARTESIAN_POINT('Ctrl Pts',(-0.231741081373355,-0.00124045334853188,
-0.00354193490480122));
#35950=CARTESIAN_POINT('Ctrl Pts',(-0.2309214360969,-0.00131911447555364,
-0.00255390765191895));
#35951=CARTESIAN_POINT('',(-0.230921436096816,-0.00121884911973092,-0.00255390765181755));
#35952=CARTESIAN_POINT('',(-0.2309214360969,-0.00203858085746875,-0.00255390765191895));
#35953=CARTESIAN_POINT('Ctrl Pts',(-0.2309214360969,-0.00121884911929219,
-0.00255390765191893));
#35954=CARTESIAN_POINT('Ctrl Pts',(-0.231731717669817,-0.00114029951282499,
-0.00353064758997169));
#35955=CARTESIAN_POINT('Ctrl Pts',(-0.232531008931408,-0.000909424775714629,
-0.00449413944691078));
#35956=CARTESIAN_POINT('Ctrl Pts',(-0.233297221966274,-0.000517292730967896,
-0.00541775772631526));
#35957=CARTESIAN_POINT('Ctrl Pts',(-0.23406343500114,-0.000125160686221158,
-0.00634137600571974));
#35958=CARTESIAN_POINT('Ctrl Pts',(-0.23479656980928,0.000428228666161958,
-0.00722512070758961));
#35959=CARTESIAN_POINT('Ctrl Pts',(-0.235454855653561,0.00116121765859052,
-0.00801864001773443));
#35960=CARTESIAN_POINT('Ctrl Pts',(-0.236113141497842,0.00189420665101909,
-0.00881215932787925));
#35961=CARTESIAN_POINT('Ctrl Pts',(-0.236696578378263,0.0028067952834931,
-0.00951545324629902));
#35962=CARTESIAN_POINT('Ctrl Pts',(-0.237112279773004,0.00389578721949753,
-0.0100165533183223));
#35963=CARTESIAN_POINT('Ctrl Pts',(-0.237527981167745,0.00498477915550195,
-0.0105176533903456));
#35964=CARTESIAN_POINT('Ctrl Pts',(-0.237775947076806,0.0062501743950368,
-0.0108165596159724));
#35965=CARTESIAN_POINT('Ctrl Pts',(-0.237775416097689,0.00751077204058868,
-0.0108159195563599));
#35966=CARTESIAN_POINT('Ctrl Pts',(-0.237774885118572,0.00877136968614057,
-0.0108152794967474));
#35967=CARTESIAN_POINT('Ctrl Pts',(-0.237525857251278,0.0100271697377095,
-0.0105150931518957));
#35968=CARTESIAN_POINT('Ctrl Pts',(-0.237109005915905,0.011112676361498,
-0.0100126069037839));
#35969=CARTESIAN_POINT('Ctrl Pts',(-0.236692154580533,0.0121981829852864,
-0.00951012065567206));
#35970=CARTESIAN_POINT('Ctrl Pts',(-0.236107479777082,0.0131133961812944,
-0.00880533450430022));
#35971=CARTESIAN_POINT('Ctrl Pts',(-0.235447733272926,0.0138467040480916,
-0.00801005446691648));
#35972=CARTESIAN_POINT('Ctrl Pts',(-0.234787986768769,0.0145800119148888,
-0.00721477442953273));
#35973=CARTESIAN_POINT('Ctrl Pts',(-0.234053168563907,0.0151314144524751,
-0.00632900050613708));
#35974=CARTESIAN_POINT('Ctrl Pts',(-0.2332889897904,0.0155214971606677,
-0.00540783439198091));
#35975=CARTESIAN_POINT('Ctrl Pts',(-0.232524811016894,0.0159115798688603,
-0.00448666827782475));
#35976=CARTESIAN_POINT('Ctrl Pts',(-0.231731271674744,0.0161403427476591,
-0.00353010997290807));
#35977=CARTESIAN_POINT('Ctrl Pts',(-0.2309214360969,0.0162188491192864,
-0.00255390765191896));
#35978=CARTESIAN_POINT('Origin',(-0.234,-0.00203858085746875,0.));
#35979=CARTESIAN_POINT('',(-0.230644549324729,-0.00134174864052366,-0.00217737244536236));
#35980=CARTESIAN_POINT('Ctrl Pts',(-0.230921436078517,-0.00131911447736198,
-0.00255390762975915));
#35981=CARTESIAN_POINT('Ctrl Pts',(-0.230882799080788,-0.00132291515868807,
-0.00250733332704017));
#35982=CARTESIAN_POINT('Ctrl Pts',(-0.230847896563029,-0.00132621572305467,
-0.00246332967147474));
#35983=CARTESIAN_POINT('Ctrl Pts',(-0.23081093623588,-0.00132932875912759,
-0.00241451285115208));
#35984=CARTESIAN_POINT('Ctrl Pts',(-0.230773975902869,-0.00133244179569423,
-0.0023656960230872));
#35985=CARTESIAN_POINT('Ctrl Pts',(-0.230735375114978,-0.00133536730390772,
-0.00231172564600153));
#35986=CARTESIAN_POINT('Ctrl Pts',(-0.230710890470543,-0.00133716751732438,
-0.00227634762354863));
#35987=CARTESIAN_POINT('Ctrl Pts',(-0.230686405826108,-0.00133896773074104,
-0.00224096960109574));
#35988=CARTESIAN_POINT('Ctrl Pts',(-0.230675274796775,-0.00133964264936088,
-0.00222472208742556));
#35989=CARTESIAN_POINT('Ctrl Pts',(-0.230644549324729,-0.00134174864052366,
-0.00217737244536236));
#35990=CARTESIAN_POINT('',(-0.230177928184924,-0.00137996828035668,-0.00117973176629321));
#35991=CARTESIAN_POINT('Ctrl Pts',(-0.230644549324729,-0.00134174864052366,
-0.00217737244536236));
#35992=CARTESIAN_POINT('Ctrl Pts',(-0.230613823852683,-0.00134385463168645,
-0.00213002280329915));
#35993=CARTESIAN_POINT('Ctrl Pts',(-0.230564811227978,-0.00134739169539217,
-0.00205070191669902));
#35994=CARTESIAN_POINT('Ctrl Pts',(-0.230526711870365,-0.00135027334534756,
-0.00198400341948652));
#35995=CARTESIAN_POINT('Ctrl Pts',(-0.230488612512752,-0.00135315499530295,
-0.00191730492227402));
#35996=CARTESIAN_POINT('Ctrl Pts',(-0.230460264018485,-0.00135538123150799,
-0.00186386387206019));
#35997=CARTESIAN_POINT('Ctrl Pts',(-0.230432675646478,-0.00135759386813896,
-0.00180947422108362));
#35998=CARTESIAN_POINT('Ctrl Pts',(-0.23040508727447,-0.00135980650476992,
-0.00175508457010705));
#35999=CARTESIAN_POINT('Ctrl Pts',(-0.2303785700858,-0.00136200554182681,
-0.00169961760553389));
#36000=CARTESIAN_POINT('Ctrl Pts',(-0.23035438300816,-0.00136405859429202,
-0.00164604882941069));
#36001=CARTESIAN_POINT('Ctrl Pts',(-0.230330195930519,-0.00136611164675724,
-0.00159248005328749));
#36002=CARTESIAN_POINT('Ctrl Pts',(-0.230308335987054,-0.00136801871463078,
-0.0015407943852381));
#36003=CARTESIAN_POINT('Ctrl Pts',(-0.230289909162091,-0.00136966752380675,
-0.00149506721402873));
#36004=CARTESIAN_POINT('Ctrl Pts',(-0.230271482337128,-0.00137131633298271,
-0.00144934004281937));
#36005=CARTESIAN_POINT('Ctrl Pts',(-0.230256225289845,-0.00137270688346108,
-0.00140968640751628));
#36006=CARTESIAN_POINT('Ctrl Pts',(-0.230237435583795,-0.00137442065668314,
-0.00135761151067073));
#36007=CARTESIAN_POINT('Ctrl Pts',(-0.230218645877745,-0.00137613442990519,
-0.00130553661382518));
#36008=CARTESIAN_POINT('Ctrl Pts',(-0.230196798002912,-0.00137817142587091,
-0.00124086583214421));
#36009=CARTESIAN_POINT('Ctrl Pts',(-0.230177928184924,-0.00137996828035668,
-0.00117973176629321));
#36010=CARTESIAN_POINT('',(-0.230090092993501,-0.00138849741546914,0.000844172494537475));
#36011=CARTESIAN_POINT('Ctrl Pts',(-0.230177928184924,-0.00137996828035668,
-0.00117973176629321));
#36012=CARTESIAN_POINT('Ctrl Pts',(-0.230159058366936,-0.00138176513484245,
-0.00111859770044221));
#36013=CARTESIAN_POINT('Ctrl Pts',(-0.230142844554009,-0.00138332184784826,
-0.00106109506496594));
#36014=CARTESIAN_POINT('Ctrl Pts',(-0.230127856833695,-0.00138477612973666,
-0.00100324837385142));
#36015=CARTESIAN_POINT('Ctrl Pts',(-0.230097881393066,-0.00138768469351348,
-0.000887554991622391));
#36016=CARTESIAN_POINT('Ctrl Pts',(-0.230073193248961,-0.00139018353282069,
-0.000770398928202508));
#36017=CARTESIAN_POINT('Ctrl Pts',(-0.230054246319814,-0.00139217250561596,
-0.000656527147420392));
#36018=CARTESIAN_POINT('Ctrl Pts',(-0.230016352461521,-0.00139615045120648,
-0.000428783585856158));
#36019=CARTESIAN_POINT('Ctrl Pts',(-0.229999991480358,-0.00139808893074921,
-0.000214343200170112));
#36020=CARTESIAN_POINT('Ctrl Pts',(-0.230000000003157,-0.00139808796585182,
1.58931735004758E-7));
#36021=CARTESIAN_POINT('Ctrl Pts',(-0.230000008525956,-0.00139808700095444,
0.000214661063640121));
#36022=CARTESIAN_POINT('Ctrl Pts',(-0.230016386700035,-0.00139614659161695,
0.000429102397676562));
#36023=CARTESIAN_POINT('Ctrl Pts',(-0.230054299127194,-0.00139216694241518,
0.000656844443027331));
#36024=CARTESIAN_POINT('Ctrl Pts',(-0.230064575031583,-0.00139108828568537,
0.000718572368636326));
#36025=CARTESIAN_POINT('Ctrl Pts',(-0.230076537999235,-0.00138985981742396,
0.000781265223738882));
#36026=CARTESIAN_POINT('Ctrl Pts',(-0.230090092993501,-0.00138849741546914,
0.000844172494537474));
#36027=CARTESIAN_POINT('',(-0.230631851022661,-0.00134262389237757,0.00215767756313376));
#36028=CARTESIAN_POINT('Ctrl Pts',(-0.230090092993501,-0.00138849741546914,
0.000844172494537474));
#36029=CARTESIAN_POINT('Ctrl Pts',(-0.230101586445131,-0.00138734656102728,
0.000897305354721647));
#36030=CARTESIAN_POINT('Ctrl Pts',(-0.230114209192546,-0.0013861001369068,
0.000950592216182026));
#36031=CARTESIAN_POINT('Ctrl Pts',(-0.230127941497652,-0.0013847677136554,
0.00100357508657684));
#36032=CARTESIAN_POINT('Ctrl Pts',(-0.230142935923704,-0.00138331282885944,
0.00106142755387902));
#36033=CARTESIAN_POINT('Ctrl Pts',(-0.230159157926241,-0.00138175541030722,
0.00111893911964585));
#36034=CARTESIAN_POINT('Ctrl Pts',(-0.230178031105433,-0.00137995842001515,
0.00118006515453991));
#36035=CARTESIAN_POINT('Ctrl Pts',(-0.230196904284625,-0.00137816142972308,
0.00124119118943398));
#36036=CARTESIAN_POINT('Ctrl Pts',(-0.23021874909407,-0.00137612486769115,
0.00130583742520534));
#36037=CARTESIAN_POINT('Ctrl Pts',(-0.230237558682426,-0.00137440934020132,
0.0013579526250255));
#36038=CARTESIAN_POINT('Ctrl Pts',(-0.230256368270783,-0.0013726938127115,
0.00141006782484567));
#36039=CARTESIAN_POINT('Ctrl Pts',(-0.230271669717474,-0.00137129931976377,
0.00144982607665868));
#36040=CARTESIAN_POINT('Ctrl Pts',(-0.230290148658564,-0.00136964611118522,
0.00149566140033204));
#36041=CARTESIAN_POINT('Ctrl Pts',(-0.230308627599653,-0.00136799290260666,
0.0015414967240054));
#36042=CARTESIAN_POINT('Ctrl Pts',(-0.230330546798724,-0.00136608097839726,
0.00159329422029309));
#36043=CARTESIAN_POINT('Ctrl Pts',(-0.230354813070871,-0.00136402176524664,
0.00164700098715987));
#36044=CARTESIAN_POINT('Ctrl Pts',(-0.230379079343017,-0.00136196255209602,
0.00170070775402666));
#36045=CARTESIAN_POINT('Ctrl Pts',(-0.230405696697909,-0.00135975605000417,
0.00175633858822025));
#36046=CARTESIAN_POINT('Ctrl Pts',(-0.230433388432851,-0.0013575363023856,
0.0018108787726071));
#36047=CARTESIAN_POINT('Ctrl Pts',(-0.230461080167794,-0.00135531655476703,
0.00186541895699396));
#36048=CARTESIAN_POINT('Ctrl Pts',(-0.230489531299431,-0.00135308356162173,
0.00191899887599725));
#36049=CARTESIAN_POINT('Ctrl Pts',(-0.230527819237574,-0.00135018972260209,
0.00198594077279254));
#36050=CARTESIAN_POINT('Ctrl Pts',(-0.230560639448383,-0.00134770913964887,
0.00204332299997208));
#36051=CARTESIAN_POINT('Ctrl Pts',(-0.230601554664194,-0.00134474297874676,
0.00211004895575857));
#36052=CARTESIAN_POINT('Ctrl Pts',(-0.230631851022661,-0.00134262389237757,
0.00215767756313376));
#36053=CARTESIAN_POINT('',(-0.230921436098924,-0.00131911515712292,0.00255390765436055));
#36054=CARTESIAN_POINT('Ctrl Pts',(-0.230631851022661,-0.00134262389237757,
0.00215767756313376));
#36055=CARTESIAN_POINT('Ctrl Pts',(-0.230636938528349,-0.00134227086032266,
0.00216558622571961));
#36056=CARTESIAN_POINT('Ctrl Pts',(-0.230641697776003,-0.00134194133826565,
0.00217298659707199));
#36057=CARTESIAN_POINT('Ctrl Pts',(-0.230646076892515,-0.00134164148808831,
0.00217972470488308));
#36058=CARTESIAN_POINT('Ctrl Pts',(-0.230676741798038,-0.00133954177748817,
0.00222690852355222));
#36059=CARTESIAN_POINT('Ctrl Pts',(-0.230687445580514,-0.00133889704118191,
0.00224249809727657));
#36060=CARTESIAN_POINT('Ctrl Pts',(-0.230711699376962,-0.00133711083075126,
0.0022775159741538));
#36061=CARTESIAN_POINT('Ctrl Pts',(-0.230735953173409,-0.00133532462032062,
0.00231253385103102));
#36062=CARTESIAN_POINT('Ctrl Pts',(-0.230774523982444,-0.0013323969357656,
0.00236643847055));
#36063=CARTESIAN_POINT('Ctrl Pts',(-0.230811381856284,-0.00132929059247327,
0.00241510130917168));
#36064=CARTESIAN_POINT('Ctrl Pts',(-0.230848239724272,-0.00132618424967403,
0.00246376414006875));
#36065=CARTESIAN_POINT('Ctrl Pts',(-0.230882962056323,-0.0013228992481942,
0.00250752978309291));
#36066=CARTESIAN_POINT('Ctrl Pts',(-0.230921436078578,-0.00131911464972426,
0.00255390762983318));
#36067=CARTESIAN_POINT('',(-0.230921436096816,-0.00121884929995214,0.00255390765181725));
#36068=CARTESIAN_POINT('',(-0.2309214360969,-0.00203858085746875,0.00255390765191894));
#36069=CARTESIAN_POINT('',(-0.230686015102297,-0.00123880444284725,0.00223997859315595));
#36070=CARTESIAN_POINT('Ctrl Pts',(-0.230921436096798,-0.00121884929952187,
0.0025539076517962));
#36071=CARTESIAN_POINT('Ctrl Pts',(-0.230882799449418,-0.00122268836356969,
0.00250733377201141));
#36072=CARTESIAN_POINT('Ctrl Pts',(-0.230848935241631,-0.00122594473354211,
0.00246470149188065));
#36073=CARTESIAN_POINT('Ctrl Pts',(-0.230810937523616,-0.00122916575459618,
0.00241451455197912));
#36074=CARTESIAN_POINT('Ctrl Pts',(-0.2307729398056,-0.00123238677565026,
0.00236432761207759));
#36075=CARTESIAN_POINT('Ctrl Pts',(-0.230731466942441,-0.00123557244778599,
0.00230607861984655));
#36076=CARTESIAN_POINT('Ctrl Pts',(-0.230710893414538,-0.00123708073550189,
0.00227635187734016));
#36077=CARTESIAN_POINT('Ctrl Pts',(-0.230700606650587,-0.00123783487935984,
0.00226148850608696));
#36078=CARTESIAN_POINT('Ctrl Pts',(-0.230695395139944,-0.00123816967711283,
0.00225385609323441));
#36079=CARTESIAN_POINT('Ctrl Pts',(-0.230686015102297,-0.00123880444284725,
0.00223997859315595));
#36080=CARTESIAN_POINT('',(-0.230177916607466,-0.00127992933296153,0.00117969425721745));
#36081=CARTESIAN_POINT('Ctrl Pts',(-0.230686015102297,-0.00123880444284725,
0.00223997859315595));
#36082=CARTESIAN_POINT('Ctrl Pts',(-0.23067663506465,-0.00123943920858166,
0.00222610109307748));
#36083=CARTESIAN_POINT('Ctrl Pts',(-0.230663124603842,-0.0012403739422975,
0.00220595594828946));
#36084=CARTESIAN_POINT('Ctrl Pts',(-0.23064607382111,-0.00124156614273087,
0.00217971997893273));
#36085=CARTESIAN_POINT('Ctrl Pts',(-0.230611972255647,-0.0012439505435976,
0.00212724804021926));
#36086=CARTESIAN_POINT('Ctrl Pts',(-0.230564381867535,-0.00124736481133447,
0.00204995014329134));
#36087=CARTESIAN_POINT('Ctrl Pts',(-0.230526713362572,-0.00125020352011288,
0.00198400603181192));
#36088=CARTESIAN_POINT('Ctrl Pts',(-0.23048904485761,-0.00125304222889129,
0.00191806192033251));
#36089=CARTESIAN_POINT('Ctrl Pts',(-0.230460339630388,-0.00125530537871126,
0.00186401604814319));
#36090=CARTESIAN_POINT('Ctrl Pts',(-0.230432634059847,-0.00125753302523568,
0.00180939223194782));
#36091=CARTESIAN_POINT('Ctrl Pts',(-0.230404928489305,-0.0012597606717601,
0.00175476841575245));
#36092=CARTESIAN_POINT('Ctrl Pts',(-0.230378492299106,-0.00126195281498897,
0.00169944971928871));
#36093=CARTESIAN_POINT('Ctrl Pts',(-0.230354332272838,-0.00126400452606611,
0.00164593645780533));
#36094=CARTESIAN_POINT('Ctrl Pts',(-0.230330172246571,-0.00126605623714324,
0.00159242319632194));
#36095=CARTESIAN_POINT('Ctrl Pts',(-0.230308296038245,-0.00126796751606864,
0.00154069824975554));
#36096=CARTESIAN_POINT('Ctrl Pts',(-0.230289875122175,-0.00126961802260417,
0.00149498273934548));
#36097=CARTESIAN_POINT('Ctrl Pts',(-0.230271454206105,-0.00127126852913971,
0.00144926722893541));
#36098=CARTESIAN_POINT('Ctrl Pts',(-0.230256221881221,-0.0012726582632854,
0.00140967676806264));
#36099=CARTESIAN_POINT('Ctrl Pts',(-0.23023743718714,-0.00127437351484988,
0.00135761595426707));
#36100=CARTESIAN_POINT('Ctrl Pts',(-0.230218652493058,-0.00127608876641436,
0.00130555514047149));
#36101=CARTESIAN_POINT('Ctrl Pts',(-0.230196792075838,-0.00127812953539765,
0.00124084875869349));
#36102=CARTESIAN_POINT('Ctrl Pts',(-0.230177916607466,-0.00127992933296153,
0.00117969425721745));
#36103=CARTESIAN_POINT('',(-0.230089138316471,-0.00128856509794021,-0.00083973858569693));
#36104=CARTESIAN_POINT('Ctrl Pts',(-0.230177916607466,-0.00127992933296153,
0.00117969425721745));
#36105=CARTESIAN_POINT('Ctrl Pts',(-0.230159041139093,-0.00128172913052541,
0.00111853975574141));
#36106=CARTESIAN_POINT('Ctrl Pts',(-0.230142827170788,-0.00128328795666989,
0.00106103218438422));
#36107=CARTESIAN_POINT('Ctrl Pts',(-0.230127839090187,-0.00128474428551632,
0.00100317988841401));
#36108=CARTESIAN_POINT('Ctrl Pts',(-0.230097862928986,-0.00128765694320919,
0.000887475296473585));
#36109=CARTESIAN_POINT('Ctrl Pts',(-0.230073174819639,-0.00129015961170986,
0.000770305086855483));
#36110=CARTESIAN_POINT('Ctrl Pts',(-0.23005423052057,-0.00129215159395536,
0.000656432186292065));
#36111=CARTESIAN_POINT('Ctrl Pts',(-0.230016341922432,-0.00129613555844635,
0.000428686385165228));
#36112=CARTESIAN_POINT('Ctrl Pts',(-0.229999991618744,-0.00129807677791666,
0.000214296247717829));
#36113=CARTESIAN_POINT('Ctrl Pts',(-0.230000000003057,-0.0012980758241512,
-1.56385361932959E-7));
#36114=CARTESIAN_POINT('Ctrl Pts',(-0.23000000838737,-0.00129807487038574,
-0.000214609018441695));
#36115=CARTESIAN_POINT('Ctrl Pts',(-0.230016375665871,-0.00129613174338452,
-0.00042900110087048));
#36116=CARTESIAN_POINT('Ctrl Pts',(-0.2300542827742,-0.00129214607791548,
-0.000656746202139764));
#36117=CARTESIAN_POINT('Ctrl Pts',(-0.230064320562544,-0.00129109067516511,
-0.000717053021196674));
#36118=CARTESIAN_POINT('Ctrl Pts',(-0.230075969322042,-0.00128989205197605,
-0.000778284469665095));
#36119=CARTESIAN_POINT('Ctrl Pts',(-0.230089138316471,-0.00128856509794021,
-0.00083973858569693));
#36120=CARTESIAN_POINT('',(-0.230625302305309,-0.00124302410204978,-0.00214742065498236));
#36121=CARTESIAN_POINT('Ctrl Pts',(-0.230089138316471,-0.00128856509794021,
-0.00083973858569693));
#36122=CARTESIAN_POINT('Ctrl Pts',(-0.230100879996404,-0.00128738647063385,
-0.000894316709739802));
#36123=CARTESIAN_POINT('Ctrl Pts',(-0.230113816044822,-0.00128610659862752,
-0.000949071248456438));
#36124=CARTESIAN_POINT('Ctrl Pts',(-0.230127923152874,-0.00128473591577273,
-0.00100350430489781));
#36125=CARTESIAN_POINT('Ctrl Pts',(-0.230142917929652,-0.00128327898474434,
-0.00106136248020177));
#36126=CARTESIAN_POINT('Ctrl Pts',(-0.230159140066374,-0.00128171945503964,
-0.00111887904402635));
#36127=CARTESIAN_POINT('Ctrl Pts',(-0.230178018970065,-0.00127991951244512,
-0.0011800258500632));
#36128=CARTESIAN_POINT('Ctrl Pts',(-0.230196897873756,-0.0012781195698506,
-0.00124117265610004));
#36129=CARTESIAN_POINT('Ctrl Pts',(-0.230218755423235,-0.00127607921436627,
-0.00130585509784703));
#36130=CARTESIAN_POINT('Ctrl Pts',(-0.230237559819384,-0.00127436222761337,
-0.00135795577515773));
#36131=CARTESIAN_POINT('Ctrl Pts',(-0.230256364215533,-0.00127264524086048,
-0.00141005645246844));
#36132=CARTESIAN_POINT('Ctrl Pts',(-0.230271640302773,-0.00127125162283904,
-0.00144975005927987));
#36133=CARTESIAN_POINT('Ctrl Pts',(-0.230290114091531,-0.00126959663178466,
-0.00149557565711002));
#36134=CARTESIAN_POINT('Ctrl Pts',(-0.230308587880288,-0.00126794164073029,
-0.00154140125494016));
#36135=CARTESIAN_POINT('Ctrl Pts',(-0.23033052579338,-0.00126602527664298,
-0.00159324329923622));
#36136=CARTESIAN_POINT('Ctrl Pts',(-0.230354762074236,-0.00126396768010872,
-0.00164688811537833));
#36137=CARTESIAN_POINT('Ctrl Pts',(-0.230378998355092,-0.00126191008357446,
-0.00170053293152045));
#36138=CARTESIAN_POINT('Ctrl Pts',(-0.230405525206895,-0.00125971125459324,
-0.00175599774203875));
#36139=CARTESIAN_POINT('Ctrl Pts',(-0.230433347291843,-0.00125747537258556,
-0.00181079774116085));
#36140=CARTESIAN_POINT('Ctrl Pts',(-0.23046116937679,-0.00125523949057789,
-0.00186559774028295));
#36141=CARTESIAN_POINT('Ctrl Pts',(-0.230490017676975,-0.00125296655554375,
-0.00191984949807499));
#36142=CARTESIAN_POINT('Ctrl Pts',(-0.230527822460804,-0.00125011970921519,
-0.0019859464082148));
#36143=CARTESIAN_POINT('Ctrl Pts',(-0.230558007660088,-0.00124784664705071,
-0.00203872143302736));
#36144=CARTESIAN_POINT('Ctrl Pts',(-0.230594516023534,-0.0012452077043151,
-0.00209869927530583));
#36145=CARTESIAN_POINT('Ctrl Pts',(-0.230625302305309,-0.00124302410204978,
-0.00214742065498236));
#36146=CARTESIAN_POINT('Ctrl Pts',(-0.230625302305309,-0.00124302410204978,
-0.00214742065498236));
#36147=CARTESIAN_POINT('Ctrl Pts',(-0.230633137488449,-0.00124247290005448,
-0.00215967828816978));
#36148=CARTESIAN_POINT('Ctrl Pts',(-0.230640560315198,-0.0012419507122686,
-0.00217124931158208));
#36149=CARTESIAN_POINT('Ctrl Pts',(-0.230647428858057,-0.0012414707477488,
-0.00218180355170074));
#36150=CARTESIAN_POINT('Ctrl Pts',(-0.230664468092708,-0.00124028006899138,
-0.00220798613185289));
#36151=CARTESIAN_POINT('Ctrl Pts',(-0.230677927294496,-0.001239349240261,
-0.00222802755915694));
#36152=CARTESIAN_POINT('Ctrl Pts',(-0.230687201831431,-0.00123872188163988,
-0.00224173332364162));
#36153=CARTESIAN_POINT('Ctrl Pts',(-0.230696476368366,-0.00123809452301875,
-0.0022554390881263));
#36154=CARTESIAN_POINT('Ctrl Pts',(-0.230701528656117,-0.00123777063450688,
-0.00226283144073695));
#36155=CARTESIAN_POINT('Ctrl Pts',(-0.230711703464447,-0.00123702342528048,
-0.00227752187569489));
#36156=CARTESIAN_POINT('Ctrl Pts',(-0.230732053081106,-0.00123552900682768,
-0.00230690274561076));
#36157=CARTESIAN_POINT('Ctrl Pts',(-0.230773490719382,-0.00123234130551679,
-0.0023650743467824));
#36158=CARTESIAN_POINT('Ctrl Pts',(-0.230811383628898,-0.00122912706120165,
-0.00241510364952272));
#36159=CARTESIAN_POINT('Ctrl Pts',(-0.230849276538414,-0.00122591281688652,
-0.00246513295226304));
#36160=CARTESIAN_POINT('Ctrl Pts',(-0.230882962553088,-0.00122267202956712,
-0.00250753038251587));
#36161=CARTESIAN_POINT('Ctrl Pts',(-0.230921436096799,-0.00121884911930227,
-0.0025539076517966));
#36162=CARTESIAN_POINT('Origin',(-0.234,-0.00203858085746875,0.));
#36163=CARTESIAN_POINT('',(-0.230921436096816,0.0162188492999508,0.00255390765181756));
#36164=CARTESIAN_POINT('',(-0.230921436098932,0.0163191151589042,0.00255390765437054));
#36165=CARTESIAN_POINT('',(-0.2309214360969,-0.00203858085746875,0.00255390765191894));
#36166=CARTESIAN_POINT('',(-0.230644548883471,0.0163417486711327,0.00217737176535899));
#36167=CARTESIAN_POINT('Ctrl Pts',(-0.230921436078515,0.0163191146497307,
0.0025539076297574));
#36168=CARTESIAN_POINT('Ctrl Pts',(-0.230882799131686,0.0163229152747047,
0.00250733338839475));
#36169=CARTESIAN_POINT('Ctrl Pts',(-0.230847896612009,0.0163262157976892,
0.00246332973319459));
#36170=CARTESIAN_POINT('Ctrl Pts',(-0.230810936306616,0.0163293288041934,
0.00241451294457891));
#36171=CARTESIAN_POINT('Ctrl Pts',(-0.230773975995361,0.0163324418111914,
0.00236569614822039));
#36172=CARTESIAN_POINT('Ctrl Pts',(-0.230735375247888,0.0163353673016496,
0.00231172583822521));
#36173=CARTESIAN_POINT('Ctrl Pts',(-0.230710890465089,0.0163371675185938,
0.00227634761566747));
#36174=CARTESIAN_POINT('Ctrl Pts',(-0.230686405682289,0.016338967735538,
0.00224096939310972));
#36175=CARTESIAN_POINT('Ctrl Pts',(-0.23067527434207,0.0163396426789682,
0.00222472140771315));
#36176=CARTESIAN_POINT('Ctrl Pts',(-0.230644548883471,0.0163417486711327,
0.00217737176535899));
#36177=CARTESIAN_POINT('',(-0.23017792818303,0.0163799682805405,0.00117973176015849));
#36178=CARTESIAN_POINT('Ctrl Pts',(-0.230644548883471,0.0163417486711327,
0.00217737176535899));
#36179=CARTESIAN_POINT('Ctrl Pts',(-0.230613823424872,0.0163438546632971,
0.00213002212300482));
#36180=CARTESIAN_POINT('Ctrl Pts',(-0.230564811116794,0.016347391704196,
0.00205070172250556));
#36181=CARTESIAN_POINT('Ctrl Pts',(-0.230526711864591,0.0163502733457859,
0.00198400340937967));
#36182=CARTESIAN_POINT('Ctrl Pts',(-0.230488612612389,0.0163531549873758,
0.00191730509625378));
#36183=CARTESIAN_POINT('Ctrl Pts',(-0.230460264039213,0.0163553812296567,
0.00186386391325319));
#36184=CARTESIAN_POINT('Ctrl Pts',(-0.230432675642059,0.0163575938684977,
0.0018094742123716));
#36185=CARTESIAN_POINT('Ctrl Pts',(-0.230405087244905,0.0163598065073388,
0.00175508451149002));
#36186=CARTESIAN_POINT('Ctrl Pts',(-0.230378570075895,0.0163620055427398,
0.00169961758389459));
#36187=CARTESIAN_POINT('Ctrl Pts',(-0.230354383004713,0.0163640585945882,
0.00164604882177632));
#36188=CARTESIAN_POINT('Ctrl Pts',(-0.23033019593353,0.0163661116464366,
0.00159248005965805));
#36189=CARTESIAN_POINT('Ctrl Pts',(-0.230308335985599,0.0163680187147322,
0.00154079438187499));
#36190=CARTESIAN_POINT('Ctrl Pts',(-0.230289909159302,0.0163696675240572,
0.00149506720710742));
#36191=CARTESIAN_POINT('Ctrl Pts',(-0.230271482333005,0.0163713163333821,
0.00144934003233984));
#36192=CARTESIAN_POINT('Ctrl Pts',(-0.230256225286953,0.0163727068837364,
0.00140968639978936));
#36193=CARTESIAN_POINT('Ctrl Pts',(-0.23023743558141,0.0163744206569048,
0.00135761150406173));
#36194=CARTESIAN_POINT('Ctrl Pts',(-0.230218645875867,0.0163761344300732,
0.00130553660833409));
#36195=CARTESIAN_POINT('Ctrl Pts',(-0.230196798000944,0.0163781714260557,
0.0012408658261171));
#36196=CARTESIAN_POINT('Ctrl Pts',(-0.23017792818303,0.0163799682805405,
0.00117973176015849));
#36197=CARTESIAN_POINT('',(-0.230090093999453,0.0163884973145555,-0.000844177153733135));
#36198=CARTESIAN_POINT('Ctrl Pts',(-0.23017792818303,0.0163799682805405,
0.00117973176015849));
#36199=CARTESIAN_POINT('Ctrl Pts',(-0.230159058365117,0.0163817651350253,
0.00111859769419988));
#36200=CARTESIAN_POINT('Ctrl Pts',(-0.230142844552385,0.0163833218480123,
0.00106109505904679));
#36201=CARTESIAN_POINT('Ctrl Pts',(-0.230127856832223,0.0163847761298856,
0.00100324836817062));
#36202=CARTESIAN_POINT('Ctrl Pts',(-0.230097881391899,0.0163876846936321,
0.000887554986418291));
#36203=CARTESIAN_POINT('Ctrl Pts',(-0.230073193247974,0.0163901835329237,
0.000770398923136304));
#36204=CARTESIAN_POINT('Ctrl Pts',(-0.230054246319006,0.0163921725057037,
0.000656527142561015));
#36205=CARTESIAN_POINT('Ctrl Pts',(-0.230016352461069,0.0163961504512636,
0.000428783581410437));
#36206=CARTESIAN_POINT('Ctrl Pts',(-0.229999991480161,0.016398088930777,
0.000214343196413871));
#36207=CARTESIAN_POINT('Ctrl Pts',(-0.230000000003158,0.0163980879658518,
-1.58935424071983E-7));
#36208=CARTESIAN_POINT('Ctrl Pts',(-0.230000008526154,0.0163980870009266,
-0.000214661067262015));
#36209=CARTESIAN_POINT('Ctrl Pts',(-0.230016386700467,0.0163961465915627,
-0.000429102401853301));
#36210=CARTESIAN_POINT('Ctrl Pts',(-0.230054299127932,0.0163921669423355,
-0.000656844447461795));
#36211=CARTESIAN_POINT('Ctrl Pts',(-0.230064575285859,0.0163910882589937,
-0.000718573895662374));
#36212=CARTESIAN_POINT('Ctrl Pts',(-0.230076538590272,0.0163898597567301,
-0.000781268320935413));
#36213=CARTESIAN_POINT('Ctrl Pts',(-0.230090093999453,0.0163884973145555,
-0.000844177153733135));
#36214=CARTESIAN_POINT('',(-0.230631848315212,0.0163426240801819,-0.00215767333678148));
#36215=CARTESIAN_POINT('Ctrl Pts',(-0.230090093999453,0.0163884973145555,
-0.000844177153733135));
#36216=CARTESIAN_POINT('Ctrl Pts',(-0.230101587183355,0.016387346488129,
-0.00089730847127423));
#36217=CARTESIAN_POINT('Ctrl Pts',(-0.230114209594691,0.0163861000978827,
-0.000950593768044107));
#36218=CARTESIAN_POINT('Ctrl Pts',(-0.230127941498946,0.0163847677135248,
-0.00100357509156707));
#36219=CARTESIAN_POINT('Ctrl Pts',(-0.230142935925125,0.016383312828716,
-0.00106142755905526));
#36220=CARTESIAN_POINT('Ctrl Pts',(-0.230159157927828,0.0163817554101476,
-0.00111893912508747));
#36221=CARTESIAN_POINT('Ctrl Pts',(-0.23017803110707,0.0163799584198563,
-0.00118006515984195));
#36222=CARTESIAN_POINT('Ctrl Pts',(-0.230196904286312,0.0163781614295651,
-0.00124119119459644));
#36223=CARTESIAN_POINT('Ctrl Pts',(-0.230218749095649,0.016376124867551,
-0.00130583742982536));
#36224=CARTESIAN_POINT('Ctrl Pts',(-0.230237558684458,0.0163744093400124,
-0.00135795263065568));
#36225=CARTESIAN_POINT('Ctrl Pts',(-0.230256368273268,0.0163726938124738,
-0.001410067831486));
#36226=CARTESIAN_POINT('Ctrl Pts',(-0.230271669721095,0.0163712993194106,
-0.00144982608584323));
#36227=CARTESIAN_POINT('Ctrl Pts',(-0.23029014866085,0.0163696461109798,
-0.00149566140600394));
#36228=CARTESIAN_POINT('Ctrl Pts',(-0.230308627600605,0.0163679929025489,
-0.00154149672616465));
#36229=CARTESIAN_POINT('Ctrl Pts',(-0.23033054679533,0.0163660809787502,
-0.00159329421301259));
#36230=CARTESIAN_POINT('Ctrl Pts',(-0.230354813073543,0.0163640217650164,
-0.00164700099307509));
#36231=CARTESIAN_POINT('Ctrl Pts',(-0.230379079351757,0.0163619625512826,
-0.0017007077731376));
#36232=CARTESIAN_POINT('Ctrl Pts',(-0.23040569672531,0.0163597560476136,
-0.00175633864242895));
#36233=CARTESIAN_POINT('Ctrl Pts',(-0.230433388436071,0.0163575363021224,
-0.001810878778949));
#36234=CARTESIAN_POINT('Ctrl Pts',(-0.230461080146832,0.0163553165566312,
-0.00186541891546905));
#36235=CARTESIAN_POINT('Ctrl Pts',(-0.230489531202867,0.0163530835693178,
-0.00191899870747605));
#36236=CARTESIAN_POINT('Ctrl Pts',(-0.230527819241536,0.0163501897222977,
-0.00198594077971958));
#36237=CARTESIAN_POINT('Ctrl Pts',(-0.230560638422925,0.016347709216804,
-0.00204332120681471));
#36238=CARTESIAN_POINT('Ctrl Pts',(-0.230601552207351,0.0163447431562081,
-0.00211004493906512));
#36239=CARTESIAN_POINT('Ctrl Pts',(-0.230631848315212,0.0163426240801819,
-0.00215767333678148));
#36240=CARTESIAN_POINT('Ctrl Pts',(-0.230631848315212,0.0163426240801819,
-0.00215767333678148));
#36241=CARTESIAN_POINT('Ctrl Pts',(-0.230636936996691,0.0163422709658182,
-0.00216558384271426));
#36242=CARTESIAN_POINT('Ctrl Pts',(-0.23064169730074,0.0163419413701478,
-0.00217298586863137));
#36243=CARTESIAN_POINT('Ctrl Pts',(-0.230646077312613,0.0163416414589317,
-0.00217972535128352));
#36244=CARTESIAN_POINT('Ctrl Pts',(-0.230676742231324,0.0163395417493127,
-0.00222690917034205));
#36245=CARTESIAN_POINT('Ctrl Pts',(-0.230687445717667,0.0163388970368014,
-0.00224249829545137));
#36246=CARTESIAN_POINT('Ctrl Pts',(-0.230711699381587,0.0163371108294283,
-0.00227751598083233));
#36247=CARTESIAN_POINT('Ctrl Pts',(-0.230735953045507,0.0163353246220552,
-0.00231253366621329));
#36248=CARTESIAN_POINT('Ctrl Pts',(-0.230774523891339,0.0163323969198203,
-0.00236643834730859));
#36249=CARTESIAN_POINT('Ctrl Pts',(-0.230811381785659,0.0163292905470285,
-0.00241510121592747));
#36250=CARTESIAN_POINT('Ctrl Pts',(-0.230848239674129,0.0163261841747298,
-0.00246376407682237));
#36251=CARTESIAN_POINT('Ctrl Pts',(-0.230882962005671,0.016322899131931,
-0.00250752972203446));
#36252=CARTESIAN_POINT('Ctrl Pts',(-0.23092143607858,0.0163191144773501,
-0.00255390762983496));
#36253=CARTESIAN_POINT('',(-0.230686015407516,0.016238804421674,-0.00223997904471846));
#36254=CARTESIAN_POINT('Ctrl Pts',(-0.230921436096798,0.0162188491192965,
-0.0025539076517962));
#36255=CARTESIAN_POINT('Ctrl Pts',(-0.230882799397051,0.0162226882415039,
-0.00250733370888625));
#36256=CARTESIAN_POINT('Ctrl Pts',(-0.230848935196512,0.0162259446534774,
-0.00246470143542876));
#36257=CARTESIAN_POINT('Ctrl Pts',(-0.230810937450868,0.0162291657062486,
-0.00241451445589385));
#36258=CARTESIAN_POINT('Ctrl Pts',(-0.230772939705224,0.0162323867590198,
-0.00236432747635895));
#36259=CARTESIAN_POINT('Ctrl Pts',(-0.230731466785859,0.0162355724525887,
-0.00230607839344163));
#36260=CARTESIAN_POINT('Ctrl Pts',(-0.230710893420252,0.0162370807338301,
-0.00227635188559671));
#36261=CARTESIAN_POINT('Ctrl Pts',(-0.230700606737449,0.0162378348744508,
-0.00226148863167426));
#36262=CARTESIAN_POINT('Ctrl Pts',(-0.23069539536208,0.0162381696619895,
-0.00225385641780176));
#36263=CARTESIAN_POINT('Ctrl Pts',(-0.230686015407516,0.016238804421674,
-0.00223997904471846));
#36264=CARTESIAN_POINT('',(-0.230177916609458,0.0162799293327684,-0.00117969426367131));
#36265=CARTESIAN_POINT('Ctrl Pts',(-0.230686015407516,0.016238804421674,
-0.00223997904471846));
#36266=CARTESIAN_POINT('Ctrl Pts',(-0.230676635452952,0.0162394391813584,
-0.00222610167163516));
#36267=CARTESIAN_POINT('Ctrl Pts',(-0.230663125022571,0.0162403739131886,
-0.00220595658219773));
#36268=CARTESIAN_POINT('Ctrl Pts',(-0.230646074215495,0.0162415661152585,
-0.00217972058576994));
#36269=CARTESIAN_POINT('Ctrl Pts',(-0.230611972601341,0.0162439505193984,
-0.00212724859291435));
#36270=CARTESIAN_POINT('Ctrl Pts',(-0.230564381958858,0.0162473648044977,
-0.00204995030269808));
#36271=CARTESIAN_POINT('Ctrl Pts',(-0.230526713368632,0.0162502035196495,
-0.00198400604241944));
#36272=CARTESIAN_POINT('Ctrl Pts',(-0.230489044778405,0.0162530422348013,
-0.0019180617821408));
#36273=CARTESIAN_POINT('Ctrl Pts',(-0.230460339614821,0.0162553053800055,
-0.00186401601710155));
#36274=CARTESIAN_POINT('Ctrl Pts',(-0.230432634064514,0.0162575330248551,
-0.00180939224115048));
#36275=CARTESIAN_POINT('Ctrl Pts',(-0.230404928514207,0.0162597606697047,
-0.00175476846519941));
#36276=CARTESIAN_POINT('Ctrl Pts',(-0.230378492308048,0.0162619528141995,
-0.00169944973877708));
#36277=CARTESIAN_POINT('Ctrl Pts',(-0.230354332276493,0.0162640045257515,
-0.00164593646589942));
#36278=CARTESIAN_POINT('Ctrl Pts',(-0.230330172244938,0.0162660562373035,
-0.00159242319302175));
#36279=CARTESIAN_POINT('Ctrl Pts',(-0.230308296040165,0.0162679675159127,
-0.00154069825426019));
#36280=CARTESIAN_POINT('Ctrl Pts',(-0.230289875125128,0.0162696180223388,
-0.00149498274667557));
#36281=CARTESIAN_POINT('Ctrl Pts',(-0.230271454210092,0.016271268528765,
-0.00144926723909096));
#36282=CARTESIAN_POINT('Ctrl Pts',(-0.230256221884176,0.0162726582630083,
-0.00140967677595122));
#36283=CARTESIAN_POINT('Ctrl Pts',(-0.230237437189646,0.0162743735146171,
-0.00135761596121328));
#36284=CARTESIAN_POINT('Ctrl Pts',(-0.230218652495116,0.0162760887662258,
-0.00130555514647534));
#36285=CARTESIAN_POINT('Ctrl Pts',(-0.230196792077928,0.0162781295352002,
-0.00124084876509567));
#36286=CARTESIAN_POINT('Ctrl Pts',(-0.230177916609458,0.0162799293327684,
-0.00117969426367131));
#36287=CARTESIAN_POINT('',(-0.230089137337594,0.0162885651963867,0.000839734026817373));
#36288=CARTESIAN_POINT('Ctrl Pts',(-0.230177916609458,0.0162799293327684,
-0.00117969426367131));
#36289=CARTESIAN_POINT('Ctrl Pts',(-0.230159041140988,0.0162817291303366,
-0.00111853976224696));
#36290=CARTESIAN_POINT('Ctrl Pts',(-0.230142827172492,0.0162832879564987,
-0.00106103219059277));
#36291=CARTESIAN_POINT('Ctrl Pts',(-0.230127839091737,0.0162847442853598,
-0.00100317989439576));
#36292=CARTESIAN_POINT('Ctrl Pts',(-0.230097862930227,0.0162876569430821,
-0.000887475302001748));
#36293=CARTESIAN_POINT('Ctrl Pts',(-0.230073174820682,0.0162901596116007,
-0.000770305092210906));
#36294=CARTESIAN_POINT('Ctrl Pts',(-0.230054230521423,0.0162921515938631,
-0.000656432191416348));
#36295=CARTESIAN_POINT('Ctrl Pts',(-0.230016341922904,0.0162961355583879,
-0.000428686389827232));
#36296=CARTESIAN_POINT('Ctrl Pts',(-0.229999991618952,0.0162980767778882,
-0.000214296251682201));
#36297=CARTESIAN_POINT('Ctrl Pts',(-0.230000000003057,0.0162980758241512,
1.56381474666943E-7));
#36298=CARTESIAN_POINT('Ctrl Pts',(-0.230000008387162,0.0162980748704142,
0.000214609014631535));
#36299=CARTESIAN_POINT('Ctrl Pts',(-0.230016375665422,0.0162961317434399,
0.000429001096517139));
#36300=CARTESIAN_POINT('Ctrl Pts',(-0.230054282773425,0.0162921460779994,
0.000656746197485573));
#36301=CARTESIAN_POINT('Ctrl Pts',(-0.230064320313722,0.016291090701328,
0.000717051526717664));
#36302=CARTESIAN_POINT('Ctrl Pts',(-0.230075968745583,0.0162898921112937,
0.000778281439696839));
#36303=CARTESIAN_POINT('Ctrl Pts',(-0.230089137337594,0.0162885651963867,
0.000839734026817373));
#36304=CARTESIAN_POINT('',(-0.230625305120942,0.0162430239031887,0.00214742507977825));
#36305=CARTESIAN_POINT('Ctrl Pts',(-0.230089137337594,0.0162885651963867,
0.000839734026817373));
#36306=CARTESIAN_POINT('Ctrl Pts',(-0.230100879275725,0.0162873865419408,
0.000894313659151995));
#36307=CARTESIAN_POINT('Ctrl Pts',(-0.230113815651244,0.0162861066368743,
0.00094906972951125));
#36308=CARTESIAN_POINT('Ctrl Pts',(-0.230127923151515,0.0162847359159103,
0.00100350429965659));
#36309=CARTESIAN_POINT('Ctrl Pts',(-0.230142917928165,0.0162832789848943,
0.00106136247478748));
#36310=CARTESIAN_POINT('Ctrl Pts',(-0.230159140064727,0.0162817194552044,
0.00111887903837501));
#36311=CARTESIAN_POINT('Ctrl Pts',(-0.230178018968344,0.0162799195126125,
0.00118002584448998));
#36312=CARTESIAN_POINT('Ctrl Pts',(-0.230196897871962,0.0162781195700206,
0.00124117265060494));
#36313=CARTESIAN_POINT('Ctrl Pts',(-0.230218755421485,0.0162760792145265,
0.0013058550927437));
#36314=CARTESIAN_POINT('Ctrl Pts',(-0.230237559817246,0.0162743622278125,
0.00135795576923366));
#36315=CARTESIAN_POINT('Ctrl Pts',(-0.230256364213006,0.0162726452410985,
0.00141005644572361));
#36316=CARTESIAN_POINT('Ctrl Pts',(-0.230271640299325,0.0162712516231645,
0.00144975005051676));
#36317=CARTESIAN_POINT('Ctrl Pts',(-0.230290114089152,0.0162695966319987,
0.001495575651209));
#36318=CARTESIAN_POINT('Ctrl Pts',(-0.230308587878978,0.0162679416408329,
0.00154140125190124));
#36319=CARTESIAN_POINT('Ctrl Pts',(-0.230330525795565,0.0162660252764353,
0.00159324330383135));
#36320=CARTESIAN_POINT('Ctrl Pts',(-0.230354762071464,0.0162639676803474,
0.00164688810924254));
#36321=CARTESIAN_POINT('Ctrl Pts',(-0.230378998347364,0.0162619100842594,
0.00170053291465374));
#36322=CARTESIAN_POINT('Ctrl Pts',(-0.230405525183997,0.0162597112564811,
0.00175599769668587));
#36323=CARTESIAN_POINT('Ctrl Pts',(-0.230433347288488,0.0162574753728585,
0.00181079773455379));
#36324=CARTESIAN_POINT('Ctrl Pts',(-0.23046116939298,0.0162552394892359,
0.00186559777242172));
#36325=CARTESIAN_POINT('Ctrl Pts',(-0.230490017754343,0.0162529665497689,
0.00191984963302185));
#36326=CARTESIAN_POINT('Ctrl Pts',(-0.230527822456637,0.0162501197095321,
0.00198594640092935));
#36327=CARTESIAN_POINT('Ctrl Pts',(-0.230558008612418,0.0162478465753012,
0.00203872309831363));
#36328=CARTESIAN_POINT('Ctrl Pts',(-0.230594518257034,0.0162452075424427,
0.00209870295150882));
#36329=CARTESIAN_POINT('Ctrl Pts',(-0.230625305120942,0.0162430239031887,
0.00214742507977825));
#36330=CARTESIAN_POINT('Ctrl Pts',(-0.230625305120942,0.0162430239031887,
0.00214742507977825));
#36331=CARTESIAN_POINT('Ctrl Pts',(-0.230633139129668,0.0162424727844128,
0.00215968084725818));
#36332=CARTESIAN_POINT('Ctrl Pts',(-0.230640560869481,0.0162419506734878,
0.00217125015931671));
#36333=CARTESIAN_POINT('Ctrl Pts',(-0.230647428482022,0.0162414707739622,
0.00218180297388311));
#36334=CARTESIAN_POINT('Ctrl Pts',(-0.230664467693318,0.0162402800967991,
0.00220798552802012));
#36335=CARTESIAN_POINT('Ctrl Pts',(-0.230677926924196,0.0162393492663061,
0.00222802700809956));
#36336=CARTESIAN_POINT('Ctrl Pts',(-0.230687201540453,0.0162387219019087,
0.00224173289363862));
#36337=CARTESIAN_POINT('Ctrl Pts',(-0.23069647615671,0.0162380945375114,
0.00225543877917767));
#36338=CARTESIAN_POINT('Ctrl Pts',(-0.230701528573552,0.0162377706392097,
0.00226283132146126));
#36339=CARTESIAN_POINT('Ctrl Pts',(-0.230711703459589,0.0162370234270096,
0.00227752186868137));
#36340=CARTESIAN_POINT('Ctrl Pts',(-0.230732053231664,0.0162355290026094,
0.00230690296312161));
#36341=CARTESIAN_POINT('Ctrl Pts',(-0.230773490818101,0.0162323413226155,
0.00236507448024538));
#36342=CARTESIAN_POINT('Ctrl Pts',(-0.230811383701533,0.0162291271099321,
0.00241510374542183));
#36343=CARTESIAN_POINT('Ctrl Pts',(-0.230849276584965,0.0162259128972488,
0.00246513301059828));
#36344=CARTESIAN_POINT('Ctrl Pts',(-0.230882962605203,0.0162226721518758,
0.0025075304453366));
#36345=CARTESIAN_POINT('Ctrl Pts',(-0.230921436096799,0.0162188492995221,
0.0025539076517966));
#36346=CARTESIAN_POINT('Origin',(-0.238,-0.00203858085746875,0.0110866403454819));
#36347=CARTESIAN_POINT('',(-0.235510394140372,0.001086028911646,0.00808558792816448));
#36348=CARTESIAN_POINT('Ctrl Pts',(-0.2309214360969,-0.00131911464792199,
0.00255390765191894));
#36349=CARTESIAN_POINT('Ctrl Pts',(-0.23174153296916,-0.00124041124463224,
0.00354247927317125));
#36350=CARTESIAN_POINT('Ctrl Pts',(-0.233359728852528,-0.00077441369596115,
0.00549310557359274));
#36351=CARTESIAN_POINT('Ctrl Pts',(-0.234843968024857,0.000344657188193435,
0.00728225606854703));
#36352=CARTESIAN_POINT('Ctrl Pts',(-0.235510394140372,0.001086028911646,
0.00808558792816448));
#36353=CARTESIAN_POINT('',(-0.23718847822691,0.00385255096193961,0.0101084054295328));
#36354=CARTESIAN_POINT('Ctrl Pts',(-0.235510394140372,0.001086028911646,
0.00808558792816448));
#36355=CARTESIAN_POINT('Ctrl Pts',(-0.236176820255887,0.00182740063509858,
0.00888891978778193));
#36356=CARTESIAN_POINT('Ctrl Pts',(-0.236767552900753,0.00275060863992643,
0.00960100825953967));
#36357=CARTESIAN_POINT('Ctrl Pts',(-0.23718847822691,0.00385255096193961,
0.0101084054295328));
#36358=CARTESIAN_POINT('',(-0.237859981300301,0.00751096248998218,0.0109178572204036));
#36359=CARTESIAN_POINT('Ctrl Pts',(-0.23718847822691,0.00385255096193961,
0.0101084054295328));
#36360=CARTESIAN_POINT('Ctrl Pts',(-0.237609403553067,0.00495449328395277,
0.010615802599526));
#36361=CARTESIAN_POINT('Ctrl Pts',(-0.237860521560515,0.00623516992315125,
0.0109185084677545));
#36362=CARTESIAN_POINT('Ctrl Pts',(-0.237859981300301,0.00751096248998218,
0.0109178572204036));
#36363=CARTESIAN_POINT('Ctrl Pts',(-0.237859981300301,0.00751096248998218,
0.0109178572204036));
#36364=CARTESIAN_POINT('Ctrl Pts',(-0.237859441040087,0.00878675505681313,
0.0109172059730527));
#36365=CARTESIAN_POINT('Ctrl Pts',(-0.237355043984334,0.0113285720457399,
0.0103091892471919));
#36366=CARTESIAN_POINT('Ctrl Pts',(-0.2355790521135,0.0141062321617645,
0.00816835049695678));
#36367=CARTESIAN_POINT('Ctrl Pts',(-0.233347521760492,0.0157787640062935,
0.00547839074517056));
#36368=CARTESIAN_POINT('Ctrl Pts',(-0.23174108105572,0.0162404546140525,
0.00354193452191338));
#36369=CARTESIAN_POINT('Ctrl Pts',(-0.2309214360969,0.0163191146479222,
0.00255390765191895));
#36370=CARTESIAN_POINT('Ctrl Pts',(-0.2309214360969,0.016218849299512,0.00255390765191894));
#36371=CARTESIAN_POINT('Ctrl Pts',(-0.231731717357689,0.0161403008067932,
0.00353064721372319));
#36372=CARTESIAN_POINT('Ctrl Pts',(-0.23253100953097,0.0159094319151459,
0.00449414016964269));
#36373=CARTESIAN_POINT('Ctrl Pts',(-0.233297219375807,0.0155172940805772,
0.00541775460368186));
#36374=CARTESIAN_POINT('Ctrl Pts',(-0.234063429220644,0.0151251562460085,
0.00634136903772102));
#36375=CARTESIAN_POINT('Ctrl Pts',(-0.234796556737038,0.0145717494685186,
0.00722510494987985));
#36376=CARTESIAN_POINT('Ctrl Pts',(-0.235454844320089,0.0138387602641205,
0.00801862635599526));
#36377=CARTESIAN_POINT('Ctrl Pts',(-0.23611313190314,0.0131057710597224,
0.00881214776211065));
#36378=CARTESIAN_POINT('Ctrl Pts',(-0.236696579552848,0.0121931994284161,
0.00951545466218262));
#36379=CARTESIAN_POINT('Ctrl Pts',(-0.237112283509665,0.0111042149244282,
0.0100165578226166));
#36380=CARTESIAN_POINT('Ctrl Pts',(-0.237527987466483,0.0100152304204403,
0.0105176609830505));
#36381=CARTESIAN_POINT('Ctrl Pts',(-0.237775947730408,0.0087498330437706,
0.0108165604038465));
#36382=CARTESIAN_POINT('Ctrl Pts',(-0.237775416984309,0.0074892317112278,
0.0108159206251214));
#36383=CARTESIAN_POINT('Ctrl Pts',(-0.237774886238211,0.006228630378685,
0.0108152808463964));
#36384=CARTESIAN_POINT('Ctrl Pts',(-0.237525864482087,0.00497282509026909,
0.0105151018681504));
#36385=CARTESIAN_POINT('Ctrl Pts',(-0.237109010658239,0.00388732421957286,
0.0100126126203483));
#36386=CARTESIAN_POINT('Ctrl Pts',(-0.236692156834391,0.00280182334887665,
0.00951012337254628));
#36387=CARTESIAN_POINT('Ctrl Pts',(-0.236107470942817,0.00188662689590011,
0.00880532385518818));
#36388=CARTESIAN_POINT('Ctrl Pts',(-0.235447722393476,0.00115331852706932,
0.00801004135247146));
#36389=CARTESIAN_POINT('Ctrl Pts',(-0.234787973844134,0.000420010158238511,
0.00721475884975473));
#36390=CARTESIAN_POINT('Ctrl Pts',(-0.234053162637025,-0.000131410126446554,
0.00632899336167939));
#36391=CARTESIAN_POINT('Ctrl Pts',(-0.233288987015657,-0.000521498676355057,
0.00540783104721498));
#36392=CARTESIAN_POINT('Ctrl Pts',(-0.23252481139429,-0.000911587226263559,
0.00448666873275056));
#36393=CARTESIAN_POINT('Ctrl Pts',(-0.231731271358665,-0.0011403440413955,
0.00353010959189706));
#36394=CARTESIAN_POINT('Ctrl Pts',(-0.2309214360969,-0.00121884929951176,
0.00255390765191896));
#36395=CARTESIAN_POINT('Origin',(-0.194168411395185,0.0075,-0.0165));
#36396=CARTESIAN_POINT('',(-0.192751468456974,0.0155452250459276,-0.0056));
#36397=CARTESIAN_POINT('Ctrl Pts',(-0.186019885831704,0.00807870931483181,
-0.00979684103423184));
#36398=CARTESIAN_POINT('Ctrl Pts',(-0.186089762480249,0.00906260833433668,
-0.00973982032171833));
#36399=CARTESIAN_POINT('Ctrl Pts',(-0.186581784748698,0.0109343901050088,
-0.00933928969553343));
#36400=CARTESIAN_POINT('Ctrl Pts',(-0.188116978636712,0.0131929004294505,
-0.00813962307738));
#36401=CARTESIAN_POINT('Ctrl Pts',(-0.190152702745521,0.0147631592433591,
-0.00671673740186432));
#36402=CARTESIAN_POINT('Ctrl Pts',(-0.191807671769535,0.0153790014730954,
-0.0058522182261825));
#36403=CARTESIAN_POINT('Ctrl Pts',(-0.192751468456974,0.0155452250459276,
-0.0056));
#36404=CARTESIAN_POINT('',(-0.192176438048886,0.0154224627179558,-0.00559999999999961));
#36405=CARTESIAN_POINT('Origin',(-0.194168411395185,0.0075,-0.0056));
#36406=CARTESIAN_POINT('Ctrl Pts',(-0.192176438048885,0.0154224627179556,
-0.00559999999999953));
#36407=CARTESIAN_POINT('Ctrl Pts',(-0.191343963173299,0.0152131505605284,
-0.00591304953429593));
#36408=CARTESIAN_POINT('Ctrl Pts',(-0.190604005308188,0.0148933286596848,
-0.00633980824174457));
#36409=CARTESIAN_POINT('Ctrl Pts',(-0.189928056093887,0.0144823257548366,
-0.00677375538217563));
#36410=CARTESIAN_POINT('Ctrl Pts',(-0.189924240326155,0.0144800056225113,
-0.00677620503587909));
#36411=CARTESIAN_POINT('Ctrl Pts',(-0.189920426601425,0.0144776825774865,
-0.00677865492356244));
#36412=CARTESIAN_POINT('Ctrl Pts',(-0.189916614915206,0.0144753566233282,
-0.00678110502583209));
#36413=CARTESIAN_POINT('Ctrl Pts',(-0.189582813506844,0.0142716654669213,
-0.00699566822470287));
#36414=CARTESIAN_POINT('Ctrl Pts',(-0.189264648232927,0.014045660164331,
-0.00721187875958755));
#36415=CARTESIAN_POINT('Ctrl Pts',(-0.188963035346507,0.0137964688081976,
-0.00742469482413229));
#36416=CARTESIAN_POINT('Ctrl Pts',(-0.188657978335366,0.0135444319300434,
-0.00763994104037826));
#36417=CARTESIAN_POINT('Ctrl Pts',(-0.188369854070253,0.0132686788741525,
-0.00785171201844442));
#36418=CARTESIAN_POINT('Ctrl Pts',(-0.188099546793334,0.0129683186589328,
-0.00805477844807097));
#36419=CARTESIAN_POINT('Ctrl Pts',(-0.188093714462902,0.0129618378862222,
-0.00805915994504986));
#36420=CARTESIAN_POINT('Ctrl Pts',(-0.188087890440239,0.012955345674165,
-0.00806353734695464));
#36421=CARTESIAN_POINT('Ctrl Pts',(-0.188082074735716,0.0129488420160566,
-0.00806791060250755));
#36422=CARTESIAN_POINT('Ctrl Pts',(-0.187818353713641,0.0126539248040995,
-0.00826622181649803));
#36423=CARTESIAN_POINT('Ctrl Pts',(-0.187571750207195,0.0123354620106826,
-0.00845600236765789));
#36424=CARTESIAN_POINT('Ctrl Pts',(-0.187347312169252,0.0119951777506216,
-0.00863133901481845));
#36425=CARTESIAN_POINT('Ctrl Pts',(-0.187117924714299,0.0116473893761944,
-0.00881054227118578));
#36426=CARTESIAN_POINT('Ctrl Pts',(-0.186911700916772,0.0112768070043132,
-0.00897465664894075));
#36427=CARTESIAN_POINT('Ctrl Pts',(-0.186733851221639,0.0108854486190338,
-0.00911727516815564));
#36428=CARTESIAN_POINT('Ctrl Pts',(-0.186727815762721,0.0108721675872344,
-0.00912211503146282));
#36429=CARTESIAN_POINT('Ctrl Pts',(-0.186721813013436,0.0108588627757301,
-0.00912692993314436));
#36430=CARTESIAN_POINT('Ctrl Pts',(-0.186715843136615,0.0108455341927419,
-0.00913171966304142));
#36431=CARTESIAN_POINT('Ctrl Pts',(-0.18654589585667,0.0104661031772941,
-0.0092680711476793));
#36432=CARTESIAN_POINT('Ctrl Pts',(-0.18640252125758,0.0100674585344605,
-0.00938407744564779));
#36433=CARTESIAN_POINT('Ctrl Pts',(-0.186289553083222,0.00965454859173225,
-0.00947595892755243));
#36434=CARTESIAN_POINT('Ctrl Pts',(-0.186172616583594,0.00922713402441014,
-0.00957106800526971));
#36435=CARTESIAN_POINT('Ctrl Pts',(-0.18608819762884,0.0087843421088577,
-0.00964038068192425));
#36436=CARTESIAN_POINT('Ctrl Pts',(-0.186041757909902,0.00833112640840616,
-0.00967861021014855));
#36437=CARTESIAN_POINT('Origin',(-0.194168411395185,0.0075,-0.0165));
#36438=CARTESIAN_POINT('',(-0.192436879758486,-0.000483789065104605,-0.00550698406469574));
#36439=CARTESIAN_POINT('Ctrl Pts',(-0.186041751543844,0.00666887245842392,
-0.00967861584559627));
#36440=CARTESIAN_POINT('Ctrl Pts',(-0.186136921847663,0.00573830927961182,
-0.00960028215025333));
#36441=CARTESIAN_POINT('Ctrl Pts',(-0.186644248953973,0.00396647107157331,
-0.00918383236544583));
#36442=CARTESIAN_POINT('Ctrl Pts',(-0.188108094123016,0.00183866584854421,
-0.00802791806514813));
#36443=CARTESIAN_POINT('Ctrl Pts',(-0.190013954849379,0.000329756393205286,
-0.00666415905021552));
#36444=CARTESIAN_POINT('Ctrl Pts',(-0.191565762541839,-0.000294497235608542,
-0.0057981387366561));
#36445=CARTESIAN_POINT('Ctrl Pts',(-0.192436909186995,-0.000483437444660073,
-0.00550752136853039));
#36446=CARTESIAN_POINT('',(-0.192760058267355,-0.000547543173123365,-0.00559773047754231));
#36447=CARTESIAN_POINT('Ctrl Pts',(-0.192436908306343,-0.000483685301569694,
-0.00550688979015399));
#36448=CARTESIAN_POINT('Ctrl Pts',(-0.192468053494424,-0.000490526619111128,
-0.00550953117142323));
#36449=CARTESIAN_POINT('Ctrl Pts',(-0.192500024893769,-0.000497440829550889,
-0.00551318415929702));
#36450=CARTESIAN_POINT('Ctrl Pts',(-0.192526030662271,-0.000502770803046763,
-0.00551666078240278));
#36451=CARTESIAN_POINT('Ctrl Pts',(-0.192552036430774,-0.000508100776542638,
-0.00552013740550853));
#36452=CARTESIAN_POINT('Ctrl Pts',(-0.192572075699273,-0.000512091086316927,
-0.00552287359103419));
#36453=CARTESIAN_POINT('Ctrl Pts',(-0.192606479483278,-0.000519208585877513,
-0.00553001925783382));
#36454=CARTESIAN_POINT('Ctrl Pts',(-0.192640883267283,-0.000526326085438099,
-0.00553716492463345));
#36455=CARTESIAN_POINT('Ctrl Pts',(-0.192689655216252,-0.0005355448116613,
-0.005549838644018));
#36456=CARTESIAN_POINT('Ctrl Pts',(-0.192718970945351,-0.000540610831352234,
-0.00556188714561741));
#36457=CARTESIAN_POINT('Ctrl Pts',(-0.192748285725897,-0.000545676687124638,
-0.0055739352573698));
#36458=CARTESIAN_POINT('Ctrl Pts',(-0.192758140601795,-0.000547978991753478,
-0.00558509522749682));
#36459=CARTESIAN_POINT('Ctrl Pts',(-0.192759751083746,-0.000548263549761792,
-0.00559775493557849));
#36460=CARTESIAN_POINT('Ctrl Pts',(-0.192759756876124,-0.000546680419632493,
-0.00559779101339214));
#36461=CARTESIAN_POINT('Ctrl Pts',(-0.191825165385716,-0.000383070526138125,
-0.00584619740310806));
#36462=CARTESIAN_POINT('Ctrl Pts',(-0.190150361296732,0.000235470075430173,
-0.00671609199811723));
#36463=CARTESIAN_POINT('Ctrl Pts',(-0.1881181529752,0.00180741978905575,
-0.00813941771993866));
#36464=CARTESIAN_POINT('Ctrl Pts',(-0.186582686445248,0.00406221483284674,
-0.00933836675647093));
#36465=CARTESIAN_POINT('Ctrl Pts',(-0.18608965503935,0.00593890428125912,
-0.00973990799217201));
#36466=CARTESIAN_POINT('Ctrl Pts',(-0.186019885804631,0.00692129106638248,
-0.00979684105632399));
#36467=CARTESIAN_POINT('Origin',(-0.194168411395185,0.0075,-0.0165));
#36468=CARTESIAN_POINT('',(-0.192176435205664,0.015422462003074,0.00560000000000063));
#36469=CARTESIAN_POINT('',(-0.192751465176479,0.0155452244681588,0.0056));
#36470=CARTESIAN_POINT('Origin',(-0.194168411395185,0.0075,0.0056));
#36471=CARTESIAN_POINT('Ctrl Pts',(-0.192751465176479,0.0155452244681588,
0.00560000000000577));
#36472=CARTESIAN_POINT('Ctrl Pts',(-0.191813525435382,0.0153800320394353,
0.0058506525472026));
#36473=CARTESIAN_POINT('Ctrl Pts',(-0.190145096657311,0.0147607301998181,
0.00672019516858599));
#36474=CARTESIAN_POINT('Ctrl Pts',(-0.188114479081028,0.0131886463237939,
0.00814201325558834));
#36475=CARTESIAN_POINT('Ctrl Pts',(-0.18658186007787,0.0109350717238122,
0.00933911242506903));
#36476=CARTESIAN_POINT('Ctrl Pts',(-0.186089586988853,0.00906013840632952,
0.00973996390275296));
#36477=CARTESIAN_POINT('Ctrl Pts',(-0.186019885767525,0.00807870841113033,
0.00979684126041441));
#36478=CARTESIAN_POINT('Ctrl Pts',(-0.186041751490874,0.00833112702364014,
0.00967861612727941));
#36479=CARTESIAN_POINT('Ctrl Pts',(-0.186134520211485,0.00923820839715129,
0.00960225940762806));
#36480=CARTESIAN_POINT('Ctrl Pts',(-0.1866209358955,0.0109672061146848,
0.00920310409653587));
#36481=CARTESIAN_POINT('Ctrl Pts',(-0.188024941690495,0.0130628185286647,
0.00809245011053833));
#36482=CARTESIAN_POINT('Ctrl Pts',(-0.189858840973276,0.0145715969653575,
0.00676934907065498));
#36483=CARTESIAN_POINT('Ctrl Pts',(-0.191348256704472,0.0152142297825336,
0.0059114330126843));
#36484=CARTESIAN_POINT('Ctrl Pts',(-0.192176435205665,0.015422462003074,
0.00560000000000055));
#36485=CARTESIAN_POINT('Origin',(-0.194168411395185,0.0075,-0.0165));
#36486=CARTESIAN_POINT('',(-0.192751465176499,-0.000545224468162299,0.0056));
#36487=CARTESIAN_POINT('Ctrl Pts',(-0.186019885794595,0.00692129120770981,
0.00979684123832483));
#36488=CARTESIAN_POINT('Ctrl Pts',(-0.186089603411304,0.00593963099051061,
0.00973995050071142));
#36489=CARTESIAN_POINT('Ctrl Pts',(-0.186581991646468,0.00406427983701678,
0.00933894129944149));
#36490=CARTESIAN_POINT('Ctrl Pts',(-0.188115599150068,0.0018103891583067,
0.00814136010924737));
#36491=CARTESIAN_POINT('Ctrl Pts',(-0.190145486706124,0.000238420026637399,
0.0067193088022048));
#36492=CARTESIAN_POINT('Ctrl Pts',(-0.191818089971992,-0.000380835957701934,
0.00584943273245187));
#36493=CARTESIAN_POINT('Ctrl Pts',(-0.192751465176499,-0.000545224468162312,
0.00559999999999996));
#36494=CARTESIAN_POINT('',(-0.192176435205669,-0.000422462003075014,0.00559999999999858));
#36495=CARTESIAN_POINT('Origin',(-0.194168411395185,0.0075,0.0056));
#36496=CARTESIAN_POINT('Ctrl Pts',(-0.192176435205669,-0.00042246200307506,
0.0055999999999985));
#36497=CARTESIAN_POINT('Ctrl Pts',(-0.191343960306167,-0.000213149521988604,
0.00591304865504301));
#36498=CARTESIAN_POINT('Ctrl Pts',(-0.190604002024927,0.000106672964546729,
0.00633980594928245));
#36499=CARTESIAN_POINT('Ctrl Pts',(-0.1899280529401,0.000517676161234743,
0.00677375261658828));
#36500=CARTESIAN_POINT('Ctrl Pts',(-0.18992423716161,0.000519996302192667,
0.00677620227499601));
#36501=CARTESIAN_POINT('Ctrl Pts',(-0.189920423426153,0.000522319355858489,
0.00677865216741516));
#36502=CARTESIAN_POINT('Ctrl Pts',(-0.189916611729236,0.000524645318665928,
0.00678110227445219));
#36503=CARTESIAN_POINT('Ctrl Pts',(-0.189582810400498,0.000728336612260569,
0.0069956652374637));
#36504=CARTESIAN_POINT('Ctrl Pts',(-0.189264645340128,0.000954341979308797,
0.00721187576892209));
#36505=CARTESIAN_POINT('Ctrl Pts',(-0.188963032722283,0.00120353333031646,
0.00742469200704865));
#36506=CARTESIAN_POINT('Ctrl Pts',(-0.188657975972295,0.00145557021195114,
0.00763993840625852));
#36507=CARTESIAN_POINT('Ctrl Pts',(-0.188369852025587,0.00173132320188797,
0.00785170974812982));
#36508=CARTESIAN_POINT('Ctrl Pts',(-0.188099545041626,0.00203168328517292,
0.00805477666142801));
#36509=CARTESIAN_POINT('Ctrl Pts',(-0.188093712707518,0.00203816406614484,
0.00805915817635282));
#36510=CARTESIAN_POINT('Ctrl Pts',(-0.188087888681199,0.00204465628647009,
0.00806353559624864));
#36511=CARTESIAN_POINT('Ctrl Pts',(-0.188082072973036,0.00205115995285323,
0.00806790886983681));
#36512=CARTESIAN_POINT('Ctrl Pts',(-0.187818352247886,0.00234607702340897,
0.00826622055425919));
#36513=CARTESIAN_POINT('Ctrl Pts',(-0.187571749013941,0.00266453960709992,
0.00845600169657692));
#36514=CARTESIAN_POINT('Ctrl Pts',(-0.187347311208284,0.00300482365954855,
0.00863133886161257));
#36515=CARTESIAN_POINT('Ctrl Pts',(-0.18711792398207,0.00335261183493064,
0.00881054265404897));
#36516=CARTESIAN_POINT('Ctrl Pts',(-0.186911700373378,0.0037231940118813,
0.00897465749008297));
#36517=CARTESIAN_POINT('Ctrl Pts',(-0.186733850811817,0.00411455227599193,
0.0091172761862189));
#36518=CARTESIAN_POINT('Ctrl Pts',(-0.186727815350132,0.0041278333197421,
0.00912211606138361));
#36519=CARTESIAN_POINT('Ctrl Pts',(-0.186721812598099,0.00414113814333308,
0.00912693097454919));
#36520=CARTESIAN_POINT('Ctrl Pts',(-0.186715842718546,0.00415446673854782,
0.00913172071554889));
#36521=CARTESIAN_POINT('Ctrl Pts',(-0.186545895573612,0.00453389762703021,
0.00926807234554705));
#36522=CARTESIAN_POINT('Ctrl Pts',(-0.186402521055717,0.00493254220704179,
0.0093840785323548));
#36523=CARTESIAN_POINT('Ctrl Pts',(-0.186289552931936,0.00534545209131564,
0.00947595982899907));
#36524=CARTESIAN_POINT('Ctrl Pts',(-0.186172616479694,0.00577286661628877,
0.00957106871898892));
#36525=CARTESIAN_POINT('Ctrl Pts',(-0.186088197541083,0.00621565849694276,
0.00964038112619589));
#36526=CARTESIAN_POINT('Ctrl Pts',(-0.186041757857161,0.0066688741095359,
0.00967861049200898));
#36527=CARTESIAN_POINT('Ctrl Pts',(-0.214908904387703,-0.000412819837817,
0.00549924362755427));
#36528=CARTESIAN_POINT('Ctrl Pts',(-0.214908556120093,-0.000352592236114761,
0.00549921336268601));
#36529=CARTESIAN_POINT('Ctrl Pts',(-0.214907538880938,-0.000324420911413182,
0.0055524795130164));
#36530=CARTESIAN_POINT('Ctrl Pts',(-0.215674937410034,-0.000408049554921536,
0.00551196603108662));
#36531=CARTESIAN_POINT('Ctrl Pts',(-0.215679462273084,-0.000347576983031315,
0.00551248972391986));
#36532=CARTESIAN_POINT('Ctrl Pts',(-0.215687503951218,-0.000319594653488507,
0.00556554866444318));
#36533=CARTESIAN_POINT('Ctrl Pts',(-0.217146688138541,-0.000581852351431893,
0.00522168675990709));
#36534=CARTESIAN_POINT('Ctrl Pts',(-0.217202909083221,-0.000525975536923966,
0.00520094287146893));
#36535=CARTESIAN_POINT('Ctrl Pts',(-0.217185883978921,-0.00049120191472606,
0.00527389759715679));
#36536=CARTESIAN_POINT('Ctrl Pts',(-0.2186746596929,-0.00100105768310807,
0.00420084069381812));
#36537=CARTESIAN_POINT('Ctrl Pts',(-0.21871285197137,-0.000931067325908604,
0.00416353700088283));
#36538=CARTESIAN_POINT('Ctrl Pts',(-0.218741209646565,-0.000905486334259725,
0.00424664847380188));
#36539=CARTESIAN_POINT('Ctrl Pts',(-0.219590982556484,-0.00126551964588667,
0.00309225172418097));
#36540=CARTESIAN_POINT('Ctrl Pts',(-0.219605834846954,-0.00117755767893153,
0.00306843118737349));
#36541=CARTESIAN_POINT('Ctrl Pts',(-0.219673746789243,-0.00116683843606389,
0.00313100836683839));
#36542=CARTESIAN_POINT('Ctrl Pts',(-0.220279879401475,-0.00140079103123703,
0.00181632836118542));
#36543=CARTESIAN_POINT('Ctrl Pts',(-0.22028722062927,-0.00130284471617747,
0.00179819091483098));
#36544=CARTESIAN_POINT('Ctrl Pts',(-0.220374608257138,-0.00130053614138798,
0.00184630444409877));
#36545=CARTESIAN_POINT('Ctrl Pts',(-0.220646769346283,-0.00147114957019175,
2.23648118814017E-6));
#36546=CARTESIAN_POINT('Ctrl Pts',(-0.220641282870505,-0.00137222086809375,
2.22945995551979E-6));
#36547=CARTESIAN_POINT('Ctrl Pts',(-0.220747708299123,-0.00137133940053372,
2.26820978703318E-6));
#36548=CARTESIAN_POINT('Ctrl Pts',(-0.220279811878892,-0.00140077718961124,
-0.00181691872560231));
#36549=CARTESIAN_POINT('Ctrl Pts',(-0.220287131950059,-0.00130282536243108,
-0.00179879800073754));
#36550=CARTESIAN_POINT('Ctrl Pts',(-0.220374539523279,-0.00130052234399854,
-0.00184690438226544));
#36551=CARTESIAN_POINT('Ctrl Pts',(-0.219591001090582,-0.00126552646557676,
-0.00309233014391036));
#36552=CARTESIAN_POINT('Ctrl Pts',(-0.219605890119876,-0.00117757433237593,
-0.00306847780184537));
#36553=CARTESIAN_POINT('Ctrl Pts',(-0.219673765728205,-0.00116684522595654,
-0.00313108606374142));
#36554=CARTESIAN_POINT('Ctrl Pts',(-0.218672731854415,-0.00100053740872269,
-0.00420257854676322));
#36555=CARTESIAN_POINT('Ctrl Pts',(-0.218710929056937,-0.000930569929864368,
-0.00416525928590887));
#36556=CARTESIAN_POINT('Ctrl Pts',(-0.218739247444545,-0.000904972171632613,
-0.00424839789736909));
#36557=CARTESIAN_POINT('Ctrl Pts',(-0.217149041162339,-0.000582287155663073,
-0.00522050661308843));
#36558=CARTESIAN_POINT('Ctrl Pts',(-0.217205169333144,-0.000526365237140583,
-0.00519985099062644));
#36559=CARTESIAN_POINT('Ctrl Pts',(-0.217188279312873,-0.000491631333474201,
-0.00527271044190245));
#36560=CARTESIAN_POINT('Ctrl Pts',(-0.215673971815205,-0.000408030032539972,
-0.00551201428777479));
#36561=CARTESIAN_POINT('Ctrl Pts',(-0.215678500833659,-0.000347560008737919,
-0.00551253254967125));
#36562=CARTESIAN_POINT('Ctrl Pts',(-0.215686520820721,-0.000319575241216833,
-0.0055655974225352));
#36563=CARTESIAN_POINT('Ctrl Pts',(-0.214909020286864,-0.000412822472739081,
-0.00549924062753781));
#36564=CARTESIAN_POINT('Ctrl Pts',(-0.214908671883726,-0.000352594303262603,
-0.00549921069462562));
#36565=CARTESIAN_POINT('Ctrl Pts',(-0.214907656887067,-0.000324423258678074,
-0.00555247701276162));
#36566=CARTESIAN_POINT('Origin',(-0.214999964648729,-0.000412689929438997,
0.00559999998627548));
#36567=CARTESIAN_POINT('Origin',(-0.214999964645672,-0.000412691090472084,
-0.0055999999862731));
#36568=CARTESIAN_POINT('Origin',(-0.195909555102848,-0.000340904441697687,
-0.00560539994565062));
#36569=CARTESIAN_POINT('Ctrl Pts',(-0.19218256102446,-0.000325378183934642,
-0.00549961012006739));
#36570=CARTESIAN_POINT('Ctrl Pts',(-0.192184843256322,-0.000306151782977641,
-0.00549964929320649));
#36571=CARTESIAN_POINT('Ctrl Pts',(-0.192188722368746,-0.000279214203787051,
-0.00550497831707243));
#36572=CARTESIAN_POINT('Ctrl Pts',(-0.192196136252542,-0.000255497248569862,
-0.0055282091349877));
#36573=CARTESIAN_POINT('Ctrl Pts',(-0.192197708531578,-0.000250467540456901,
-0.00553313574686807));
#36574=CARTESIAN_POINT('Ctrl Pts',(-0.192199363429286,-0.000245783086052327,
-0.00553879864269582));
#36575=CARTESIAN_POINT('Ctrl Pts',(-0.192200962785523,-0.000241733447191861,
-0.00554503445704357));
#36576=CARTESIAN_POINT('Origin',(-0.195910717308576,-0.000340907999567637,
0.00560539870829468));
#36577=CARTESIAN_POINT('Origin',(-0.192200813655166,-0.000326595300734187,
0.00560462943321518));
#36578=CARTESIAN_POINT('Ctrl Pts',(-0.193540678138372,-0.000649552417819318,
-0.00523737591822536));
#36579=CARTESIAN_POINT('Ctrl Pts',(-0.193441105496944,-0.000646194280369797,
-0.00486953098091726));
#36580=CARTESIAN_POINT('Ctrl Pts',(-0.193548680125377,-0.00046236752507203,
-0.00518741811674645));
#36581=CARTESIAN_POINT('Ctrl Pts',(-0.19221784368241,-0.000532942846040005,
-0.00544735829321972));
#36582=CARTESIAN_POINT('Ctrl Pts',(-0.192317692121799,-0.000539647098916115,
-0.00504480941502384));
#36583=CARTESIAN_POINT('Ctrl Pts',(-0.192242056430693,-0.000348629122757424,
-0.00539460937276613));
#36584=CARTESIAN_POINT('Ctrl Pts',(-0.190280755377544,0.000121068599940136,
-0.00647511727459894));
#36585=CARTESIAN_POINT('Ctrl Pts',(-0.190539954106928,-4.11033634603214E-5,
-0.00602341757418173));
#36586=CARTESIAN_POINT('Ctrl Pts',(-0.190329131797122,0.000290675906173524,
-0.00641082489689668));
#36587=CARTESIAN_POINT('Ctrl Pts',(-0.188108313415062,0.00183522217201885,
-0.00802874354108597));
#36588=CARTESIAN_POINT('Ctrl Pts',(-0.188185831714158,0.00174861716519636,
-0.00778938974969843));
#36589=CARTESIAN_POINT('Ctrl Pts',(-0.18818459172986,0.00196541394824739,
-0.00794671383597527));
#36590=CARTESIAN_POINT('Ctrl Pts',(-0.186442115636933,0.00425799506259359,
-0.00934492203853191));
#36591=CARTESIAN_POINT('Ctrl Pts',(-0.186505177095779,0.00413522900627745,
-0.00917361754652802));
#36592=CARTESIAN_POINT('Ctrl Pts',(-0.186539821858752,0.00433279168103422,
-0.0092481696460331));
#36593=CARTESIAN_POINT('Ctrl Pts',(-0.185949933848258,0.00649864288516591,
-0.00975604832858269));
#36594=CARTESIAN_POINT('Ctrl Pts',(-0.185938996922361,0.00650356966711613,
-0.0096606155981595));
#36595=CARTESIAN_POINT('Ctrl Pts',(-0.186054161082477,0.00652165633138307,
-0.00965452990509759));
#36596=CARTESIAN_POINT('Ctrl Pts',(-0.186008609242487,0.00779556652501847,
-0.00970683855217618));
#36597=CARTESIAN_POINT('Ctrl Pts',(-0.186012519244314,0.00779930724970625,
-0.00959773856785611));
#36598=CARTESIAN_POINT('Ctrl Pts',(-0.186112045272954,0.00778881516418459,
-0.00960591497712815));
#36599=CARTESIAN_POINT('Ctrl Pts',(-0.192436962091582,-0.000483455930974332,
-0.0055068000272665));
#36600=CARTESIAN_POINT('Ctrl Pts',(-0.192417454388871,-0.000479179295420767,
-0.0055051608623328));
#36601=CARTESIAN_POINT('Ctrl Pts',(-0.192398518083474,-0.000474037136212224,
-0.00550349916183664));
#36602=CARTESIAN_POINT('Ctrl Pts',(-0.192358508328238,-0.000461146975878049,
-0.00550076542168802));
#36603=CARTESIAN_POINT('Ctrl Pts',(-0.192338355794539,-0.000453479114128204,
-0.00549985112232206));
#36604=CARTESIAN_POINT('Ctrl Pts',(-0.192317960073385,-0.000445032779133932,
-0.00549999396547274));
#36605=CARTESIAN_POINT('Ctrl Pts',(-0.186146182193085,0.00666198610159568,
-0.00957677543676099));
#36606=CARTESIAN_POINT('Ctrl Pts',(-0.186108276179088,0.00665976117994766,
-0.00957572084247029));
#36607=CARTESIAN_POINT('Ctrl Pts',(-0.186076614916844,0.00665569960762129,
-0.00959771890028863));
#36608=CARTESIAN_POINT('Ctrl Pts',(-0.186061509823992,0.00665290370623444,
-0.00961964518377239));
#36609=CARTESIAN_POINT('Ctrl Pts',(-0.186052741584085,0.00665128073480653,
-0.0096323730044966));
#36610=CARTESIAN_POINT('Ctrl Pts',(-0.186048069026781,0.00664991367016798,
-0.00964523184213603));
#36611=CARTESIAN_POINT('Ctrl Pts',(-0.186045770369396,0.00664869276501877,
-0.00965738685531515));
#36612=CARTESIAN_POINT('Ctrl Pts',(-0.186005598851858,0.00774016753564896,
0.00970831679928731));
#36613=CARTESIAN_POINT('Ctrl Pts',(-0.186009670836186,0.00774304435209903,
0.00960230395719931));
#36614=CARTESIAN_POINT('Ctrl Pts',(-0.186108014816518,0.00773474456881634,
0.00960842057355287));
#36615=CARTESIAN_POINT('Ctrl Pts',(-0.185960333964487,0.00648227707345362,
0.00974617139101431));
#36616=CARTESIAN_POINT('Ctrl Pts',(-0.185952179587332,0.00648769121866751,
0.00965136579735061));
#36617=CARTESIAN_POINT('Ctrl Pts',(-0.186063352151639,0.00650542775407373,
0.00964582108962002));
#36618=CARTESIAN_POINT('Ctrl Pts',(-0.186428987223196,0.00432575778421166,
0.00935548962635469));
#36619=CARTESIAN_POINT('Ctrl Pts',(-0.186483364142072,0.00421970259174358,
0.00919520509208301));
#36620=CARTESIAN_POINT('Ctrl Pts',(-0.186525917729122,0.00439824791225163,
0.00925957076353963));
#36621=CARTESIAN_POINT('Ctrl Pts',(-0.188010036483664,0.00195171154641976,
0.00810342874470907));
#36622=CARTESIAN_POINT('Ctrl Pts',(-0.188076570799909,0.00187804731004616,
0.00788256538710582));
#36623=CARTESIAN_POINT('Ctrl Pts',(-0.188086956158076,0.00207818061049679,
0.00802123465030675));
#36624=CARTESIAN_POINT('Ctrl Pts',(-0.190096769641379,0.000230160943820068,
0.00659753516612828));
#36625=CARTESIAN_POINT('Ctrl Pts',(-0.190313514403938,8.77705727554797E-5,
0.00619100739750346));
#36626=CARTESIAN_POINT('Ctrl Pts',(-0.190147199090351,0.000396274459653245,
0.0065322762088843));
#36627=CARTESIAN_POINT('Ctrl Pts',(-0.191946116765636,-0.000455424949601966,
0.00557143365312373));
#36628=CARTESIAN_POINT('Ctrl Pts',(-0.192036696545771,-0.000459166706784753,
0.00520128186042438));
#36629=CARTESIAN_POINT('Ctrl Pts',(-0.191973611942258,-0.000273697961367191,
0.00551749368314696));
#36630=CARTESIAN_POINT('Ctrl Pts',(-0.193225816082199,-0.000619663171657372,
0.00528509249354492));
#36631=CARTESIAN_POINT('Ctrl Pts',(-0.193123350533271,-0.000605932760873667,
0.00495167335479587));
#36632=CARTESIAN_POINT('Ctrl Pts',(-0.193237683484677,-0.000433914425303821,
0.00523470332505228));
#36633=CARTESIAN_POINT('Origin',(-0.192200819635387,-0.000325480563679127,
0.00560000000000713));
#36634=CARTESIAN_POINT('Ctrl Pts',(-0.186045766963236,0.00664869409545193,
0.00965738640065765));
#36635=CARTESIAN_POINT('Ctrl Pts',(-0.186050130369219,0.00665101100562805,
0.00963431766854684));
#36636=CARTESIAN_POINT('Ctrl Pts',(-0.186063617073953,0.00665414856520909,
0.00960600839114813));
#36637=CARTESIAN_POINT('Ctrl Pts',(-0.186096378519772,0.00665778543826778,
0.00958849515329468));
#36638=CARTESIAN_POINT('Ctrl Pts',(-0.186110518764896,0.00665935515765138,
0.00958093622327859));
#36639=CARTESIAN_POINT('Ctrl Pts',(-0.186128098007252,0.00666092475184653,
0.00957627595969465));
#36640=CARTESIAN_POINT('Ctrl Pts',(-0.186146182039353,0.00666198624828256,
0.00957677958184586));
#36641=CARTESIAN_POINT('Origin',(-0.187920131339758,0.00750009680678902,
-0.000575225526917647));
#36642=CARTESIAN_POINT('Ctrl Pts',(-0.186045768135075,0.00835131759320733,
-0.00965738542725037));
#36643=CARTESIAN_POINT('Ctrl Pts',(-0.186050128411678,0.00834900218136687,
-0.00963433280458853));
#36644=CARTESIAN_POINT('Ctrl Pts',(-0.186063611063362,0.00834585919375938,
-0.00960601547883551));
#36645=CARTESIAN_POINT('Ctrl Pts',(-0.186096369868285,0.0083422188034536,
-0.00958849943088495));
#36646=CARTESIAN_POINT('Ctrl Pts',(-0.186110513510244,0.00834064706183503,
-0.00958093686224691));
#36647=CARTESIAN_POINT('Ctrl Pts',(-0.186128096876543,0.00833907596658786,
-0.0095762756193603));
#36648=CARTESIAN_POINT('Ctrl Pts',(-0.186146182113142,0.00833801422983676,
-0.00957677929432219));
#36649=CARTESIAN_POINT('Origin',(-0.187954144158173,0.0074999097326559,
0.000581964911843834));
#36650=CARTESIAN_POINT('Ctrl Pts',(-0.186146182120156,0.00833801356110422,
0.00957677710043646));
#36651=CARTESIAN_POINT('Ctrl Pts',(-0.186108254991117,0.00834023913104114,
0.00957572208550327));
#36652=CARTESIAN_POINT('Ctrl Pts',(-0.186076596831025,0.00834429292618449,
0.00959772857351143));
#36653=CARTESIAN_POINT('Ctrl Pts',(-0.186061488244737,0.00834708538103843,
0.00961967482382124));
#36654=CARTESIAN_POINT('Ctrl Pts',(-0.186052741256565,0.00834870204914431,
0.00963238041971281));
#36655=CARTESIAN_POINT('Ctrl Pts',(-0.186048067263802,0.00835006607147121,
0.00964522644092186));
#36656=CARTESIAN_POINT('Ctrl Pts',(-0.186045767212607,0.00835128750327599,
0.00965738803265854));
#36657=CARTESIAN_POINT('Ctrl Pts',(-0.186005598759832,0.00725983232716103,
-0.00970831661057972));
#36658=CARTESIAN_POINT('Ctrl Pts',(-0.186009670651558,0.00725695543053303,
-0.00960230389666019));
#36659=CARTESIAN_POINT('Ctrl Pts',(-0.186108014721025,0.00726525532639936,
-0.00960842038224571));
#36660=CARTESIAN_POINT('Ctrl Pts',(-0.185960334112893,0.00851772391887955,
-0.00974617155991487));
#36661=CARTESIAN_POINT('Ctrl Pts',(-0.185952179909706,0.00851230994790259,
-0.00965136574061983));
#36662=CARTESIAN_POINT('Ctrl Pts',(-0.186063352297074,0.00849457313387128,
-0.00964582125981882));
#36663=CARTESIAN_POINT('Ctrl Pts',(-0.186428987230586,0.0106742426078354,
-0.00935548690241927));
#36664=CARTESIAN_POINT('Ctrl Pts',(-0.186483363531177,0.0107802970046063,
-0.00919520299654669));
#36665=CARTESIAN_POINT('Ctrl Pts',(-0.186525917701738,0.0106017524957044,
-0.00925956807298176));
#36666=CARTESIAN_POINT('Ctrl Pts',(-0.188010038139295,0.0130482906965545,
-0.00810343096067351));
#36667=CARTESIAN_POINT('Ctrl Pts',(-0.188076573310405,0.0131219557179719,
-0.00788256757658765));
#36668=CARTESIAN_POINT('Ctrl Pts',(-0.188086957836586,0.0129218218041267,
-0.00802123671042419));
#36669=CARTESIAN_POINT('Ctrl Pts',(-0.190096773684561,0.014769841299388,
-0.00659753906857564));
#36670=CARTESIAN_POINT('Ctrl Pts',(-0.190313521732662,0.0149122337257658,
-0.00619100814431022));
#36671=CARTESIAN_POINT('Ctrl Pts',(-0.190147203120692,0.0146037275463174,
-0.00653228029147483));
#36672=CARTESIAN_POINT('Ctrl Pts',(-0.191946119174527,0.0154554254581438,
-0.00557143325871853));
#36673=CARTESIAN_POINT('Ctrl Pts',(-0.192036697189508,0.0154591661112836,
-0.0052012805696902));
#36674=CARTESIAN_POINT('Ctrl Pts',(-0.191973614322155,0.0152736983544835,
-0.00551749349096378));
#36675=CARTESIAN_POINT('Ctrl Pts',(-0.193225819175554,0.0156196636689472,
-0.00528509177693916));
#36676=CARTESIAN_POINT('Ctrl Pts',(-0.193123353574421,0.0156059338233821,
-0.0049516714716164));
#36677=CARTESIAN_POINT('Ctrl Pts',(-0.193237686540076,0.0154339148303609,
-0.00523470274052404));
#36678=CARTESIAN_POINT('Origin',(-0.192200822443804,0.0153254812698099,
-0.00560000000000634));
#36679=CARTESIAN_POINT('Ctrl Pts',(-0.193214260006029,0.0156168327619888,
0.00529060396926718));
#36680=CARTESIAN_POINT('Ctrl Pts',(-0.193105326746743,0.0156061976053113,
0.00495284829763268));
#36681=CARTESIAN_POINT('Ctrl Pts',(-0.19322590280958,0.0154311830256504,
0.00523902729326042));
#36682=CARTESIAN_POINT('Ctrl Pts',(-0.191955055227124,0.0154575099667713,
0.00556923862400056));
#36683=CARTESIAN_POINT('Ctrl Pts',(-0.192046773552436,0.0154646012482818,
0.00519213961909146));
#36684=CARTESIAN_POINT('Ctrl Pts',(-0.191982782338575,0.0152758375961863,
0.00551388949624999));
#36685=CARTESIAN_POINT('Ctrl Pts',(-0.190092180578751,0.014769053477849,
0.00660075597892395));
#36686=CARTESIAN_POINT('Ctrl Pts',(-0.190314395130687,0.0149176874591946,
0.00618689814909584));
#36687=CARTESIAN_POINT('Ctrl Pts',(-0.190143807260092,0.0146038314661997,
0.00653331286575727));
#36688=CARTESIAN_POINT('Ctrl Pts',(-0.18800611600784,0.0130431899705215,
0.00810777841374931));
#36689=CARTESIAN_POINT('Ctrl Pts',(-0.188072355662852,0.013119110276285,
0.00788470947760386));
#36690=CARTESIAN_POINT('Ctrl Pts',(-0.188083496099574,0.0129174748375354,
0.00802401143707513));
#36691=CARTESIAN_POINT('Ctrl Pts',(-0.186423687793365,0.0106657581153738,
0.00936054389127776));
#36692=CARTESIAN_POINT('Ctrl Pts',(-0.186478607626537,0.0107749341497348,
0.00919840721838609));
#36693=CARTESIAN_POINT('Ctrl Pts',(-0.186521060649371,0.0105944580941384,
0.00926327090558671));
#36694=CARTESIAN_POINT('Ctrl Pts',(-0.185956374325204,0.00849572718688238,
0.00975032638663647));
#36695=CARTESIAN_POINT('Ctrl Pts',(-0.185946971953686,0.00849053224154058,
0.00965520189867485));
#36696=CARTESIAN_POINT('Ctrl Pts',(-0.186059252699007,0.00847305358346526,
0.00964917339214119));
#36697=CARTESIAN_POINT('Ctrl Pts',(-0.186007036580647,0.00723972881157616,
0.00970794245356266));
#36698=CARTESIAN_POINT('Ctrl Pts',(-0.186010557211458,0.00723652449630214,
0.00960090529757225));
#36699=CARTESIAN_POINT('Ctrl Pts',(-0.186109360775984,0.00724557446066228,
0.0096071910993323));
#36700=CARTESIAN_POINT('Origin',(-0.192200819635407,0.0153254805636842,
0.0056));
#36701=CARTESIAN_POINT('Origin',(-0.195909629570911,0.0153409047393749,
-0.0056053999692199));
#36702=CARTESIAN_POINT('Origin',(-0.192200816462806,0.0153265960442655,
-0.00560463083553559));
#36703=CARTESIAN_POINT('Origin',(-0.214999964645852,0.0154126910904719,
-0.00559999998627319));
#36704=CARTESIAN_POINT('Origin',(-0.195910759730015,0.0153409081694028,
0.00560539872657712));
#36705=CARTESIAN_POINT('Origin',(-0.192200813655147,0.0153265953091492,
0.00560462944582787));
#36706=CARTESIAN_POINT('Origin',(-0.214999964648748,0.0154126899294396,
0.00559999998627548));
#36707=CARTESIAN_POINT('Ctrl Pts',(-0.21490892586111,0.0154128208581019,
-0.0054992439839607));
#36708=CARTESIAN_POINT('Ctrl Pts',(-0.21490857773275,0.0153525928800433,
-0.00549921373553946));
#36709=CARTESIAN_POINT('Ctrl Pts',(-0.214907560745888,0.0153244216769054,
-0.00555248035802741));
#36710=CARTESIAN_POINT('Ctrl Pts',(-0.215674951408508,0.0154080524844426,
-0.00551196326634576));
#36711=CARTESIAN_POINT('Ctrl Pts',(-0.215679476448769,0.0153475795412595,
-0.00551248680902352));
#36712=CARTESIAN_POINT('Ctrl Pts',(-0.215687518203886,0.0153195973000356,
-0.00556554638259137));
#36713=CARTESIAN_POINT('Ctrl Pts',(-0.217146694343493,0.0155818524774486,
-0.00522168280336377));
#36714=CARTESIAN_POINT('Ctrl Pts',(-0.217202913591221,0.0155259749241154,
-0.00520093965385637));
#36715=CARTESIAN_POINT('Ctrl Pts',(-0.217185890291163,0.0154912018795859,
-0.00527389396523135));
#36716=CARTESIAN_POINT('Ctrl Pts',(-0.218674660178022,0.0160010546194908,
-0.00420084024173932));
#36717=CARTESIAN_POINT('Ctrl Pts',(-0.218712852213832,0.0159310643238046,
-0.00416353684961489));
#36718=CARTESIAN_POINT('Ctrl Pts',(-0.218741210132284,0.0159054833219791,
-0.00424664790585557));
#36719=CARTESIAN_POINT('Ctrl Pts',(-0.219590982727002,0.0162655190811837,
-0.00309225143892686));
#36720=CARTESIAN_POINT('Ctrl Pts',(-0.219605835201339,0.0161775572907052,
-0.00306843062806678));
#36721=CARTESIAN_POINT('Ctrl Pts',(-0.219673746959147,0.0161668379039925,
-0.00313100785533165));
#36722=CARTESIAN_POINT('Ctrl Pts',(-0.220279879435486,0.0164007913673191,
-0.00181632823374506));
#36723=CARTESIAN_POINT('Ctrl Pts',(-0.22028722076064,0.0163028450056265,
-0.00179819050090137));
#36724=CARTESIAN_POINT('Ctrl Pts',(-0.220374608289813,0.0163005364595407,
-0.00184630444517829));
#36725=CARTESIAN_POINT('Ctrl Pts',(-0.220646769339641,0.0164711495711873,
-2.23629763584961E-6));
#36726=CARTESIAN_POINT('Ctrl Pts',(-0.220641282865907,0.016372220872245,
-2.22983725660083E-6));
#36727=CARTESIAN_POINT('Ctrl Pts',(-0.220747708289112,0.0163713394014852,
-2.26793534779618E-6));
#36728=CARTESIAN_POINT('Ctrl Pts',(-0.220279811864962,0.0164007768505767,
0.00181691874798004));
#36729=CARTESIAN_POINT('Ctrl Pts',(-0.220287131833914,0.0163028250756232,
0.00179879831642603));
#36730=CARTESIAN_POINT('Ctrl Pts',(-0.220374539505672,0.0163005220232469,
0.00184690427045525));
#36731=CARTESIAN_POINT('Ctrl Pts',(-0.219591001034938,0.0162655270612487,
0.00309233026324212));
#36732=CARTESIAN_POINT('Ctrl Pts',(-0.219605889878344,0.016177574754681,
0.00306847819752524));
#36733=CARTESIAN_POINT('Ctrl Pts',(-0.219673765670875,0.0161668457892537,
0.00313108640475189));
#36734=CARTESIAN_POINT('Ctrl Pts',(-0.218672731422678,0.016000540491302,
0.0042025789662199));
#36735=CARTESIAN_POINT('Ctrl Pts',(-0.218710928868343,0.0159305729552991,
0.0041652594003139));
#36736=CARTESIAN_POINT('Ctrl Pts',(-0.21873924701127,0.0159049752045155,
0.00424839842626237));
#36737=CARTESIAN_POINT('Ctrl Pts',(-0.217149046760076,0.0155822902582286,
0.00522050271701136));
#36738=CARTESIAN_POINT('Ctrl Pts',(-0.217205175745837,0.0155263687734777,
0.00519984674122877));
#36739=CARTESIAN_POINT('Ctrl Pts',(-0.21718828501593,0.0154916345616469,
0.00527270616715176));
#36740=CARTESIAN_POINT('Ctrl Pts',(-0.21567398590997,0.0154080304197497,
0.00551201150898643));
#36741=CARTESIAN_POINT('Ctrl Pts',(-0.215678515075149,0.0153475607801394,
0.00551252965151365));
#36742=CARTESIAN_POINT('Ctrl Pts',(-0.215686535169183,0.0153195758716015,
0.00556559413069578));
#36743=CARTESIAN_POINT('Ctrl Pts',(-0.214909041723364,0.0154128211845327,
0.00549924098553293));
#36744=CARTESIAN_POINT('Ctrl Pts',(-0.214908693448483,0.0153525933808177,
0.00549921106697866));
#36745=CARTESIAN_POINT('Ctrl Pts',(-0.214907678712506,0.0153244222242064,
0.00555247689767116));
#36746=CARTESIAN_POINT('Ctrl Pts',(-0.2309214360969,0.0162188491192864,
-0.00255390765191895));
#36747=CARTESIAN_POINT('Ctrl Pts',(-0.230917643433025,0.016122876817595,
-0.00254933585070519));
#36748=CARTESIAN_POINT('Ctrl Pts',(-0.23084354609566,0.0161191167494639,
-0.00261050295657583));
#36749=CARTESIAN_POINT('Ctrl Pts',(-0.231731271674744,0.0161403427476591,
-0.00353010997290807));
#36750=CARTESIAN_POINT('Ctrl Pts',(-0.231695499917477,0.0160542517468595,
-0.00348698952548079));
#36751=CARTESIAN_POINT('Ctrl Pts',(-0.231653762816047,0.0160414018930904,
-0.00357577197956242));
#36752=CARTESIAN_POINT('Ctrl Pts',(-0.233318350359044,0.0156828169900615,
-0.00544322658274142));
#36753=CARTESIAN_POINT('Ctrl Pts',(-0.233239475942029,0.015640840163108,
-0.00534814877797674));
#36754=CARTESIAN_POINT('Ctrl Pts',(-0.233241585595557,0.0155889048507678,
-0.00546766123177619));
#36755=CARTESIAN_POINT('Ctrl Pts',(-0.235522804973632,0.0140286093773024,
-0.00810054835292838));
#36756=CARTESIAN_POINT('Ctrl Pts',(-0.235456558010287,0.0140244277754155,
-0.00802069209427084));
#36757=CARTESIAN_POINT('Ctrl Pts',(-0.235447062611451,0.0139534444838987,
-0.00809510346252179));
#36758=CARTESIAN_POINT('Ctrl Pts',(-0.237276829383983,0.0112829697892784,
-0.0102149068070439));
#36759=CARTESIAN_POINT('Ctrl Pts',(-0.237233935149465,0.0113000460915102,
-0.0101632006923216));
#36760=CARTESIAN_POINT('Ctrl Pts',(-0.237201895619677,0.0112392878602733,
-0.010185602465943));
#36761=CARTESIAN_POINT('Ctrl Pts',(-0.238023912985867,0.00751556963457164,
-0.0111154658415992));
#36762=CARTESIAN_POINT('Ctrl Pts',(-0.237996530980257,0.00751544365575127,
-0.0110824586755033));
#36763=CARTESIAN_POINT('Ctrl Pts',(-0.237949322608371,0.00751538718331989,
-0.0110759389184273));
#36764=CARTESIAN_POINT('Ctrl Pts',(-0.237280015258684,0.00371938391596711,
-0.0102187471647188));
#36765=CARTESIAN_POINT('Ctrl Pts',(-0.237237148916806,0.00370230591124238,
-0.0101670746726941));
#36766=CARTESIAN_POINT('Ctrl Pts',(-0.237205082965768,0.00376303943723787,
-0.0101893990031388));
#36767=CARTESIAN_POINT('Ctrl Pts',(-0.235529704617421,0.000981618018545073,
-0.00810886540945947));
#36768=CARTESIAN_POINT('Ctrl Pts',(-0.235463830484283,0.000985956441676499,
-0.0080294585725564));
#36769=CARTESIAN_POINT('Ctrl Pts',(-0.235453965445146,0.00105666489234918,
-0.00810332645705537));
#36770=CARTESIAN_POINT('Ctrl Pts',(-0.233330300192999,-0.000678550038604275,
-0.00545763130384987));
#36771=CARTESIAN_POINT('Ctrl Pts',(-0.233250985436449,-0.000636996429499461,
-0.00536202269932594));
#36772=CARTESIAN_POINT('Ctrl Pts',(-0.233253541020546,-0.000584686101854415,
-0.00548190240738322));
#36773=CARTESIAN_POINT('Ctrl Pts',(-0.231731717669817,-0.00114029951282499,
-0.00353064758997168));
#36774=CARTESIAN_POINT('Ctrl Pts',(-0.231695913807421,-0.0010542152324075,
-0.00348748844212362));
#36775=CARTESIAN_POINT('Ctrl Pts',(-0.231654209020796,-0.00104135909373062,
-0.00357630357546777));
#36776=CARTESIAN_POINT('Ctrl Pts',(-0.2309214360969,-0.00121884911929219,
-0.00255390765191891));
#36777=CARTESIAN_POINT('Ctrl Pts',(-0.230917643433025,-0.00112287681760122,
-0.00254933585070488));
#36778=CARTESIAN_POINT('Ctrl Pts',(-0.23084354609566,-0.00111911674946971,
-0.00261050295657523));
#36779=CARTESIAN_POINT('Ctrl Pts',(-0.2309214360969,0.0162188491192864,
-0.00255390765191895));
#36780=CARTESIAN_POINT('Ctrl Pts',(-0.230919775033979,0.0161747085289458,
-0.00255190535228738));
#36781=CARTESIAN_POINT('Ctrl Pts',(-0.230893153703761,0.0161330891388246,
-0.00257080002687729));
#36782=CARTESIAN_POINT('Ctrl Pts',(-0.230859886434142,0.0161221790363513,
-0.00259732739947869));
#36783=CARTESIAN_POINT('Ctrl Pts',(-0.23085451814243,0.0161204184887214,
-0.00260160808364952));
#36784=CARTESIAN_POINT('Ctrl Pts',(-0.230849026328935,0.0161193903409544,
-0.00260604101323845));
#36785=CARTESIAN_POINT('Ctrl Pts',(-0.230843551760371,0.0161191162061102,
-0.00261050970535095));
#36786=CARTESIAN_POINT('Ctrl Pts',(-0.230843551742607,-0.00111911620782001,
-0.0026105096841861));
#36787=CARTESIAN_POINT('Ctrl Pts',(-0.23087747757725,-0.00112081501570214,
-0.002582817285748));
#36788=CARTESIAN_POINT('Ctrl Pts',(-0.23091000473876,-0.00115445692580184,
-0.0025584489568953));
#36789=CARTESIAN_POINT('Ctrl Pts',(-0.230918875913022,-0.00119762015153162,
-0.00255440400298611));
#36790=CARTESIAN_POINT('Ctrl Pts',(-0.230920307572675,-0.00120458597668313,
-0.00255375121484989));
#36791=CARTESIAN_POINT('Ctrl Pts',(-0.230921168038885,-0.00121172579473758,
-0.00255358452601128));
#36792=CARTESIAN_POINT('Ctrl Pts',(-0.2309214360969,-0.00121884911929219,
-0.00255390765191891));
#36793=CARTESIAN_POINT('Origin',(-0.23397514962969,-0.000958411587553637,
-2.1312647177279E-10));
#36794=CARTESIAN_POINT('Ctrl Pts',(-0.2309214360969,-0.00121884929951176,
0.00255390765191896));
#36795=CARTESIAN_POINT('Ctrl Pts',(-0.230919775047316,-0.00117470864868834,
0.00255190536836447));
#36796=CARTESIAN_POINT('Ctrl Pts',(-0.230893153683133,-0.00113308926455962,
0.0025708001043909));
#36797=CARTESIAN_POINT('Ctrl Pts',(-0.230859886422908,-0.00112217919297818,
0.00259732750272073));
#36798=CARTESIAN_POINT('Ctrl Pts',(-0.230854518134609,-0.00112041865095552,
0.00260160818953043));
#36799=CARTESIAN_POINT('Ctrl Pts',(-0.230849026325164,-0.00111939050845762,
0.00260604112123923));
#36800=CARTESIAN_POINT('Ctrl Pts',(-0.230843551761021,-0.00111911637834476,
0.00261050981525893));
#36801=CARTESIAN_POINT('Origin',(-0.233975149629148,0.015958411588167,2.19838690515469E-10));
#36802=CARTESIAN_POINT('Ctrl Pts',(-0.230843551743257,0.0161191163800488,
0.00261050979409577));
#36803=CARTESIAN_POINT('Ctrl Pts',(-0.230877477562569,0.0161208151592145,
0.00258281737399711));
#36804=CARTESIAN_POINT('Ctrl Pts',(-0.230910004742525,0.016154457039061,
0.00255844899691895));
#36805=CARTESIAN_POINT('Ctrl Pts',(-0.230918875916907,0.0161976203127023,
0.00255440401393904));
#36806=CARTESIAN_POINT('Ctrl Pts',(-0.230920307576072,0.0162045861431113,
0.0025537512213432));
#36807=CARTESIAN_POINT('Ctrl Pts',(-0.230921168041133,0.0162117259677385,
0.00255358452872089));
#36808=CARTESIAN_POINT('Ctrl Pts',(-0.2309214360969,0.016218849299512,0.00255390765191894));
#36809=CARTESIAN_POINT('Ctrl Pts',(-0.2309214360969,-0.00121884929951176,
0.00255390765191896));
#36810=CARTESIAN_POINT('Ctrl Pts',(-0.230917643482494,-0.00112287692579763,
0.00254933591033698));
#36811=CARTESIAN_POINT('Ctrl Pts',(-0.230843546096085,-0.00111911692171259,
0.00261050306621451));
#36812=CARTESIAN_POINT('Ctrl Pts',(-0.231731271358665,-0.0011403440413955,
0.00353010959189706));
#36813=CARTESIAN_POINT('Ctrl Pts',(-0.231695500440064,-0.00105425268533019,
0.00348699015503689));
#36814=CARTESIAN_POINT('Ctrl Pts',(-0.231653762502425,-0.00104140314540818,
0.00357577200213956));
#36815=CARTESIAN_POINT('Ctrl Pts',(-0.233318351429915,-0.000682830411131618,
0.00544322787360406));
#36816=CARTESIAN_POINT('Ctrl Pts',(-0.233239475950391,-0.000640855225105034,
0.00534814878822644));
#36817=CARTESIAN_POINT('Ctrl Pts',(-0.233241586693064,-0.000588918662889074,
0.00546766133448137));
#36818=CARTESIAN_POINT('Ctrl Pts',(-0.235522785051244,0.000971430442923571,
0.00810052433783006));
#36819=CARTESIAN_POINT('Ctrl Pts',(-0.235456540369885,0.000975613862285589,
0.00802067082991012));
#36820=CARTESIAN_POINT('Ctrl Pts',(-0.235447042598565,0.00104659521317374,
0.00809507963380781));
#36821=CARTESIAN_POINT('Ctrl Pts',(-0.237276842725964,0.00371701980185319,
0.0102149228899044));
#36822=CARTESIAN_POINT('Ctrl Pts',(-0.237233947381609,0.00369994316081699,
0.0101632154373597));
#36823=CARTESIAN_POINT('Ctrl Pts',(-0.237201908997141,0.00376070251875742,
0.0101856188837833));
#36824=CARTESIAN_POINT('Ctrl Pts',(-0.238023907994334,0.00748443566710092,
0.0111154598246424));
#36825=CARTESIAN_POINT('Ctrl Pts',(-0.237996526448544,0.00748456159372698,
0.0110824532128226));
#36826=CARTESIAN_POINT('Ctrl Pts',(-0.237949317601923,0.00748461804540081,
0.0110759327314131));
#36827=CARTESIAN_POINT('Ctrl Pts',(-0.237280027202557,0.0112806277971099,
0.0102187615622546));
#36828=CARTESIAN_POINT('Ctrl Pts',(-0.237237159718854,0.0112977061424594,
0.0101670876938473));
#36829=CARTESIAN_POINT('Ctrl Pts',(-0.23720509494468,0.0112369714924193,
0.0101894137458077));
#36830=CARTESIAN_POINT('Ctrl Pts',(-0.235529684253431,0.0140183426910286,
0.00810884086203866));
#36831=CARTESIAN_POINT('Ctrl Pts',(-0.235463812480867,0.0140140023765735,
0.00802943687061338));
#36832=CARTESIAN_POINT('Ctrl Pts',(-0.235453944990362,0.0139432959143817,
0.00810330212192403));
#36833=CARTESIAN_POINT('Ctrl Pts',(-0.233330301704251,0.0156785630234985,
0.00545763312556219));
#36834=CARTESIAN_POINT('Ctrl Pts',(-0.233250985892042,0.0156370110386122,
0.0053620232486558));
#36835=CARTESIAN_POINT('Ctrl Pts',(-0.233253542558448,0.0155846994939661,
0.00548190301630521));
#36836=CARTESIAN_POINT('Ctrl Pts',(-0.231731717357689,0.0161403008067932,
0.00353064721372319));
#36837=CARTESIAN_POINT('Ctrl Pts',(-0.231695914333758,0.0160542161711817,
0.00348748907626018));
#36838=CARTESIAN_POINT('Ctrl Pts',(-0.231654208711274,0.016041360346251,
0.00357630360283988));
#36839=CARTESIAN_POINT('Ctrl Pts',(-0.2309214360969,0.016218849299512,0.00255390765191894));
#36840=CARTESIAN_POINT('Ctrl Pts',(-0.230917643482494,0.0161228769257979,
0.00254933591033697));
#36841=CARTESIAN_POINT('Ctrl Pts',(-0.230843546096085,0.0161191169217128,
0.00261050306621451));
#36842=CARTESIAN_POINT('Origin',(-0.192200819635407,0.0153254805636842,
0.0056));
#36843=CARTESIAN_POINT('Origin',(-0.192200819635407,0.0153254805636842,
0.00559999999999991));
#36844=CARTESIAN_POINT('Origin',(-0.194168411395185,0.0075,0.0056));
#36845=CARTESIAN_POINT('Origin',(-0.192768810476938,0.0154467402534237,
0.0056));
#36846=CARTESIAN_POINT('Origin',(-0.203884397086387,0.0154879659720582,
0.00559998733259232));
#36847=CARTESIAN_POINT('Origin',(-0.192768785940054,0.0154467401648028,
0.00559999999397933));
#36848=CARTESIAN_POINT('Origin',(-0.215,0.0155256283130765,0.0056));
#36849=CARTESIAN_POINT('Ctrl Pts',(-0.213229729843132,0.0157022153177789,
0.00520680787665651));
#36850=CARTESIAN_POINT('Ctrl Pts',(-0.213345218715168,0.0158225893493084,
0.00528453405189864));
#36851=CARTESIAN_POINT('Ctrl Pts',(-0.213196001721802,0.0157923672594748,
0.00534544678633676));
#36852=CARTESIAN_POINT('Ctrl Pts',(-0.214547134769444,0.0154162104902854,
0.00565430653154903));
#36853=CARTESIAN_POINT('Ctrl Pts',(-0.214582356671007,0.0156149459953766,
0.00559914657177998));
#36854=CARTESIAN_POINT('Ctrl Pts',(-0.214538193317879,0.0155026474148113,
0.00580706225979799));
#36855=CARTESIAN_POINT('Ctrl Pts',(-0.216690019804745,0.0155682893667712,
0.00552681293735305));
#36856=CARTESIAN_POINT('Ctrl Pts',(-0.216451145680206,0.0156840968084039,
0.00562885092889451));
#36857=CARTESIAN_POINT('Ctrl Pts',(-0.216722901066365,0.0156574855861506,
0.00567355244670012));
#36858=CARTESIAN_POINT('Ctrl Pts',(-0.218675003043817,0.0161056764401404,
0.00420057423278555));
#36859=CARTESIAN_POINT('Ctrl Pts',(-0.218617098144112,0.0162182154556049,
0.00425851519670619));
#36860=CARTESIAN_POINT('Ctrl Pts',(-0.218743439038924,0.0162011697080541,
0.00430773273508922));
#36861=CARTESIAN_POINT('Ctrl Pts',(-0.219591213832591,0.016366893294022,
0.00309190376565664));
#36862=CARTESIAN_POINT('Ctrl Pts',(-0.219573634362248,0.016475367130996,
0.00312025455357957));
#36863=CARTESIAN_POINT('Ctrl Pts',(-0.21967659313197,0.0164655000154654,
0.00316589708552006));
#36864=CARTESIAN_POINT('Ctrl Pts',(-0.22028001583951,0.0165005526889646,
0.00181590820288125));
#36865=CARTESIAN_POINT('Ctrl Pts',(-0.220272524676665,0.0166017602705409,
0.00183458973337379));
#36866=CARTESIAN_POINT('Ctrl Pts',(-0.220378568714464,0.0166007864600911,
0.00185228354006585));
#36867=CARTESIAN_POINT('Ctrl Pts',(-0.22064664085763,0.0165713244858559,
2.35907764938227E-6));
#36868=CARTESIAN_POINT('Ctrl Pts',(-0.220652325872645,0.0166753647140379,
2.36179922074191E-6));
#36869=CARTESIAN_POINT('Ctrl Pts',(-0.220752242592502,0.0166711024300162,
2.41267673127293E-6));
#36870=CARTESIAN_POINT('Ctrl Pts',(-0.220280060746434,0.0165005514591195,
-0.00181618365853376));
#36871=CARTESIAN_POINT('Ctrl Pts',(-0.220272599527913,0.0166017669045666,
-0.0018348368457429));
#36872=CARTESIAN_POINT('Ctrl Pts',(-0.220378614204616,0.0166007849096865,
-0.00185256631919835));
#36873=CARTESIAN_POINT('Ctrl Pts',(-0.219591366060322,0.0163669363399105,
-0.00309179373683757));
#36874=CARTESIAN_POINT('Ctrl Pts',(-0.219573740983601,0.016475396719567,
-0.00312018560140071));
#36875=CARTESIAN_POINT('Ctrl Pts',(-0.219676748701557,0.0164655437352039,
-0.00316578368963275));
#36876=CARTESIAN_POINT('Ctrl Pts',(-0.218673191355524,0.0161051953605198,
-0.00420222688246931));
#36877=CARTESIAN_POINT('Ctrl Pts',(-0.218615263580567,0.0162177542044613,
-0.00426021396407952));
#36878=CARTESIAN_POINT('Ctrl Pts',(-0.218741593455134,0.0162006827472677,
-0.00430943468512786));
#36879=CARTESIAN_POINT('Ctrl Pts',(-0.216693610859714,0.0155689870287889,
-0.00552479954599455));
#36880=CARTESIAN_POINT('Ctrl Pts',(-0.216455449539926,0.0156849298060722,
-0.00562628440487122));
#36881=CARTESIAN_POINT('Ctrl Pts',(-0.216726553008683,0.0156581905368916,
-0.00567148258730312));
#36882=CARTESIAN_POINT('Ctrl Pts',(-0.214542851116322,0.0154156975121673,
-0.00565574169440847));
#36883=CARTESIAN_POINT('Ctrl Pts',(-0.214576974400863,0.0156142882723724,
-0.00560107345113347));
#36884=CARTESIAN_POINT('Ctrl Pts',(-0.214533839877423,0.0155021297478814,
-0.00580853651161884));
#36885=CARTESIAN_POINT('Ctrl Pts',(-0.213238161199259,0.0157028755263122,
-0.00520501194558692));
#36886=CARTESIAN_POINT('Ctrl Pts',(-0.213354454181688,0.0158232964870154,
-0.00528243459469491));
#36887=CARTESIAN_POINT('Ctrl Pts',(-0.213204580729378,0.0157930357316283,
-0.00534359720917359));
#36888=CARTESIAN_POINT('Origin',(-0.215,0.0155256291596528,-0.00560000000000002));
#36889=CARTESIAN_POINT('Origin',(-0.203884398706272,0.0154879667406767,
-0.0055999873317088));
#36890=CARTESIAN_POINT('Origin',(-0.192768785327122,0.0154485451014724,
-0.00559995859404333));
#36891=CARTESIAN_POINT('Ctrl Pts',(-0.186128733753088,0.00811916857619173,
0.00989255350779034));
#36892=CARTESIAN_POINT('Ctrl Pts',(-0.186018778618736,0.00811313503271661,
0.00990168049066551));
#36893=CARTESIAN_POINT('Ctrl Pts',(-0.186023944961261,0.00811996577256876,
0.00979312213356084));
#36894=CARTESIAN_POINT('Ctrl Pts',(-0.186018485294857,0.00670554737044195,
0.00998601759439623));
#36895=CARTESIAN_POINT('Ctrl Pts',(-0.185922064757894,0.00670303587685495,
0.00998410879659885));
#36896=CARTESIAN_POINT('Ctrl Pts',(-0.185913335621815,0.00670391887197537,
0.00988488069051847));
#36897=CARTESIAN_POINT('Ctrl Pts',(-0.186483100624033,0.00435893839440719,
0.0095907193630887));
#36898=CARTESIAN_POINT('Ctrl Pts',(-0.186324782316601,0.00446640991982842,
0.00964072473835667));
#36899=CARTESIAN_POINT('Ctrl Pts',(-0.186378987360796,0.0043601940661907,
0.00949725178366898));
#36900=CARTESIAN_POINT('Ctrl Pts',(-0.188201072765365,0.00181549250946339,
0.00821893131634974));
#36901=CARTESIAN_POINT('Ctrl Pts',(-0.188078336118818,0.0018504078480918,
0.0082484121438556));
#36902=CARTESIAN_POINT('Ctrl Pts',(-0.188118956208556,0.00180751667010245,
0.00813902082106135));
#36903=CARTESIAN_POINT('Ctrl Pts',(-0.190470772042906,4.0286060397758E-5,
0.0065914793017016));
#36904=CARTESIAN_POINT('Ctrl Pts',(-0.190354564891624,6.51615565258696E-5,
0.00662079265626122));
#36905=CARTESIAN_POINT('Ctrl Pts',(-0.190415663760779,2.89000666232802E-5,
0.0065295234995035));
#36906=CARTESIAN_POINT('Ctrl Pts',(-0.192527761414073,-0.000596244059895659,
0.00555832684088505));
#36907=CARTESIAN_POINT('Ctrl Pts',(-0.19249929215549,-0.000615208227213908,
0.00553484330744896));
#36908=CARTESIAN_POINT('Ctrl Pts',(-0.192505145382581,-0.000612248109762194,
0.00550334510791334));
#36909=CARTESIAN_POINT('Ctrl Pts',(-0.193914490094568,-0.000653721049803873,
0.00545568506849627));
#36910=CARTESIAN_POINT('Ctrl Pts',(-0.193918273424759,-0.000668045313244978,
0.00543022477246777));
#36911=CARTESIAN_POINT('Ctrl Pts',(-0.19391192840682,-0.000669112281798238,
0.00540217205656248));
#36912=CARTESIAN_POINT('Origin',(-0.192768810476942,-0.000446740253424534,
0.00560000000000438));
#36913=CARTESIAN_POINT('Ctrl Pts',(-0.186116972251352,0.00692238523863633,
0.0098966261734716));
#36914=CARTESIAN_POINT('Ctrl Pts',(-0.186078299389446,0.00691967369755638,
0.0098954315730185));
#36915=CARTESIAN_POINT('Ctrl Pts',(-0.186041366807831,0.00691866352655612,
0.00986822062204796));
#36916=CARTESIAN_POINT('Ctrl Pts',(-0.186027502170506,0.00691962821437211,
0.0098347241084879));
#36917=CARTESIAN_POINT('Ctrl Pts',(-0.186022400056034,0.00691998321447427,
0.00982239756560122));
#36918=CARTESIAN_POINT('Ctrl Pts',(-0.186019959759874,0.00692055847709167,
0.00980946425272828));
#36919=CARTESIAN_POINT('Ctrl Pts',(-0.186019887800529,0.00692126510446277,
0.00979701417759536));
#36920=CARTESIAN_POINT('Origin',(-0.185989784446262,0.00750308162677683,
0.00987843431341192));
#36921=CARTESIAN_POINT('Origin',(-0.185989783463039,0.00749692179129775,
0.00987845623397708));
#36922=CARTESIAN_POINT('Ctrl Pts',(-0.186019887786807,0.00807873471322789,
0.00979701374348257));
#36923=CARTESIAN_POINT('Ctrl Pts',(-0.186020093677862,0.0080807581272644,
0.00983266188385409));
#36924=CARTESIAN_POINT('Ctrl Pts',(-0.186043173449962,0.00808148714810779,
0.00987274783946665));
#36925=CARTESIAN_POINT('Ctrl Pts',(-0.186081182198031,0.00807971774323728,
0.00988879730954875));
#36926=CARTESIAN_POINT('Ctrl Pts',(-0.186092525490223,0.0080791896838438,
0.00989358709710865));
#36927=CARTESIAN_POINT('Ctrl Pts',(-0.186104812966911,0.008078467319158,
0.00989625064514937));
#36928=CARTESIAN_POINT('Ctrl Pts',(-0.186116972833414,0.0080776147210469,
0.0098966261914198));
#36929=CARTESIAN_POINT('Ctrl Pts',(-0.186023972731768,0.00688051014267458,
0.00979310237707671));
#36930=CARTESIAN_POINT('Ctrl Pts',(-0.186018810213327,0.00688730839985145,
0.00990129751290525));
#36931=CARTESIAN_POINT('Ctrl Pts',(-0.186128366061288,0.00688133137396351,
0.009892610868904));
#36932=CARTESIAN_POINT('Ctrl Pts',(-0.185913319128721,0.00829598470916531,
0.00988477449605492));
#36933=CARTESIAN_POINT('Ctrl Pts',(-0.185921918992968,0.00829687156644818,
0.00998368580418176));
#36934=CARTESIAN_POINT('Ctrl Pts',(-0.186018138486974,0.00829436520850232,
0.00998594242117922));
#36935=CARTESIAN_POINT('Ctrl Pts',(-0.186379085964777,0.0106388494478239,
0.00949735159004442));
#36936=CARTESIAN_POINT('Ctrl Pts',(-0.186325170520145,0.0105330510663237,
0.00964031833428041));
#36937=CARTESIAN_POINT('Ctrl Pts',(-0.186482574570187,0.0106396543485447,
0.00959107234597323));
#36938=CARTESIAN_POINT('Ctrl Pts',(-0.188116939791643,0.0131908723913694,
0.00814009748260041));
#36939=CARTESIAN_POINT('Ctrl Pts',(-0.188076305605751,0.0131480938494406,
0.00824921860919713));
#36940=CARTESIAN_POINT('Ctrl Pts',(-0.188198545915983,0.0131827291314941,
0.00822019894550857));
#36941=CARTESIAN_POINT('Ctrl Pts',(-0.190415937111015,0.0149698341055998,
0.00653082897886206));
#36942=CARTESIAN_POINT('Ctrl Pts',(-0.190355170838482,0.0149336698703752,
0.006621860304423));
#36943=CARTESIAN_POINT('Ctrl Pts',(-0.190470436359477,0.0149583114745633,
0.00659299102128988));
#36944=CARTESIAN_POINT('Ctrl Pts',(-0.192492055253889,0.0156105230518145,
0.00550622573432866));
#36945=CARTESIAN_POINT('Ctrl Pts',(-0.192486126269825,0.0156134661142462,
0.00553773279556526));
#36946=CARTESIAN_POINT('Ctrl Pts',(-0.192514707567575,0.0155946170172933,
0.00556113935696853));
#36947=CARTESIAN_POINT('Ctrl Pts',(-0.193930356418938,0.0156719780414651,
0.00539761904618806));
#36948=CARTESIAN_POINT('Ctrl Pts',(-0.193936349353485,0.0156708752141232,
0.00542558152286841));
#36949=CARTESIAN_POINT('Ctrl Pts',(-0.193932726634534,0.0156566594700174,
0.0054509632651032));
#36950=CARTESIAN_POINT('Origin',(-0.19276881047694,0.015446740253424,0.00560000000000575));
#36951=CARTESIAN_POINT('Origin',(-0.192768810476937,0.0154467402534276,
0.0056));
#36952=CARTESIAN_POINT('Origin',(-0.185989784252021,0.00749691842201206,
-0.00987843432316569));
#36953=CARTESIAN_POINT('Ctrl Pts',(-0.186116972293536,0.00807761530404597,
-0.00989662596793202));
#36954=CARTESIAN_POINT('Ctrl Pts',(-0.186078299413494,0.00808032684892871,
-0.00989543136817047));
#36955=CARTESIAN_POINT('Ctrl Pts',(-0.186041366832626,0.00808133701405912,
-0.00986822040267438));
#36956=CARTESIAN_POINT('Ctrl Pts',(-0.186027502200621,0.00808037231720565,
-0.00983472388492247));
#36957=CARTESIAN_POINT('Ctrl Pts',(-0.186022400090923,0.00808001731397372,
-0.00982239734729829));
#36958=CARTESIAN_POINT('Ctrl Pts',(-0.186019959796752,0.00807944204809531,
-0.00980946404050643));
#36959=CARTESIAN_POINT('Ctrl Pts',(-0.186019887837588,0.00807873541742951,
-0.00979701396990226));
#36960=CARTESIAN_POINT('Ctrl Pts',(-0.193944739328741,0.0156748013854394,
-0.00539335846462329));
#36961=CARTESIAN_POINT('Ctrl Pts',(-0.193950405063627,0.0156736055039752,
-0.00542214039838788));
#36962=CARTESIAN_POINT('Ctrl Pts',(-0.193946792457245,0.0156587687228256,
-0.0054479092071319));
#36963=CARTESIAN_POINT('Ctrl Pts',(-0.192479951547028,0.0156079751812,-0.00551008560225899));
#36964=CARTESIAN_POINT('Ctrl Pts',(-0.192474038576552,0.0156110162627067,
-0.00554243345066391));
#36965=CARTESIAN_POINT('Ctrl Pts',(-0.192504190847607,0.0155911177095731,
-0.00556621720267825));
#36966=CARTESIAN_POINT('Ctrl Pts',(-0.190424348361861,0.0149720682294561,
-0.00652716548449426));
#36967=CARTESIAN_POINT('Ctrl Pts',(-0.190362307407983,0.0149351914758667,
-0.00662047975539135));
#36968=CARTESIAN_POINT('Ctrl Pts',(-0.190484255774687,0.0149617060832159,
-0.0065878831497931));
#36969=CARTESIAN_POINT('Ctrl Pts',(-0.188119418738792,0.0131951211101891,
-0.00813770573613879));
#36970=CARTESIAN_POINT('Ctrl Pts',(-0.188077128181627,0.0131507446359388,
-0.00825043507259777));
#36971=CARTESIAN_POINT('Ctrl Pts',(-0.188206302928862,0.0131885075000646,
-0.00821645594207363));
#36972=CARTESIAN_POINT('Ctrl Pts',(-0.18637868791602,0.0106375219868189,
-0.00949784839851767));
#36973=CARTESIAN_POINT('Ctrl Pts',(-0.186322706105325,0.0105275875956226,
-0.00964615897678578));
#36974=CARTESIAN_POINT('Ctrl Pts',(-0.186488066256925,0.0106423773751142,
-0.00958965009614401));
#36975=CARTESIAN_POINT('Ctrl Pts',(-0.185913669513949,0.00830000359003704,
-0.00988441259603338));
#36976=CARTESIAN_POINT('Ctrl Pts',(-0.185922643233334,0.00830115989286702,
-0.00998702246588958));
#36977=CARTESIAN_POINT('Ctrl Pts',(-0.186021834644838,0.00829826476234554,
-0.00998560862165242));
#36978=CARTESIAN_POINT('Ctrl Pts',(-0.186023567857763,0.00687519942614235,
-0.0097934618530046));
#36979=CARTESIAN_POINT('Ctrl Pts',(-0.186018168818418,0.00688206724060213,
-0.00990578909223112));
#36980=CARTESIAN_POINT('Ctrl Pts',(-0.186131856313941,0.00687583464295538,
-0.00989260188754259));
#36981=CARTESIAN_POINT('Origin',(-0.192768813717277,0.0154467408241202,
-0.0056));
#36982=CARTESIAN_POINT('Origin',(-0.192768813717277,0.0154467408241202,
-0.0056));
#36983=CARTESIAN_POINT('Origin',(-0.192768813717277,0.0154467408241202,
-0.0056));
#36984=CARTESIAN_POINT('Origin',(-0.194168411395185,0.0075,-0.0056));
#36985=CARTESIAN_POINT('Origin',(-0.192200822443821,0.0153254812698141,
-0.0056));
#36986=CARTESIAN_POINT('Origin',(-0.192200822443821,0.0153254812698141,
-0.0056));
#36987=CARTESIAN_POINT('Origin',(-0.18598978326554,0.00750307815796359,
-0.00987845625295267));
#36988=CARTESIAN_POINT('Ctrl Pts',(-0.186019887823865,0.00692126476492155,
-0.00979701353578103));
#36989=CARTESIAN_POINT('Ctrl Pts',(-0.186020093714527,0.00691924134015948,
-0.00983266168510107));
#36990=CARTESIAN_POINT('Ctrl Pts',(-0.186043173490947,0.00691851231002105,
-0.00987274764345759));
#36991=CARTESIAN_POINT('Ctrl Pts',(-0.186081182254119,0.00692028171431255,
-0.00988879711126473));
#36992=CARTESIAN_POINT('Ctrl Pts',(-0.186092525541513,0.00692080977310006,
-0.00989358689421662));
#36993=CARTESIAN_POINT('Ctrl Pts',(-0.186104813013035,0.00692153213765697,
-0.00989625044013151));
#36994=CARTESIAN_POINT('Ctrl Pts',(-0.186116972875644,0.00692238473624832,
-0.00989662598588015));
#36995=CARTESIAN_POINT('Ctrl Pts',(-0.186024639723174,0.00812811219565812,
-0.00979252019536039));
#36996=CARTESIAN_POINT('Ctrl Pts',(-0.186019307378118,0.00812086552414072,
-0.00990231673970523));
#36997=CARTESIAN_POINT('Ctrl Pts',(-0.186130557641939,0.00812738702814064,
-0.00989184348985861));
#36998=CARTESIAN_POINT('Ctrl Pts',(-0.185911665726943,0.00670243418658247,
-0.00988630161052383));
#36999=CARTESIAN_POINT('Ctrl Pts',(-0.185920664362397,0.00670182531369318,
-0.00998651802648809));
#37000=CARTESIAN_POINT('Ctrl Pts',(-0.186017796509969,0.00670406967969763,
-0.00998748004843489));
#37001=CARTESIAN_POINT('Ctrl Pts',(-0.186383092477577,0.00434243298325542,
-0.00949365754992548));
#37002=CARTESIAN_POINT('Ctrl Pts',(-0.186327057599337,0.00445165179097786,
-0.00963954915710208));
#37003=CARTESIAN_POINT('Ctrl Pts',(-0.186488965294518,0.00433989462961623,
-0.00958646459001603));
#37004=CARTESIAN_POINT('Ctrl Pts',(-0.18814229846019,0.00178054587572309,
-0.00812126933382206));
#37005=CARTESIAN_POINT('Ctrl Pts',(-0.188100433060655,0.00182438698528336,
-0.00823203675775219));
#37006=CARTESIAN_POINT('Ctrl Pts',(-0.188225725746846,0.00178808327780345,
-0.00820056143173852));
#37007=CARTESIAN_POINT('Ctrl Pts',(-0.19044452191719,1.6202403067083E-5,
-0.00651141629438544));
#37008=CARTESIAN_POINT('Ctrl Pts',(-0.19038385400963,5.14577023083873E-5,
-0.00660218703061461));
#37009=CARTESIAN_POINT('Ctrl Pts',(-0.190500763004092,2.74049476685753E-5,
-0.00657287877422572));
#37010=CARTESIAN_POINT('Ctrl Pts',(-0.19253117826135,-0.000615266065116062,
-0.00549731033749768));
#37011=CARTESIAN_POINT('Ctrl Pts',(-0.192526147348343,-0.000618092939049415,
-0.00552868410424512));
#37012=CARTESIAN_POINT('Ctrl Pts',(-0.19255375702597,-0.000599009037967802,
-0.00555258554180868));
#37013=CARTESIAN_POINT('Ctrl Pts',(-0.193918783756537,-0.000668624514627959,
-0.00540402469955559));
#37014=CARTESIAN_POINT('Ctrl Pts',(-0.193924564628155,-0.000667662297456414,
-0.00543253495238252));
#37015=CARTESIAN_POINT('Ctrl Pts',(-0.193921264643106,-0.000653011155466118,
-0.00545790459201301));
#37016=CARTESIAN_POINT('Ctrl Pts',(-0.192768459141627,-0.000531128306595919,
-0.00565363457355974));
#37017=CARTESIAN_POINT('Ctrl Pts',(-0.19276562570579,-0.000541650536466089,
-0.00563706845375414));
#37018=CARTESIAN_POINT('Ctrl Pts',(-0.192762819238559,-0.000547210055500382,
-0.00561736740483649));
#37019=CARTESIAN_POINT('Ctrl Pts',(-0.192760018688902,-0.000546732541444601,
-0.00559775525115174));
#37020=CARTESIAN_POINT('Origin',(-0.203590952700175,-0.000486871388071358,
-0.0055999858664995));
#37021=CARTESIAN_POINT('Origin',(-0.215,-0.000525629159653763,-0.0056));
#37022=CARTESIAN_POINT('Ctrl Pts',(-0.213229730364857,-0.000702212951003181,
-0.00520680784009235));
#37023=CARTESIAN_POINT('Ctrl Pts',(-0.21334554019071,-0.000822928423967307,
-0.0052847510567193));
#37024=CARTESIAN_POINT('Ctrl Pts',(-0.213195754239947,-0.000792314496048851,
-0.00534554749344366));
#37025=CARTESIAN_POINT('Ctrl Pts',(-0.214547134435015,-0.000416213562106486,
-0.00565430653835661));
#37026=CARTESIAN_POINT('Ctrl Pts',(-0.214582465858957,-0.00061556757186644,
-0.00559897618104724));
#37027=CARTESIAN_POINT('Ctrl Pts',(-0.214538126572902,-0.000502481732189858,
-0.00580737405250504));
#37028=CARTESIAN_POINT('Ctrl Pts',(-0.216690020107536,-0.000568288146151568,
-0.00552681299596838));
#37029=CARTESIAN_POINT('Ctrl Pts',(-0.216450453443573,-0.000684435862739555,
-0.00562914645532142));
#37030=CARTESIAN_POINT('Ctrl Pts',(-0.216723337291576,-0.00065744162975446,
-0.00567362346679069));
#37031=CARTESIAN_POINT('Ctrl Pts',(-0.218675003475181,-0.00110567341750779,
-0.00420057382676157));
#37032=CARTESIAN_POINT('Ctrl Pts',(-0.218616955185385,-0.00121849151929721,
-0.0042586581440736));
#37033=CARTESIAN_POINT('Ctrl Pts',(-0.218743679225851,-0.00120113404056507,
-0.00430782564282987));
#37034=CARTESIAN_POINT('Ctrl Pts',(-0.21959121396959,-0.00136689275323617,
-0.0030919035315441));
#37035=CARTESIAN_POINT('Ctrl Pts',(-0.219573593820357,-0.0014756160323326,
-0.00312031990591821));
#37036=CARTESIAN_POINT('Ctrl Pts',(-0.219676803998535,-0.00146547899713251,
-0.00316599038852783));
#37037=CARTESIAN_POINT('Ctrl Pts',(-0.220280015856011,-0.00150055300539941,
-0.00181590812685752));
#37038=CARTESIAN_POINT('Ctrl Pts',(-0.220272508157456,-0.0016019827403939,
-0.00183463094445556));
#37039=CARTESIAN_POINT('Ctrl Pts',(-0.220378796107586,-0.00160078446929803,
-0.00185232121959389));
#37040=CARTESIAN_POINT('Ctrl Pts',(-0.220646640852067,-0.00157132448681648,
-2.35895081128692E-6));
#37041=CARTESIAN_POINT('Ctrl Pts',(-0.220652338405761,-0.00167559421886387,
-2.36109324866209E-6));
#37042=CARTESIAN_POINT('Ctrl Pts',(-0.22075245579331,-0.00167109309083381,
-2.41275124305137E-6));
#37043=CARTESIAN_POINT('Ctrl Pts',(-0.220280060746729,-0.00150055113982659,
0.00181618363817644));
#37044=CARTESIAN_POINT('Ctrl Pts',(-0.220272583236875,-0.00160198890362842,
0.00183487750996121));
#37045=CARTESIAN_POINT('Ctrl Pts',(-0.220378841515704,-0.00160078222822346,
0.00185260440179092));
#37046=CARTESIAN_POINT('Ctrl Pts',(-0.219591366035501,-0.00136693691002698,
0.00309179380892092));
#37047=CARTESIAN_POINT('Ctrl Pts',(-0.219573700695601,-0.00147564663065069,
0.0031202505503224));
#37048=CARTESIAN_POINT('Ctrl Pts',(-0.219676959497499,-0.00146552392066298,
0.00316587679000158));
#37049=CARTESIAN_POINT('Ctrl Pts',(-0.218673190971741,-0.00110519840036426,
0.0042022272613154));
#37050=CARTESIAN_POINT('Ctrl Pts',(-0.21861511946106,-0.00121803612509124,
0.0042603583574915));
#37051=CARTESIAN_POINT('Ctrl Pts',(-0.218741832748112,-0.00120065320451856,
0.00430952815393783));
#37052=CARTESIAN_POINT('Ctrl Pts',(-0.216693610695147,-0.000568988272581022,
0.00552479943366079));
#37053=CARTESIAN_POINT('Ctrl Pts',(-0.216454744952011,-0.000685269450178146,
0.00562658481509268));
#37054=CARTESIAN_POINT('Ctrl Pts',(-0.216726987943305,-0.000658148482718064,
0.00567155509388602));
#37055=CARTESIAN_POINT('Ctrl Pts',(-0.214542851347544,-0.000415694418949238,
0.00565574173556768));
#37056=CARTESIAN_POINT('Ctrl Pts',(-0.214577081649168,-0.000614907730571467,
0.00560090086194077));
#37057=CARTESIAN_POINT('Ctrl Pts',(-0.214533775275375,-0.000501957450787837,
0.00580884872688636));
#37058=CARTESIAN_POINT('Ctrl Pts',(-0.21323816078666,-0.000702877922631073,
0.0052050119165415));
#37059=CARTESIAN_POINT('Ctrl Pts',(-0.213354787946414,-0.000823638003085672,
0.00528265601711787));
#37060=CARTESIAN_POINT('Ctrl Pts',(-0.213204331015681,-0.000792987504077056,
0.00534369882673873));
#37061=CARTESIAN_POINT('Origin',(-0.215,-0.000525628313076073,0.0056));
#37062=CARTESIAN_POINT('Origin',(-0.2038843971522,-0.000487965972298664,
0.00559998733259273));
#37063=CARTESIAN_POINT('Origin',(-0.192768785940078,-0.000446740164802543,
0.00559999999397934));
#37064=CARTESIAN_POINT('Origin',(-0.192768810476959,-0.00044674025342738,
0.0056));
#37065=CARTESIAN_POINT('Origin',(-0.192768810476942,-0.000446740253424536,
0.00560000000000438));
#37066=CARTESIAN_POINT('Origin',(-0.194168411395185,0.0075,0.0056));
#37067=CARTESIAN_POINT('Origin',(-0.192200819635406,-0.000325480563683811,
0.0056));
#37068=CARTESIAN_POINT('Origin',(-0.192200819635406,-0.000325480563683833,
0.0056));
#37069=CARTESIAN_POINT('Origin',(-0.23397529105232,0.0160594292892167,-2.10028825614146E-10));
#37070=CARTESIAN_POINT('Origin',(-0.230844479079951,0.0163191139685996,
0.00261776387735059));
#37071=CARTESIAN_POINT('Origin',(-0.230844479057671,0.0163191137983529,
-0.0026177638505009));
#37072=CARTESIAN_POINT('Ctrl Pts',(-0.228930011320165,-0.00121666210944132,
-0.000153558508944395));
#37073=CARTESIAN_POINT('Ctrl Pts',(-0.228925068649108,-0.00130356078038321,
-0.00014061325969051));
#37074=CARTESIAN_POINT('Ctrl Pts',(-0.228852816272702,-0.00131993372474197,
-0.000198511747305299));
#37075=CARTESIAN_POINT('Ctrl Pts',(-0.230431551941403,-0.00149901747374101,
-0.00196359261958752));
#37076=CARTESIAN_POINT('Ctrl Pts',(-0.230546199755791,-0.00163485191727014,
-0.00209314633244308));
#37077=CARTESIAN_POINT('Ctrl Pts',(-0.230356760340796,-0.00160667853259381,
-0.00203317374358696));
#37078=CARTESIAN_POINT('Ctrl Pts',(-0.232741868391858,-0.00122412725612965,
-0.00474856455279266));
#37079=CARTESIAN_POINT('Ctrl Pts',(-0.233002328000619,-0.00122807080927364,
-0.00505085271150412));
#37080=CARTESIAN_POINT('Ctrl Pts',(-0.232669082600517,-0.00132530889872912,
-0.00485258198260278));
#37081=CARTESIAN_POINT('Ctrl Pts',(-0.235571864603083,0.000893540287141985,
-0.00815998429435824));
#37082=CARTESIAN_POINT('Ctrl Pts',(-0.235780526318094,0.000886440100530878,
-0.00839417044424366));
#37083=CARTESIAN_POINT('Ctrl Pts',(-0.23549602082886,0.000816861323350659,
-0.00829967543390585));
#37084=CARTESIAN_POINT('Ctrl Pts',(-0.237350191606613,0.00367117676218051,
-0.0103036684753349));
#37085=CARTESIAN_POINT('Ctrl Pts',(-0.237562885455937,0.00375230645071915,
-0.0105367888728918));
#37086=CARTESIAN_POINT('Ctrl Pts',(-0.237273146969764,0.00362802005513088,
-0.0104664740917656));
#37087=CARTESIAN_POINT('Ctrl Pts',(-0.237978275379249,0.00684374843593728,
-0.011060791815887));
#37088=CARTESIAN_POINT('Ctrl Pts',(-0.23815533351796,0.00681408943718553,
-0.0112478230763381));
#37089=CARTESIAN_POINT('Ctrl Pts',(-0.237900276754974,0.00683577450692037,
-0.011231052981414));
#37090=CARTESIAN_POINT('Ctrl Pts',(-0.237735579461005,0.00941406809132023,
-0.0107682341472069));
#37091=CARTESIAN_POINT('Ctrl Pts',(-0.237905547438819,0.00945031005365003,
-0.0109479806253355));
#37092=CARTESIAN_POINT('Ctrl Pts',(-0.237657647464612,0.00943669370360537,
-0.010935275193432));
#37093=CARTESIAN_POINT('Ctrl Pts',(-0.237055387725117,0.0117812538241882,
-0.00994829713676746));
#37094=CARTESIAN_POINT('Ctrl Pts',(-0.237219994321457,0.0118075629637152,
-0.0101246180217082));
#37095=CARTESIAN_POINT('Ctrl Pts',(-0.236977820224706,0.0118312943583801,
-0.0101063746716028));
#37096=CARTESIAN_POINT('Ctrl Pts',(-0.235580244204118,0.0140975190661438,
-0.00817008549077605));
#37097=CARTESIAN_POINT('Ctrl Pts',(-0.23578623244027,0.0141029322156517,
-0.00840102389984029));
#37098=CARTESIAN_POINT('Ctrl Pts',(-0.235504346470908,0.01417405436759,
-0.00830983268046781));
#37099=CARTESIAN_POINT('Ctrl Pts',(-0.232754563684081,0.0162205064390394,
-0.00476386809962718));
#37100=CARTESIAN_POINT('Ctrl Pts',(-0.233017755071115,0.0162243053630947,
-0.005069430660515));
#37101=CARTESIAN_POINT('Ctrl Pts',(-0.232681829483814,0.016321647383219,
-0.00486812521810131));
#37102=CARTESIAN_POINT('Ctrl Pts',(-0.230420611920092,0.0165030822444603,
-0.00195040496493689));
#37103=CARTESIAN_POINT('Ctrl Pts',(-0.230536669856679,0.0166381031145872,
-0.0020816713149296));
#37104=CARTESIAN_POINT('Ctrl Pts',(-0.230345861479217,0.0166107689301663,
-0.00201988343589639));
#37105=CARTESIAN_POINT('Ctrl Pts',(-0.22894365783775,0.0162108337471327,
-0.000170008710922436));
#37106=CARTESIAN_POINT('Ctrl Pts',(-0.228934589862323,0.0162990618020438,
-0.000152076705750483));
#37107=CARTESIAN_POINT('Ctrl Pts',(-0.228866347045808,0.0163140754347603,
-0.00021501163526663));
#37108=CARTESIAN_POINT('Origin',(-0.230844479079726,-0.00131911379624309,
-0.00261776387708007));
#37109=CARTESIAN_POINT('Ctrl Pts',(-0.228930018643561,0.0162166782265411,
0.000153567348635035));
#37110=CARTESIAN_POINT('Ctrl Pts',(-0.228925034474289,0.0163035747204591,
0.000140571617611529));
#37111=CARTESIAN_POINT('Ctrl Pts',(-0.228852822004403,0.0163199491706983,
0.00019852322100711));
#37112=CARTESIAN_POINT('Ctrl Pts',(-0.230431547159926,0.0164990010424598,
0.00196358686148426));
#37113=CARTESIAN_POINT('Ctrl Pts',(-0.230546210928832,0.0166348359316639,
0.00209315975026496));
#37114=CARTESIAN_POINT('Ctrl Pts',(-0.23035675495291,0.0166066625558943,
0.00203316613867527));
#37115=CARTESIAN_POINT('Ctrl Pts',(-0.232741874999713,0.0162241552295754,
0.00474857253009821));
#37116=CARTESIAN_POINT('Ctrl Pts',(-0.233002336525729,0.0162280967339862,
0.00505086248822097));
#37117=CARTESIAN_POINT('Ctrl Pts',(-0.232669087560718,0.0163253369091607,
0.00485259065406883));
#37118=CARTESIAN_POINT('Ctrl Pts',(-0.235571844631025,0.0141064194522958,
0.00815996023088895));
#37119=CARTESIAN_POINT('Ctrl Pts',(-0.235780503221004,0.0141135232971628,
0.00839414213517375));
#37120=CARTESIAN_POINT('Ctrl Pts',(-0.235495999776369,0.0141830986004907,
0.00829965082076248));
#37121=CARTESIAN_POINT('Ctrl Pts',(-0.23735020499403,0.0113288345386507,
0.0103036846257339));
#37122=CARTESIAN_POINT('Ctrl Pts',(-0.237562903802203,0.0112477073380563,
0.0105368103191969));
#37123=CARTESIAN_POINT('Ctrl Pts',(-0.237273159453406,0.0113719926988885,
0.0104664898863485));
#37124=CARTESIAN_POINT('Ctrl Pts',(-0.237978272727021,0.00815624622582596,
0.0110607886321847));
#37125=CARTESIAN_POINT('Ctrl Pts',(-0.238155332546526,0.0081858990714908,
0.0112478210492935));
#37126=CARTESIAN_POINT('Ctrl Pts',(-0.23790027337051,0.00816421945360661,
0.0112310497653436));
#37127=CARTESIAN_POINT('Ctrl Pts',(-0.237735583958034,0.00558592810337824,
0.0107682395816002));
#37128=CARTESIAN_POINT('Ctrl Pts',(-0.237905555367753,0.00554968907454929,
0.0109479892946036));
#37129=CARTESIAN_POINT('Ctrl Pts',(-0.237657651224066,0.00556330322602589,
0.0109352808534232));
#37130=CARTESIAN_POINT('Ctrl Pts',(-0.237055393487095,0.00321874016769531,
0.00994830409475942));
#37131=CARTESIAN_POINT('Ctrl Pts',(-0.23722000314611,0.0031924317775692,
0.0101246280895804));
#37132=CARTESIAN_POINT('Ctrl Pts',(-0.236977825203511,0.00316869826984275,
0.0101063812287948));
#37133=CARTESIAN_POINT('Ctrl Pts',(-0.235580224122505,0.000902521439204644,
0.00817006129529639));
#37134=CARTESIAN_POINT('Ctrl Pts',(-0.235786207806912,0.000897102342494172,
0.00840099372924289));
#37135=CARTESIAN_POINT('Ctrl Pts',(-0.235504325292979,0.000825986039287472,
0.00830980795273018));
#37136=CARTESIAN_POINT('Ctrl Pts',(-0.232754570759086,-0.00122053420958835,
0.00476387664005792));
#37137=CARTESIAN_POINT('Ctrl Pts',(-0.233017765329059,-0.00122432956214392,
0.00506944252624999));
#37138=CARTESIAN_POINT('Ctrl Pts',(-0.232681834927955,-0.00132167522919554,
0.00486813447178729));
#37139=CARTESIAN_POINT('Ctrl Pts',(-0.230420606752338,-0.00150306601983695,
0.00195039874119751));
#37140=CARTESIAN_POINT('Ctrl Pts',(-0.230536680061682,-0.00163808816037902,
0.00208168356580272));
#37141=CARTESIAN_POINT('Ctrl Pts',(-0.23034585568313,-0.00161075313981024,
0.00201987533518042));
#37142=CARTESIAN_POINT('Ctrl Pts',(-0.228943665649166,-0.00121084957355264,
0.000170018138880857));
#37143=CARTESIAN_POINT('Ctrl Pts',(-0.228934556962248,-0.00129907450314452,
0.000152036599788699));
#37144=CARTESIAN_POINT('Ctrl Pts',(-0.228866353311391,-0.00131409060945743,
0.000215023759721046));
#37145=CARTESIAN_POINT('Origin',(-0.230844479057897,-0.00131911397071442,
0.00261776385077347));
#37146=CARTESIAN_POINT('Origin',(-0.233975291052864,-0.00105942928952791,
2.16727099247223E-10));
#37147=CARTESIAN_POINT('Origin',(-0.226549796019406,0.0104788589677295,
-0.00737701084641453));
#37148=CARTESIAN_POINT('Ctrl Pts',(-0.225965068063626,0.0102955231026494,
-0.0103688478531334));
#37149=CARTESIAN_POINT('Ctrl Pts',(-0.225965835469434,0.0102847030452682,
-0.0103375543236173));
#37150=CARTESIAN_POINT('Ctrl Pts',(-0.22596662506635,0.0102740358497316,
-0.0103060888750999));
#37151=CARTESIAN_POINT('Ctrl Pts',(-0.225967436625428,0.0102635326203732,
-0.0102744751969217));
#37152=CARTESIAN_POINT('Ctrl Pts',(-0.224903047769934,0.0163974953490442,
0.00232527569536224));
#37153=CARTESIAN_POINT('Ctrl Pts',(-0.228003678801843,0.0163652528946496,
0.00231821622721085));
#37154=CARTESIAN_POINT('Ctrl Pts',(-0.23110431006382,0.0163330357098684,
0.00231114482972889));
#37155=CARTESIAN_POINT('Ctrl Pts',(-0.234204941533998,0.0163008422866106,
0.00230405918705812));
#37156=CARTESIAN_POINT('Ctrl Pts',(-0.224902923051373,0.016421905903896,
0.001999690061282));
#37157=CARTESIAN_POINT('Ctrl Pts',(-0.228003554472057,0.0163857948128496,
0.00199154431614981));
#37158=CARTESIAN_POINT('Ctrl Pts',(-0.231104186130884,0.0163497065102629,
0.00198339075959686));
#37159=CARTESIAN_POINT('Ctrl Pts',(-0.23420481801057,0.0163136399270852,
0.00197522735965944));
#37160=CARTESIAN_POINT('Ctrl Pts',(-0.224902686634519,0.0164496060066283,
0.00134999605462854));
#37161=CARTESIAN_POINT('Ctrl Pts',(-0.228003316903349,0.0164061218898441,
0.00134119319572166));
#37162=CARTESIAN_POINT('Ctrl Pts',(-0.231103947348719,0.0163626446434222,
0.00133240817680761));
#37163=CARTESIAN_POINT('Ctrl Pts',(-0.234204577993315,0.0163191760221561,
0.00132364096404516));
#37164=CARTESIAN_POINT('Ctrl Pts',(-0.22490247733934,0.0164891827557564,
8.48946422705292E-5));
#37165=CARTESIAN_POINT('Ctrl Pts',(-0.2280031047451,0.0164387037966636,
8.36968421714054E-5));
#37166=CARTESIAN_POINT('Ctrl Pts',(-0.231103732057188,0.01638822192355,
8.25020821930779E-5));
#37167=CARTESIAN_POINT('Ctrl Pts',(-0.234204359262361,0.016337735996471,
8.13110569434896E-5));
#37168=CARTESIAN_POINT('Ctrl Pts',(-0.224902601832635,0.0164577305274795,
-0.00116946331798178));
#37169=CARTESIAN_POINT('Ctrl Pts',(-0.22800323228218,0.0164115731563456,
-0.00115947279336496));
#37170=CARTESIAN_POINT('Ctrl Pts',(-0.231103862912676,0.016365419418937,
-0.00114950763219157));
#37171=CARTESIAN_POINT('Ctrl Pts',(-0.234204493754791,0.0163192718567599,
-0.00113956819841304));
#37172=CARTESIAN_POINT('Ctrl Pts',(-0.2249031047193,0.016401050271707,-0.00247428944274167));
#37173=CARTESIAN_POINT('Ctrl Pts',(-0.228003735976318,0.016370691448232,
-0.00246735407024901));
#37174=CARTESIAN_POINT('Ctrl Pts',(-0.231104367476673,0.0163403620163895,
-0.00246039974613875));
#37175=CARTESIAN_POINT('Ctrl Pts',(-0.234204999188339,0.0163100597051565,
-0.00245342363871553));
#37176=CARTESIAN_POINT('Ctrl Pts',(-0.224903620482978,0.0162331344936927,
-0.00377581649114323));
#37177=CARTESIAN_POINT('Ctrl Pts',(-0.228004247053984,0.0162183248288798,
-0.00377611183675602));
#37178=CARTESIAN_POINT('Ctrl Pts',(-0.231104873706723,0.0162035348039987,
-0.00377640360674382));
#37179=CARTESIAN_POINT('Ctrl Pts',(-0.23420550044494,0.0161887639228305,
-0.00377669038870648));
#37180=CARTESIAN_POINT('Ctrl Pts',(-0.224904244439412,0.0157454055087051,
-0.00535508843351867));
#37181=CARTESIAN_POINT('Ctrl Pts',(-0.228004869356698,0.015745877431058,
-0.00536654194974573));
#37182=CARTESIAN_POINT('Ctrl Pts',(-0.231105494288016,0.0157463686608469,
-0.00537798949180189));
#37183=CARTESIAN_POINT('Ctrl Pts',(-0.234206119236561,0.0157468784277487,
-0.00538942975580705));
#37184=CARTESIAN_POINT('Ctrl Pts',(-0.224904927056323,0.014756116525245,
-0.0070809462510311));
#37185=CARTESIAN_POINT('Ctrl Pts',(-0.228005551277712,0.0147682738612367,
-0.00710847555851588));
#37186=CARTESIAN_POINT('Ctrl Pts',(-0.231106175457583,0.0147804448844733,
-0.00713600323790223));
#37187=CARTESIAN_POINT('Ctrl Pts',(-0.234206799604821,0.014792629252247,
-0.00716352865861212));
#37188=CARTESIAN_POINT('Ctrl Pts',(-0.224905705935764,0.0129587456084716,
-0.00904270204015799));
#37189=CARTESIAN_POINT('Ctrl Pts',(-0.228006331471737,0.0129775263446935,
-0.00909152831654588));
#37190=CARTESIAN_POINT('Ctrl Pts',(-0.231106956961612,0.0129963155259409,
-0.00914035417356039));
#37191=CARTESIAN_POINT('Ctrl Pts',(-0.234207582410669,0.0130151128918419,
-0.00918917939755658));
#37192=CARTESIAN_POINT('Ctrl Pts',(-0.224906344901157,0.00996717482975785,
-0.0106558172504251));
#37193=CARTESIAN_POINT('Ctrl Pts',(-0.228006973196984,0.00997888641244874,
-0.0107253416344494));
#37194=CARTESIAN_POINT('Ctrl Pts',(-0.23110760149003,0.00999060093234777,
-0.0107948661290257));
#37195=CARTESIAN_POINT('Ctrl Pts',(-0.234208229780548,0.0100023182636535,
-0.010864390745125));
#37196=CARTESIAN_POINT('Ctrl Pts',(-0.224906421473904,0.00588448586822914,
-0.0108495989887083));
#37197=CARTESIAN_POINT('Ctrl Pts',(-0.228007050197119,0.00587660352368733,
-0.0109217704181749));
#37198=CARTESIAN_POINT('Ctrl Pts',(-0.231107678925808,0.00586871925150363,
-0.0109939418074081));
#37199=CARTESIAN_POINT('Ctrl Pts',(-0.23420830765933,0.00586083314294305,
-0.0110661131658069));
#37200=CARTESIAN_POINT('Ctrl Pts',(-0.224905896797368,0.00275206275993148,
-0.00952499259309634));
#37201=CARTESIAN_POINT('Ctrl Pts',(-0.22800652301585,0.00273399542249794,
-0.00957977151548));
#37202=CARTESIAN_POINT('Ctrl Pts',(-0.231107149196805,0.00271592133715538,
-0.00963455045765119));
#37203=CARTESIAN_POINT('Ctrl Pts',(-0.234207775344483,0.00269784071003669,
-0.00968932931015458));
#37204=CARTESIAN_POINT('Ctrl Pts',(-0.224905188461513,0.000775386387695849,
-0.00774097724716007));
#37205=CARTESIAN_POINT('Ctrl Pts',(-0.228005812987761,0.000760338332521188,
-0.0077754138708565));
#37206=CARTESIAN_POINT('Ctrl Pts',(-0.231106437467874,0.000745278047377309,
-0.00780984908461508));
#37207=CARTESIAN_POINT('Ctrl Pts',(-0.234207061909447,0.000730205873823641,
-0.00784428237662763));
#37208=CARTESIAN_POINT('Ctrl Pts',(-0.224904545212544,-0.00037433699893992,
-0.00611286595312136));
#37209=CARTESIAN_POINT('Ctrl Pts',(-0.228005169500613,-0.000380655003703386,
-0.00613103039787742));
#37210=CARTESIAN_POINT('Ctrl Pts',(-0.231105793767721,-0.000386989095479687,
-0.00614919200572512));
#37211=CARTESIAN_POINT('Ctrl Pts',(-0.234206418022201,-0.000393338834079428,
-0.00616734988680402));
#37212=CARTESIAN_POINT('Ctrl Pts',(-0.224903937950997,-0.00100476933014151,
-0.00458381173225385));
#37213=CARTESIAN_POINT('Ctrl Pts',(-0.228004563842973,-0.000997949740617374,
-0.00458943898701532));
#37214=CARTESIAN_POINT('Ctrl Pts',(-0.231105189790958,-0.000991151361328939,
-0.00459505880592969));
#37215=CARTESIAN_POINT('Ctrl Pts',(-0.234205815794275,-0.000984373265027772,
-0.00460066961067425));
#37216=CARTESIAN_POINT('Ctrl Pts',(-0.224903434943426,-0.00130314167877163,
-0.00330350941820122));
#37217=CARTESIAN_POINT('Ctrl Pts',(-0.228004062879574,-0.00128286930948369,
-0.00330122419140405));
#37218=CARTESIAN_POINT('Ctrl Pts',(-0.231104690943801,-0.00126261869681616,
-0.0032989320974583));
#37219=CARTESIAN_POINT('Ctrl Pts',(-0.234205319131308,-0.00124238896138437,
-0.00329663139924215));
#37220=CARTESIAN_POINT('Ctrl Pts',(-0.224903041260456,-0.00140805611840559,
-0.00232453718253355));
#37221=CARTESIAN_POINT('Ctrl Pts',(-0.228003673257076,-0.0013756315595115,
-0.00231672000225054));
#37222=CARTESIAN_POINT('Ctrl Pts',(-0.231104305522642,-0.00134323774830377,
-0.00230888218475535));
#37223=CARTESIAN_POINT('Ctrl Pts',(-0.234204938019884,-0.00131087220379368,
-0.00230102069899992));
#37224=CARTESIAN_POINT('Ctrl Pts',(-0.224902686634356,-0.00144960594189391,
-0.00134999602285112));
#37225=CARTESIAN_POINT('Ctrl Pts',(-0.228003316903184,-0.00140612182039602,
-0.00134119316178982));
#37226=CARTESIAN_POINT('Ctrl Pts',(-0.23110394734855,-0.00136264456921374,
-0.00133240814074275));
#37227=CARTESIAN_POINT('Ctrl Pts',(-0.234204577993143,-0.00131917594314456,
-0.00132364092587474));
#37228=CARTESIAN_POINT('Ctrl Pts',(-0.22490247733939,-0.0014891827680679,
-8.48946648711828E-5));
#37229=CARTESIAN_POINT('Ctrl Pts',(-0.228003104745152,-0.00143870380997731,
-8.36968663193096E-5));
#37230=CARTESIAN_POINT('Ctrl Pts',(-0.231103732057244,-0.00138822193789455,
-8.25021078797203E-5));
#37231=CARTESIAN_POINT('Ctrl Pts',(-0.23420435926242,-0.00133773601187166,
-8.1311084157012E-5));
#37232=CARTESIAN_POINT('Ctrl Pts',(-0.22490260183294,-0.0014577307002292,
0.00116946334942344));
#37233=CARTESIAN_POINT('Ctrl Pts',(-0.228003232282475,-0.00141157334093523,
0.00115947282708936));
#37234=CARTESIAN_POINT('Ctrl Pts',(-0.231103862912961,-0.00136541961535455,
0.00114950766822477));
#37235=CARTESIAN_POINT('Ctrl Pts',(-0.234204493755065,-0.001319272064998,
0.00113956823678177));
#37236=CARTESIAN_POINT('Ctrl Pts',(-0.224903104718753,-0.00140104996632292,
0.00247428939345485));
#37237=CARTESIAN_POINT('Ctrl Pts',(-0.228003735975788,-0.00137069112187628,
0.00246735401736931));
#37238=CARTESIAN_POINT('Ctrl Pts',(-0.231104367476161,-0.0013403616690761,
0.00246039968961847));
#37239=CARTESIAN_POINT('Ctrl Pts',(-0.234204999187845,-0.00131005933689176,
0.00245342357850486));
#37240=CARTESIAN_POINT('Ctrl Pts',(-0.224903620487317,-0.00123313642614889,
0.00377581720335721));
#37241=CARTESIAN_POINT('Ctrl Pts',(-0.228004247058324,-0.00121832689931329,
0.00377611259775251));
#37242=CARTESIAN_POINT('Ctrl Pts',(-0.231104873711069,-0.00120353701330459,
0.00377640441621043));
#37243=CARTESIAN_POINT('Ctrl Pts',(-0.234205500449294,-0.00118876627184354,
0.00377669124621538));
#37244=CARTESIAN_POINT('Ctrl Pts',(-0.224904244452509,-0.000745411287960432,
0.00535508951527424));
#37245=CARTESIAN_POINT('Ctrl Pts',(-0.228004869369835,-0.000745883603517816,
0.00536654310520161));
#37246=CARTESIAN_POINT('Ctrl Pts',(-0.231105494301186,-0.000746375225293753,
0.00537799072107391));
#37247=CARTESIAN_POINT('Ctrl Pts',(-0.234206119249757,-0.000746885383007411,
0.00538943105918803));
#37248=CARTESIAN_POINT('Ctrl Pts',(-0.224904927022406,0.000243903830950042,
0.00708094602779947));
#37249=CARTESIAN_POINT('Ctrl Pts',(-0.22800555124417,0.000231747907332828,
0.00710847531073915));
#37250=CARTESIAN_POINT('Ctrl Pts',(-0.231106175424446,0.00021957829815924,
0.00713600296412369));
#37251=CARTESIAN_POINT('Ctrl Pts',(-0.234206799572117,0.000207395346249357,
0.0071635283576419));
#37252=CARTESIAN_POINT('Ctrl Pts',(-0.224905705882564,0.00204129536417242,
0.00904270545084878));
#37253=CARTESIAN_POINT('Ctrl Pts',(-0.228006331417495,0.00202251745037019,
0.00909153197079319));
#37254=CARTESIAN_POINT('Ctrl Pts',(-0.231106956906316,0.00200373108991613,
0.00914035807264341));
#37255=CARTESIAN_POINT('Ctrl Pts',(-0.234207582354303,0.00198493654309014,
0.00918918354252649));
#37256=CARTESIAN_POINT('Ctrl Pts',(-0.224906344934492,0.00503279669879239,
0.0106558220281949));
#37257=CARTESIAN_POINT('Ctrl Pts',(-0.228006973230644,0.00502108315461209,
0.0107253467403358));
#37258=CARTESIAN_POINT('Ctrl Pts',(-0.231107601524016,0.00500936667421796,
0.0107948715627757));
#37259=CARTESIAN_POINT('Ctrl Pts',(-0.234208229814862,0.00499764738343722,
0.0108643965065502));
#37260=CARTESIAN_POINT('Ctrl Pts',(-0.22490642148267,0.00911553811978304,
0.0108495997280891));
#37261=CARTESIAN_POINT('Ctrl Pts',(-0.22800705020616,0.00912342211753167,
0.0109217712057851));
#37262=CARTESIAN_POINT('Ctrl Pts',(-0.231107678935135,0.0091313080421625,
0.0109939426427322));
#37263=CARTESIAN_POINT('Ctrl Pts',(-0.234208307668951,0.00913919580236395,
0.0110661140483708));
#37264=CARTESIAN_POINT('Ctrl Pts',(-0.224905896781363,0.0122479140000228,
0.00952499840433065));
#37265=CARTESIAN_POINT('Ctrl Pts',(-0.228006522998932,0.0122659797356893,
0.00957977773742142));
#37266=CARTESIAN_POINT('Ctrl Pts',(-0.231107149178945,0.012284052220171,
0.00963455709198015));
#37267=CARTESIAN_POINT('Ctrl Pts',(-0.234207775325653,0.0123021312474762,
0.00968933635838273));
#37268=CARTESIAN_POINT('Ctrl Pts',(-0.224905188406661,0.0142245802852993,
0.00774097735435126));
#37269=CARTESIAN_POINT('Ctrl Pts',(-0.228005812932864,0.014239626038719,
0.0077754139801973));
#37270=CARTESIAN_POINT('Ctrl Pts',(-0.231106437412959,0.0142546840218181,
0.00780984919513146));
#37271=CARTESIAN_POINT('Ctrl Pts',(-0.234207061854539,0.014269753892948,
0.00784428248742507));
#37272=CARTESIAN_POINT('Ctrl Pts',(-0.224904545213284,0.0153743354777482,
0.00611286639462737));
#37273=CARTESIAN_POINT('Ctrl Pts',(-0.228005169501712,0.0153806533667306,
0.00613103086359291));
#37274=CARTESIAN_POINT('Ctrl Pts',(-0.231105793769188,0.0153869873403304,
0.0061491924949429));
#37275=CARTESIAN_POINT('Ctrl Pts',(-0.234206418024041,0.0153933369583363,
0.00616735039916125));
#37276=CARTESIAN_POINT('Ctrl Pts',(-0.224903937959543,0.0160047733300576,
0.00458381273421664));
#37277=CARTESIAN_POINT('Ctrl Pts',(-0.228004563851456,0.015997954017428,
0.00458944005855562));
#37278=CARTESIAN_POINT('Ctrl Pts',(-0.231105189799372,0.0159911559151915,
0.00459505994710943));
#37279=CARTESIAN_POINT('Ctrl Pts',(-0.234205815802617,0.0159843780961064,
0.00460067082154373));
#37280=CARTESIAN_POINT('Ctrl Pts',(-0.224903434945887,0.0163031426775171,
0.00330350985910996));
#37281=CARTESIAN_POINT('Ctrl Pts',(-0.228004062882068,0.0162828703806443,
0.0033012246620879));
#37282=CARTESIAN_POINT('Ctrl Pts',(-0.231104690946332,0.0162626198410551,
0.00329893259759974));
#37283=CARTESIAN_POINT('Ctrl Pts',(-0.23420531913388,0.0162423901793082,
0.00329663192843727));
#37284=CARTESIAN_POINT('Ctrl Pts',(-0.224903172488496,0.0163730847941923,
0.00265086132944247));
#37285=CARTESIAN_POINT('Ctrl Pts',(-0.22800380313163,0.0163447109764496,
0.00264488813827189));
#37286=CARTESIAN_POINT('Ctrl Pts',(-0.231104433996755,0.0163163649094739,
0.00263889889986091));
#37287=CARTESIAN_POINT('Ctrl Pts',(-0.234205065057425,0.0162880446461359,
0.00263289101445681));
#37288=CARTESIAN_POINT('Ctrl Pts',(-0.224903047769934,0.0163974953490442,
0.00232527569536224));
#37289=CARTESIAN_POINT('Ctrl Pts',(-0.228003678801843,0.0163652528946496,
0.00231821622721085));
#37290=CARTESIAN_POINT('Ctrl Pts',(-0.23110431006382,0.0163330357098684,
0.00231114482972889));
#37291=CARTESIAN_POINT('Ctrl Pts',(-0.234204941533998,0.0163008422866106,
0.00230405918705812));
#37292=CARTESIAN_POINT('',(-0.227006637251675,0.0126927900142701,-0.00906369458471356));
#37293=CARTESIAN_POINT('Ctrl Pts',(-0.227310930575325,0.0119192283365604,
-0.00956777733553797));
#37294=CARTESIAN_POINT('Ctrl Pts',(-0.227301909529503,0.0119391596141039,
-0.00955613795792144));
#37295=CARTESIAN_POINT('Ctrl Pts',(-0.227293027054935,0.0119591053495831,
-0.00954439308709731));
#37296=CARTESIAN_POINT('Ctrl Pts',(-0.227284273384487,0.0119790594444581,
-0.00953254512793306));
#37297=CARTESIAN_POINT('Ctrl Pts',(-0.227231597305896,0.012099135185951,
-0.00946124886063881));
#37298=CARTESIAN_POINT('Ctrl Pts',(-0.227183591614038,0.0122195086983642,
-0.0093862131580218));
#37299=CARTESIAN_POINT('Ctrl Pts',(-0.227138063814653,0.01233888863127,
-0.0093079134742992));
#37300=CARTESIAN_POINT('Ctrl Pts',(-0.227092536015269,0.0124582685641757,
-0.0092296137905766));
#37301=CARTESIAN_POINT('Ctrl Pts',(-0.227049486174156,0.0125766585785184,
-0.00914804828974315));
#37302=CARTESIAN_POINT('Ctrl Pts',(-0.227006637251675,0.0126927900142701,
-0.00906369458471356));
#37303=CARTESIAN_POINT('',(-0.22626372592396,0.0126609459515122,-0.00907137389400092));
#37304=CARTESIAN_POINT('Ctrl Pts',(-0.226263728585857,0.0126609457742137,
-0.00907137404226376));
#37305=CARTESIAN_POINT('Ctrl Pts',(-0.226386619259017,0.0126771073815086,
-0.00906231630609566));
#37306=CARTESIAN_POINT('Ctrl Pts',(-0.226510405436089,0.0126878531263563,
-0.0090570429094382));
#37307=CARTESIAN_POINT('Ctrl Pts',(-0.226758531947056,0.0126985222461932,
-0.00905426871011949));
#37308=CARTESIAN_POINT('Ctrl Pts',(-0.226882687732036,0.0126984539951922,
-0.00905675848878095));
#37309=CARTESIAN_POINT('Ctrl Pts',(-0.227006496256814,0.012692991252369,
-0.00906311899234723));
#37310=CARTESIAN_POINT('',(-0.226391100213263,0.0131362729035505,-0.00871148491867768));
#37311=CARTESIAN_POINT('Origin',(-0.227688300131171,0.00723376617371606,
-0.00189119032934214));
#37312=CARTESIAN_POINT('',(-0.225391419217308,0.0131367695109091,-0.00869218205150295));
#37313=CARTESIAN_POINT('Ctrl Pts',(-0.226391100213325,0.0131362728985425,
-0.00871148491535396));
#37314=CARTESIAN_POINT('Ctrl Pts',(-0.226224497789347,0.0131363544611319,
-0.00870826654206384));
#37315=CARTESIAN_POINT('Ctrl Pts',(-0.226057895192789,0.013136436623428,
-0.00870504888489742));
#37316=CARTESIAN_POINT('Ctrl Pts',(-0.225724668190818,0.013136602159935,
-0.00869861459466251));
#37317=CARTESIAN_POINT('Ctrl Pts',(-0.225558043667431,0.0131366855343623,
-0.00869539795950626));
#37318=CARTESIAN_POINT('Ctrl Pts',(-0.225391419217304,0.0131367695104093,
-0.00869218205167778));
#37319=CARTESIAN_POINT('',(-0.225267117543399,0.0126690414880847,-0.00904616167166099));
#37320=CARTESIAN_POINT('Origin',(-0.226746990060653,0.00723483562453479,
-0.00187833795146874));
#37321=CARTESIAN_POINT('',(-0.224973343469933,0.0127081065850716,-0.00901241391075122));
#37322=CARTESIAN_POINT('Ctrl Pts',(-0.224972872689331,0.0127080240555426,
-0.00901235812756441));
#37323=CARTESIAN_POINT('Ctrl Pts',(-0.225023054977778,0.0127112197679192,
-0.0090110474151989));
#37324=CARTESIAN_POINT('Ctrl Pts',(-0.2250734691889,0.012709520923146,-0.00901326014049183));
#37325=CARTESIAN_POINT('Ctrl Pts',(-0.225172251825652,0.0126964311153787,
-0.00902458937587981));
#37326=CARTESIAN_POINT('Ctrl Pts',(-0.225220266854037,0.0126851548120693,
-0.00903361573608797));
#37327=CARTESIAN_POINT('Ctrl Pts',(-0.225266060957984,0.0126693218437064,
-0.00904576810780379));
#37328=CARTESIAN_POINT('Ctrl Pts',(-0.225105867141788,0.0119077821064707,
-0.00952780373316783));
#37329=CARTESIAN_POINT('Ctrl Pts',(-0.225095444062685,0.0120459270894792,
-0.00944903969813657));
#37330=CARTESIAN_POINT('Ctrl Pts',(-0.225079187043228,0.0121814942140962,
-0.00936678104310605));
#37331=CARTESIAN_POINT('Ctrl Pts',(-0.225034785732628,0.012448678452175,
-0.00919471546264362));
#37332=CARTESIAN_POINT('Ctrl Pts',(-0.225006520539429,0.0125799968801818,
-0.00910496411764648));
#37333=CARTESIAN_POINT('Ctrl Pts',(-0.224972407900901,0.0127079109487015,
-0.0090124302414561));
#37334=CARTESIAN_POINT('Origin',(-0.203568281266003,0.00750000064956461,
-0.000977039010395701));
#37335=CARTESIAN_POINT('',(-0.203180932155927,0.0122574475529592,-0.00887884679402051));
#37336=CARTESIAN_POINT('',(-0.203099975589327,0.00748772692520692,-0.0102016315939729));
#37337=CARTESIAN_POINT('Ctrl Pts',(-0.203180932155927,0.0122574475529592,
-0.00887884679402051));
#37338=CARTESIAN_POINT('Ctrl Pts',(-0.203144389557098,0.0120211460710307,
-0.00902023995050872));
#37339=CARTESIAN_POINT('Ctrl Pts',(-0.203099004528403,0.0117059840990509,
-0.00918853528176113));
#37340=CARTESIAN_POINT('Ctrl Pts',(-0.203054201982351,0.0113485760860837,
-0.00935714677214135));
#37341=CARTESIAN_POINT('Ctrl Pts',(-0.203033800001085,0.0111722119519007,
-0.00943586125013318));
#37342=CARTESIAN_POINT('Ctrl Pts',(-0.203004790952906,0.0108566700800293,
-0.00956601535400645));
#37343=CARTESIAN_POINT('Ctrl Pts',(-0.202980217443486,0.010477728951912,
-0.00970594622761543));
#37344=CARTESIAN_POINT('Ctrl Pts',(-0.202964642390056,0.00996004413167459,
-0.0098682196553169));
#37345=CARTESIAN_POINT('Ctrl Pts',(-0.202970397699778,0.00949324515176631,
-0.00998162264848546));
#37346=CARTESIAN_POINT('Ctrl Pts',(-0.202983931631907,0.00912176212646602,
-0.0100529635069714));
#37347=CARTESIAN_POINT('Ctrl Pts',(-0.20299393266481,0.00891420132184156,
-0.0100873844335844));
#37348=CARTESIAN_POINT('Ctrl Pts',(-0.203004460841773,0.00872918961470634,
-0.0101141562984169));
#37349=CARTESIAN_POINT('Ctrl Pts',(-0.203010134685348,0.00864074678625943,
-0.0101255182078198));
#37350=CARTESIAN_POINT('Ctrl Pts',(-0.203021726690619,0.00846795517814871,
-0.0101463016488843));
#37351=CARTESIAN_POINT('Ctrl Pts',(-0.203045893326094,0.00813922185990422,
-0.01017849081334));
#37352=CARTESIAN_POINT('Ctrl Pts',(-0.203075503013031,0.00777516939207381,
-0.0101975550358818));
#37353=CARTESIAN_POINT('Ctrl Pts',(-0.203099132557942,0.00750037293252254,
-0.0101980787679676));
#37354=CARTESIAN_POINT('',(-0.203173200311358,0.00274689768564807,-0.008881289974441));
#37355=CARTESIAN_POINT('Ctrl Pts',(-0.203103782510698,0.00748459366645466,
-0.0101981667986033));
#37356=CARTESIAN_POINT('Ctrl Pts',(-0.203056815772698,0.00710265220262713,
-0.0101965099598228));
#37357=CARTESIAN_POINT('Ctrl Pts',(-0.203021349803096,0.0067170805498119,
-0.0101713884403401));
#37358=CARTESIAN_POINT('Ctrl Pts',(-0.202934394875737,0.00526489448036165,
-0.00998387785797495));
#37359=CARTESIAN_POINT('Ctrl Pts',(-0.202965303386757,0.00422151948414504,
-0.0096619097669541));
#37360=CARTESIAN_POINT('Ctrl Pts',(-0.203118124523932,0.00308108700338837,
-0.0090738493251725));
#37361=CARTESIAN_POINT('Ctrl Pts',(-0.203144125164855,0.00291254238670889,
-0.00898020598093925));
#37362=CARTESIAN_POINT('Ctrl Pts',(-0.203173200310812,0.00274689768556089,
-0.00888128997442626));
#37363=CARTESIAN_POINT('',(-0.204179808594537,0.00274695694953536,-0.00890316850546251));
#37364=CARTESIAN_POINT('Ctrl Pts',(-0.203173200311351,0.00274689768609342,
-0.00888128997475801));
#37365=CARTESIAN_POINT('Ctrl Pts',(-0.203511887957009,0.00274691735937696,
-0.00888865115679395));
#37366=CARTESIAN_POINT('Ctrl Pts',(-0.2038476742076,0.00274693265699481,
-0.00889594675021198));
#37367=CARTESIAN_POINT('Ctrl Pts',(-0.204179864222553,0.00274694378498237,
-0.00890316180123792));
#37368=CARTESIAN_POINT('',(-0.204098753207029,0.00750019449511319,-0.010219767218868));
#37369=CARTESIAN_POINT('Ctrl Pts',(-0.204179808594537,0.00274695694953536,
-0.00890316850546251));
#37370=CARTESIAN_POINT('Ctrl Pts',(-0.204143308707588,0.00298395730820233,
-0.0090448031502624));
#37371=CARTESIAN_POINT('Ctrl Pts',(-0.204097954903568,0.00330018647005424,
-0.00921338606909646));
#37372=CARTESIAN_POINT('Ctrl Pts',(-0.204053158933222,0.00365864570901938,
-0.00938214415921903));
#37373=CARTESIAN_POINT('Ctrl Pts',(-0.204032678472951,0.00383632055569296,
-0.00946122584533509));
#37374=CARTESIAN_POINT('Ctrl Pts',(-0.204003768789267,0.00415082622990258,
-0.00959060202023825));
#37375=CARTESIAN_POINT('Ctrl Pts',(-0.203979179919398,0.00452842436729695,
-0.00972964246551787));
#37376=CARTESIAN_POINT('Ctrl Pts',(-0.203963454897067,0.00503954981670578,
-0.00988970685319689));
#37377=CARTESIAN_POINT('Ctrl Pts',(-0.203968942557704,0.00550841835918545,
-0.0100036492041412));
#37378=CARTESIAN_POINT('Ctrl Pts',(-0.203982363369764,0.00587797498451415,
-0.0100745671040912));
#37379=CARTESIAN_POINT('Ctrl Pts',(-0.20399231704185,0.00608447450262321,
-0.0101088319704821));
#37380=CARTESIAN_POINT('Ctrl Pts',(-0.204002786998696,0.00626792725225948,
-0.0101354241310119));
#37381=CARTESIAN_POINT('Ctrl Pts',(-0.204008516600288,0.00635676412948642,
-0.0101468715278863));
#37382=CARTESIAN_POINT('Ctrl Pts',(-0.204020200606318,0.00652958263497338,
-0.0101677050009321));
#37383=CARTESIAN_POINT('Ctrl Pts',(-0.204044661227922,0.00685904773966244,
-0.0102000610115712));
#37384=CARTESIAN_POINT('Ctrl Pts',(-0.20407472551262,0.00722428924687252,
-0.0102192517952231));
#37385=CARTESIAN_POINT('Ctrl Pts',(-0.204098753205607,0.00750019441693834,
-0.0102197672188388));
#37386=CARTESIAN_POINT('',(-0.204181212510367,0.0122570585516106,-0.00890078076054459));
#37387=CARTESIAN_POINT('Ctrl Pts',(-0.204098753207029,0.00750019449511319,
-0.010219767218868));
#37388=CARTESIAN_POINT('Ctrl Pts',(-0.204074969826491,0.00777525417200037,
-0.010219245316851));
#37389=CARTESIAN_POINT('Ctrl Pts',(-0.20404518935886,0.00813953722805785,
-0.0102001521705759));
#37390=CARTESIAN_POINT('Ctrl Pts',(-0.204020924281112,0.00846830075501304,
-0.0101679429006501));
#37391=CARTESIAN_POINT('Ctrl Pts',(-0.204009307531493,0.00864098654128726,
-0.0101471667925929));
#37392=CARTESIAN_POINT('Ctrl Pts',(-0.204003623011863,0.00872944215982944,
-0.0101357983481098));
#37393=CARTESIAN_POINT('Ctrl Pts',(-0.203993124102833,0.00891393094068779,
-0.0101091022096258));
#37394=CARTESIAN_POINT('Ctrl Pts',(-0.203983158153701,0.00912121165876486,
-0.010074736990353));
#37395=CARTESIAN_POINT('Ctrl Pts',(-0.203969711708032,0.00949232807053968,
-0.0100035209917527));
#37396=CARTESIAN_POINT('Ctrl Pts',(-0.203964148109392,0.00996155782354372,
-0.00988948548415189));
#37397=CARTESIAN_POINT('Ctrl Pts',(-0.203979984609945,0.0104768772720125,
-0.00972790469770468));
#37398=CARTESIAN_POINT('Ctrl Pts',(-0.204004794840732,0.0108561848221544,
-0.00958791591559206));
#37399=CARTESIAN_POINT('Ctrl Pts',(-0.204034076180802,0.0111727868553702,
-0.00945731833040206));
#37400=CARTESIAN_POINT('Ctrl Pts',(-0.204054512850181,0.0113489102407224,
-0.00937869140214235));
#37401=CARTESIAN_POINT('Ctrl Pts',(-0.204099372796569,0.0117062274665102,
-0.00921011084626496));
#37402=CARTESIAN_POINT('Ctrl Pts',(-0.204144720651052,0.0120210387403513,
-0.009041989911057));
#37403=CARTESIAN_POINT('Ctrl Pts',(-0.204181212510367,0.0122570585516106,
-0.00890078076054459));
#37404=CARTESIAN_POINT('Ctrl Pts',(-0.204181268812703,0.012257066354676,
-0.00890077728725559));
#37405=CARTESIAN_POINT('Ctrl Pts',(-0.203847894597336,0.0122571900460014,
-0.00889347070490962));
#37406=CARTESIAN_POINT('Ctrl Pts',(-0.203514406607199,0.0122573177004729,
-0.00888615926607952));
#37407=CARTESIAN_POINT('Ctrl Pts',(-0.203181012549154,0.0122574492374588,
-0.00887884752447026));
#37408=CARTESIAN_POINT('Origin',(-0.205569668377583,0.00750000053546121,
-0.00105476362107362));
#37409=CARTESIAN_POINT('',(-0.205181486251685,0.0122552975429564,-0.00891989779273504));
#37410=CARTESIAN_POINT('',(-0.205098440188702,0.00750015102883512,-0.0102432543024386));
#37411=CARTESIAN_POINT('Ctrl Pts',(-0.205181486251685,0.0122552975429564,
-0.00891989779273504));
#37412=CARTESIAN_POINT('Ctrl Pts',(-0.205145010746124,0.0120195671299043,
-0.00906154417007191));
#37413=CARTESIAN_POINT('Ctrl Pts',(-0.205099665823808,0.0117050967237337,
-0.00923018880615341));
#37414=CARTESIAN_POINT('Ctrl Pts',(-0.20505473701453,0.0113479801935507,
-0.00939935025380538));
#37415=CARTESIAN_POINT('Ctrl Pts',(-0.205034268942562,0.0111721994041601,
-0.00947814554233864));
#37416=CARTESIAN_POINT('Ctrl Pts',(-0.205004748571038,0.0108549239719047,
-0.00960952696160696));
#37417=CARTESIAN_POINT('Ctrl Pts',(-0.204979722424145,0.010475498663842,
-0.00975002068728981));
#37418=CARTESIAN_POINT('Ctrl Pts',(-0.20496362799297,0.00996219476279488,
-0.00991159079101826));
#37419=CARTESIAN_POINT('Ctrl Pts',(-0.204969004055025,0.00949117200399576,
-0.0100264939808952));
#37420=CARTESIAN_POINT('Ctrl Pts',(-0.204982377945537,0.009120408049961,
-0.010097842256249));
#37421=CARTESIAN_POINT('Ctrl Pts',(-0.204992318932816,0.0089133766789427,
-0.0101322743370575));
#37422=CARTESIAN_POINT('Ctrl Pts',(-0.205002800013507,0.00872932653396566,
-0.0101589956283636));
#37423=CARTESIAN_POINT('Ctrl Pts',(-0.205008498844975,0.00864085623694867,
-0.0101704072675598));
#37424=CARTESIAN_POINT('Ctrl Pts',(-0.205020148419491,0.00846828167738281,
-0.0101912420545331));
#37425=CARTESIAN_POINT('Ctrl Pts',(-0.205044525931656,0.00813958304043702,
-0.0102235622044265));
#37426=CARTESIAN_POINT('Ctrl Pts',(-0.205074491969353,0.00777527627334546,
-0.010242729856909));
#37427=CARTESIAN_POINT('Ctrl Pts',(-0.205098440307258,0.00750015170665339,
-0.0102432543053281));
#37428=CARTESIAN_POINT('',(-0.205180409732413,0.00274852659771838,-0.00892218213689432));
#37429=CARTESIAN_POINT('Ctrl Pts',(-0.205098440247425,0.00750015102368582,
-0.0102432543040401));
#37430=CARTESIAN_POINT('Ctrl Pts',(-0.205093952951413,0.00744893039446262,
-0.0102431577065131));
#37431=CARTESIAN_POINT('Ctrl Pts',(-0.205080198588494,0.00729028603855544,
-0.0102413201101437));
#37432=CARTESIAN_POINT('Ctrl Pts',(-0.205060248277069,0.00705318842883126,
-0.0102327637584102));
#37433=CARTESIAN_POINT('Ctrl Pts',(-0.205037071982337,0.00676558988861412,
-0.0102143707027614));
#37434=CARTESIAN_POINT('Ctrl Pts',(-0.205019741813002,0.00653305075314794,
-0.01019134977702));
#37435=CARTESIAN_POINT('Ctrl Pts',(-0.205008015508058,0.00636038697474645,
-0.0101705570943968));
#37436=CARTESIAN_POINT('Ctrl Pts',(-0.205002287358874,0.00627190834821762,
-0.0101591465651645));
#37437=CARTESIAN_POINT('Ctrl Pts',(-0.204991791760696,0.00608850277435127,
-0.0101325524012929));
#37438=CARTESIAN_POINT('Ctrl Pts',(-0.204981832022474,0.00588182305608673,
-0.0100982193342052));
#37439=CARTESIAN_POINT('Ctrl Pts',(-0.204968413283859,0.00551192613026262,
-0.0100272159798676));
#37440=CARTESIAN_POINT('Ctrl Pts',(-0.204963297415599,0.00503789180459126,
-0.00991130245284762));
#37441=CARTESIAN_POINT('Ctrl Pts',(-0.204978689645553,0.00453288307852895,
-0.00975337405009284));
#37442=CARTESIAN_POINT('Ctrl Pts',(-0.205001886359724,0.00418947678318943,
-0.00962547804925551));
#37443=CARTESIAN_POINT('Ctrl Pts',(-0.205017689619932,0.00400142298949485,
-0.00955045506899675));
#37444=CARTESIAN_POINT('Ctrl Pts',(-0.205033338680103,0.00384193801459521,
-0.00948318984329787));
#37445=CARTESIAN_POINT('Ctrl Pts',(-0.205042517205282,0.00375845349593796,
-0.00944652183840551));
#37446=CARTESIAN_POINT('Ctrl Pts',(-0.205060590791516,0.00360208362519979,
-0.00937617788322102));
#37447=CARTESIAN_POINT('Ctrl Pts',(-0.205098306119765,0.00330504246940279,
-0.00923472043191907));
#37448=CARTESIAN_POINT('Ctrl Pts',(-0.205144087161525,0.00298418033850801,
-0.00906362922856368));
#37449=CARTESIAN_POINT('Ctrl Pts',(-0.205180409732413,0.00274852659771838,
-0.00892218213689432));
#37450=CARTESIAN_POINT('',(-0.206180961328082,0.00274847806016448,-0.00894387894537355));
#37451=CARTESIAN_POINT('Ctrl Pts',(-0.205180479464195,0.00274853066302267,
-0.00892218610479268));
#37452=CARTESIAN_POINT('Ctrl Pts',(-0.205511119540387,0.00274851289143719,
-0.00892935493901173));
#37453=CARTESIAN_POINT('Ctrl Pts',(-0.205844838618331,0.00274849107317641,
-0.00893658818851419));
#37454=CARTESIAN_POINT('Ctrl Pts',(-0.206181011406301,0.00274846505131942,
-0.00894387218078926));
#37455=CARTESIAN_POINT('',(-0.206098160870363,0.00750010608734745,-0.010264959897942));
#37456=CARTESIAN_POINT('Ctrl Pts',(-0.206180961328082,0.00274847806016448,
-0.00894387894537355));
#37457=CARTESIAN_POINT('Ctrl Pts',(-0.206144503244658,0.0029851394815468,
-0.00908593313274618));
#37458=CARTESIAN_POINT('Ctrl Pts',(-0.206099163905087,0.00330094991332194,
-0.00925502338592517));
#37459=CARTESIAN_POINT('Ctrl Pts',(-0.206054223946957,0.00365935700615154,
-0.00942444106050021));
#37460=CARTESIAN_POINT('Ctrl Pts',(-0.206033685907648,0.00383642966844798,
-0.00950359601200414));
#37461=CARTESIAN_POINT('Ctrl Pts',(-0.206004239839081,0.00415297153187771,
-0.00963430969563866));
#37462=CARTESIAN_POINT('Ctrl Pts',(-0.20597916333659,0.00453120900848722,
-0.00977393705103434));
#37463=CARTESIAN_POINT('Ctrl Pts',(-0.20596285353138,0.0050377641666255,
-0.00993320305773024));
#37464=CARTESIAN_POINT('Ctrl Pts',(-0.205967863395825,0.00551099034506471,
-0.0100486504485952));
#37465=CARTESIAN_POINT('Ctrl Pts',(-0.205981049669001,0.00587956688186075,
-0.0101195069636298));
#37466=CARTESIAN_POINT('Ctrl Pts',(-0.205990901558899,0.00608537450600959,
-0.0101537508288514));
#37467=CARTESIAN_POINT('Ctrl Pts',(-0.206001282208726,0.00626761766659463,
-0.0101802563825301));
#37468=CARTESIAN_POINT('Ctrl Pts',(-0.206007030871337,0.00635656589256591,
-0.0101917668973418));
#37469=CARTESIAN_POINT('Ctrl Pts',(-0.206018754543683,0.006529146193304,
-0.0102126501798417));
#37470=CARTESIAN_POINT('Ctrl Pts',(-0.20604340588525,0.00685855965021963,
-0.0102451399879971));
#37471=CARTESIAN_POINT('Ctrl Pts',(-0.206073816600126,0.00722395965705849,
-0.0102644346030527));
#37472=CARTESIAN_POINT('Ctrl Pts',(-0.206098160870452,0.00750010608733958,
-0.0102649598979439));
#37473=CARTESIAN_POINT('',(-0.206181715574144,0.0122551196169534,-0.00894171946680973));
#37474=CARTESIAN_POINT('Ctrl Pts',(-0.206098160870363,0.00750010608734745,
-0.010264959897942));
#37475=CARTESIAN_POINT('Ctrl Pts',(-0.206074054827856,0.00777528552125095,
-0.0102644332675757));
#37476=CARTESIAN_POINT('Ctrl Pts',(-0.206043911255022,0.00813957901293385,
-0.0102452587525356));
#37477=CARTESIAN_POINT('Ctrl Pts',(-0.206019426951112,0.00846815073558031,
-0.0102129497512625));
#37478=CARTESIAN_POINT('Ctrl Pts',(-0.206007747489499,0.0086405593599698,
-0.0101921395316813));
#37479=CARTESIAN_POINT('Ctrl Pts',(-0.206002034855823,0.0087290293396645,
-0.0101807278839575));
#37480=CARTESIAN_POINT('Ctrl Pts',(-0.205991576991469,0.00891250482133831,
-0.0101541029899592));
#37481=CARTESIAN_POINT('Ctrl Pts',(-0.205981666019672,0.00911922871637835,
-0.0101197394207395));
#37482=CARTESIAN_POINT('Ctrl Pts',(-0.20596833683428,0.0094893100438307,
-0.0100486653436722));
#37483=CARTESIAN_POINT('Ctrl Pts',(-0.205963343815955,0.0099645263554711,
-0.00993235088092946));
#37484=CARTESIAN_POINT('Ctrl Pts',(-0.205978910244621,0.0104689773112782,
-0.00977445835237511));
#37485=CARTESIAN_POINT('Ctrl Pts',(-0.206002303757198,0.0108128077782491,
-0.00964632045704586));
#37486=CARTESIAN_POINT('Ctrl Pts',(-0.206018229482252,0.0110011334046898,
-0.00957112831725541));
#37487=CARTESIAN_POINT('Ctrl Pts',(-0.206033997054145,0.0111609344223277,
-0.00950367117882155));
#37488=CARTESIAN_POINT('Ctrl Pts',(-0.206043234920356,0.0112445506318481,
-0.00946691067775824));
#37489=CARTESIAN_POINT('Ctrl Pts',(-0.206061414877685,0.0114011476494823,
-0.00939639690988238));
#37490=CARTESIAN_POINT('Ctrl Pts',(-0.206099313687172,0.0116984707478102,
-0.00925466076457502));
#37491=CARTESIAN_POINT('Ctrl Pts',(-0.206145270450179,0.0120194511993669,
-0.00908332193822784));
#37492=CARTESIAN_POINT('Ctrl Pts',(-0.206181715574144,0.0122551196169534,
-0.00894171946680973));
#37493=CARTESIAN_POINT('Ctrl Pts',(-0.206181766675709,0.0122551273964408,
-0.00894171587571898));
#37494=CARTESIAN_POINT('Ctrl Pts',(-0.205849139539492,0.0122551803210089,
-0.0089344628329478));
#37495=CARTESIAN_POINT('Ctrl Pts',(-0.205515630029343,0.0122552371745374,
-0.00892718825993729));
#37496=CARTESIAN_POINT('Ctrl Pts',(-0.205181559737592,0.0122552979498864,
-0.0089198991421701));
#37497=CARTESIAN_POINT('Origin',(-0.207569531999201,0.00750000042399001,
-0.0011316682782873));
#37498=CARTESIAN_POINT('',(-0.207182021343611,0.0122531890606491,-0.00896101780551548));
#37499=CARTESIAN_POINT('',(-0.207097778441897,0.00750000135331723,-0.0102884291114441));
#37500=CARTESIAN_POINT('Ctrl Pts',(-0.207182021343611,0.0122531890606491,
-0.00896101780551548));
#37501=CARTESIAN_POINT('Ctrl Pts',(-0.207145589529982,0.012017810159708,
-0.00910303844719066));
#37502=CARTESIAN_POINT('Ctrl Pts',(-0.207114946631626,0.0118040522654641,
-0.00921766339889173));
#37503=CARTESIAN_POINT('Ctrl Pts',(-0.207090279354578,0.0116196010293119,
-0.00930996556537863));
#37504=CARTESIAN_POINT('Ctrl Pts',(-0.207077945716054,0.0115273754112358,
-0.00935611664862208));
#37505=CARTESIAN_POINT('Ctrl Pts',(-0.207067105565684,0.0114424881905947,
-0.00939670623860649));
#37506=CARTESIAN_POINT('Ctrl Pts',(-0.207057415290073,0.0113620447273888,
-0.00943388414297075));
#37507=CARTESIAN_POINT('Ctrl Pts',(-0.207052570152267,0.0113218229957858,
-0.00945247309515288));
#37508=CARTESIAN_POINT('Ctrl Pts',(-0.207048013105317,0.0112826983783498,
-0.00947018048739905));
#37509=CARTESIAN_POINT('Ctrl Pts',(-0.20704419346178,0.0112492058999985,
-0.00948511621392071));
#37510=CARTESIAN_POINT('Ctrl Pts',(-0.207040373818242,0.0112157134216472,
-0.00950005194044236));
#37511=CARTESIAN_POINT('Ctrl Pts',(-0.207037289600169,0.0111878944163724,
-0.00951230704660541));
#37512=CARTESIAN_POINT('Ctrl Pts',(-0.207033098186437,0.0111473183720926,
-0.00952982204190615));
#37513=CARTESIAN_POINT('Ctrl Pts',(-0.207028906772705,0.0111067423278128,
-0.00954733703720688));
#37514=CARTESIAN_POINT('Ctrl Pts',(-0.207023611716941,0.0110533378977748,
-0.00956994834796696));
#37515=CARTESIAN_POINT('Ctrl Pts',(-0.207018960141398,0.0110030579020677,
-0.00959064979089299));
#37516=CARTESIAN_POINT('Ctrl Pts',(-0.207014308565855,0.0109527779063606,
-0.00961135123381902));
#37517=CARTESIAN_POINT('Ctrl Pts',(-0.20701029799187,0.0109056687548309,
-0.00963025690129191));
#37518=CARTESIAN_POINT('Ctrl Pts',(-0.207006500480265,0.0108578827174683,
-0.00964899548438834));
#37519=CARTESIAN_POINT('Ctrl Pts',(-0.206998905457053,0.0107623106427431,
-0.00968647265058121));
#37520=CARTESIAN_POINT('Ctrl Pts',(-0.206992165145035,0.0106639906501456,
-0.00972316816953493));
#37521=CARTESIAN_POINT('Ctrl Pts',(-0.206986617295028,0.0105649667408118,
-0.0097581953819392));
#37522=CARTESIAN_POINT('Ctrl Pts',(-0.206975521595013,0.0103669189221444,
-0.00982824980674773));
#37523=CARTESIAN_POINT('Ctrl Pts',(-0.20696919711927,0.0101660098746444,
-0.00989156765480013));
#37524=CARTESIAN_POINT('Ctrl Pts',(-0.206967001402819,0.0099701265364059,
-0.00994635646975916));
#37525=CARTESIAN_POINT('Ctrl Pts',(-0.206964805686368,0.00977424319816743,
-0.0100011452847182));
#37526=CARTESIAN_POINT('Ctrl Pts',(-0.206966726116684,0.00958356196070715,
-0.0100479856097936));
#37527=CARTESIAN_POINT('Ctrl Pts',(-0.206972407397417,0.00937916938864513,
-0.0100909377062068));
#37528=CARTESIAN_POINT('Ctrl Pts',(-0.206975248037783,0.00927697310261412,
-0.0101124137544134));
#37529=CARTESIAN_POINT('Ctrl Pts',(-0.206979032483084,0.0091713144408141,
-0.0101327523961511));
#37530=CARTESIAN_POINT('Ctrl Pts',(-0.206983588109306,0.0090672379345247,
-0.0101509193285515));
#37531=CARTESIAN_POINT('Ctrl Pts',(-0.206985865922417,0.00901519968138,
-0.0101600027947517));
#37532=CARTESIAN_POINT('Ctrl Pts',(-0.206988335561166,0.00896356508380256,
-0.0101685879622218));
#37533=CARTESIAN_POINT('Ctrl Pts',(-0.206991307138919,0.00890723708154231,
-0.0101774073832468));
#37534=CARTESIAN_POINT('Ctrl Pts',(-0.206994278716672,0.00885090907928206,
-0.0101862268042718));
#37535=CARTESIAN_POINT('Ctrl Pts',(-0.20699775554717,0.00878986325834849,
-0.0101951279537617));
#37536=CARTESIAN_POINT('Ctrl Pts',(-0.207000448895413,0.00874458601643362,
-0.0102013940653026));
#37537=CARTESIAN_POINT('Ctrl Pts',(-0.207003142243657,0.00869930877451875,
-0.0102076601768436));
#37538=CARTESIAN_POINT('Ctrl Pts',(-0.207005047495907,0.00866982864377494,
-0.0102115036111103));
#37539=CARTESIAN_POINT('Ctrl Pts',(-0.207007461526474,0.00863355577397413,
-0.0102160782502125));
#37540=CARTESIAN_POINT('Ctrl Pts',(-0.207009875557042,0.00859728290417331,
-0.0102206528893147));
#37541=CARTESIAN_POINT('Ctrl Pts',(-0.20701280082912,0.00855420375341624,
-0.0102258453580294));
#37542=CARTESIAN_POINT('Ctrl Pts',(-0.207015921463241,0.0085098402872069,
-0.0102308325011764));
#37543=CARTESIAN_POINT('Ctrl Pts',(-0.207022162731483,0.00842111335478822,
-0.0102408067874703));
#37544=CARTESIAN_POINT('Ctrl Pts',(-0.207029182339711,0.00832726285498634,
-0.0102501028339772));
#37545=CARTESIAN_POINT('Ctrl Pts',(-0.207037228948747,0.00822421591382894,
-0.0102584479867199));
#37546=CARTESIAN_POINT('Ctrl Pts',(-0.20705332216682,0.00801812203151415,
-0.0102751382922053));
#37547=CARTESIAN_POINT('Ctrl Pts',(-0.207073526056755,0.00777524126012205,
-0.0102879021939248));
#37548=CARTESIAN_POINT('Ctrl Pts',(-0.207097778441897,0.00750000135331723,
-0.0102884291114441));
#37549=CARTESIAN_POINT('',(-0.207181532792705,0.00275005700218644,-0.0089629743514168));
#37550=CARTESIAN_POINT('Ctrl Pts',(-0.207097778313067,0.00749999989891767,
-0.010288429108645));
#37551=CARTESIAN_POINT('Ctrl Pts',(-0.207073419625904,0.00722500789874744,
-0.0102878998379192));
#37552=CARTESIAN_POINT('Ctrl Pts',(-0.207042990834877,0.006861018988083,
-0.0102686874301281));
#37553=CARTESIAN_POINT('Ctrl Pts',(-0.207018331514006,0.00653274297319404,
-0.0102363194044195));
#37554=CARTESIAN_POINT('Ctrl Pts',(-0.207006602442421,0.00636060530882933,
-0.0102154904597151));
#37555=CARTESIAN_POINT('Ctrl Pts',(-0.207000862677054,0.00627205965399394,
-0.0102040358443934));
#37556=CARTESIAN_POINT('Ctrl Pts',(-0.206990449366781,0.00608957659382692,
-0.0101774937656562));
#37557=CARTESIAN_POINT('Ctrl Pts',(-0.206980590513266,0.0058834710399858,
-0.0101431671415748));
#37558=CARTESIAN_POINT('Ctrl Pts',(-0.206967394593663,0.00551434385411936,
-0.0100721886506396));
#37559=CARTESIAN_POINT('Ctrl Pts',(-0.206962734755496,0.00503619279538927,
-0.00995481286789569));
#37560=CARTESIAN_POINT('Ctrl Pts',(-0.20697864418332,0.00453579661021954,
-0.00979775023715801));
#37561=CARTESIAN_POINT('Ctrl Pts',(-0.207002283619446,0.00419160943361069,
-0.00966922538535609));
#37562=CARTESIAN_POINT('Ctrl Pts',(-0.207018336605471,0.00400301457636903,
-0.00959373456705133));
#37563=CARTESIAN_POINT('Ctrl Pts',(-0.207034242024311,0.0038424762579756,
-0.00952577398159521));
#37564=CARTESIAN_POINT('Ctrl Pts',(-0.20704345921084,0.00375923635338582,
-0.00948906520200336));
#37565=CARTESIAN_POINT('Ctrl Pts',(-0.207061638331585,0.00360277318013875,
-0.00941840556840703));
#37566=CARTESIAN_POINT('Ctrl Pts',(-0.207099453178564,0.0033059120017622,
-0.00927646000782889));
#37567=CARTESIAN_POINT('Ctrl Pts',(-0.207145244487981,0.00298536163401571,
-0.00910481968417944));
#37568=CARTESIAN_POINT('Ctrl Pts',(-0.207181532792705,0.00275005700218644,
-0.0089629743514168));
#37569=CARTESIAN_POINT('',(-0.208182049566434,0.00275001859964783,-0.00898469078812813));
#37570=CARTESIAN_POINT('Ctrl Pts',(-0.207181595750663,0.00275006108290852,
-0.00896297819299416));
#37571=CARTESIAN_POINT('Ctrl Pts',(-0.207511950573292,0.00275004656769739,
-0.00897014750465242));
#37572=CARTESIAN_POINT('Ctrl Pts',(-0.207845671547403,0.00275002816037635,
-0.00897738759838072));
#37573=CARTESIAN_POINT('Ctrl Pts',(-0.208182094596618,0.0027500056881023,
-0.00898468393992406));
#37574=CARTESIAN_POINT('',(-0.208097512100336,0.00749999999333244,-0.0103101497453589));
#37575=CARTESIAN_POINT('Ctrl Pts',(-0.208182049566434,0.00275001859964783,
-0.00898469078812813));
#37576=CARTESIAN_POINT('Ctrl Pts',(-0.208145638937197,0.00298627876255052,
-0.00912711411657463));
#37577=CARTESIAN_POINT('Ctrl Pts',(-0.208099688434819,0.00330817190051734,
-0.0092993952508412));
#37578=CARTESIAN_POINT('Ctrl Pts',(-0.208061716122496,0.00360646955884461,
-0.00944187715419658));
#37579=CARTESIAN_POINT('Ctrl Pts',(-0.208043467883132,0.00376356938216498,
-0.00951273322332168));
#37580=CARTESIAN_POINT('Ctrl Pts',(-0.208034173093545,0.00384757541839402,
-0.00954971832383919));
#37581=CARTESIAN_POINT('Ctrl Pts',(-0.208018311977663,0.00400760211155766,
-0.00961734982946915));
#37582=CARTESIAN_POINT('Ctrl Pts',(-0.208002254883357,0.00419574367676322,
-0.00969254902841235));
#37583=CARTESIAN_POINT('Ctrl Pts',(-0.207978587895246,0.00453876056307716,
-0.0098204277346072));
#37584=CARTESIAN_POINT('Ctrl Pts',(-0.207962491805793,0.00503450927170103,
-0.00997600800815991));
#37585=CARTESIAN_POINT('Ctrl Pts',(-0.207966830101282,0.00551329932707707,
-0.0100936573257618));
#37586=CARTESIAN_POINT('Ctrl Pts',(-0.207979805946424,0.00588082572595351,
-0.0101643937148489));
#37587=CARTESIAN_POINT('Ctrl Pts',(-0.20798954667625,0.00608609437374459,
-0.0101986511546884));
#37588=CARTESIAN_POINT('Ctrl Pts',(-0.20799983239929,0.00626736392668125,
-0.0102251009669269));
#37589=CARTESIAN_POINT('Ctrl Pts',(-0.208005585937768,0.00635637311449185,
-0.0102366662104294));
#37590=CARTESIAN_POINT('Ctrl Pts',(-0.208017332757161,0.006528741960817,
-0.0102576007511969));
#37591=CARTESIAN_POINT('Ctrl Pts',(-0.208042143315929,0.00685809179282729,
-0.0102902189911923));
#37592=CARTESIAN_POINT('Ctrl Pts',(-0.20807287172922,0.00722363415368649,
-0.0103096143982934));
#37593=CARTESIAN_POINT('Ctrl Pts',(-0.208097512282003,0.00749999794611554,
-0.0103101497493061));
#37594=CARTESIAN_POINT('',(-0.208182230285086,0.0122530779316807,-0.00898281412196308));
#37595=CARTESIAN_POINT('Ctrl Pts',(-0.208097512100336,0.00749999999333126,
-0.0103101497453589));
#37596=CARTESIAN_POINT('Ctrl Pts',(-0.208073095868969,0.00777529216228051,
-0.0103096192065392));
#37597=CARTESIAN_POINT('Ctrl Pts',(-0.208052770097806,0.00801816593243897,
-0.0102968489434138));
#37598=CARTESIAN_POINT('Ctrl Pts',(-0.208036595893026,0.00822421145027163,
-0.0102801607371037));
#37599=CARTESIAN_POINT('Ctrl Pts',(-0.208028508790636,0.00832723420918796,
-0.0102718166339487));
#37600=CARTESIAN_POINT('Ctrl Pts',(-0.208021458921539,0.00842105016711052,
-0.0102625233446917));
#37601=CARTESIAN_POINT('Ctrl Pts',(-0.208015198382678,0.00850971509292231,
-0.0102525567157745));
#37602=CARTESIAN_POINT('Ctrl Pts',(-0.208012068113248,0.0085540475558282,
-0.0102475734013159));
#37603=CARTESIAN_POINT('Ctrl Pts',(-0.208009135949875,0.00859708885229161,
-0.0102423861496861));
#37604=CARTESIAN_POINT('Ctrl Pts',(-0.208006716705287,0.00863334075408494,
-0.0102378148682447));
#37605=CARTESIAN_POINT('Ctrl Pts',(-0.208004297460699,0.00866959265587827,
-0.0102332435868033));
#37606=CARTESIAN_POINT('Ctrl Pts',(-0.20800238868474,0.00869906863367712,
-0.0102294010507216));
#37607=CARTESIAN_POINT('Ctrl Pts',(-0.207999697808039,0.00874426209474986,
-0.0102231481050333));
#37608=CARTESIAN_POINT('Ctrl Pts',(-0.207997006931337,0.0087894555558226,
-0.010216895159345));
#37609=CARTESIAN_POINT('Ctrl Pts',(-0.20799353853445,0.00885033817316214,
-0.0102080209706738));
#37610=CARTESIAN_POINT('Ctrl Pts',(-0.207990574887146,0.00890654940277088,
-0.0101992242222599));
#37611=CARTESIAN_POINT('Ctrl Pts',(-0.207987611239842,0.00896276063237962,
-0.010190427473846));
#37612=CARTESIAN_POINT('Ctrl Pts',(-0.207985149057711,0.00901432467196044,
-0.0101818593407826));
#37613=CARTESIAN_POINT('Ctrl Pts',(-0.207982879750747,0.00906629658792817,
-0.0101727931378578));
#37614=CARTESIAN_POINT('Ctrl Pts',(-0.20797834113682,0.00917024041986364,
-0.010154660732008));
#37615=CARTESIAN_POINT('Ctrl Pts',(-0.207974577832061,0.00927578369170264,
-0.0101343607483211));
#37616=CARTESIAN_POINT('Ctrl Pts',(-0.207971762511418,0.00937804782437877,
-0.0101128843431944));
#37617=CARTESIAN_POINT('Ctrl Pts',(-0.207966131870133,0.00958257608973103,
-0.0100699315329408));
#37618=CARTESIAN_POINT('Ctrl Pts',(-0.20796427977108,0.0097741179809218,
-0.0100228895524523));
#37619=CARTESIAN_POINT('Ctrl Pts',(-0.207966549569727,0.00996992151477133,
-0.00996812951220845));
#37620=CARTESIAN_POINT('Ctrl Pts',(-0.207968819368374,0.0101657250486209,
-0.00991336947196463));
#37621=CARTESIAN_POINT('Ctrl Pts',(-0.207975222005227,0.0103656352498877,
-0.00985038778992463));
#37622=CARTESIAN_POINT('Ctrl Pts',(-0.207986417905805,0.010563559735708,
-0.00978041553776925));
#37623=CARTESIAN_POINT('Ctrl Pts',(-0.207992015856095,0.0106625219786182,
-0.00974542941169156));
#37624=CARTESIAN_POINT('Ctrl Pts',(-0.20799881204306,0.0107609944554867,
-0.00970869929203595));
#37625=CARTESIAN_POINT('Ctrl Pts',(-0.208006463466485,0.0108567448312281,
-0.00967116784099722));
#37626=CARTESIAN_POINT('Ctrl Pts',(-0.208010289178198,0.0109046200190988,
-0.00965240211547786));
#37627=CARTESIAN_POINT('Ctrl Pts',(-0.208014328064145,0.0109518251710427,
-0.00963346528036175));
#37628=CARTESIAN_POINT('Ctrl Pts',(-0.20801901390864,0.0110022628486564,
-0.00961270486607612));
#37629=CARTESIAN_POINT('Ctrl Pts',(-0.208023699753135,0.0110527005262702,
-0.0095919444517905));
#37630=CARTESIAN_POINT('Ctrl Pts',(-0.208029035072463,0.0111063236122112,
-0.00956924463408429));
#37631=CARTESIAN_POINT('Ctrl Pts',(-0.20803324932473,0.0111470006771207,
-0.00955168810886531));
#37632=CARTESIAN_POINT('Ctrl Pts',(-0.208037463576997,0.0111876777420301,
-0.00953413158364634));
#37633=CARTESIAN_POINT('Ctrl Pts',(-0.208040553165688,0.0112154809968615,
-0.00952188389873837));
#37634=CARTESIAN_POINT('Ctrl Pts',(-0.20804438099605,0.0112489841224429,
-0.0095069446265188));
#37635=CARTESIAN_POINT('Ctrl Pts',(-0.208048208826411,0.0112824872480244,
-0.00949200535429924));
#37636=CARTESIAN_POINT('Ctrl Pts',(-0.208052776893594,0.0113216485495595,
-0.00947428265767254));
#37637=CARTESIAN_POINT('Ctrl Pts',(-0.20805763091643,0.011361898207728,
-0.00945568176171258));
#37638=CARTESIAN_POINT('Ctrl Pts',(-0.208067338962103,0.011442397524065,
-0.00941847996979267));
#37639=CARTESIAN_POINT('Ctrl Pts',(-0.208078188322781,0.0115273059902323,
-0.00937788080676488));
#37640=CARTESIAN_POINT('Ctrl Pts',(-0.208090526205669,0.0116195439206632,
-0.00933172437706195));
#37641=CARTESIAN_POINT('Ctrl Pts',(-0.208115201971445,0.0118040197815248,
-0.0092394115176561));
#37642=CARTESIAN_POINT('Ctrl Pts',(-0.208145833538144,0.0120177654804916,
-0.00912479078211141));
#37643=CARTESIAN_POINT('Ctrl Pts',(-0.208182230285086,0.0122530779316807,
-0.00898281412196308));
#37644=CARTESIAN_POINT('Ctrl Pts',(-0.208182276449934,0.0122530856411887,
-0.00898281044739297));
#37645=CARTESIAN_POINT('Ctrl Pts',(-0.207850571746568,0.0122531164075521,
-0.00897558571096322));
#37646=CARTESIAN_POINT('Ctrl Pts',(-0.207517024495258,0.0122531509908904,
-0.00896831863032881));
#37647=CARTESIAN_POINT('Ctrl Pts',(-0.207182088327276,0.0122531894495252,
-0.00896101902474837));
#37648=CARTESIAN_POINT('Origin',(-0.209569677721342,0.00750000034173499,
-0.00120784314777216));
#37649=CARTESIAN_POINT('',(-0.209182495727072,0.0122512742386181,-0.00900210870397552));
#37650=CARTESIAN_POINT('',(-0.209097173656828,0.00749996683895177,-0.0103336053779799));
#37651=CARTESIAN_POINT('Ctrl Pts',(-0.209182495727072,0.0122512742386181,
-0.00900210870397552));
#37652=CARTESIAN_POINT('Ctrl Pts',(-0.209146116898134,0.0120162484633245,
-0.0091444993018481));
#37653=CARTESIAN_POINT('Ctrl Pts',(-0.209115485562962,0.0118027042814943,
-0.00925946898166217));
#37654=CARTESIAN_POINT('Ctrl Pts',(-0.209090795759128,0.0116183929515475,
-0.0093520603329931));
#37655=CARTESIAN_POINT('Ctrl Pts',(-0.209078450857211,0.0115262372865741,
-0.00939835600865857));
#37656=CARTESIAN_POINT('Ctrl Pts',(-0.209067590900416,0.0114414021296796,
-0.00943907723696154));
#37657=CARTESIAN_POINT('Ctrl Pts',(-0.209057864907749,0.0113609473140376,
-0.00947640086291531));
#37658=CARTESIAN_POINT('Ctrl Pts',(-0.209053001911415,0.0113207199062166,
-0.00949506267589219));
#37659=CARTESIAN_POINT('Ctrl Pts',(-0.209048423039397,0.0112815734658911,
-0.00951284595782519));
#37660=CARTESIAN_POINT('Ctrl Pts',(-0.209044587689804,0.0112481086307926,
-0.00952782476656639));
#37661=CARTESIAN_POINT('Ctrl Pts',(-0.209040752340212,0.0112146437956942,
-0.00954280357530759));
#37662=CARTESIAN_POINT('Ctrl Pts',(-0.209037658496315,0.0111869028464035,
-0.00955507067833089));
#37663=CARTESIAN_POINT('Ctrl Pts',(-0.209033422336463,0.0111461861938047,
-0.00957271035297675));
#37664=CARTESIAN_POINT('Ctrl Pts',(-0.20902918617661,0.011105469541206,
-0.00959035002762261));
#37665=CARTESIAN_POINT('Ctrl Pts',(-0.209023811347096,0.0110517037399591,
-0.00961319454862126));
#37666=CARTESIAN_POINT('Ctrl Pts',(-0.209019091651199,0.01100117207776,
-0.00963406841813438));
#37667=CARTESIAN_POINT('Ctrl Pts',(-0.209014371955302,0.010950640415561,
-0.00965494228764749));
#37668=CARTESIAN_POINT('Ctrl Pts',(-0.209010304834951,0.0109033909435601,
-0.00967396317346768));
#37669=CARTESIAN_POINT('Ctrl Pts',(-0.209006450770597,0.0108554755926814,
-0.00969280968065493));
#37670=CARTESIAN_POINT('Ctrl Pts',(-0.208998742641888,0.010759644890924,
-0.00973050269502944));
#37671=CARTESIAN_POINT('Ctrl Pts',(-0.208991889348806,0.0106611071742381,
-0.00976737806350049));
#37672=CARTESIAN_POINT('Ctrl Pts',(-0.208986238313865,0.0105622377320011,
-0.00980244686196568));
#37673=CARTESIAN_POINT('Ctrl Pts',(-0.208974936243982,0.0103644988475271,
-0.00987258445889605));
#37674=CARTESIAN_POINT('Ctrl Pts',(-0.208968442737192,0.0101654202293464,
-0.0099355173677369));
#37675=CARTESIAN_POINT('Ctrl Pts',(-0.208966088716348,0.00996977678241938,
-0.00999042751774837));
#37676=CARTESIAN_POINT('Ctrl Pts',(-0.208963734695503,0.00977413333549238,
-0.0100453376677598));
#37677=CARTESIAN_POINT('Ctrl Pts',(-0.208965510366025,0.00958206588990063,
-0.0100926755906785));
#37678=CARTESIAN_POINT('Ctrl Pts',(-0.208971084439266,0.00937745137366946,
-0.0101357826877813));
#37679=CARTESIAN_POINT('Ctrl Pts',(-0.208973871475886,0.00927514411555387,
-0.0101573362363327));
#37680=CARTESIAN_POINT('Ctrl Pts',(-0.208977611311151,0.00916966863997126,
-0.0101776849801711));
#37681=CARTESIAN_POINT('Ctrl Pts',(-0.20898213094383,0.00906579616679699,
-0.0101958616298435));
#37682=CARTESIAN_POINT('Ctrl Pts',(-0.208984390760169,0.00901385993020985,
-0.0102049499546797));
#37683=CARTESIAN_POINT('Ctrl Pts',(-0.208986844580244,0.00896233246271355,
-0.010213538751811));
#37684=CARTESIAN_POINT('Ctrl Pts',(-0.208989799995037,0.00890618019447978,
-0.0102223541299263));
#37685=CARTESIAN_POINT('Ctrl Pts',(-0.208992755409829,0.00885002792624601,
-0.0102311695080417));
#37686=CARTESIAN_POINT('Ctrl Pts',(-0.208996215703227,0.00878922659380881,
-0.010240060417762));
#37687=CARTESIAN_POINT('Ctrl Pts',(-0.208998902942324,0.00874408042561425,
-0.0102463272818958));
#37688=CARTESIAN_POINT('Ctrl Pts',(-0.209001590181421,0.00869893425741969,
-0.0102525941460297));
#37689=CARTESIAN_POINT('Ctrl Pts',(-0.209003499782319,0.00866947167989352,
-0.0102564478100287));
#37690=CARTESIAN_POINT('Ctrl Pts',(-0.209005922071796,0.0086332384398221,
-0.010261031993143));
#37691=CARTESIAN_POINT('Ctrl Pts',(-0.209008344361273,0.00859700519975068,
-0.0102656161762573));
#37692=CARTESIAN_POINT('Ctrl Pts',(-0.209011281793522,0.0085539877664341,
-0.0102708179931996));
#37693=CARTESIAN_POINT('Ctrl Pts',(-0.209014420106914,0.00850967487191003,
-0.0102758160109009));
#37694=CARTESIAN_POINT('Ctrl Pts',(-0.209020696733697,0.00842104908286189,
-0.0102858120463034));
#37695=CARTESIAN_POINT('Ctrl Pts',(-0.209027773784346,0.0083272551517127,
-0.0102951355071637));
#37696=CARTESIAN_POINT('Ctrl Pts',(-0.209035898856334,0.00822424368548321,
-0.0103035078611286));
#37697=CARTESIAN_POINT('Ctrl Pts',(-0.209052149000311,0.00801822075302423,
-0.0103202525690584));
#37698=CARTESIAN_POINT('Ctrl Pts',(-0.209072593856506,0.00777532666243376,
-0.0103330720239394));
#37699=CARTESIAN_POINT('Ctrl Pts',(-0.209097173656828,0.00749996683895177,
-0.0103336053779799));
#37700=CARTESIAN_POINT('',(-0.209182613690262,0.00275154001515932,-0.00900382387632688));
#37701=CARTESIAN_POINT('Ctrl Pts',(-0.20909717356973,0.00749996586807601,
-0.0103336053760826));
#37702=CARTESIAN_POINT('Ctrl Pts',(-0.209072489707309,0.00722481928663946,
-0.01033306766277));
#37703=CARTESIAN_POINT('Ctrl Pts',(-0.20904171049841,0.00686077358303126,
-0.0103137662843188));
#37704=CARTESIAN_POINT('Ctrl Pts',(-0.209016873870949,0.00653266430565598,
-0.010281293384316));
#37705=CARTESIAN_POINT('Ctrl Pts',(-0.209005115616393,0.00636077619910354,
-0.0102604255694866));
#37706=CARTESIAN_POINT('Ctrl Pts',(-0.208999372618018,0.00627224778053745,
-0.0102489323528682));
#37707=CARTESIAN_POINT('Ctrl Pts',(-0.208989045745688,0.0060906225411391,
-0.0102224377908441));
#37708=CARTESIAN_POINT('Ctrl Pts',(-0.208979290894002,0.00588500517489839,
-0.0101881039000263));
#37709=CARTESIAN_POINT('Ctrl Pts',(-0.208966327046493,0.00551658091107566,
-0.0101171362638947));
#37710=CARTESIAN_POINT('Ctrl Pts',(-0.208962151603096,0.00503451819218248,
-0.00999833805250308));
#37711=CARTESIAN_POINT('Ctrl Pts',(-0.208978587062817,0.00453890814300135,
-0.00984222924809274));
#37712=CARTESIAN_POINT('Ctrl Pts',(-0.209002677049482,0.00419387918757995,
-0.00971306850389939));
#37713=CARTESIAN_POINT('Ctrl Pts',(-0.209018982861624,0.00400468657447842,
-0.0096370935893603));
#37714=CARTESIAN_POINT('Ctrl Pts',(-0.209035148855368,0.0038430099342979,
-0.00956840324924233));
#37715=CARTESIAN_POINT('Ctrl Pts',(-0.209044401153986,0.00376000689156962,
-0.00953165274028389));
#37716=CARTESIAN_POINT('Ctrl Pts',(-0.209062680278958,0.00360343910340024,
-0.00946067603908059));
#37717=CARTESIAN_POINT('Ctrl Pts',(-0.209100582810176,0.00330674321880253,
-0.00931824322218647));
#37718=CARTESIAN_POINT('Ctrl Pts',(-0.209146370547163,0.00298649792918081,
-0.00914605984684738));
#37719=CARTESIAN_POINT('Ctrl Pts',(-0.209182613690262,0.00275154001515932,
-0.00900382387632688));
#37720=CARTESIAN_POINT('',(-0.210183371239666,0.00275146176851279,-0.00902553543512514));
#37721=CARTESIAN_POINT('Ctrl Pts',(-0.209182669503787,0.00275154408037991,
-0.00900382756445142));
#37722=CARTESIAN_POINT('Ctrl Pts',(-0.209514380222137,0.00275151621947163,
-0.00901102289771852));
#37723=CARTESIAN_POINT('Ctrl Pts',(-0.209848122110046,0.00275148453891749,
-0.00901826006884851));
#37724=CARTESIAN_POINT('Ctrl Pts',(-0.21018341152138,0.00275144896457034,
-0.00902552851673686));
#37725=CARTESIAN_POINT('',(-0.210096846436932,0.00749994274414048,-0.0103553392159764));
#37726=CARTESIAN_POINT('Ctrl Pts',(-0.210183371239666,0.00275146176851279,
-0.00902553543512514));
#37727=CARTESIAN_POINT('Ctrl Pts',(-0.210146994593344,0.0029873235141714,
-0.00916832180670742));
#37728=CARTESIAN_POINT('Ctrl Pts',(-0.210116353263695,0.00320164542671377,
-0.00928356921553769));
#37729=CARTESIAN_POINT('Ctrl Pts',(-0.210091638158358,0.00338667278164948,
-0.0093763774552128));
#37730=CARTESIAN_POINT('Ctrl Pts',(-0.21007928060569,0.00347918645911733,
-0.00942278157505036));
#37731=CARTESIAN_POINT('Ctrl Pts',(-0.210068404179204,0.00356436440277715,
-0.00946359567450267));
#37732=CARTESIAN_POINT('Ctrl Pts',(-0.21005865995935,0.00364512021905286,
-0.00950098725273489));
#37733=CARTESIAN_POINT('Ctrl Pts',(-0.210053787849423,0.00368549812719071,
-0.00951968304185099));
#37734=CARTESIAN_POINT('Ctrl Pts',(-0.210049199422547,0.00372478455364116,
-0.00953749416088998));
#37735=CARTESIAN_POINT('Ctrl Pts',(-0.21004535108913,0.00375841244086312,
-0.00955251441648829));
#37736=CARTESIAN_POINT('Ctrl Pts',(-0.210041502755713,0.00379204032808509,
-0.00956753467208659));
#37737=CARTESIAN_POINT('Ctrl Pts',(-0.210038392506187,0.00381996763616456,
-0.00957985649103939));
#37738=CARTESIAN_POINT('Ctrl Pts',(-0.210034148670161,0.00386075504915408,
-0.00959748660077347));
#37739=CARTESIAN_POINT('Ctrl Pts',(-0.210029904834134,0.00390154246214361,
-0.00961511671050755));
#37740=CARTESIAN_POINT('Ctrl Pts',(-0.210024531039477,0.00395526288300835,
-0.00963788825278974));
#37741=CARTESIAN_POINT('Ctrl Pts',(-0.210019806380593,0.0040057336415685,
-0.00965868830426901));
#37742=CARTESIAN_POINT('Ctrl Pts',(-0.210015081721709,0.00405620440012864,
-0.00967948835574828));
#37743=CARTESIAN_POINT('Ctrl Pts',(-0.210011003655277,0.00410337781766793,
-0.0096984338930203));
#37744=CARTESIAN_POINT('Ctrl Pts',(-0.21000713624919,0.00415119528734392,
-0.0097171980344378));
#37745=CARTESIAN_POINT('Ctrl Pts',(-0.209999401437016,0.0042468302266959,
-0.0097547263172728));
#37746=CARTESIAN_POINT('Ctrl Pts',(-0.209992511923845,0.00434508601214227,
-0.00979140678221356));
#37747=CARTESIAN_POINT('Ctrl Pts',(-0.209986811465036,0.00444335069677145,
-0.00982618735090269));
#37748=CARTESIAN_POINT('Ctrl Pts',(-0.209975410547418,0.0046398800660298,
-0.00989574848828094));
#37749=CARTESIAN_POINT('Ctrl Pts',(-0.209968763765471,0.00483642846725269,
-0.00995780579218629));
#37750=CARTESIAN_POINT('Ctrl Pts',(-0.209966215642179,0.00503111252250329,
-0.0100124209606021));
#37751=CARTESIAN_POINT('Ctrl Pts',(-0.209963667518888,0.0052257965777539,
-0.0100670361290179));
#37752=CARTESIAN_POINT('Ctrl Pts',(-0.209965211079014,0.00541851214447677,
-0.0101145299821102));
#37753=CARTESIAN_POINT('Ctrl Pts',(-0.209970565738309,0.00562248776116485,
-0.0101574995487602));
#37754=CARTESIAN_POINT('Ctrl Pts',(-0.209973243067956,0.00572447556950889,
-0.0101789843320852));
#37755=CARTESIAN_POINT('Ctrl Pts',(-0.209976875917157,0.00582930603355706,
-0.0101992117990275));
#37756=CARTESIAN_POINT('Ctrl Pts',(-0.20998129401994,0.00593255289743084,
-0.0102172968845377));
#37757=CARTESIAN_POINT('Ctrl Pts',(-0.209983503071332,0.00598417632936772,
-0.0102263394272928));
#37758=CARTESIAN_POINT('Ctrl Pts',(-0.209985907538537,0.00603539616134188,
-0.0102348876589781));
#37759=CARTESIAN_POINT('Ctrl Pts',(-0.209988804349278,0.006091090092447,
-0.0102436475952405));
#37760=CARTESIAN_POINT('Ctrl Pts',(-0.20999170116002,0.00614678402355212,
-0.0102524075315029));
#37761=CARTESIAN_POINT('Ctrl Pts',(-0.209995093480332,0.00620697551148496,
-0.0102612335501065));
#37762=CARTESIAN_POINT('Ctrl Pts',(-0.2099977485288,0.00625192088319922,
-0.0102674923467883));
#37763=CARTESIAN_POINT('Ctrl Pts',(-0.210000403577268,0.00629686625491348,
-0.0102737511434701));
#37764=CARTESIAN_POINT('Ctrl Pts',(-0.210002316904279,0.00632653780075192,
-0.0102776473796006));
#37765=CARTESIAN_POINT('Ctrl Pts',(-0.210004741283944,0.00636289412582311,
-0.0102822627645651));
#37766=CARTESIAN_POINT('Ctrl Pts',(-0.210007165663609,0.00639925045089429,
-0.0102868781495297));
#37767=CARTESIAN_POINT('Ctrl Pts',(-0.21001010349879,0.00644230485879222,
-0.0102921021626682));
#37768=CARTESIAN_POINT('Ctrl Pts',(-0.210013249753823,0.00648669002716698,
-0.0102971263935411));
#37769=CARTESIAN_POINT('Ctrl Pts',(-0.210019542263891,0.00657546036391651,
-0.0103071748552868));
#37770=CARTESIAN_POINT('Ctrl Pts',(-0.21002666540856,0.00666954022906901,
-0.0103165642357206));
#37771=CARTESIAN_POINT('Ctrl Pts',(-0.210034860263665,0.00677289174688065,
-0.0103249978927266));
#37772=CARTESIAN_POINT('Ctrl Pts',(-0.210051249973874,0.00697959478250394,
-0.0103418652067386));
#37773=CARTESIAN_POINT('Ctrl Pts',(-0.210071929000393,0.00722338510027445,
-0.0103547958065898));
#37774=CARTESIAN_POINT('Ctrl Pts',(-0.210096846437032,0.00749994274413152,
-0.0103553392159786));
#37775=CARTESIAN_POINT('',(-0.210182952559,0.0122509750948127,-0.0090240400549463));
#37776=CARTESIAN_POINT('Ctrl Pts',(-0.210096846436932,0.00749994274414048,
-0.0103553392159764));
#37777=CARTESIAN_POINT('Ctrl Pts',(-0.210096421573129,0.00750467804303478,
-0.0103553300078083));
#37778=CARTESIAN_POINT('Ctrl Pts',(-0.210094091070512,0.00753069899736505,
-0.0103552503224888));
#37779=CARTESIAN_POINT('Ctrl Pts',(-0.210092277287072,0.00755102334106925,
-0.0103550973215045));
#37780=CARTESIAN_POINT('Ctrl Pts',(-0.210090463503631,0.00757134768477346,
-0.0103549443205201));
#37781=CARTESIAN_POINT('Ctrl Pts',(-0.210089165078757,0.00758597569404241,
-0.0103547805867168));
#37782=CARTESIAN_POINT('Ctrl Pts',(-0.210087794381028,0.00760145938077238,
-0.0103545787390152));
#37783=CARTESIAN_POINT('Ctrl Pts',(-0.210085052985569,0.00763242675423232,
-0.0103541750436119));
#37784=CARTESIAN_POINT('Ctrl Pts',(-0.210082023924896,0.00766681588579745,
-0.0103535532925314));
#37785=CARTESIAN_POINT('Ctrl Pts',(-0.210079125509802,0.00769995376384079,
-0.0103527644907727));
#37786=CARTESIAN_POINT('Ctrl Pts',(-0.210073328679614,0.00776622951992748,
-0.0103511868872554));
#37787=CARTESIAN_POINT('Ctrl Pts',(-0.21006805238263,0.00782750311150865,
-0.0103490353326892));
#37788=CARTESIAN_POINT('Ctrl Pts',(-0.210062967839213,0.00788740023130505,
-0.010346381440422));
#37789=CARTESIAN_POINT('Ctrl Pts',(-0.210057883295797,0.00794729735110145,
-0.0103437275481549));
#37790=CARTESIAN_POINT('Ctrl Pts',(-0.210052991179761,0.00800581599859524,
-0.0103405403250739));
#37791=CARTESIAN_POINT('Ctrl Pts',(-0.210048369589446,0.00806208143919039,
-0.0103369699750641));
#37792=CARTESIAN_POINT('Ctrl Pts',(-0.210043747999131,0.00811834687978555,
-0.0103333996250543));
#37793=CARTESIAN_POINT('Ctrl Pts',(-0.210039396828702,0.00817235991846103,
-0.0103294510161944));
#37794=CARTESIAN_POINT('Ctrl Pts',(-0.210035314943403,0.00822397052514526,
-0.0103252576166531));
#37795=CARTESIAN_POINT('Ctrl Pts',(-0.210027151172807,0.00832719173851372,
-0.0103168708175704));
#37796=CARTESIAN_POINT('Ctrl Pts',(-0.210020063277611,0.00842080552037382,
-0.0103075630469351));
#37797=CARTESIAN_POINT('Ctrl Pts',(-0.210013778935997,0.00850937355036198,
-0.0102975762177072));
#37798=CARTESIAN_POINT('Ctrl Pts',(-0.21001063676519,0.00855365756535605,
-0.0102925828030932));
#37799=CARTESIAN_POINT('Ctrl Pts',(-0.210007696289592,0.00859667666147962,
-0.0102873825130392));
#37800=CARTESIAN_POINT('Ctrl Pts',(-0.210005271703267,0.00863292877725493,
-0.0102827971657773));
#37801=CARTESIAN_POINT('Ctrl Pts',(-0.210002847116943,0.00866918089303023,
-0.0102782118185155));
#37802=CARTESIAN_POINT('Ctrl Pts',(-0.210000935973877,0.0086986795055452,
-0.0102743539231139));
#37803=CARTESIAN_POINT('Ctrl Pts',(-0.209998256336171,0.00874376620306087,
-0.0102680969834612));
#37804=CARTESIAN_POINT('Ctrl Pts',(-0.209995576698465,0.00878885290057654,
-0.0102618400438085));
#37805=CARTESIAN_POINT('Ctrl Pts',(-0.209992133114742,0.00884949947558208,
-0.010252974837074));
#37806=CARTESIAN_POINT('Ctrl Pts',(-0.209989192135327,0.00890555230308399,
-0.010244179247103));
#37807=CARTESIAN_POINT('Ctrl Pts',(-0.209986251155911,0.0089616051305859,
-0.010235383657132));
#37808=CARTESIAN_POINT('Ctrl Pts',(-0.209983809530347,0.00901308822745524,
-0.0102268071956456));
#37809=CARTESIAN_POINT('Ctrl Pts',(-0.209981563015109,0.00906497838414453,
-0.0102177320221761));
#37810=CARTESIAN_POINT('Ctrl Pts',(-0.209977069984633,0.0091687586975231,
-0.0101995816752372));
#37811=CARTESIAN_POINT('Ctrl Pts',(-0.209973361104316,0.0092741356329341,
-0.0101792658831118));
#37812=CARTESIAN_POINT('Ctrl Pts',(-0.209970608023758,0.00937649422666917,
-0.0101577136994801));
#37813=CARTESIAN_POINT('Ctrl Pts',(-0.209965101862643,0.0095812114141393,
-0.0101146093322166));
#37814=CARTESIAN_POINT('Ctrl Pts',(-0.209963406965898,0.00977397402149797,
-0.0100671083632951));
#37815=CARTESIAN_POINT('Ctrl Pts',(-0.209965844413768,0.0099694793343208,
-0.0100122458991389));
#37816=CARTESIAN_POINT('Ctrl Pts',(-0.209968281861638,0.0101649846471436,
-0.0099573834349827));
#37817=CARTESIAN_POINT('Ctrl Pts',(-0.209974859957364,0.0103631109907,-0.00989477754227005));
#37818=CARTESIAN_POINT('Ctrl Pts',(-0.209986266187064,0.0105607267647511,
-0.0098247250529686));
#37819=CARTESIAN_POINT('Ctrl Pts',(-0.209991969301913,0.0106595346517767,
-0.00978969880831788));
#37820=CARTESIAN_POINT('Ctrl Pts',(-0.209998879810517,0.0107582137766952,
-0.00975279434377352));
#37821=CARTESIAN_POINT('Ctrl Pts',(-0.210006645172636,0.0108542149694637,
-0.00971505164932369));
#37822=CARTESIAN_POINT('Ctrl Pts',(-0.210010527853695,0.010902215565848,
-0.00969618030209878));
#37823=CARTESIAN_POINT('Ctrl Pts',(-0.21001462357696,0.0109495579232455,
-0.00967713027028166));
#37824=CARTESIAN_POINT('Ctrl Pts',(-0.2100193774721,0.0110002414631578,
-0.00965620063211537));
#37825=CARTESIAN_POINT('Ctrl Pts',(-0.210024131367239,0.0110509250030702,
-0.00963527099394908));
#37826=CARTESIAN_POINT('Ctrl Pts',(-0.210029546028417,0.01110490099765,
-0.00961234242141701));
#37827=CARTESIAN_POINT('Ctrl Pts',(-0.210033805218153,0.0111457179693001,
-0.00959466225771742));
#37828=CARTESIAN_POINT('Ctrl Pts',(-0.210038064407889,0.0111865349409501,
-0.00957698209401783));
#37829=CARTESIAN_POINT('Ctrl Pts',(-0.210041164439004,0.0112142671573592,
-0.00956471994512065));
#37830=CARTESIAN_POINT('Ctrl Pts',(-0.210045008403367,0.0112477443471597,
-0.00954973750983502));
#37831=CARTESIAN_POINT('Ctrl Pts',(-0.21004885236773,0.0112812215369602,
-0.00953475507454939));
#37832=CARTESIAN_POINT('Ctrl Pts',(-0.210053442297848,0.0113204010892225,
-0.00951695885970419));
#37833=CARTESIAN_POINT('Ctrl Pts',(-0.210058314380606,0.0113606536646177,
-0.00949828722445998));
#37834=CARTESIAN_POINT('Ctrl Pts',(-0.210068058546121,0.0114411588154081,
-0.00946094395397156));
#37835=CARTESIAN_POINT('Ctrl Pts',(-0.210078928773307,0.011526012881933,
-0.00942021624837313));
#37836=CARTESIAN_POINT('Ctrl Pts',(-0.210091279231665,0.0116181773530369,
-0.00937391926268402));
#37837=CARTESIAN_POINT('Ctrl Pts',(-0.21011598014838,0.0118025062952446,
-0.0092813252913058));
#37838=CARTESIAN_POINT('Ctrl Pts',(-0.210146603778555,0.0120160267225188,
-0.00916637191627331));
#37839=CARTESIAN_POINT('Ctrl Pts',(-0.210182952559,0.0122509750948127,-0.0090240400549463));
#37840=CARTESIAN_POINT('Ctrl Pts',(-0.210182993958729,0.0122509825883683,
-0.00902403639013458));
#37841=CARTESIAN_POINT('Ctrl Pts',(-0.209849556732748,0.012251076389419,
-0.00901673059642433));
#37842=CARTESIAN_POINT('Ctrl Pts',(-0.209516008085114,0.012251173766512,
-0.00900942019982785));
#37843=CARTESIAN_POINT('Ctrl Pts',(-0.209182556323231,0.0122512746577035,
-0.00900210976597304));
#37844=CARTESIAN_POINT('Origin',(-0.193568907911486,0.00750000067102937,
-0.00057655143392958));
#37845=CARTESIAN_POINT('',(-0.193177238558164,0.0122676067884443,-0.00867531668264591));
#37846=CARTESIAN_POINT('',(-0.193103863223514,0.00750326208931829,-0.00997223504951149));
#37847=CARTESIAN_POINT('Ctrl Pts',(-0.193177238558164,0.0122676067884443,
-0.00867531668264591));
#37848=CARTESIAN_POINT('Ctrl Pts',(-0.193141277408561,0.0120297062798438,
-0.00881450643419947));
#37849=CARTESIAN_POINT('Ctrl Pts',(-0.193096702853472,0.0117128138412265,
-0.00898007212936678));
#37850=CARTESIAN_POINT('Ctrl Pts',(-0.193053007151483,0.0113544430299681,
-0.00914564853116907));
#37851=CARTESIAN_POINT('Ctrl Pts',(-0.193033159712931,0.011177123403759,
-0.00922315221236596));
#37852=CARTESIAN_POINT('Ctrl Pts',(-0.193005590632074,0.0108636784687834,
-0.00934989089102075));
#37853=CARTESIAN_POINT('Ctrl Pts',(-0.192982407950007,0.0104851086177235,
-0.00948721987317339));
#37854=CARTESIAN_POINT('Ctrl Pts',(-0.192968408173786,0.00996069993436876,
-0.00964846359291627));
#37855=CARTESIAN_POINT('Ctrl Pts',(-0.192975189033209,0.00950003337125401,
-0.00975833993598715));
#37856=CARTESIAN_POINT('Ctrl Pts',(-0.192989252673654,0.00912702910240768,
-0.00982891691881178));
#37857=CARTESIAN_POINT('Ctrl Pts',(-0.19299947871711,0.00891840860987315,
-0.00986296989761181));
#37858=CARTESIAN_POINT('Ctrl Pts',(-0.193010186783734,0.00873159276027399,
-0.00988956309502806));
#37859=CARTESIAN_POINT('Ctrl Pts',(-0.193015853940037,0.00864328838181661,
-0.00990071154504017));
#37860=CARTESIAN_POINT('Ctrl Pts',(-0.193027433931117,0.00847013191613375,
-0.0099211982004547));
#37861=CARTESIAN_POINT('Ctrl Pts',(-0.193051412520838,0.00814133853363067,
-0.0099528640409497));
#37862=CARTESIAN_POINT('Ctrl Pts',(-0.193080619914893,0.00777761606572264,
-0.00997163740758629));
#37863=CARTESIAN_POINT('Ctrl Pts',(-0.193103863741755,0.00750326261887232,
-0.00997223506269818));
#37864=CARTESIAN_POINT('',(-0.193178837423798,0.00273574495468982,-0.0086773204769601));
#37865=CARTESIAN_POINT('Ctrl Pts',(-0.193103863693919,0.0075032620497559,
-0.00997223506186141));
#37866=CARTESIAN_POINT('Ctrl Pts',(-0.193101982070691,0.00748087649952758,
-0.00997220214559293));
#37867=CARTESIAN_POINT('Ctrl Pts',(-0.193094992227577,0.0073973397143487,
-0.00997171707917436));
#37868=CARTESIAN_POINT('Ctrl Pts',(-0.193084786939789,0.00727362393760784,
-0.00996941923967326));
#37869=CARTESIAN_POINT('Ctrl Pts',(-0.193066650048077,0.00704999053098598,
-0.00996215274241276));
#37870=CARTESIAN_POINT('Ctrl Pts',(-0.193045003613772,0.00677035458551498,
-0.00994422576682089));
#37871=CARTESIAN_POINT('Ctrl Pts',(-0.193027940246176,0.00653410165293154,
-0.00992165651782325));
#37872=CARTESIAN_POINT('Ctrl Pts',(-0.193016479642015,0.00636065866460942,
-0.00990121037081368));
#37873=CARTESIAN_POINT('Ctrl Pts',(-0.193010824022097,0.00627131283022669,
-0.00988995406090102));
#37874=CARTESIAN_POINT('Ctrl Pts',(-0.193000398980532,0.00608661552070766,
-0.00986374663195098));
#37875=CARTESIAN_POINT('Ctrl Pts',(-0.192990329008554,0.00587750923105183,
-0.00982974235804112));
#37876=CARTESIAN_POINT('Ctrl Pts',(-0.192976630034204,0.00550500463892925,
-0.00975946406604019));
#37877=CARTESIAN_POINT('Ctrl Pts',(-0.192970301148135,0.00504236762906688,
-0.00964933948491919));
#37878=CARTESIAN_POINT('Ctrl Pts',(-0.192984713678361,0.00451957126348969,
-0.009488820974985));
#37879=CARTESIAN_POINT('Ctrl Pts',(-0.193008070991626,0.00414029891002481,
-0.00935148376040879));
#37880=CARTESIAN_POINT('Ctrl Pts',(-0.193035766744627,0.00382550828794464,
-0.00922433195482671));
#37881=CARTESIAN_POINT('Ctrl Pts',(-0.193055511987502,0.00364845234953881,
-0.00914699638297536));
#37882=CARTESIAN_POINT('Ctrl Pts',(-0.193098939509399,0.00329032861337595,
-0.00898168634553191));
#37883=CARTESIAN_POINT('Ctrl Pts',(-0.19314316987124,0.00297358087421801,
-0.00881634617994497));
#37884=CARTESIAN_POINT('Ctrl Pts',(-0.193178837423798,0.00273574495468982,
-0.0086773204769601));
#37885=CARTESIAN_POINT('',(-0.194178126336983,0.00273578034803723,-0.00869894669169024));
#37886=CARTESIAN_POINT('Ctrl Pts',(-0.193178923166509,0.00273574786287452,
-0.00867732404017732));
#37887=CARTESIAN_POINT('Ctrl Pts',(-0.193516558232873,0.00273575905641843,
-0.00868463055489243));
#37888=CARTESIAN_POINT('Ctrl Pts',(-0.19384994814426,0.00273576515675357,
-0.00869184229227085));
#37889=CARTESIAN_POINT('Ctrl Pts',(-0.194178193748642,0.00273576655198442,
-0.00869894004011713));
#37890=CARTESIAN_POINT('',(-0.194103296318277,0.00750354445494538,-0.00999384110469418));
#37891=CARTESIAN_POINT('Ctrl Pts',(-0.194178126336983,0.00273578034803723,
-0.00869894669169024));
#37892=CARTESIAN_POINT('Ctrl Pts',(-0.194142042098836,0.00297492111932904,
-0.00883872879554135));
#37893=CARTESIAN_POINT('Ctrl Pts',(-0.194097326545317,0.00329355354970724,
-0.00900492219595842));
#37894=CARTESIAN_POINT('Ctrl Pts',(-0.194053576967989,0.00365337062553203,
-0.00917080388678816));
#37895=CARTESIAN_POINT('Ctrl Pts',(-0.194033651716486,0.00383231370014839,
-0.00924877799144863));
#37896=CARTESIAN_POINT('Ctrl Pts',(-0.194006380571071,0.0041439301034018,
-0.00937441384127908));
#37897=CARTESIAN_POINT('Ctrl Pts',(-0.193983325356653,0.0045212416713753,
-0.00951094738593517));
#37898=CARTESIAN_POINT('Ctrl Pts',(-0.193969309601735,0.00504288807939639,
-0.0096710240379633));
#37899=CARTESIAN_POINT('Ctrl Pts',(-0.193975851273483,0.00550315434166333,
-0.0097806464712603));
#37900=CARTESIAN_POINT('Ctrl Pts',(-0.193989630863608,0.00587518475769505,
-0.00985093422918167));
#37901=CARTESIAN_POINT('Ctrl Pts',(-0.193999709756721,0.00608390961146259,
-0.00988494053456836));
#37902=CARTESIAN_POINT('Ctrl Pts',(-0.194010169566569,0.00626911514536853,
-0.00991126905619667));
#37903=CARTESIAN_POINT('Ctrl Pts',(-0.194015815544633,0.00635836535611191,
-0.00992254085629852));
#37904=CARTESIAN_POINT('Ctrl Pts',(-0.194027313474826,0.00653237287800241,
-0.00994305673262293));
#37905=CARTESIAN_POINT('Ctrl Pts',(-0.194044176847623,0.00676648600438274,
-0.00996570757859934));
#37906=CARTESIAN_POINT('Ctrl Pts',(-0.194071045174016,0.0071131119218024,
-0.00998731884686608));
#37907=CARTESIAN_POINT('Ctrl Pts',(-0.194090771216625,0.00735428354209366,
-0.0099936266379733));
#37908=CARTESIAN_POINT('Ctrl Pts',(-0.194103296319129,0.00750354416285038,
-0.0099938411048228));
#37909=CARTESIAN_POINT('',(-0.194177646062722,0.0122674896816452,-0.00869701042615392));
#37910=CARTESIAN_POINT('Ctrl Pts',(-0.194103296318277,0.00750354445494538,
-0.00999384110469418));
#37911=CARTESIAN_POINT('Ctrl Pts',(-0.194079958518618,0.00777941560445015,
-0.00999323250307843));
#37912=CARTESIAN_POINT('Ctrl Pts',(-0.194050661160514,0.00814497169210634,
-0.00997425522747218));
#37913=CARTESIAN_POINT('Ctrl Pts',(-0.194026644350104,0.00847534629457309,
-0.00994226043412574));
#37914=CARTESIAN_POINT('Ctrl Pts',(-0.194015080223235,0.00864898723807135,
-0.0099216166364075));
#37915=CARTESIAN_POINT('Ctrl Pts',(-0.194009390838132,0.00873816803744379,
-0.00991028930259834));
#37916=CARTESIAN_POINT('Ctrl Pts',(-0.193998842516715,0.00892342055893506,
-0.00988379830463233));
#37917=CARTESIAN_POINT('Ctrl Pts',(-0.193988741548766,0.00913090327575872,
-0.0098498322196108));
#37918=CARTESIAN_POINT('Ctrl Pts',(-0.193974878568344,0.00950167412757212,
-0.00977954635796348));
#37919=CARTESIAN_POINT('Ctrl Pts',(-0.193968222648747,0.00996018041429022,
-0.0096701523381651));
#37920=CARTESIAN_POINT('Ctrl Pts',(-0.193982176036166,0.0104821187883598,
-0.00950980282130545));
#37921=CARTESIAN_POINT('Ctrl Pts',(-0.194005272373616,0.010859398120637,
-0.00937311789949069));
#37922=CARTESIAN_POINT('Ctrl Pts',(-0.194032635572663,0.0111712397791765,
-0.00924724964660917));
#37923=CARTESIAN_POINT('Ctrl Pts',(-0.194052607422482,0.0113499762585385,
-0.00916927820776025));
#37924=CARTESIAN_POINT('Ctrl Pts',(-0.19409651347767,0.0117097359836059,
-0.00900325799596129));
#37925=CARTESIAN_POINT('Ctrl Pts',(-0.194141409034745,0.0120283418044791,
-0.00883692360353074));
#37926=CARTESIAN_POINT('Ctrl Pts',(-0.194177646062722,0.0122674896816452,
-0.00869701042615392));
#37927=CARTESIAN_POINT('Ctrl Pts',(-0.194177713311809,0.0122674988402921,
-0.0086970064915523));
#37928=CARTESIAN_POINT('Ctrl Pts',(-0.19384633828666,0.0122675305238753,
-0.00868982483646655));
#37929=CARTESIAN_POINT('Ctrl Pts',(-0.193512706876837,0.0122675670396735,
-0.00868259156414702));
#37930=CARTESIAN_POINT('Ctrl Pts',(-0.19317732938957,0.0122676084977587,
-0.00867531764039759));
#37931=CARTESIAN_POINT('Origin',(-0.213568579064389,0.00750000008594914,
-0.00135799511692069));
#37932=CARTESIAN_POINT('',(-0.21318423872705,0.0122469018747551,-0.00908490848644239));
#37933=CARTESIAN_POINT('',(-0.213095878685918,0.0075001804210207,-0.0104239546847203));
#37934=CARTESIAN_POINT('Ctrl Pts',(-0.21318423872705,0.0122469018747551,
-0.00908490848644239));
#37935=CARTESIAN_POINT('Ctrl Pts',(-0.213147967165249,0.0120126167213431,
-0.00922796055956868));
#37936=CARTESIAN_POINT('Ctrl Pts',(-0.213102062381918,0.0116929446600027,
-0.00940128351253897));
#37937=CARTESIAN_POINT('Ctrl Pts',(-0.213063926861882,0.0113964705502375,
-0.00954476979033539));
#37938=CARTESIAN_POINT('Ctrl Pts',(-0.213045448068908,0.0112396752196826,
-0.00961640605766646));
#37939=CARTESIAN_POINT('Ctrl Pts',(-0.213036119558812,0.0111569823392515,
-0.00965331518855872));
#37940=CARTESIAN_POINT('Ctrl Pts',(-0.213019513778469,0.0109934185748677,
-0.00972332629864973));
#37941=CARTESIAN_POINT('Ctrl Pts',(-0.213002795866849,0.0108031199259663,
-0.00980026058746646));
#37942=CARTESIAN_POINT('Ctrl Pts',(-0.212978010642917,0.0104566789835727,
-0.00993070195934068));
#37943=CARTESIAN_POINT('Ctrl Pts',(-0.212960929508415,0.00996624908753319,
-0.0100861135776349));
#37944=CARTESIAN_POINT('Ctrl Pts',(-0.212964587887053,0.00948339356377618,
-0.0102060491687593));
#37945=CARTESIAN_POINT('Ctrl Pts',(-0.212977231013709,0.00911548248511972,
-0.0102773844664645));
#37946=CARTESIAN_POINT('Ctrl Pts',(-0.2129868244226,0.00891006572109696,
-0.0103119301614037));
#37947=CARTESIAN_POINT('Ctrl Pts',(-0.212997018810102,0.00872854262977365,
-0.0103385981982886));
#37948=CARTESIAN_POINT('Ctrl Pts',(-0.213002708045327,0.00864034456961565,
-0.0103501327288066));
#37949=CARTESIAN_POINT('Ctrl Pts',(-0.213014457625488,0.00846865341581425,
-0.0103711386036274));
#37950=CARTESIAN_POINT('Ctrl Pts',(-0.21303947209247,0.0081405967091976,
-0.010403876123959));
#37951=CARTESIAN_POINT('Ctrl Pts',(-0.213070728457374,0.00777597269410619,
-0.0104234017023197));
#37952=CARTESIAN_POINT('Ctrl Pts',(-0.213095878685918,0.0075001804210207,
-0.0104239546847203));
#37953=CARTESIAN_POINT('',(-0.213185703211844,0.00275392014951917,-0.00908544467358939));
#37954=CARTESIAN_POINT('Ctrl Pts',(-0.213095878574979,0.0075001792078503,
-0.0104239546823292));
#37955=CARTESIAN_POINT('Ctrl Pts',(-0.213084624510229,0.00737722579854172,
-0.0104237121079522));
#37956=CARTESIAN_POINT('Ctrl Pts',(-0.213059646951704,0.00709723705871821,
-0.0104169601546021));
#37957=CARTESIAN_POINT('Ctrl Pts',(-0.213032355596658,0.006768339907401,
-0.0103945895617497));
#37958=CARTESIAN_POINT('Ctrl Pts',(-0.21301431087388,0.00653229766580737,
-0.0103712596161075));
#37959=CARTESIAN_POINT('Ctrl Pts',(-0.213002612318022,0.00636096639451181,
-0.0103502918217071));
#37960=CARTESIAN_POINT('Ctrl Pts',(-0.212996932214088,0.00627263427303648,
-0.0103387567924699));
#37961=CARTESIAN_POINT('Ctrl Pts',(-0.212986831556077,0.00609159909993886,
-0.0103121897259374));
#37962=CARTESIAN_POINT('Ctrl Pts',(-0.212977345692435,0.00588625226984478,
-0.0102776983880172));
#37963=CARTESIAN_POINT('Ctrl Pts',(-0.212964932877339,0.00551839699631466,
-0.0102064879064028));
#37964=CARTESIAN_POINT('Ctrl Pts',(-0.212961764061948,0.00503181826712215,
-0.010085595298052));
#37965=CARTESIAN_POINT('Ctrl Pts',(-0.212979242888073,0.00454450835103741,
-0.00993110843775244));
#37966=CARTESIAN_POINT('Ctrl Pts',(-0.213004229563994,0.00419793570972472,
-0.00980070684540739));
#37967=CARTESIAN_POINT('Ctrl Pts',(-0.213021037741107,0.00400755810154577,
-0.00972376773155705));
#37968=CARTESIAN_POINT('Ctrl Pts',(-0.213037718032556,0.00384368614291747,
-0.00965364519619393));
#37969=CARTESIAN_POINT('Ctrl Pts',(-0.213047047347857,0.00376108604420927,
-0.00961678428468142));
#37970=CARTESIAN_POINT('Ctrl Pts',(-0.21306553657481,0.00360429517525143,
-0.00954516870914107));
#37971=CARTESIAN_POINT('Ctrl Pts',(-0.213103652569734,0.00330787216258413,
-0.00940174125825834));
#37972=CARTESIAN_POINT('Ctrl Pts',(-0.213149495293687,0.00298820619271435,
-0.00922846437602459));
#37973=CARTESIAN_POINT('Ctrl Pts',(-0.213185703211844,0.00275392014951917,
-0.00908544467358939));
#37974=CARTESIAN_POINT('',(-0.214186413679644,0.00275332976643362,-0.0091068676959076));
#37975=CARTESIAN_POINT('Ctrl Pts',(-0.213185747109477,0.00275392392937051,
-0.00908544794936231));
#37976=CARTESIAN_POINT('Ctrl Pts',(-0.213519286834764,0.00275372517702273,
-0.00909258710293668));
#37977=CARTESIAN_POINT('Ctrl Pts',(-0.213852922274175,0.00275352290283973,
-0.00909972616793565));
#37978=CARTESIAN_POINT('Ctrl Pts',(-0.214186444847692,0.00275331723326959,
-0.00910686068007963));
#37979=CARTESIAN_POINT('',(-0.214095608114984,0.00750036597474129,-0.0104457182539273));
#37980=CARTESIAN_POINT('Ctrl Pts',(-0.214186413679644,0.00275332976643362,
-0.0091068676959076));
#37981=CARTESIAN_POINT('Ctrl Pts',(-0.214150100837136,0.00298844890012589,
-0.0092504211566524));
#37982=CARTESIAN_POINT('Ctrl Pts',(-0.214119444326417,0.00320233065924093,
-0.00936639784249271));
#37983=CARTESIAN_POINT('Ctrl Pts',(-0.214094651401162,0.00338708449027663,
-0.0094598261305769));
#37984=CARTESIAN_POINT('Ctrl Pts',(-0.214082254938534,0.00347946140579449,
-0.00950654027461899));
#37985=CARTESIAN_POINT('Ctrl Pts',(-0.214071323897576,0.00356454301339925,
-0.00954763912430158));
#37986=CARTESIAN_POINT('Ctrl Pts',(-0.214061493118068,0.00364534081995737,
-0.00958534769706394));
#37987=CARTESIAN_POINT('Ctrl Pts',(-0.214056577728313,0.00368573972323644,
-0.00960420198344512));
#37988=CARTESIAN_POINT('Ctrl Pts',(-0.214051938059047,0.00372508235601198,
-0.00962217860736835));
#37989=CARTESIAN_POINT('Ctrl Pts',(-0.214048052778835,0.00375866104194653,
-0.00963729427663179));
#37990=CARTESIAN_POINT('Ctrl Pts',(-0.214044167498623,0.00379223972788107,
-0.00965240994589524));
#37991=CARTESIAN_POINT('Ctrl Pts',(-0.214041034514651,0.00382001038131348,
-0.00966476079415632));
#37992=CARTESIAN_POINT('Ctrl Pts',(-0.214036691234293,0.00386111054867081,
-0.00968266254234618));
#37993=CARTESIAN_POINT('Ctrl Pts',(-0.214032347953934,0.00390221071602813,
-0.00970056429053603));
#37994=CARTESIAN_POINT('Ctrl Pts',(-0.214026798204625,0.00395671784545832,
-0.00972384112484572));
#37995=CARTESIAN_POINT('Ctrl Pts',(-0.214021921739019,0.0040077473839752,
-0.00974501814468437));
#37996=CARTESIAN_POINT('Ctrl Pts',(-0.214017045273413,0.00405877692249209,
-0.00976619516452301));
#37997=CARTESIAN_POINT('Ctrl Pts',(-0.214012839378027,0.00410627766752427,
-0.00978539701428086));
#37998=CARTESIAN_POINT('Ctrl Pts',(-0.21400884316301,0.00415439357417544,
-0.0098043993375676));
#37999=CARTESIAN_POINT('Ctrl Pts',(-0.214000850732976,0.00425062538747779,
-0.00984240398414109));
#38000=CARTESIAN_POINT('Ctrl Pts',(-0.213993699966926,0.00434936831381604,
-0.00987947535998419));
#38001=CARTESIAN_POINT('Ctrl Pts',(-0.213987755470683,0.00444744652452595,
-0.00991438998611061));
#38002=CARTESIAN_POINT('Ctrl Pts',(-0.213975866478195,0.00464360294594576,
-0.00998421923836345));
#38003=CARTESIAN_POINT('Ctrl Pts',(-0.213968797477862,0.00483703112941228,
-0.0100456551680694));
#38004=CARTESIAN_POINT('Ctrl Pts',(-0.213965833535144,0.00503082262064919,
-0.0101004046276131));
#38005=CARTESIAN_POINT('Ctrl Pts',(-0.213962869592426,0.00522461411188609,
-0.0101551540871568));
#38006=CARTESIAN_POINT('Ctrl Pts',(-0.213964007769243,0.00541871567763622,
-0.0102033520378653));
#38007=CARTESIAN_POINT('Ctrl Pts',(-0.213969011116721,0.00562297644438124,
-0.0102466576087607));
#38008=CARTESIAN_POINT('Ctrl Pts',(-0.21397151279046,0.00572510682775375,
-0.0102683103942083));
#38009=CARTESIAN_POINT('Ctrl Pts',(-0.213974983020484,0.00582980111776385,
-0.0102886361041918));
#38010=CARTESIAN_POINT('Ctrl Pts',(-0.213979254459626,0.00593296549140293,
-0.0103068209009627));
#38011=CARTESIAN_POINT('Ctrl Pts',(-0.213981390179197,0.00598454767822248,
-0.0103159132993481));
#38012=CARTESIAN_POINT('Ctrl Pts',(-0.21398372532838,0.00603573973725164,
-0.0103245105559012));
#38013=CARTESIAN_POINT('Ctrl Pts',(-0.213986547384677,0.00609134377532499,
-0.0103333119158729));
#38014=CARTESIAN_POINT('Ctrl Pts',(-0.213989369440973,0.00614694781339835,
-0.0103421132758447));
#38015=CARTESIAN_POINT('Ctrl Pts',(-0.213992681559152,0.00620698734528899,
-0.010350973822987));
#38016=CARTESIAN_POINT('Ctrl Pts',(-0.213995287493455,0.00625187779379209,
-0.0103572658605673));
#38017=CARTESIAN_POINT('Ctrl Pts',(-0.213997893427757,0.00629676824229519,
-0.0103635578981476));
#38018=CARTESIAN_POINT('Ctrl Pts',(-0.213999788731873,0.00632648178341135,
-0.0103674856704243));
#38019=CARTESIAN_POINT('Ctrl Pts',(-0.214002198062836,0.00636282859077894,
-0.0103721304048202));
#38020=CARTESIAN_POINT('Ctrl Pts',(-0.214004607393799,0.00639917539814654,
-0.0103767751392161));
#38021=CARTESIAN_POINT('Ctrl Pts',(-0.214007533141689,0.00644216866290085,
-0.0103820270457493));
#38022=CARTESIAN_POINT('Ctrl Pts',(-0.214010691369336,0.00648662577075809,
-0.0103870930993818));
#38023=CARTESIAN_POINT('Ctrl Pts',(-0.214017007824629,0.00657553998647256,
-0.0103972252066467));
#38024=CARTESIAN_POINT('Ctrl Pts',(-0.214024251660544,0.0066703007446929,
-0.0104067305057084));
#38025=CARTESIAN_POINT('Ctrl Pts',(-0.214032473075476,0.00677290354355626,
-0.0104151593879221));
#38026=CARTESIAN_POINT('Ctrl Pts',(-0.214040694490407,0.00687550634241962,
-0.0104235882701358));
#38027=CARTESIAN_POINT('Ctrl Pts',(-0.214049891976939,0.0069859388533199,
-0.0104310099796013));
#38028=CARTESIAN_POINT('Ctrl Pts',(-0.214060738298118,0.00711087507504844,
-0.0104366099394931));
#38029=CARTESIAN_POINT('Ctrl Pts',(-0.214071584619298,0.00723581129677699,
-0.0104422098993849));
#38030=CARTESIAN_POINT('Ctrl Pts',(-0.214084090997818,0.00737527186877879,
-0.0104454725859727));
#38031=CARTESIAN_POINT('Ctrl Pts',(-0.214095608115094,0.00750036597473118,
-0.0104457182539297));
#38032=CARTESIAN_POINT('',(-0.214184696860609,0.0122470177333751,-0.00910661628414272));
#38033=CARTESIAN_POINT('Ctrl Pts',(-0.214095608114984,0.00750036597474129,
-0.0104457182539273));
#38034=CARTESIAN_POINT('Ctrl Pts',(-0.214070334864979,0.00777590223793459,
-0.010445156937743));
#38035=CARTESIAN_POINT('Ctrl Pts',(-0.214049409271727,0.00801878429478129,
-0.010432220268336));
#38036=CARTESIAN_POINT('Ctrl Pts',(-0.214032886378828,0.00822460765478433,
-0.0104153680821803));
#38037=CARTESIAN_POINT('Ctrl Pts',(-0.214024624932379,0.00832751933478585,
-0.0104069419891024));
#38038=CARTESIAN_POINT('Ctrl Pts',(-0.214017463510113,0.008421166572945,
-0.0103975669167598));
#38039=CARTESIAN_POINT('Ctrl Pts',(-0.214011156716459,0.00850959622371078,
-0.0103875270045182));
#38040=CARTESIAN_POINT('Ctrl Pts',(-0.214008003319632,0.00855381104909367,
-0.0103825070483974));
#38041=CARTESIAN_POINT('Ctrl Pts',(-0.214005064359136,0.00859671801361874,
-0.0103772850899157));
#38042=CARTESIAN_POINT('Ctrl Pts',(-0.214002650767299,0.00863283383294724,
-0.0103726871256275));
#38043=CARTESIAN_POINT('Ctrl Pts',(-0.214000237175461,0.00866894965227573,
-0.0103680891613394));
#38044=CARTESIAN_POINT('Ctrl Pts',(-0.213998346489832,0.00869828797601001,
-0.0103642283066615));
#38045=CARTESIAN_POINT('Ctrl Pts',(-0.213995701917154,0.00874328117754318,
-0.0103579458563784));
#38046=CARTESIAN_POINT('Ctrl Pts',(-0.213993057344476,0.00878827437907636,
-0.0103516634060952));
#38047=CARTESIAN_POINT('Ctrl Pts',(-0.213989663478094,0.00884889382545365,
-0.0103427483596567));
#38048=CARTESIAN_POINT('Ctrl Pts',(-0.213986772711712,0.00890490784218023,
-0.0103339050625407));
#38049=CARTESIAN_POINT('Ctrl Pts',(-0.21398388194533,0.00896092185890681,
-0.0103250617654246));
#38050=CARTESIAN_POINT('Ctrl Pts',(-0.213981490994779,0.00901235485834678,
-0.0103164410798053));
#38051=CARTESIAN_POINT('Ctrl Pts',(-0.213979298224174,0.00906419019480051,
-0.0103073200461676));
#38052=CARTESIAN_POINT('Ctrl Pts',(-0.213974912682964,0.00916786086770796,
-0.0102890779788922));
#38053=CARTESIAN_POINT('Ctrl Pts',(-0.213971323529434,0.00927310895773648,
-0.0102686660302547));
#38054=CARTESIAN_POINT('Ctrl Pts',(-0.213968703904558,0.00937559067791705,
-0.0102469536514785));
#38055=CARTESIAN_POINT('Ctrl Pts',(-0.213963464654806,0.00958055411827819,
-0.0102035288939261));
#38056=CARTESIAN_POINT('Ctrl Pts',(-0.213962093405312,0.00977455790650294,
-0.0101553670319792));
#38057=CARTESIAN_POINT('Ctrl Pts',(-0.213964868649422,0.00996900504123913,
-0.0101004321413189));
#38058=CARTESIAN_POINT('Ctrl Pts',(-0.213967643893531,0.0101634521759753,
-0.0100454972506585));
#38059=CARTESIAN_POINT('Ctrl Pts',(-0.213974569916396,0.0103582714553616,
-0.00998359248621707));
#38060=CARTESIAN_POINT('Ctrl Pts',(-0.213986389893635,0.0105553207042468,
-0.00991337070712582));
#38061=CARTESIAN_POINT('Ctrl Pts',(-0.213992299882255,0.0106538453286895,
-0.00987825981758019));
#38062=CARTESIAN_POINT('Ctrl Pts',(-0.213999434474098,0.0107529130711297,
-0.00984101847227842));
#38063=CARTESIAN_POINT('Ctrl Pts',(-0.21400742187768,0.0108494164592589,
-0.00980285548237111));
#38064=CARTESIAN_POINT('Ctrl Pts',(-0.214011415579471,0.0108976681533235,
-0.00978377398741745));
#38065=CARTESIAN_POINT('Ctrl Pts',(-0.214015621743677,0.0109452914242763,
-0.00976449609826157));
#38066=CARTESIAN_POINT('Ctrl Pts',(-0.214020508513958,0.0109964792354597,
-0.00974322294100645));
#38067=CARTESIAN_POINT('Ctrl Pts',(-0.21402539528424,0.0110476670466431,
-0.00972194978375133));
#38068=CARTESIAN_POINT('Ctrl Pts',(-0.214030965417441,0.01110236730927,
-0.00969855471836265));
#38069=CARTESIAN_POINT('Ctrl Pts',(-0.214035309917913,0.0111434638323282,
-0.00968062761879806));
#38070=CARTESIAN_POINT('Ctrl Pts',(-0.214039654418384,0.0111845603553864,
-0.00966270051923346));
#38071=CARTESIAN_POINT('Ctrl Pts',(-0.214042769408935,0.0112121317202152,
-0.00965041949073069));
#38072=CARTESIAN_POINT('Ctrl Pts',(-0.214046641062954,0.0112455515375233,
-0.00963535490389684));
#38073=CARTESIAN_POINT('Ctrl Pts',(-0.214050512716972,0.0112789713548313,
-0.00962029031706299));
#38074=CARTESIAN_POINT('Ctrl Pts',(-0.214055143146001,0.0113181950816343,
-0.0096023451745143));
#38075=CARTESIAN_POINT('Ctrl Pts',(-0.214060047891704,0.0113584579042877,
-0.00958353178581492));
#38076=CARTESIAN_POINT('Ctrl Pts',(-0.214069857383109,0.0114389835495945,
-0.00954590500841617));
#38077=CARTESIAN_POINT('Ctrl Pts',(-0.214080761500679,0.0115237248101962,
-0.00950492654375179));
#38078=CARTESIAN_POINT('Ctrl Pts',(-0.214093129479694,0.0116157377101813,
-0.00945835647233302));
#38079=CARTESIAN_POINT('Ctrl Pts',(-0.214117865437726,0.0117997635101515,
-0.00936521632949548));
#38080=CARTESIAN_POINT('Ctrl Pts',(-0.214148458802816,0.0120128210029322,
-0.00924961966466249));
#38081=CARTESIAN_POINT('Ctrl Pts',(-0.214184696860609,0.0122470177333751,
-0.00910661628414272));
#38082=CARTESIAN_POINT('Ctrl Pts',(-0.214184729330674,0.0122470252836163,
-0.00910661235527564));
#38083=CARTESIAN_POINT('Ctrl Pts',(-0.213850288464871,0.0122469812246611,
-0.00909935897740313));
#38084=CARTESIAN_POINT('Ctrl Pts',(-0.213516684455692,0.0122469406317341,
-0.00909212168842724));
#38085=CARTESIAN_POINT('Ctrl Pts',(-0.213184287727917,0.0122469034874106,
-0.00908490856303434));
#38086=CARTESIAN_POINT('Origin',(-0.223675719604735,0.00750000372932125,
-0.00172559146420468));
#38087=CARTESIAN_POINT('',(-0.223392319497656,0.0131379432052361,-0.00865273962921209));
#38088=CARTESIAN_POINT('',(-0.223092851198727,0.00750411713615694,-0.0106501152360551));
#38089=CARTESIAN_POINT('Ctrl Pts',(-0.223392319497656,0.0131379432052361,
-0.00865273962921209));
#38090=CARTESIAN_POINT('Ctrl Pts',(-0.223319870738354,0.0128800952029135,
-0.00886095679640992));
#38091=CARTESIAN_POINT('Ctrl Pts',(-0.223230386950221,0.0125275741399707,
-0.00911169714258552));
#38092=CARTESIAN_POINT('Ctrl Pts',(-0.223144924851994,0.0121246045072842,
-0.00936277629811845));
#38093=CARTESIAN_POINT('Ctrl Pts',(-0.223105570798993,0.0119109143796109,
-0.0094873958280264));
#38094=CARTESIAN_POINT('Ctrl Pts',(-0.223059101856131,0.0115847145998169,
-0.00966392505257264));
#38095=CARTESIAN_POINT('Ctrl Pts',(-0.223024275136112,0.011255422652783,
-0.00982367547305012));
#38096=CARTESIAN_POINT('Ctrl Pts',(-0.22299626632418,0.0108976150018631,
-0.00998025904879322));
#38097=CARTESIAN_POINT('Ctrl Pts',(-0.222969189537975,0.0103675478402047,
-0.0101824958926781));
#38098=CARTESIAN_POINT('Ctrl Pts',(-0.222960837342892,0.00989357905788291,
-0.0103271516041799));
#38099=CARTESIAN_POINT('Ctrl Pts',(-0.222966854203074,0.0094544751161954,
-0.0104324699590511));
#38100=CARTESIAN_POINT('Ctrl Pts',(-0.222973927346185,0.00921413881180308,
-0.0104823626331397));
#38101=CARTESIAN_POINT('Ctrl Pts',(-0.222982423102499,0.00900963355855106,
-0.0105197667134106));
#38102=CARTESIAN_POINT('Ctrl Pts',(-0.222988265756248,0.00889796473082585,
-0.0105380791660538));
#38103=CARTESIAN_POINT('Ctrl Pts',(-0.223000296289551,0.00869011684464469,
-0.0105697181567833));
#38104=CARTESIAN_POINT('Ctrl Pts',(-0.22302756304511,0.00828858110951311,
-0.0106196678946535));
#38105=CARTESIAN_POINT('Ctrl Pts',(-0.223063364931254,0.00784225216468286,
-0.0106493264355849));
#38106=CARTESIAN_POINT('Ctrl Pts',(-0.223092851198727,0.00750411713615694,
-0.0106501152360551));
#38107=CARTESIAN_POINT('',(-0.223398276290135,0.00187668424502486,-0.00866473290108311));
#38108=CARTESIAN_POINT('Ctrl Pts',(-0.223092851083271,0.00750411580413045,
-0.0106501152341876));
#38109=CARTESIAN_POINT('Ctrl Pts',(-0.223087327232776,0.00744038676315757,
-0.0106500258777345));
#38110=CARTESIAN_POINT('Ctrl Pts',(-0.223070830151961,0.0072462764610065,
-0.0106473681726595));
#38111=CARTESIAN_POINT('Ctrl Pts',(-0.223046896389284,0.00695246582810878,
-0.0106342335993294));
#38112=CARTESIAN_POINT('Ctrl Pts',(-0.223020042570552,0.0065999218171742,
-0.0106059269867326));
#38113=CARTESIAN_POINT('Ctrl Pts',(-0.22300100412444,0.00631589831769131,
-0.0105704887939461));
#38114=CARTESIAN_POINT('Ctrl Pts',(-0.222989208447741,0.00610913959330224,
-0.0105392233303175));
#38115=CARTESIAN_POINT('Ctrl Pts',(-0.222983537274156,0.00599855057050103,
-0.0105211674311498));
#38116=CARTESIAN_POINT('Ctrl Pts',(-0.222975416165749,0.0057972222654291,
-0.0104845864027248));
#38117=CARTESIAN_POINT('Ctrl Pts',(-0.222968660064301,0.00555785014105163,
-0.0104352496583974));
#38118=CARTESIAN_POINT('Ctrl Pts',(-0.222963230580807,0.00512057842839108,
-0.0103310664826879));
#38119=CARTESIAN_POINT('Ctrl Pts',(-0.222972107074572,0.00464542086187804,
-0.0101870267964044));
#38120=CARTESIAN_POINT('Ctrl Pts',(-0.222999678112803,0.00411212165983419,
-0.00998434144011729));
#38121=CARTESIAN_POINT('Ctrl Pts',(-0.223027825900457,0.00375402649109574,
-0.00982811005214637));
#38122=CARTESIAN_POINT('Ctrl Pts',(-0.223062687117585,0.00342540405800575,
-0.00966912797513253));
#38123=CARTESIAN_POINT('Ctrl Pts',(-0.223108723891955,0.00310293757098118,
-0.0094952680541608));
#38124=CARTESIAN_POINT('Ctrl Pts',(-0.223148477674354,0.00288825845475733,
-0.00937061521761407));
#38125=CARTESIAN_POINT('Ctrl Pts',(-0.223234583481303,0.00248626659602517,
-0.0091211101373121));
#38126=CARTESIAN_POINT('Ctrl Pts',(-0.223325021475566,0.00213415979343589,
-0.00887172811568694));
#38127=CARTESIAN_POINT('Ctrl Pts',(-0.223398276290135,0.00187668424502486,
-0.00866473290108311));
#38128=CARTESIAN_POINT('',(-0.224398147996022,0.00187716923648251,-0.0086866135867605));
#38129=CARTESIAN_POINT('Ctrl Pts',(-0.223398267584606,0.0018766830097055,
-0.00866473171331845));
#38130=CARTESIAN_POINT('Ctrl Pts',(-0.223731547637729,0.00187684536702503,
-0.00867202562098763));
#38131=CARTESIAN_POINT('Ctrl Pts',(-0.224064903826057,0.00187700183853765,
-0.00867931638700321));
#38132=CARTESIAN_POINT('Ctrl Pts',(-0.224398132591523,0.00187715232727695,
-0.00868659956029552));
#38133=CARTESIAN_POINT('',(-0.224092577864133,0.00750459921737242,-0.0106715875712242));
#38134=CARTESIAN_POINT('Ctrl Pts',(-0.224398147996022,0.00187716923648251,
-0.0086866135867605));
#38135=CARTESIAN_POINT('Ctrl Pts',(-0.224324606355394,0.00213579320645476,
-0.00889450206705218));
#38136=CARTESIAN_POINT('Ctrl Pts',(-0.224233796543426,0.00248988624564132,
-0.00914510760840042));
#38137=CARTESIAN_POINT('Ctrl Pts',(-0.224147406194117,0.00289433113124562,
-0.00939577762286241));
#38138=CARTESIAN_POINT('Ctrl Pts',(-0.224107349701666,0.00311189725424205,
-0.00952178404242857));
#38139=CARTESIAN_POINT('Ctrl Pts',(-0.224061875704077,0.00343247296487068,
-0.00969417693164834));
#38140=CARTESIAN_POINT('Ctrl Pts',(-0.224027253567691,0.00376014454372357,
-0.00985239135964685));
#38141=CARTESIAN_POINT('Ctrl Pts',(-0.223999340389896,0.00411678701536448,
-0.0100076863622763));
#38142=CARTESIAN_POINT('Ctrl Pts',(-0.223971952688012,0.0046474445615379,
-0.0102091401480788));
#38143=CARTESIAN_POINT('Ctrl Pts',(-0.223963070619058,0.00512398064154051,
-0.0103535176057558));
#38144=CARTESIAN_POINT('Ctrl Pts',(-0.223968602205114,0.00556175319243944,
-0.0104576018845324));
#38145=CARTESIAN_POINT('Ctrl Pts',(-0.223975415699836,0.0058015783603966,
-0.0105069145861535));
#38146=CARTESIAN_POINT('Ctrl Pts',(-0.223983597663641,0.00600344362452778,
-0.0105434921756839));
#38147=CARTESIAN_POINT('Ctrl Pts',(-0.223989361337856,0.00611564279954052,
-0.0105617243244171));
#38148=CARTESIAN_POINT('Ctrl Pts',(-0.224001170014523,0.00632279525898115,
-0.0105929495573639));
#38149=CARTESIAN_POINT('Ctrl Pts',(-0.224020493150551,0.00661020725445457,
-0.0106281277231074));
#38150=CARTESIAN_POINT('Ctrl Pts',(-0.224046205769023,0.0069490878284383,
-0.0106560024836772));
#38151=CARTESIAN_POINT('Ctrl Pts',(-0.224072028233643,0.00726436926979324,
-0.0106689252057769));
#38152=CARTESIAN_POINT('Ctrl Pts',(-0.2240842252329,0.00740810682501627,
-0.010671457912672));
#38153=CARTESIAN_POINT('Ctrl Pts',(-0.224092577864133,0.00750459921737242,
-0.0106715875712242));
#38154=CARTESIAN_POINT('',(-0.224391717827447,0.0131382574628826,-0.00867393727785756));
#38155=CARTESIAN_POINT('Ctrl Pts',(-0.224092578003526,0.00750460082767304,
-0.0106715875733879));
#38156=CARTESIAN_POINT('Ctrl Pts',(-0.22406295489172,0.00784473299941522,
-0.010670775927101));
#38157=CARTESIAN_POINT('Ctrl Pts',(-0.224027030414954,0.00829347663740902,
-0.0106407627709499));
#38158=CARTESIAN_POINT('Ctrl Pts',(-0.223999740369017,0.008697043734868,
-0.0105902556410251));
#38159=CARTESIAN_POINT('Ctrl Pts',(-0.223987747099335,0.00890554018645671,
-0.0105583463523279));
#38160=CARTESIAN_POINT('Ctrl Pts',(-0.223981909747232,0.00901824998727424,
-0.010539746396188));
#38161=CARTESIAN_POINT('Ctrl Pts',(-0.223973591662315,0.00922104189434486,
-0.0105024653322432));
#38162=CARTESIAN_POINT('Ctrl Pts',(-0.223966650813448,0.0094600836684451,
-0.0104526716603005));
#38163=CARTESIAN_POINT('Ctrl Pts',(-0.22396082625537,0.00989692323941784,
-0.0103475911356174));
#38164=CARTESIAN_POINT('Ctrl Pts',(-0.2239690669497,0.0103666723157455,
-0.0102042766054829));
#38165=CARTESIAN_POINT('Ctrl Pts',(-0.223996160315981,0.0108988366543281,
-0.0100012575347548));
#38166=CARTESIAN_POINT('Ctrl Pts',(-0.22402419040041,0.0112571751904465,
-0.00984433623679992));
#38167=CARTESIAN_POINT('Ctrl Pts',(-0.224059042622487,0.0115869929132631,
-0.00968423835129144));
#38168=CARTESIAN_POINT('Ctrl Pts',(-0.224105611700866,0.011913804457731,
-0.00950722646718586));
#38169=CARTESIAN_POINT('Ctrl Pts',(-0.224144860648786,0.012126837978164,
-0.00938288306593188));
#38170=CARTESIAN_POINT('Ctrl Pts',(-0.224230166524884,0.012529155718252,
-0.0091320634968813));
#38171=CARTESIAN_POINT('Ctrl Pts',(-0.224319441634422,0.0128809283761845,
-0.00888175630073892));
#38172=CARTESIAN_POINT('Ctrl Pts',(-0.224391717827447,0.0131382574628826,
-0.00867393727785756));
#38173=CARTESIAN_POINT('Ctrl Pts',(-0.224391700636746,0.013138269070805,
-0.00867392746427423));
#38174=CARTESIAN_POINT('Ctrl Pts',(-0.224058345684202,0.0131381552026779,
-0.00866686423347615));
#38175=CARTESIAN_POINT('Ctrl Pts',(-0.223725131075681,0.0131380471806954,
-0.00865979925365354));
#38176=CARTESIAN_POINT('Ctrl Pts',(-0.223392308938441,0.0131379450563949,
-0.00865273789653389));
#38177=CARTESIAN_POINT('Origin',(-0.211568189915785,0.00750000024019488,
-0.00128323523926141));
#38178=CARTESIAN_POINT('',(-0.21118342070055,0.0122493195087978,-0.009043325341704));
#38179=CARTESIAN_POINT('',(-0.211096534876114,0.00750002174791387,-0.0103787794824388));
#38180=CARTESIAN_POINT('Ctrl Pts',(-0.21118342070055,0.0122493195087978,
-0.009043325341704));
#38181=CARTESIAN_POINT('Ctrl Pts',(-0.211147075853411,0.0120146153758137,
-0.00918609110004283));
#38182=CARTESIAN_POINT('Ctrl Pts',(-0.211101126056254,0.0116945334709256,
-0.00935899282289318));
#38183=CARTESIAN_POINT('Ctrl Pts',(-0.211063031695026,0.0113977919415671,
-0.00950208910682082));
#38184=CARTESIAN_POINT('Ctrl Pts',(-0.211044625840369,0.0112410518606829,
-0.0095734525507458));
#38185=CARTESIAN_POINT('Ctrl Pts',(-0.211035314537477,0.0111580846306274,
-0.00961034898322537));
#38186=CARTESIAN_POINT('Ctrl Pts',(-0.211018942999683,0.0109956430019049,
-0.00967965113480102));
#38187=CARTESIAN_POINT('Ctrl Pts',(-0.211002445396812,0.0108059307774903,
-0.00975612785596291));
#38188=CARTESIAN_POINT('Ctrl Pts',(-0.210978052341354,0.0104602185049158,
-0.00988599885738961));
#38189=CARTESIAN_POINT('Ctrl Pts',(-0.210961408558488,0.0099657835293919,
-0.0100422465505005));
#38190=CARTESIAN_POINT('Ctrl Pts',(-0.21096547560556,0.00948426681055532,
-0.0101613871041555));
#38191=CARTESIAN_POINT('Ctrl Pts',(-0.210978341736303,0.00911600746241873,
-0.0102326044618298));
#38192=CARTESIAN_POINT('Ctrl Pts',(-0.210988044352495,0.00891043600357915,
-0.0102670716292219));
#38193=CARTESIAN_POINT('Ctrl Pts',(-0.210998326477394,0.00872874261242559,
-0.0102936849955648));
#38194=CARTESIAN_POINT('Ctrl Pts',(-0.211004044914085,0.00864037334831602,
-0.0103052055025708));
#38195=CARTESIAN_POINT('Ctrl Pts',(-0.211015798923584,0.00846851034186375,
-0.0103261628486553));
#38196=CARTESIAN_POINT('Ctrl Pts',(-0.21104070236026,0.00814026567965264,
-0.0103588017271737));
#38197=CARTESIAN_POINT('Ctrl Pts',(-0.211071667771316,0.00777569081607782,
-0.0103782378584628));
#38198=CARTESIAN_POINT('Ctrl Pts',(-0.211096534876114,0.00750002174791387,
-0.0103787794824388));
#38199=CARTESIAN_POINT('',(-0.211184192776991,0.00275281494927484,-0.00904464640986752));
#38200=CARTESIAN_POINT('Ctrl Pts',(-0.211096534773062,0.00750002061052517,
-0.0103787794801929));
#38201=CARTESIAN_POINT('Ctrl Pts',(-0.211096372089148,0.00749822498476027,
-0.0103787759245625));
#38202=CARTESIAN_POINT('Ctrl Pts',(-0.211091269818405,0.00744179752197237,
-0.010378568095464));
#38203=CARTESIAN_POINT('Ctrl Pts',(-0.211086202258332,0.00738520865215235,
-0.0103778882206662));
#38204=CARTESIAN_POINT('Ctrl Pts',(-0.211075357694199,0.00726324121015861,
-0.0103757196011447));
#38205=CARTESIAN_POINT('Ctrl Pts',(-0.211062090540266,0.00711042797893358,
-0.0103702493396725));
#38206=CARTESIAN_POINT('Ctrl Pts',(-0.211047251633211,0.00693429006983655,
-0.0103606551626359));
#38207=CARTESIAN_POINT('Ctrl Pts',(-0.211029718484758,0.00671798930303775,
-0.0103446970608107));
#38208=CARTESIAN_POINT('Ctrl Pts',(-0.211015469076438,0.00653052937502733,
-0.0103260547268499));
#38209=CARTESIAN_POINT('Ctrl Pts',(-0.211003724232673,0.00635858874913573,
-0.0103050683605631));
#38210=CARTESIAN_POINT('Ctrl Pts',(-0.210998005903544,0.00626993368874563,
-0.010293494688143));
#38211=CARTESIAN_POINT('Ctrl Pts',(-0.210987839649527,0.00608916568458587,
-0.010266999569767));
#38212=CARTESIAN_POINT('Ctrl Pts',(-0.210978254538632,0.00588405688678575,
-0.0102326085786644));
#38213=CARTESIAN_POINT('Ctrl Pts',(-0.210965627361286,0.00551657670016644,
-0.0101615840585635));
#38214=CARTESIAN_POINT('Ctrl Pts',(-0.210961985602812,0.00503295150595074,
-0.0100418962433909));
#38215=CARTESIAN_POINT('Ctrl Pts',(-0.210978985441477,0.00454104539977056,
-0.00988643540233352));
#38216=CARTESIAN_POINT('Ctrl Pts',(-0.211003574831235,0.00419499500178585,
-0.00975651549375403));
#38217=CARTESIAN_POINT('Ctrl Pts',(-0.21102015926641,0.00400507401732748,
-0.00967997805343405));
#38218=CARTESIAN_POINT('Ctrl Pts',(-0.211036621559236,0.00384205348628263,
-0.00961043850454111));
#38219=CARTESIAN_POINT('Ctrl Pts',(-0.211045891149871,0.00375951174937592,
-0.00957373108287534));
#38220=CARTESIAN_POINT('Ctrl Pts',(-0.211064262875409,0.00360301705517485,
-0.00950249609276564));
#38221=CARTESIAN_POINT('Ctrl Pts',(-0.211102233289035,0.00330686034690693,
-0.009359722009264));
#38222=CARTESIAN_POINT('Ctrl Pts',(-0.211148004045778,0.00298722410298725,
-0.00918714660229151));
#38223=CARTESIAN_POINT('Ctrl Pts',(-0.211184192776991,0.00275281494927484,
-0.00904464640986752));
#38224=CARTESIAN_POINT('',(-0.212184966502507,0.00275261962744201,-0.009066300433649));
#38225=CARTESIAN_POINT('Ctrl Pts',(-0.211184242601052,0.00275281783271421,
-0.00904464925643142));
#38226=CARTESIAN_POINT('Ctrl Pts',(-0.211517534893567,0.00275275115143515,
-0.00905185979923313));
#38227=CARTESIAN_POINT('Ctrl Pts',(-0.211851205378944,0.00275268083048704,
-0.00905907634424748));
#38228=CARTESIAN_POINT('Ctrl Pts',(-0.212185002205565,0.00275260690551022,
-0.00906629343342788));
#38229=CARTESIAN_POINT('',(-0.212096215740483,0.00750006061885404,-0.0104005278051053));
#38230=CARTESIAN_POINT('Ctrl Pts',(-0.212184966502507,0.00275261962744201,
-0.009066300433649));
#38231=CARTESIAN_POINT('Ctrl Pts',(-0.212148608821063,0.00298809828782967,
-0.00920945875312566));
#38232=CARTESIAN_POINT('Ctrl Pts',(-0.212117948616956,0.00320218746771227,
-0.00932506036133119));
#38233=CARTESIAN_POINT('Ctrl Pts',(-0.212093184999995,0.00338706586627467,
-0.00941816979041781));
#38234=CARTESIAN_POINT('Ctrl Pts',(-0.212080803191514,0.00347950506555587,
-0.00946472450496112));
#38235=CARTESIAN_POINT('Ctrl Pts',(-0.212069895077993,0.00356462887386294,
-0.00950567694212421));
#38236=CARTESIAN_POINT('Ctrl Pts',(-0.212060103592096,0.00364539886507545,
-0.00954322274361884));
#38237=CARTESIAN_POINT('Ctrl Pts',(-0.212055207849147,0.0036857838606817,
-0.00956199564436615));
#38238=CARTESIAN_POINT('Ctrl Pts',(-0.212050591906104,0.00372509475974982,
-0.00957988733157869));
#38239=CARTESIAN_POINT('Ctrl Pts',(-0.21204672334139,0.00375869560595558,
-0.00959495384536575));
#38240=CARTESIAN_POINT('Ctrl Pts',(-0.212042854776675,0.00379229645216134,
-0.00961002035915281));
#38241=CARTESIAN_POINT('Ctrl Pts',(-0.212039731540024,0.00382014420653861,
-0.00962235593746418));
#38242=CARTESIAN_POINT('Ctrl Pts',(-0.21203543633928,0.0038610821910094,
-0.00964011866024805));
#38243=CARTESIAN_POINT('Ctrl Pts',(-0.212031141138537,0.00390202017548019,
-0.00965788138303192));
#38244=CARTESIAN_POINT('Ctrl Pts',(-0.212025677698956,0.00395612350844896,
-0.00968090002320027));
#38245=CARTESIAN_POINT('Ctrl Pts',(-0.212020875548343,0.0040068650364192,
-0.00970188426642679));
#38246=CARTESIAN_POINT('Ctrl Pts',(-0.21201607339773,0.00405760656438943,
-0.00972286850965331));
#38247=CARTESIAN_POINT('Ctrl Pts',(-0.212011929909662,0.00410493688815609,
-0.00974193907695546));
#38248=CARTESIAN_POINT('Ctrl Pts',(-0.212007996642503,0.00415289807641202,
-0.00976081980110558));
#38249=CARTESIAN_POINT('Ctrl Pts',(-0.212000130108185,0.00424882045292389,
-0.00979858124940582));
#38250=CARTESIAN_POINT('Ctrl Pts',(-0.211993107258692,0.00434731387725675,
-0.00983545457074571));
#38251=CARTESIAN_POINT('Ctrl Pts',(-0.21198728236806,0.00444547316953737,
-0.00987029799021983));
#38252=CARTESIAN_POINT('Ctrl Pts',(-0.211975632586797,0.00464179175409861,
-0.00993998482916808));
#38253=CARTESIAN_POINT('Ctrl Pts',(-0.211968770979782,0.00483672941011492,
-0.0100017203464364));
#38254=CARTESIAN_POINT('Ctrl Pts',(-0.211966011865899,0.00503103822754167,
-0.0100564228393022));
#38255=CARTESIAN_POINT('Ctrl Pts',(-0.211963252752017,0.00522534704496841,
-0.010111125332168));
#38256=CARTESIAN_POINT('Ctrl Pts',(-0.211964591385878,0.00541895104039878,
-0.0101590129190598));
#38257=CARTESIAN_POINT('Ctrl Pts',(-0.211969770051672,0.00562307980497558,
-0.0102021454556335));
#38258=CARTESIAN_POINT('Ctrl Pts',(-0.211972359384569,0.00572514418726399,
-0.0102237117239204));
#38259=CARTESIAN_POINT('Ctrl Pts',(-0.211975911186776,0.00582986526912701,
-0.0102439760950727));
#38260=CARTESIAN_POINT('Ctrl Pts',(-0.211980255990761,0.00593300677166175,
-0.0102620974047736));
#38261=CARTESIAN_POINT('Ctrl Pts',(-0.211982428392754,0.00598457752292912,
-0.010271158059624));
#38262=CARTESIAN_POINT('Ctrl Pts',(-0.211984798161859,0.00603574571201802,
-0.0102797235514748));
#38263=CARTESIAN_POINT('Ctrl Pts',(-0.211987658262279,0.00609135335842438,
-0.0102884971298513));
#38264=CARTESIAN_POINT('Ctrl Pts',(-0.211990518362698,0.00614696100483073,
-0.0102972707082277));
#38265=CARTESIAN_POINT('Ctrl Pts',(-0.211993871951416,0.00620703157474658,
-0.0103061072618912));
#38266=CARTESIAN_POINT('Ctrl Pts',(-0.211996503008621,0.00625191141560677,
-0.0103123775364578));
#38267=CARTESIAN_POINT('Ctrl Pts',(-0.211999134065825,0.00629679125646696,
-0.0103186478110244));
#38268=CARTESIAN_POINT('Ctrl Pts',(-0.212001038147609,0.00632645261086889,
-0.0103225560719346));
#38269=CARTESIAN_POINT('Ctrl Pts',(-0.21200345637053,0.00636279070500133,
-0.0103271848758392));
#38270=CARTESIAN_POINT('Ctrl Pts',(-0.212005874593451,0.00639912879913378,
-0.0103318136797438));
#38271=CARTESIAN_POINT('Ctrl Pts',(-0.212008809361001,0.00644215698030905,
-0.0103370525494413));
#38272=CARTESIAN_POINT('Ctrl Pts',(-0.212011958500563,0.00648652347538562,
-0.0103420922865668));
#38273=CARTESIAN_POINT('Ctrl Pts',(-0.212018256779686,0.00657525646553876,
-0.0103521717608177));
#38274=CARTESIAN_POINT('Ctrl Pts',(-0.212025409498654,0.00666932914028881,
-0.0103615948168621));
#38275=CARTESIAN_POINT('Ctrl Pts',(-0.212033655768505,0.00677269298518827,
-0.0103700605683433));
#38276=CARTESIAN_POINT('Ctrl Pts',(-0.212050148308207,0.00697942067498721,
-0.0103869920713057));
#38277=CARTESIAN_POINT('Ctrl Pts',(-0.212071017506775,0.00722331365218771,
-0.0103999814945091));
#38278=CARTESIAN_POINT('Ctrl Pts',(-0.212096215740485,0.00750006061883522,
-0.0104005278051053));
#38279=CARTESIAN_POINT('',(-0.212183785378815,0.0122487124732956,-0.0090654584774169));
#38280=CARTESIAN_POINT('Ctrl Pts',(-0.212096215740483,0.00750006061885404,
-0.0104005278051053));
#38281=CARTESIAN_POINT('Ctrl Pts',(-0.212071084803046,0.00777720907168359,
-0.0103999791884765));
#38282=CARTESIAN_POINT('Ctrl Pts',(-0.212050255631567,0.00802145530645392,
-0.0103869514333805));
#38283=CARTESIAN_POINT('Ctrl Pts',(-0.212033775329214,0.00822850316358781,
-0.0103699670068986));
#38284=CARTESIAN_POINT('Ctrl Pts',(-0.212025535178038,0.00833202709215476,
-0.0103614747936577));
#38285=CARTESIAN_POINT('Ctrl Pts',(-0.212018381635708,0.00842625156415626,
-0.0103520213798588));
#38286=CARTESIAN_POINT('Ctrl Pts',(-0.212012075565743,0.00851511137322495,
-0.0103419112432895));
#38287=CARTESIAN_POINT('Ctrl Pts',(-0.21200892253076,0.00855954127775929,
-0.0103368561750048));
#38288=CARTESIAN_POINT('Ctrl Pts',(-0.212005982124083,0.00860262662677667,
-0.0103316019817392));
#38289=CARTESIAN_POINT('Ctrl Pts',(-0.212003556482991,0.00863903890015032,
-0.010326956172219));
#38290=CARTESIAN_POINT('Ctrl Pts',(-0.212001130841899,0.00867545117352398,
-0.0103223103626988));
#38291=CARTESIAN_POINT('Ctrl Pts',(-0.211999217569435,0.00870520370405761,
-0.0103183831165034));
#38292=CARTESIAN_POINT('Ctrl Pts',(-0.211996575654735,0.00875009675291833,
-0.0103121005759226));
#38293=CARTESIAN_POINT('Ctrl Pts',(-0.211993933740034,0.00879498980177905,
-0.0103058180353417));
#38294=CARTESIAN_POINT('Ctrl Pts',(-0.211990567611169,0.00885499566654293,
-0.0102969766573737));
#38295=CARTESIAN_POINT('Ctrl Pts',(-0.211987691838397,0.00891053313075946,
-0.0102882017827607));
#38296=CARTESIAN_POINT('Ctrl Pts',(-0.211984816065626,0.00896607059497598,
-0.0102794269081478));
#38297=CARTESIAN_POINT('Ctrl Pts',(-0.211982427503353,0.00901716305253132,
-0.0102708631292185));
#38298=CARTESIAN_POINT('Ctrl Pts',(-0.211980234043084,0.00906865320441798,
-0.0102618062674016));
#38299=CARTESIAN_POINT('Ctrl Pts',(-0.211975847122544,0.00917163350819128,
-0.0102436925437678));
#38300=CARTESIAN_POINT('Ctrl Pts',(-0.211972244195427,0.00927617380797614,
-0.0102234416789181));
#38301=CARTESIAN_POINT('Ctrl Pts',(-0.211969587228889,0.00937781729810693,
-0.0102019519260732));
#38302=CARTESIAN_POINT('Ctrl Pts',(-0.211964273295813,0.00958110427836849,
-0.0101589724203835));
#38303=CARTESIAN_POINT('Ctrl Pts',(-0.211962731868439,0.00977291813170571,
-0.0101115584715891));
#38304=CARTESIAN_POINT('Ctrl Pts',(-0.211965304925825,0.00996713451424829,
-0.0100569216533234));
#38305=CARTESIAN_POINT('Ctrl Pts',(-0.211967877983211,0.0101613508967909,
-0.0100022848350576));
#38306=CARTESIAN_POINT('Ctrl Pts',(-0.211974572774418,0.0103578615668069,
-0.00994009192707719));
#38307=CARTESIAN_POINT('Ctrl Pts',(-0.211986103882925,0.010554810494706,
-0.00987017052721041));
#38308=CARTESIAN_POINT('Ctrl Pts',(-0.211991869437178,0.0106532849586555,
-0.00983520982727702));
#38309=CARTESIAN_POINT('Ctrl Pts',(-0.211998844621251,0.0107518644913665,
-0.00979829169999918));
#38310=CARTESIAN_POINT('Ctrl Pts',(-0.212006673594954,0.010847876094752,
-0.00976048395358538));
#38311=CARTESIAN_POINT('Ctrl Pts',(-0.212010588081806,0.0108958818964447,
-0.00974158008037848));
#38312=CARTESIAN_POINT('Ctrl Pts',(-0.212014715332133,0.0109432572343657,
-0.00972248524111358));
#38313=CARTESIAN_POINT('Ctrl Pts',(-0.212019502672067,0.0109940178498293,
-0.00970148646569386));
#38314=CARTESIAN_POINT('Ctrl Pts',(-0.212024290012001,0.0110447784652929,
-0.00968048769027414));
#38315=CARTESIAN_POINT('Ctrl Pts',(-0.212029740059852,0.0110988751152101,
-0.0096574646208909));
#38316=CARTESIAN_POINT('Ctrl Pts',(-0.212034028469476,0.0111398206347841,
-0.00963969316884266));
#38317=CARTESIAN_POINT('Ctrl Pts',(-0.212038316879101,0.011180766154358,
-0.00962192171679442));
#38318=CARTESIAN_POINT('Ctrl Pts',(-0.212041439931195,0.0112086355631204,
-0.00960957285060339));
#38319=CARTESIAN_POINT('Ctrl Pts',(-0.212045308690276,0.0112422548710201,
-0.00959449336407188));
#38320=CARTESIAN_POINT('Ctrl Pts',(-0.212049177449357,0.0112758741789197,
-0.00957941387754037));
#38321=CARTESIAN_POINT('Ctrl Pts',(-0.212053793964691,0.0113152003528337,
-0.00956150957010244));
#38322=CARTESIAN_POINT('Ctrl Pts',(-0.212058692181928,0.0113556016114075,
-0.00954272312340504));
#38323=CARTESIAN_POINT('Ctrl Pts',(-0.2120684886164,0.011436404128555,-0.00950515023001024));
#38324=CARTESIAN_POINT('Ctrl Pts',(-0.212079409287647,0.0115215644114706,
-0.00946416695603335));
#38325=CARTESIAN_POINT('Ctrl Pts',(-0.212091810164631,0.0116140405560105,
-0.0094175780460792));
#38326=CARTESIAN_POINT('Ctrl Pts',(-0.212116611918599,0.0117989928450904,
-0.00932440022617091));
#38327=CARTESIAN_POINT('Ctrl Pts',(-0.212147336299191,0.0120131578667162,
-0.00920871694976559));
#38328=CARTESIAN_POINT('Ctrl Pts',(-0.212183785378815,0.0122487124732956,
-0.0090654584774169));
#38329=CARTESIAN_POINT('Ctrl Pts',(-0.21218382236874,0.0122487203634196,
-0.00906545445695096));
#38330=CARTESIAN_POINT('Ctrl Pts',(-0.211850415340402,0.0122489172355382,
-0.00905808114379708));
#38331=CARTESIAN_POINT('Ctrl Pts',(-0.211516897126879,0.0122491175732441,
-0.0090507032823604));
#38332=CARTESIAN_POINT('Ctrl Pts',(-0.211183475876664,0.0122493212504455,
-0.00904332547672575));
#38333=CARTESIAN_POINT('Origin',(-0.201568762588454,0.00750000073597594,
-0.000898605665389165));
#38334=CARTESIAN_POINT('',(-0.201180432939979,0.0122595231330948,-0.00883793092373448));
#38335=CARTESIAN_POINT('',(-0.201099841269113,0.00750066886075073,-0.0101529052291387));
#38336=CARTESIAN_POINT('Ctrl Pts',(-0.201180432939979,0.0122595231330948,
-0.00883793092373448));
#38337=CARTESIAN_POINT('Ctrl Pts',(-0.201143740554226,0.0120228137257047,
-0.00897895597246862));
#38338=CARTESIAN_POINT('Ctrl Pts',(-0.20109822872155,0.0117071699584008,
-0.00914678199504796));
#38339=CARTESIAN_POINT('Ctrl Pts',(-0.20105352550923,0.0113497843899364,
-0.00931471227512171));
#38340=CARTESIAN_POINT('Ctrl Pts',(-0.201033187159162,0.0111728352939134,
-0.00939335080989536));
#38341=CARTESIAN_POINT('Ctrl Pts',(-0.201004811740894,0.0108597897901084,
-0.00952200041603991));
#38342=CARTESIAN_POINT('Ctrl Pts',(-0.200980796925748,0.0104817056607582,
-0.00966132613367734));
#38343=CARTESIAN_POINT('Ctrl Pts',(-0.200965879775637,0.00995831253814996,
-0.00982474718393346));
#38344=CARTESIAN_POINT('Ctrl Pts',(-0.200972104318261,0.00949743717135199,
-0.00993630501398072));
#38345=CARTESIAN_POINT('Ctrl Pts',(-0.200985841120966,0.00912458516838106,
-0.0100078469251149));
#38346=CARTESIAN_POINT('Ctrl Pts',(-0.200995917543769,0.00891603011605418,
-0.0100423599010609));
#38347=CARTESIAN_POINT('Ctrl Pts',(-0.201006511373127,0.00872931824135355,
-0.0100692983593163));
#38348=CARTESIAN_POINT('Ctrl Pts',(-0.201012139020932,0.00864096664753087,
-0.0100806012456826));
#38349=CARTESIAN_POINT('Ctrl Pts',(-0.201023644166776,0.00846779200223077,
-0.0101013573951201));
#38350=CARTESIAN_POINT('Ctrl Pts',(-0.201047512603945,0.00813892243805578,
-0.0101334243263926));
#38351=CARTESIAN_POINT('Ctrl Pts',(-0.201076639535349,0.00777509809593754,
-0.0101523824149227));
#38352=CARTESIAN_POINT('Ctrl Pts',(-0.20109984171623,0.00750066914084511,
-0.0101529052406882));
#38353=CARTESIAN_POINT('',(-0.201177675620458,0.00274510091024268,-0.00884063751610791));
#38354=CARTESIAN_POINT('Ctrl Pts',(-0.201099841689236,0.00750066882484645,
-0.0101529052401256));
#38355=CARTESIAN_POINT('Ctrl Pts',(-0.201097897029398,0.00747790081601996,
-0.0101528647152854));
#38356=CARTESIAN_POINT('Ctrl Pts',(-0.201090755424158,0.00739389932697868,
-0.0101523381855469));
#38357=CARTESIAN_POINT('Ctrl Pts',(-0.201080428616844,0.0072706848013662,
-0.0101499681004645));
#38358=CARTESIAN_POINT('Ctrl Pts',(-0.201062017942989,0.00704727154987918,
-0.0101425305811733));
#38359=CARTESIAN_POINT('Ctrl Pts',(-0.201040076465639,0.0067682941608778,
-0.0101242894215651));
#38360=CARTESIAN_POINT('Ctrl Pts',(-0.201022784868407,0.0065326874925701,
-0.0101013964972095));
#38361=CARTESIAN_POINT('Ctrl Pts',(-0.201011167483721,0.00635960375819356,
-0.0100806496042055));
#38362=CARTESIAN_POINT('Ctrl Pts',(-0.20100547097909,0.00627106324120422,
-0.0100693241425073));
#38363=CARTESIAN_POINT('Ctrl Pts',(-0.200994813431936,0.00608513452974621,
-0.0100425115383475));
#38364=CARTESIAN_POINT('Ctrl Pts',(-0.200984632920064,0.00587674000196599,
-0.0100080544960793));
#38365=CARTESIAN_POINT('Ctrl Pts',(-0.200970747022194,0.00550448498314526,
-0.00993669158873135));
#38366=CARTESIAN_POINT('Ctrl Pts',(-0.20096438802479,0.00504326515784926,
-0.0098251294401078));
#38367=CARTESIAN_POINT('Ctrl Pts',(-0.200979186972993,0.00452135562915181,
-0.00966231257002147));
#38368=CARTESIAN_POINT('Ctrl Pts',(-0.201003103960677,0.00414328927105012,
-0.0095231669350311));
#38369=CARTESIAN_POINT('Ctrl Pts',(-0.20103144157648,0.00382962576004159,
-0.00939437461606553));
#38370=CARTESIAN_POINT('Ctrl Pts',(-0.201051630275061,0.00365329789975121,
-0.00931606955853783));
#38371=CARTESIAN_POINT('Ctrl Pts',(-0.201096047091507,0.00329650799822964,
-0.00914858984126155));
#38372=CARTESIAN_POINT('Ctrl Pts',(-0.20114124093058,0.00298143730432313,
-0.00898125778455622));
#38373=CARTESIAN_POINT('Ctrl Pts',(-0.201177675620458,0.00274510091024268,
-0.00884063751610791));
#38374=CARTESIAN_POINT('',(-0.202178390238509,0.00274518461141551,-0.00886238765667538));
#38375=CARTESIAN_POINT('Ctrl Pts',(-0.201177763351363,0.00274510393520155,
-0.00884064122847788));
#38376=CARTESIAN_POINT('Ctrl Pts',(-0.201513793943995,0.00274513082230744,
-0.00884794399274696));
#38377=CARTESIAN_POINT('Ctrl Pts',(-0.201847555253796,0.00274515324551409,
-0.00885519487746271));
#38378=CARTESIAN_POINT('Ctrl Pts',(-0.202178455596619,0.00274517135762337,
-0.0088623811438036));
#38379=CARTESIAN_POINT('',(-0.202099486167777,0.00750048618412189,-0.0101745790373482));
#38380=CARTESIAN_POINT('Ctrl Pts',(-0.202178390238509,0.00274518461141551,
-0.00886238765667538));
#38381=CARTESIAN_POINT('Ctrl Pts',(-0.202141642700174,0.00298280250174922,
-0.00900376430935615));
#38382=CARTESIAN_POINT('Ctrl Pts',(-0.202096073383157,0.00329970770692211,
-0.00917193867634351));
#38383=CARTESIAN_POINT('Ctrl Pts',(-0.202051385104703,0.00365806649196233,
-0.00933994400439029));
#38384=CARTESIAN_POINT('Ctrl Pts',(-0.202031013291299,0.00383620024345885,
-0.00941887465041026));
#38385=CARTESIAN_POINT('Ctrl Pts',(-0.202002918010045,0.00414758988742412,
-0.0095464889586151));
#38386=CARTESIAN_POINT('Ctrl Pts',(-0.201979077837791,0.00452405425854171,
-0.00968486858469979));
#38387=CARTESIAN_POINT('Ctrl Pts',(-0.201964259756075,0.00504260003922919,
-0.00984656774115697));
#38388=CARTESIAN_POINT('Ctrl Pts',(-0.201970466218556,0.00550352850911395,
-0.00995814839597316));
#38389=CARTESIAN_POINT('Ctrl Pts',(-0.20198425173622,0.0058749187926387,
-0.0100293983289797));
#38390=CARTESIAN_POINT('Ctrl Pts',(-0.201994368236462,0.0060828133308569,
-0.0100638226599408));
#38391=CARTESIAN_POINT('Ctrl Pts',(-0.20200497764798,0.00626846786176619,
-0.0100906480095422));
#38392=CARTESIAN_POINT('Ctrl Pts',(-0.202010677229979,0.00635725597980151,
-0.0101020286816427));
#38393=CARTESIAN_POINT('Ctrl Pts',(-0.20202228103975,0.00653043393283875,
-0.0101228400557603));
#38394=CARTESIAN_POINT('Ctrl Pts',(-0.202039641458584,0.00676707384825273,
-0.0101458231096576));
#38395=CARTESIAN_POINT('Ctrl Pts',(-0.202061412767996,0.00704417286928311,
-0.0101641363102107));
#38396=CARTESIAN_POINT('Ctrl Pts',(-0.202082889000625,0.00730462260352203,
-0.0101726906059738));
#38397=CARTESIAN_POINT('Ctrl Pts',(-0.202092355332572,0.00741701669310581,
-0.0101744288378058));
#38398=CARTESIAN_POINT('Ctrl Pts',(-0.20209948616598,0.00750048592111213,
-0.0101745790373231));
#38399=CARTESIAN_POINT('',(-0.202180670184565,0.0122592735600236,-0.00885976401094108));
#38400=CARTESIAN_POINT('Ctrl Pts',(-0.202099486167777,0.00750048618412189,
-0.0101745790373482));
#38401=CARTESIAN_POINT('Ctrl Pts',(-0.202076106016961,0.00777643690849919,
-0.0101740575426325));
#38402=CARTESIAN_POINT('Ctrl Pts',(-0.202046783464256,0.00814210139549289,
-0.0101549087136242));
#38403=CARTESIAN_POINT('Ctrl Pts',(-0.202022790521316,0.00847257147790718,
-0.0101225200596911));
#38404=CARTESIAN_POINT('Ctrl Pts',(-0.202011260789241,0.00864623057456113,
-0.0101016120625616));
#38405=CARTESIAN_POINT('Ctrl Pts',(-0.202005589674707,0.00873549249903804,
-0.0100901265418475));
#38406=CARTESIAN_POINT('Ctrl Pts',(-0.201995124325738,0.0089205474429524,
-0.0100633132683614));
#38407=CARTESIAN_POINT('Ctrl Pts',(-0.201985141205441,0.00912791605188965,
-0.0100289077382085));
#38408=CARTESIAN_POINT('Ctrl Pts',(-0.201971560044696,0.0094984739199577,
-0.00995769693082072));
#38409=CARTESIAN_POINT('Ctrl Pts',(-0.201965440095476,0.00995740917196224,
-0.00984660305171449));
#38410=CARTESIAN_POINT('Ctrl Pts',(-0.201980326512632,0.0104783224757965,
-0.00968411601573794));
#38411=CARTESIAN_POINT('Ctrl Pts',(-0.202004276740897,0.0108552791705883,
-0.009545404489792));
#38412=CARTESIAN_POINT('Ctrl Pts',(-0.202032481994145,0.0111669978914189,
-0.00941752983743049));
#38413=CARTESIAN_POINT('Ctrl Pts',(-0.202052945089522,0.0113452706979188,
-0.0093384552071316));
#38414=CARTESIAN_POINT('Ctrl Pts',(-0.202097867963932,0.0117040370740209,
-0.00917008223814911));
#38415=CARTESIAN_POINT('Ctrl Pts',(-0.202143701978128,0.0120213473325891,
-0.00900150217001001));
#38416=CARTESIAN_POINT('Ctrl Pts',(-0.202180670184565,0.0122592735600236,
-0.00885976401094108));
#38417=CARTESIAN_POINT('Ctrl Pts',(-0.202180736625232,0.012259282168623,
-0.00885976029392518));
#38418=CARTESIAN_POINT('Ctrl Pts',(-0.20184764381904,0.0122593589071325,
-0.00885249339404029));
#38419=CARTESIAN_POINT('Ctrl Pts',(-0.201514155362888,0.0122594397984704,
-0.008845215427718));
#38420=CARTESIAN_POINT('Ctrl Pts',(-0.201180522815623,0.0122595247994947,
-0.00883793187370074));
#38421=CARTESIAN_POINT('Origin',(-0.199568871480718,0.0075000007634268,
-0.000819355499014377));
#38422=CARTESIAN_POINT('',(-0.199179703927896,0.0122617568640769,-0.00879700974463651));
#38423=CARTESIAN_POINT('',(-0.199100855044633,0.00750164282994255,-0.0101077379410075));
#38424=CARTESIAN_POINT('Ctrl Pts',(-0.199179703927896,0.0122617568640769,
-0.00879700974463651));
#38425=CARTESIAN_POINT('Ctrl Pts',(-0.199143204201,0.0120247611072695,-0.00893759561857762));
#38426=CARTESIAN_POINT('Ctrl Pts',(-0.199097939428168,0.0117088168372167,
-0.00910488168002557));
#38427=CARTESIAN_POINT('Ctrl Pts',(-0.199053503138609,0.0113512026808426,
-0.0092722473869251));
#38428=CARTESIAN_POINT('Ctrl Pts',(-0.199033293522739,0.0111741545475986,
-0.00935061960017856));
#38429=CARTESIAN_POINT('Ctrl Pts',(-0.199005137616745,0.0108610682528071,
-0.00947879250595618));
#38430=CARTESIAN_POINT('Ctrl Pts',(-0.198981346397536,0.0104828930260802,
-0.00961764034004101));
#38431=CARTESIAN_POINT('Ctrl Pts',(-0.198966676100586,0.00995915763679357,
-0.00978057905748434));
#38432=CARTESIAN_POINT('Ctrl Pts',(-0.198973041715815,0.00949846961319302,
-0.00989171088830268));
#38433=CARTESIAN_POINT('Ctrl Pts',(-0.198986847549745,0.00912555823936307,
-0.00996303926878747));
#38434=CARTESIAN_POINT('Ctrl Pts',(-0.198996951253955,0.00891696971379377,
-0.0099974514904745));
#38435=CARTESIAN_POINT('Ctrl Pts',(-0.199007563060688,0.00873019692801794,
-0.0100243178043377));
#38436=CARTESIAN_POINT('Ctrl Pts',(-0.199013193043944,0.00864186587218177,
-0.0100355847905736));
#38437=CARTESIAN_POINT('Ctrl Pts',(-0.199024702404667,0.00846869292596894,
-0.0100562817337783));
#38438=CARTESIAN_POINT('Ctrl Pts',(-0.199048566807395,0.00813984594312779,
-0.0100882617902053));
#38439=CARTESIAN_POINT('Ctrl Pts',(-0.199077674466065,0.00777604990432176,
-0.0101071872672199));
#38440=CARTESIAN_POINT('Ctrl Pts',(-0.199100855518735,0.00750164301569709,
-0.0101077379539484));
#38441=CARTESIAN_POINT('',(-0.199174890168764,0.00274277102513258,-0.00879960252067264));
#38442=CARTESIAN_POINT('Ctrl Pts',(-0.199100855499581,0.00750164279111966,
-0.010107737953573));
#38443=CARTESIAN_POINT('Ctrl Pts',(-0.199096512842791,0.0074507254531517,
-0.0101076528529768));
#38444=CARTESIAN_POINT('Ctrl Pts',(-0.199083134658093,0.0072923247860624,
-0.0101058783397399));
#38445=CARTESIAN_POINT('Ctrl Pts',(-0.199063642168381,0.0070548680736872,
-0.010097459801595));
#38446=CARTESIAN_POINT('Ctrl Pts',(-0.199040944663942,0.00676685079174908,
-0.0100792908277045));
#38447=CARTESIAN_POINT('Ctrl Pts',(-0.199023857146907,0.00653361641306146,
-0.0100564833735876));
#38448=CARTESIAN_POINT('Ctrl Pts',(-0.199012188872024,0.00636007042461428,
-0.0100358089039185));
#38449=CARTESIAN_POINT('Ctrl Pts',(-0.199006474143519,0.0062713629778719,
-0.010024496770625));
#38450=CARTESIAN_POINT('Ctrl Pts',(-0.19899579505426,0.00608569538297935,
-0.00999783233827452));
#38451=CARTESIAN_POINT('Ctrl Pts',(-0.198985535474748,0.00587698222152784,
-0.00996346271303501));
#38452=CARTESIAN_POINT('Ctrl Pts',(-0.198971489215569,0.00550454656573253,
-0.00989233175470144));
#38453=CARTESIAN_POINT('Ctrl Pts',(-0.198964807417977,0.0050434817823875,
-0.0097812491317302));
#38454=CARTESIAN_POINT('Ctrl Pts',(-0.198979069999859,0.00452083414037976,
-0.00961883927653868));
#38455=CARTESIAN_POINT('Ctrl Pts',(-0.199002513849818,0.0041425196065762,
-0.00948013203005093));
#38456=CARTESIAN_POINT('Ctrl Pts',(-0.199030389517277,0.00382879040644363,
-0.0093518231363092));
#38457=CARTESIAN_POINT('Ctrl Pts',(-0.19905031989914,0.00365219450905632,
-0.00927371564898574));
#38458=CARTESIAN_POINT('Ctrl Pts',(-0.199094175364824,0.00329507035401741,
-0.00910675653462751));
#38459=CARTESIAN_POINT('Ctrl Pts',(-0.199138855829589,0.00297952240380151,
-0.00893987067691832));
#38460=CARTESIAN_POINT('Ctrl Pts',(-0.199174890168764,0.00274277102513258,
-0.00879960252067264));
#38461=CARTESIAN_POINT('',(-0.200176298967052,0.00274312284324985,-0.00882151165036355));
#38462=CARTESIAN_POINT('Ctrl Pts',(-0.199174978504506,0.0027427741926983,
-0.00879960632195548));
#38463=CARTESIAN_POINT('Ctrl Pts',(-0.199508744817405,0.00274289029024272,
-0.00880690787508466));
#38464=CARTESIAN_POINT('Ctrl Pts',(-0.199842609566303,0.00274300207072459,
-0.00881420898572931));
#38465=CARTESIAN_POINT('Ctrl Pts',(-0.200176363703368,0.00274310946256466,
-0.00882150508214149));
#38466=CARTESIAN_POINT('',(-0.200100346793384,0.007501072560866,-0.0101293929847466));
#38467=CARTESIAN_POINT('Ctrl Pts',(-0.200176298967052,0.00274312284324985,
-0.00882151165036355));
#38468=CARTESIAN_POINT('Ctrl Pts',(-0.200139901624223,0.00298111288128331,
-0.00896249548311666));
#38469=CARTESIAN_POINT('Ctrl Pts',(-0.200094776359582,0.0032984278604287,
-0.00913017620506027));
#38470=CARTESIAN_POINT('Ctrl Pts',(-0.200050546122483,0.00365715840436292,
-0.00929766342399987));
#38471=CARTESIAN_POINT('Ctrl Pts',(-0.20003039577123,0.0038354058170338,
-0.00937632392915631));
#38472=CARTESIAN_POINT('Ctrl Pts',(-0.200002621185558,0.00414711815629604,
-0.00950355721699447));
#38473=CARTESIAN_POINT('Ctrl Pts',(-0.199979106616714,0.00452386327719561,
-0.00964148519218933));
#38474=CARTESIAN_POINT('Ctrl Pts',(-0.199964614173862,0.00504258778238135,
-0.00980260694896718));
#38475=CARTESIAN_POINT('Ctrl Pts',(-0.199970998844043,0.00550380760441275,
-0.00991381891727839));
#38476=CARTESIAN_POINT('Ctrl Pts',(-0.199984884909593,0.0058751987753087,
-0.00998479074790535));
#38477=CARTESIAN_POINT('Ctrl Pts',(-0.199995051830887,0.00608317809692423,
-0.0100190916632865));
#38478=CARTESIAN_POINT('Ctrl Pts',(-0.200005680160915,0.00626858618305641,
-0.0100457782626161));
#38479=CARTESIAN_POINT('Ctrl Pts',(-0.200011403384908,0.00635753841527696,
-0.0100571356838335));
#38480=CARTESIAN_POINT('Ctrl Pts',(-0.200023028068371,0.00653068785947513,
-0.0100778720223878));
#38481=CARTESIAN_POINT('Ctrl Pts',(-0.200040486090422,0.00676818059405957,
-0.0101007806890797));
#38482=CARTESIAN_POINT('Ctrl Pts',(-0.200066404696961,0.00709789506032636,
-0.010122648472979));
#38483=CARTESIAN_POINT('Ctrl Pts',(-0.200089885580134,0.00737871281159999,
-0.0101291804881323));
#38484=CARTESIAN_POINT('Ctrl Pts',(-0.200100346789817,0.00750107229631922,
-0.0101293929847));
#38485=CARTESIAN_POINT('',(-0.200180012158742,0.0122615324625992,-0.00881881320672816));
#38486=CARTESIAN_POINT('Ctrl Pts',(-0.200100346793384,0.007501072560866,
-0.0101293929847466));
#38487=CARTESIAN_POINT('Ctrl Pts',(-0.200077032371193,0.00777702625121947,
-0.0101288559212946));
#38488=CARTESIAN_POINT('Ctrl Pts',(-0.200047785351717,0.00814269793645221,
-0.0101097531678741));
#38489=CARTESIAN_POINT('Ctrl Pts',(-0.200023842556866,0.00847317582369828,
-0.0100774615819148));
#38490=CARTESIAN_POINT('Ctrl Pts',(-0.20001233035194,0.00864685470632593,
-0.0100566165239891));
#38491=CARTESIAN_POINT('Ctrl Pts',(-0.200006668220042,0.00873609402904403,
-0.0100451709625597));
#38492=CARTESIAN_POINT('Ctrl Pts',(-0.199996202196605,0.00892127235517656,
-0.0100184260680742));
#38493=CARTESIAN_POINT('Ctrl Pts',(-0.199986209497443,0.00912871922182942,
-0.00998411851683095));
#38494=CARTESIAN_POINT('Ctrl Pts',(-0.199972585062777,0.00949940521822475,
-0.00991311283795994));
#38495=CARTESIAN_POINT('Ctrl Pts',(-0.199966337977404,0.00995807776149586,
-0.00980246973164739));
#38496=CARTESIAN_POINT('Ctrl Pts',(-0.199980974423784,0.0104794470890044,
-0.00964043514661892));
#38497=CARTESIAN_POINT('Ctrl Pts',(-0.200004693306816,0.01085647907637,
-0.00950220593946975));
#38498=CARTESIAN_POINT('Ctrl Pts',(-0.200032664319952,0.0111681667330681,
-0.0093748392791198));
#38499=CARTESIAN_POINT('Ctrl Pts',(-0.200052998452224,0.0113465907494263,
-0.00929601341129254));
#38500=CARTESIAN_POINT('Ctrl Pts',(-0.200097650391265,0.0117056249071542,
-0.00912819209771724));
#38501=CARTESIAN_POINT('Ctrl Pts',(-0.200143236687151,0.0120232851406314,
-0.00896013083810101));
#38502=CARTESIAN_POINT('Ctrl Pts',(-0.200180012158742,0.0122615324625992,
-0.00881881320672816));
#38503=CARTESIAN_POINT('Ctrl Pts',(-0.200180079025303,0.0122615411987862,
-0.00881880944411998));
#38504=CARTESIAN_POINT('Ctrl Pts',(-0.199847188917382,0.0122616093237988,
-0.0088115574338891));
#38505=CARTESIAN_POINT('Ctrl Pts',(-0.199513665157781,0.0122616817788384,
-0.0088042891129262));
#38506=CARTESIAN_POINT('Ctrl Pts',(-0.199179794132942,0.012261758536906,
-0.00879701070083819));
#38507=CARTESIAN_POINT('Origin',(-0.197568936813702,0.0075000008565567,
-0.000739278552754604));
#38508=CARTESIAN_POINT('',(-0.197178898213844,0.0122639308527257,-0.00875621776386257));
#38509=CARTESIAN_POINT('',(-0.197101863217746,0.00750262246797567,-0.0100625703404307));
#38510=CARTESIAN_POINT('Ctrl Pts',(-0.197178898213844,0.0122639308527257,
-0.00875621776386257));
#38511=CARTESIAN_POINT('Ctrl Pts',(-0.19714259372659,0.0120266476840343,
-0.00889635098469014));
#38512=CARTESIAN_POINT('Ctrl Pts',(-0.197097579703726,0.0117104025483866,
-0.00906308102871975));
#38513=CARTESIAN_POINT('Ctrl Pts',(-0.197053415857518,0.0113525637018549,
-0.00922986495999574));
#38514=CARTESIAN_POINT('Ctrl Pts',(-0.197033337579018,0.0111754135137217,
-0.00930796486082764));
#38515=CARTESIAN_POINT('Ctrl Pts',(-0.197005409642325,0.0108623084455755,
-0.00943564106288338));
#38516=CARTESIAN_POINT('Ctrl Pts',(-0.196981851559973,0.0104840536183527,
-0.00957399630291121));
#38517=CARTESIAN_POINT('Ctrl Pts',(-0.196967442586391,0.00995994453949125,
-0.00973644770686073));
#38518=CARTESIAN_POINT('Ctrl Pts',(-0.196973960238896,0.00949949430987693,
-0.00984713249190998));
#38519=CARTESIAN_POINT('Ctrl Pts',(-0.196987841285996,0.00912652089145974,
-0.00991824315734064));
#38520=CARTESIAN_POINT('Ctrl Pts',(-0.196997975177209,0.00891789605014179,
-0.00995255254822396));
#38521=CARTESIAN_POINT('Ctrl Pts',(-0.197008607375973,0.00873105355572069,
-0.00997934580045198));
#38522=CARTESIAN_POINT('Ctrl Pts',(-0.197014240119431,0.00864274709212368,
-0.0099905753992407));
#38523=CARTESIAN_POINT('Ctrl Pts',(-0.197025754698584,0.00846957756916279,
-0.0100112112482997));
#38524=CARTESIAN_POINT('Ctrl Pts',(-0.197049615978027,0.00814075996848684,
-0.0100431010647813));
#38525=CARTESIAN_POINT('Ctrl Pts',(-0.197078704301286,0.0077770004044274,
-0.0100619918809788));
#38526=CARTESIAN_POINT('Ctrl Pts',(-0.19710186371798,0.00750262251022666,
-0.0100625703535652));
#38527=CARTESIAN_POINT('',(-0.19717625942921,0.00274085336740581,-0.00875899754539223));
#38528=CARTESIAN_POINT('Ctrl Pts',(-0.197101863740693,0.0075026222411284,
-0.0100625703541326));
#38529=CARTESIAN_POINT('Ctrl Pts',(-0.19710000820331,0.00748080937071407,
-0.0100625363069147));
#38530=CARTESIAN_POINT('Ctrl Pts',(-0.197092850772113,0.00739629281398418,
-0.0100620378586211));
#38531=CARTESIAN_POINT('Ctrl Pts',(-0.197082572289835,0.0072731864579776,
-0.010059714804392));
#38532=CARTESIAN_POINT('Ctrl Pts',(-0.197064196962725,0.00704941232229019,
-0.0100523810870764));
#38533=CARTESIAN_POINT('Ctrl Pts',(-0.197042298317003,0.00677016330244297,
-0.0100343141173027));
#38534=CARTESIAN_POINT('Ctrl Pts',(-0.197025003299601,0.00653407818619356,
-0.0100115858250691));
#38535=CARTESIAN_POINT('Ctrl Pts',(-0.197013366326264,0.0063606929252265,
-0.00999098123439524));
#38536=CARTESIAN_POINT('Ctrl Pts',(-0.197007634588523,0.00627164901858326,
-0.00997967976748478));
#38537=CARTESIAN_POINT('Ctrl Pts',(-0.196996967220652,0.00608618549516388,
-0.00995315170376989));
#38538=CARTESIAN_POINT('Ctrl Pts',(-0.196986666483152,0.00587700992513145,
-0.00991884864512528));
#38539=CARTESIAN_POINT('Ctrl Pts',(-0.196972560336713,0.00550427978223037,
-0.0098479158597966));
#38540=CARTESIAN_POINT('Ctrl Pts',(-0.196965721899109,0.00504399465872652,
-0.00973747933000136));
#38541=CARTESIAN_POINT('Ctrl Pts',(-0.196979841087771,0.00452005502685437,
-0.00957533456267068));
#38542=CARTESIAN_POINT('Ctrl Pts',(-0.197003260603367,0.0041416367207074,
-0.0094371187180398));
#38543=CARTESIAN_POINT('Ctrl Pts',(-0.197031131766291,0.00382819529897539,
-0.00930946168380616));
#38544=CARTESIAN_POINT('Ctrl Pts',(-0.19705114822033,0.00365125562861138,
-0.00923153950398635));
#38545=CARTESIAN_POINT('Ctrl Pts',(-0.197095163150635,0.0032939066678421,
-0.00906518924055637));
#38546=CARTESIAN_POINT('Ctrl Pts',(-0.197140051657865,0.00297795351737253,
-0.00889883295406792));
#38547=CARTESIAN_POINT('Ctrl Pts',(-0.19717625942921,0.00274085336740581,
-0.00875899754539223));
#38548=CARTESIAN_POINT('',(-0.198174032768987,0.00274096783991525,-0.00878067084834629));
#38549=CARTESIAN_POINT('Ctrl Pts',(-0.1971763502326,0.00274085635926309,
-0.00875900128602603));
#38550=CARTESIAN_POINT('Ctrl Pts',(-0.197510802105109,0.00274089373748812,
-0.00876626555074249));
#38551=CARTESIAN_POINT('Ctrl Pts',(-0.197843551375065,0.00274092638819502,
-0.0087734901437584));
#38552=CARTESIAN_POINT('Ctrl Pts',(-0.198174097223676,0.00274095441811271,
-0.00878066428407293));
#38553=CARTESIAN_POINT('',(-0.198101361533896,0.00750214622993516,-0.0100842099593931));
#38554=CARTESIAN_POINT('Ctrl Pts',(-0.198174032768987,0.00274096783991525,
-0.00878067084834629));
#38555=CARTESIAN_POINT('Ctrl Pts',(-0.198138061322491,0.00297936807682186,
-0.0089212776129119));
#38556=CARTESIAN_POINT('Ctrl Pts',(-0.198093477108618,0.00329714613090043,
-0.00908848214951006));
#38557=CARTESIAN_POINT('Ctrl Pts',(-0.198049811215033,0.0036562864094438,
-0.00925545767808787));
#38558=CARTESIAN_POINT('Ctrl Pts',(-0.198029930114142,0.00383470369580787,
-0.00933386550169443));
#38559=CARTESIAN_POINT('Ctrl Pts',(-0.198002573654122,0.00414664354364956,
-0.00946066872251577));
#38560=CARTESIAN_POINT('Ctrl Pts',(-0.197979478111198,0.00452366787372502,
-0.00959814161153211));
#38561=CARTESIAN_POINT('Ctrl Pts',(-0.19796541505455,0.0050428957774833,
-0.00975876511200693));
#38562=CARTESIAN_POINT('Ctrl Pts',(-0.197972019492495,0.0055041999955818,
-0.00986953619272144));
#38563=CARTESIAN_POINT('Ctrl Pts',(-0.197985992896418,0.00587566481187643,
-0.00994023559640718));
#38564=CARTESIAN_POINT('Ctrl Pts',(-0.197996197119194,0.00608385240141643,
-0.00997442519451085));
#38565=CARTESIAN_POINT('Ctrl Pts',(-0.198006815342193,0.00626894970105581,
-0.0100009515703469));
#38566=CARTESIAN_POINT('Ctrl Pts',(-0.198012537979335,0.00635797677696961,
-0.0100122864200635));
#38567=CARTESIAN_POINT('Ctrl Pts',(-0.198024203479145,0.00653171972941347,
-0.0100329456666756));
#38568=CARTESIAN_POINT('Ctrl Pts',(-0.198041324115801,0.00676561835599725,
-0.010055764848873));
#38569=CARTESIAN_POINT('Ctrl Pts',(-0.198064034153434,0.00705384034717996,
-0.0100739406522062));
#38570=CARTESIAN_POINT('Ctrl Pts',(-0.198083644772806,0.00729297247666229,
-0.010082361311082));
#38571=CARTESIAN_POINT('Ctrl Pts',(-0.198096918465339,0.00744974375587924,
-0.0100841258368541));
#38572=CARTESIAN_POINT('Ctrl Pts',(-0.198101361530205,0.00750214596208306,
-0.0100842099593748));
#38573=CARTESIAN_POINT('',(-0.198179287823527,0.0122637027296793,-0.00877800875605197));
#38574=CARTESIAN_POINT('Ctrl Pts',(-0.198101361533896,0.00750214622993515,
-0.0100842099593931));
#38575=CARTESIAN_POINT('Ctrl Pts',(-0.198078064760131,0.00777806953424965,
-0.0100836420027939));
#38576=CARTESIAN_POINT('Ctrl Pts',(-0.198048832502402,0.00814370089079693,
-0.0100645708158547));
#38577=CARTESIAN_POINT('Ctrl Pts',(-0.198024889911693,0.00847414328964963,
-0.010032367938066));
#38578=CARTESIAN_POINT('Ctrl Pts',(-0.198013371582161,0.00864781364955267,
-0.0100115835738566));
#38579=CARTESIAN_POINT('Ctrl Pts',(-0.19800770620434,0.00873702690890067,
-0.0100001753830021));
#38580=CARTESIAN_POINT('Ctrl Pts',(-0.197997220260069,0.00892226298464491,
-0.00997350350283401));
#38581=CARTESIAN_POINT('Ctrl Pts',(-0.197987198570751,0.0091297389651211,
-0.00993929825390304));
#38582=CARTESIAN_POINT('Ctrl Pts',(-0.197973502881743,0.009500474943299,
-0.00986851018274228));
#38583=CARTESIAN_POINT('Ctrl Pts',(-0.197967115435973,0.00995897304118631,
-0.00975829178770248));
#38584=CARTESIAN_POINT('Ctrl Pts',(-0.197981507135243,0.0104806097246969,
-0.00959676986039016));
#38585=CARTESIAN_POINT('Ctrl Pts',(-0.198005003872498,0.0108576989128222,
-0.00945904051216777));
#38586=CARTESIAN_POINT('Ctrl Pts',(-0.198032755894909,0.0111693872661804,
-0.00933217581919596));
#38587=CARTESIAN_POINT('Ctrl Pts',(-0.19805296392532,0.011347923686061,
-0.00925362054200033));
#38588=CARTESIAN_POINT('Ctrl Pts',(-0.198097354270813,0.0117071893600477,
-0.0090863808984517));
#38589=CARTESIAN_POINT('Ctrl Pts',(-0.198142699816937,0.0120251604527111,
-0.00891887465281153));
#38590=CARTESIAN_POINT('Ctrl Pts',(-0.198179287823527,0.0122637027296793,
-0.00877800875605197));
#38591=CARTESIAN_POINT('Ctrl Pts',(-0.198179354943918,0.0122637115781413,
-0.00877800495436216));
#38592=CARTESIAN_POINT('Ctrl Pts',(-0.197846468878006,0.0122637807574249,
-0.00877075785975849));
#38593=CARTESIAN_POINT('Ctrl Pts',(-0.197512916440007,0.0122638544198246,
-0.00876349367670277));
#38594=CARTESIAN_POINT('Ctrl Pts',(-0.197178988840092,0.0122639325398186,
-0.00875621872371576));
#38595=CARTESIAN_POINT('Origin',(-0.195568817432697,0.00750000072543657,
-0.000658346566684942));
#38596=CARTESIAN_POINT('',(-0.195178104730999,0.0122657318419193,-0.00871574250981778));
#38597=CARTESIAN_POINT('',(-0.195102858686147,0.00750349572610613,-0.0100174023059187));
#38598=CARTESIAN_POINT('Ctrl Pts',(-0.195178104730999,0.0122657318419193,
-0.00871574250981778));
#38599=CARTESIAN_POINT('Ctrl Pts',(-0.195141971850056,0.0120281695201214,
-0.00885539096701177));
#38600=CARTESIAN_POINT('Ctrl Pts',(-0.195097177150193,0.0117116408727372,
-0.00902152489589311));
#38601=CARTESIAN_POINT('Ctrl Pts',(-0.195053245825187,0.011353580518071,
-0.00918769379669155));
#38602=CARTESIAN_POINT('Ctrl Pts',(-0.195033282223062,0.0111763704209235,
-0.00926548967369924));
#38603=CARTESIAN_POINT('Ctrl Pts',(-0.195005529791546,0.0108631259821725,
-0.00939269413058469));
#38604=CARTESIAN_POINT('Ctrl Pts',(-0.194982154210136,0.0104847570855313,
-0.00953053190643839));
#38605=CARTESIAN_POINT('Ctrl Pts',(-0.194967940414644,0.00996059210314794,
-0.00969237054229474));
#38606=CARTESIAN_POINT('Ctrl Pts',(-0.194974581042148,0.00950004130325584,
-0.00980266786669539));
#38607=CARTESIAN_POINT('Ctrl Pts',(-0.194988548178529,0.00912711026305177,
-0.0098735158134373));
#38608=CARTESIAN_POINT('Ctrl Pts',(-0.194998725529187,0.00891852251849867,
-0.00990770057596708));
#38609=CARTESIAN_POINT('Ctrl Pts',(-0.195009393305373,0.00873173227665468,
-0.00993439713830365));
#38610=CARTESIAN_POINT('Ctrl Pts',(-0.195015042871648,0.00864343621680832,
-0.00994558943115054));
#38611=CARTESIAN_POINT('Ctrl Pts',(-0.195026589264483,0.00847029750149345,
-0.00996615649178523));
#38612=CARTESIAN_POINT('Ctrl Pts',(-0.19505050856113,0.00814153252125014,
-0.00999794766159865));
#38613=CARTESIAN_POINT('Ctrl Pts',(-0.195079656832268,0.00777783275067516,
-0.010016797998545));
#38614=CARTESIAN_POINT('Ctrl Pts',(-0.195102859197629,0.00750349576939646,
-0.0100174023200885));
#38615=CARTESIAN_POINT('',(-0.19517797993867,0.00273809386567736,-0.00871799806561756));
#38616=CARTESIAN_POINT('Ctrl Pts',(-0.195102859215766,0.00750349555493702,
-0.0100174023205609));
#38617=CARTESIAN_POINT('Ctrl Pts',(-0.195100949641578,0.00748091060552787,
-0.0100173694335902));
#38618=CARTESIAN_POINT('Ctrl Pts',(-0.195093941673867,0.00739765059757744,
-0.0100168843546768));
#38619=CARTESIAN_POINT('Ctrl Pts',(-0.195083666814497,0.00727384426413517,
-0.0100145806517102));
#38620=CARTESIAN_POINT('Ctrl Pts',(-0.195065427890217,0.00705034028650716,
-0.0100072931400613));
#38621=CARTESIAN_POINT('Ctrl Pts',(-0.195043635768285,0.00677069706287903,
-0.00998930677462411));
#38622=CARTESIAN_POINT('Ctrl Pts',(-0.195026446133143,0.00653446921995725,
-0.00996665842637773));
#38623=CARTESIAN_POINT('Ctrl Pts',(-0.195014882614189,0.00636097407782196,
-0.00994612972574996));
#38624=CARTESIAN_POINT('Ctrl Pts',(-0.19500917675081,0.00627167458992341,
-0.00993483859680917));
#38625=CARTESIAN_POINT('Ctrl Pts',(-0.194998616244289,0.00608664200750535,
-0.00990848143429438));
#38626=CARTESIAN_POINT('Ctrl Pts',(-0.194988392779268,0.00587728921639411,
-0.00987429706439239));
#38627=CARTESIAN_POINT('Ctrl Pts',(-0.194974428076451,0.00550449240298873,
-0.00980364228685664));
#38628=CARTESIAN_POINT('Ctrl Pts',(-0.194967724982329,0.00504366300959344,
-0.00969353647290735));
#38629=CARTESIAN_POINT('Ctrl Pts',(-0.194981896216006,0.00451896128129825,
-0.00953177976677903));
#38630=CARTESIAN_POINT('Ctrl Pts',(-0.195005276822889,0.00414029348230681,
-0.00939400313637884));
#38631=CARTESIAN_POINT('Ctrl Pts',(-0.195033051886066,0.00382690893110969,
-0.00926688245348259));
#38632=CARTESIAN_POINT('Ctrl Pts',(-0.195053038245836,0.00364968132354558,
-0.00918915665886015));
#38633=CARTESIAN_POINT('Ctrl Pts',(-0.19509697568046,0.00329201079149359,
-0.00902334424493648));
#38634=CARTESIAN_POINT('Ctrl Pts',(-0.195141810958693,0.00297559470165675,
-0.00885745735339972));
#38635=CARTESIAN_POINT('Ctrl Pts',(-0.19517797993867,0.00273809386567736,
-0.00871799806561756));
#38636=CARTESIAN_POINT('',(-0.196177537013878,0.00273881078232022,-0.00874004887933647));
#38637=CARTESIAN_POINT('Ctrl Pts',(-0.195178071596977,0.00273809719998608,
-0.00871800201771347));
#38638=CARTESIAN_POINT('Ctrl Pts',(-0.195511220445504,0.00273833506685321,
-0.00872535085344679));
#38639=CARTESIAN_POINT('Ctrl Pts',(-0.195844467515233,0.00273856839192212,
-0.00873269911814646));
#38640=CARTESIAN_POINT('Ctrl Pts',(-0.196177604968697,0.00273879702797085,
-0.00874004222951915));
#38641=CARTESIAN_POINT('',(-0.196102482808628,0.0075031283040999,-0.0100390287523791));
#38642=CARTESIAN_POINT('Ctrl Pts',(-0.196177537013878,0.00273881078232022,
-0.00874004887933647));
#38643=CARTESIAN_POINT('Ctrl Pts',(-0.196141077813662,0.002977546954655,
-0.00888020254352069));
#38644=CARTESIAN_POINT('Ctrl Pts',(-0.1960958943586,0.003295720706571,-0.00904686057463413));
#38645=CARTESIAN_POINT('Ctrl Pts',(-0.196051682528282,0.00365512641323152,
-0.00921323603776369));
#38646=CARTESIAN_POINT('Ctrl Pts',(-0.196031544479116,0.00383389049984808,
-0.00929145057678427));
#38647=CARTESIAN_POINT('Ctrl Pts',(-0.196003981018244,0.0041452785571844,
-0.00941749978987608));
#38648=CARTESIAN_POINT('Ctrl Pts',(-0.195980695863156,0.00452230528419756,
-0.0095544680877062));
#38649=CARTESIAN_POINT('Ctrl Pts',(-0.195966579506683,0.00504344712837199,
-0.00971501996119166));
#38650=CARTESIAN_POINT('Ctrl Pts',(-0.19597325975956,0.00550360409286807,
-0.0098250504480127));
#38651=CARTESIAN_POINT('Ctrl Pts',(-0.195987256853935,0.00587551587646132,
-0.00989558612950375));
#38652=CARTESIAN_POINT('Ctrl Pts',(-0.195997482940324,0.00608413149667644,
-0.00992970850098842));
#38653=CARTESIAN_POINT('Ctrl Pts',(-0.196008100881894,0.0062693916013721,
-0.00995614659231545));
#38654=CARTESIAN_POINT('Ctrl Pts',(-0.196013821361637,0.00635852739556059,
-0.00996744984550979));
#38655=CARTESIAN_POINT('Ctrl Pts',(-0.196025488473502,0.00653255950142857,
-0.00998803747009445));
#38656=CARTESIAN_POINT('Ctrl Pts',(-0.19604251164246,0.00676571709900968,
-0.0100107659233449));
#38657=CARTESIAN_POINT('Ctrl Pts',(-0.196070031707032,0.00711557397662451,
-0.0100324670854736));
#38658=CARTESIAN_POINT('Ctrl Pts',(-0.196089303496893,0.00734820057878708,
-0.0100387954224435));
#38659=CARTESIAN_POINT('Ctrl Pts',(-0.196102482808628,0.0075031283040999,
-0.0100390287523791));
#38660=CARTESIAN_POINT('',(-0.196178484195762,0.0122657643255281,-0.00873736329835759));
#38661=CARTESIAN_POINT('Ctrl Pts',(-0.196102482807571,0.00750312859925915,
-0.0100390287522575));
#38662=CARTESIAN_POINT('Ctrl Pts',(-0.196079156242257,0.00777902017568519,
-0.0100384318480314));
#38663=CARTESIAN_POINT('Ctrl Pts',(-0.196049879511574,0.00814460596841201,
-0.0100193964106389));
#38664=CARTESIAN_POINT('Ctrl Pts',(-0.196025889608579,0.00847500825680877,
-0.00998728738456208));
#38665=CARTESIAN_POINT('Ctrl Pts',(-0.196014343371659,0.00864865962912956,
-0.00996656810576789));
#38666=CARTESIAN_POINT('Ctrl Pts',(-0.196008663300801,0.00873785767352454,
-0.00995519720228832));
#38667=CARTESIAN_POINT('Ctrl Pts',(-0.195998141861114,0.00892308850487265,
-0.00992861152525066));
#38668=CARTESIAN_POINT('Ctrl Pts',(-0.195988075859801,0.00913055848064588,
-0.00989452055980878));
#38669=CARTESIAN_POINT('Ctrl Pts',(-0.195974288909848,0.00950129545777585,
-0.00982397494050396));
#38670=CARTESIAN_POINT('Ctrl Pts',(-0.195967760794256,0.00995982623587528,
-0.00971414472348679));
#38671=CARTESIAN_POINT('Ctrl Pts',(-0.195981926030902,0.0104815441926318,
-0.00955321072493732));
#38672=CARTESIAN_POINT('Ctrl Pts',(-0.196005215231541,0.0108587298290495,
-0.00941599040482433));
#38673=CARTESIAN_POINT('Ctrl Pts',(-0.196032767263529,0.0111705199455354,
-0.00928960083841346));
#38674=CARTESIAN_POINT('Ctrl Pts',(-0.196052849549526,0.0113491432795003,
-0.00921133497787415));
#38675=CARTESIAN_POINT('Ctrl Pts',(-0.196096982103339,0.0117086492359856,
-0.00904469186630159));
#38676=CARTESIAN_POINT('Ctrl Pts',(-0.196142085551053,0.0120269270976718,
-0.00887776111976833));
#38677=CARTESIAN_POINT('Ctrl Pts',(-0.196178484195762,0.0122657643255281,
-0.00873736329835759));
#38678=CARTESIAN_POINT('Ctrl Pts',(-0.196178551300409,0.012265773450217,
-0.00873735935601521));
#38679=CARTESIAN_POINT('Ctrl Pts',(-0.195841577142587,0.0122657554214599,
-0.00873008066191514));
#38680=CARTESIAN_POINT('Ctrl Pts',(-0.195507874037976,0.0122657421970718,
-0.00872286988639498));
#38681=CARTESIAN_POINT('Ctrl Pts',(-0.195178195187604,0.0122657335081665,
-0.00871574348158736));
#38682=CARTESIAN_POINT('Origin',(-0.221676249214976,0.00750000345182045,
-0.0016541350256873));
#38683=CARTESIAN_POINT('',(-0.221393352906395,0.0131398835301861,-0.00861356300121323));
#38684=CARTESIAN_POINT('',(-0.22109337191764,0.00750288941767847,-0.0106049432732665));
#38685=CARTESIAN_POINT('Ctrl Pts',(-0.221393352906395,0.0131398835301861,
-0.00861356300121323));
#38686=CARTESIAN_POINT('Ctrl Pts',(-0.221320888392813,0.0128815572458935,
-0.00882126869267544));
#38687=CARTESIAN_POINT('Ctrl Pts',(-0.221231380503492,0.01252852322136,
-0.00907134596473989));
#38688=CARTESIAN_POINT('Ctrl Pts',(-0.221145875567908,0.012125092174896,
-0.00932172732914744));
#38689=CARTESIAN_POINT('Ctrl Pts',(-0.221106505058042,0.0119112831655975,
-0.00944594135167501));
#38690=CARTESIAN_POINT('Ctrl Pts',(-0.221059952440027,0.0115846277870923,
-0.00962205237725879));
#38691=CARTESIAN_POINT('Ctrl Pts',(-0.221025069259206,0.0112550786873381,
-0.00978133219115847));
#38692=CARTESIAN_POINT('Ctrl Pts',(-0.220997005450521,0.0108970649444057,
-0.00993743190236953));
#38693=CARTESIAN_POINT('Ctrl Pts',(-0.220969865667947,0.0103669261135731,
-0.0101389726762554));
#38694=CARTESIAN_POINT('Ctrl Pts',(-0.220961462009027,0.00989275498375296,
-0.0102831873771524));
#38695=CARTESIAN_POINT('Ctrl Pts',(-0.22096744629676,0.00945353568132999,
-0.0103881570799034));
#38696=CARTESIAN_POINT('Ctrl Pts',(-0.220974504485159,0.00921313446131081,
-0.0104378830236523));
#38697=CARTESIAN_POINT('Ctrl Pts',(-0.220982990015517,0.00900856730165844,
-0.0104751602785334));
#38698=CARTESIAN_POINT('Ctrl Pts',(-0.220988827061368,0.00889688919602636,
-0.0104934052387218));
#38699=CARTESIAN_POINT('Ctrl Pts',(-0.221000849071749,0.00868900886590427,
-0.0105249286429414));
#38700=CARTESIAN_POINT('Ctrl Pts',(-0.221028102523713,0.00828742369692355,
-0.0105746853659743));
#38701=CARTESIAN_POINT('Ctrl Pts',(-0.221063893512024,0.00784105280531206,
-0.0106042019791774));
#38702=CARTESIAN_POINT('Ctrl Pts',(-0.22109337191764,0.00750288941767847,
-0.0106049432732665));
#38703=CARTESIAN_POINT('',(-0.22139902998639,0.00187359712117749,-0.00862457485406049));
#38704=CARTESIAN_POINT('Ctrl Pts',(-0.221093371849766,0.00750288863438198,
-0.0106049432720617));
#38705=CARTESIAN_POINT('Ctrl Pts',(-0.221091363881298,0.0074797159479151,
-0.0106049076271627));
#38706=CARTESIAN_POINT('Ctrl Pts',(-0.22108194961028,0.0073703646997039,
-0.0106041605834244));
#38707=CARTESIAN_POINT('Ctrl Pts',(-0.221069464690532,0.0072219193189083,
-0.0106005848012409));
#38708=CARTESIAN_POINT('Ctrl Pts',(-0.221046833823411,0.00694579229382263,
-0.0105891976872885));
#38709=CARTESIAN_POINT('Ctrl Pts',(-0.221021019951164,0.00660573000945973,
-0.0105611718773493));
#38710=CARTESIAN_POINT('Ctrl Pts',(-0.221001657246536,0.00631766602399646,
-0.010525847242072));
#38711=CARTESIAN_POINT('Ctrl Pts',(-0.220989834644077,0.00611007473471422,
-0.0104945212917132));
#38712=CARTESIAN_POINT('Ctrl Pts',(-0.220984064213525,0.00599749977732925,
-0.0104762053650152));
#38713=CARTESIAN_POINT('Ctrl Pts',(-0.220975914169275,0.00579574674814498,
-0.0104396178511159));
#38714=CARTESIAN_POINT('Ctrl Pts',(-0.22096913371177,0.0055560142321091,
-0.0103903121251423));
#38715=CARTESIAN_POINT('Ctrl Pts',(-0.220963685764794,0.00511849775881586,
-0.0102862894875993));
#38716=CARTESIAN_POINT('Ctrl Pts',(-0.220972608026894,0.00464366850233373,
-0.0101426368830028));
#38717=CARTESIAN_POINT('Ctrl Pts',(-0.221000259014373,0.00411210701081089,
-0.00994124950673877));
#38718=CARTESIAN_POINT('Ctrl Pts',(-0.221028553541809,0.00375413270785835,
-0.00978563731322991));
#38719=CARTESIAN_POINT('Ctrl Pts',(-0.221063591079418,0.00342517423379665,
-0.0096270942958683));
#38720=CARTESIAN_POINT('Ctrl Pts',(-0.221110019595894,0.00310085946309852,
-0.00945283986597018));
#38721=CARTESIAN_POINT('Ctrl Pts',(-0.22114970684413,0.00288660051048064,
-0.00932883343947502));
#38722=CARTESIAN_POINT('Ctrl Pts',(-0.221235749347005,0.00248406090325365,
-0.00907988578428976));
#38723=CARTESIAN_POINT('Ctrl Pts',(-0.221325971848273,0.0021315329244801,
-0.00883112553951364));
#38724=CARTESIAN_POINT('Ctrl Pts',(-0.22139902998639,0.00187359712117749,
-0.00862457485406049));
#38725=CARTESIAN_POINT('',(-0.222398601135893,0.00187304432676294,-0.00864558975234265));
#38726=CARTESIAN_POINT('Ctrl Pts',(-0.221399020810814,0.00187359579475767,
-0.00862457358681791));
#38727=CARTESIAN_POINT('Ctrl Pts',(-0.22173220220163,0.00187341250573888,
-0.00863157915856683));
#38728=CARTESIAN_POINT('Ctrl Pts',(-0.222065458410509,0.00187322296472307,
-0.00863858128083836));
#38729=CARTESIAN_POINT('Ctrl Pts',(-0.222398585769511,0.00187302728847401,
-0.00864557567262578));
#38730=CARTESIAN_POINT('',(-0.222093147561648,0.00750348224479951,-0.010626397051749));
#38731=CARTESIAN_POINT('Ctrl Pts',(-0.222398601135893,0.00187304432676294,
-0.00864558975234265));
#38732=CARTESIAN_POINT('Ctrl Pts',(-0.222325187289336,0.00213211751554539,
-0.00885308354687082));
#38733=CARTESIAN_POINT('Ctrl Pts',(-0.222234524925318,0.00248667979231716,
-0.00910316494991973));
#38734=CARTESIAN_POINT('Ctrl Pts',(-0.222148227978173,0.00289157024373901,
-0.00935329853342097));
#38735=CARTESIAN_POINT('Ctrl Pts',(-0.222108220765584,0.00310913850090322,
-0.00947892012615623));
#38736=CARTESIAN_POINT('Ctrl Pts',(-0.222062653109278,0.00343043737402986,
-0.00965117347710931));
#38737=CARTESIAN_POINT('Ctrl Pts',(-0.222027988046481,0.00375836192166522,
-0.00980902455604343));
#38738=CARTESIAN_POINT('Ctrl Pts',(-0.222000028444215,0.00411514200078309,
-0.00996391832910129));
#38739=CARTESIAN_POINT('Ctrl Pts',(-0.221972599258432,0.00464539931558352,
-0.0101646755818894));
#38740=CARTESIAN_POINT('Ctrl Pts',(-0.221963654068083,0.00512236114675374,
-0.0103088523151418));
#38741=CARTESIAN_POINT('Ctrl Pts',(-0.221969164074096,0.00556028642479754,
-0.0104127201061691));
#38742=CARTESIAN_POINT('Ctrl Pts',(-0.221975961917538,0.00580006583214543,
-0.0104619198396024));
#38743=CARTESIAN_POINT('Ctrl Pts',(-0.221984154308948,0.00600232160969846,
-0.0104984854563983));
#38744=CARTESIAN_POINT('Ctrl Pts',(-0.221989901165274,0.00611425910628736,
-0.0105166446946959));
#38745=CARTESIAN_POINT('Ctrl Pts',(-0.222001733104974,0.00632170003362734,
-0.0105478047522586));
#38746=CARTESIAN_POINT('Ctrl Pts',(-0.222020833446452,0.00660650372540828,
-0.0105829082019461));
#38747=CARTESIAN_POINT('Ctrl Pts',(-0.222047295132714,0.00695403250001243,
-0.0106107762904338));
#38748=CARTESIAN_POINT('Ctrl Pts',(-0.222068563458765,0.00721452309948346,
-0.0106220642645268));
#38749=CARTESIAN_POINT('Ctrl Pts',(-0.222083067589409,0.00738637227386414,
-0.0106256474234903));
#38750=CARTESIAN_POINT('Ctrl Pts',(-0.222088227461813,0.0074466538080066,
-0.0106263135983161));
#38751=CARTESIAN_POINT('Ctrl Pts',(-0.222093147561648,0.00750348224479952,
-0.010626397051749));
#38752=CARTESIAN_POINT('',(-0.222392883415946,0.013140228421378,-0.00863472093570934));
#38753=CARTESIAN_POINT('Ctrl Pts',(-0.222093147723645,0.00750348411589117,
-0.0106263970544966));
#38754=CARTESIAN_POINT('Ctrl Pts',(-0.222063525278338,0.00784362482559292,
-0.0106256289212465));
#38755=CARTESIAN_POINT('Ctrl Pts',(-0.222027600061407,0.00829239003459411,
-0.0105957558053965));
#38756=CARTESIAN_POINT('Ctrl Pts',(-0.222000309884482,0.00869597776263445,
-0.0105454451755359));
#38757=CARTESIAN_POINT('Ctrl Pts',(-0.221988315815748,0.00890451403744728,
-0.010513649509377));
#38758=CARTESIAN_POINT('Ctrl Pts',(-0.221982480934348,0.00901718087153725,
-0.0104951271796541));
#38759=CARTESIAN_POINT('Ctrl Pts',(-0.221974154674737,0.00922020971833267,
-0.0104579384685322));
#38760=CARTESIAN_POINT('Ctrl Pts',(-0.221967213526053,0.00945940727173018,
-0.0104082849356463));
#38761=CARTESIAN_POINT('Ctrl Pts',(-0.221961400036284,0.00989642795779487,
-0.0103035206111078));
#38762=CARTESIAN_POINT('Ctrl Pts',(-0.2219696861429,0.010366178439211,-0.0101606719072326));
#38763=CARTESIAN_POINT('Ctrl Pts',(-0.221996852716048,0.0108978547518354,
-0.0099585837497828));
#38764=CARTESIAN_POINT('Ctrl Pts',(-0.222024978452534,0.0112563342759193,
-0.00980220541016363));
#38765=CARTESIAN_POINT('Ctrl Pts',(-0.222059941847575,0.0115864713196668,
-0.0096425809766981));
#38766=CARTESIAN_POINT('Ctrl Pts',(-0.222106718095268,0.0119142299650681,
-0.00946573442095913));
#38767=CARTESIAN_POINT('Ctrl Pts',(-0.222145979109298,0.0121272431546103,
-0.00934187162863571));
#38768=CARTESIAN_POINT('Ctrl Pts',(-0.222231340004308,0.0125300857742674,
-0.00909171780656154));
#38769=CARTESIAN_POINT('Ctrl Pts',(-0.222320615693346,0.0128823903637851,
-0.00884205736930132));
#38770=CARTESIAN_POINT('Ctrl Pts',(-0.222392883415946,0.013140228421378,
-0.00863472093570934));
#38771=CARTESIAN_POINT('Ctrl Pts',(-0.222392866266696,0.0131402404723726,
-0.00863471080482401));
#38772=CARTESIAN_POINT('Ctrl Pts',(-0.22205953122811,0.0131401160464593,
-0.00862766243819364));
#38773=CARTESIAN_POINT('Ctrl Pts',(-0.221726275997956,0.0131399976615517,
-0.00862061088319733));
#38774=CARTESIAN_POINT('Ctrl Pts',(-0.221393342167719,0.0131398853792589,
-0.00861356127303571));
#38775=CARTESIAN_POINT('Origin',(-0.219678482255905,0.00750000881799777,
-0.00158211078495795));
#38776=CARTESIAN_POINT('',(-0.219329719998599,0.0129300414290672,-0.00873877355437297));
#38777=CARTESIAN_POINT('',(-0.219093932882599,0.00750191497004506,-0.0105597757686429));
#38778=CARTESIAN_POINT('Ctrl Pts',(-0.219329719998599,0.0129300414290672,
-0.00873877355437297));
#38779=CARTESIAN_POINT('Ctrl Pts',(-0.219266758960484,0.0126760187611208,
-0.00893004940303019));
#38780=CARTESIAN_POINT('Ctrl Pts',(-0.219189106959152,0.0123307812499729,
-0.00915981955588401));
#38781=CARTESIAN_POINT('Ctrl Pts',(-0.219115186308461,0.011938067343623,
-0.00938941159033229));
#38782=CARTESIAN_POINT('Ctrl Pts',(-0.21908130994182,0.0117311055603115,
-0.00950289623249571));
#38783=CARTESIAN_POINT('Ctrl Pts',(-0.219041424917209,0.011413227212336,
-0.00966452028186231));
#38784=CARTESIAN_POINT('Ctrl Pts',(-0.219002241537353,0.0109931559754825,
-0.00985732695261662));
#38785=CARTESIAN_POINT('Ctrl Pts',(-0.218968699515465,0.0103634071969913,
-0.0101006309736288));
#38786=CARTESIAN_POINT('Ctrl Pts',(-0.218962334120046,0.00978510275003089,
-0.0102674656157249));
#38787=CARTESIAN_POINT('Ctrl Pts',(-0.218970038446411,0.00936589217437247,
-0.0103626156626804));
#38788=CARTESIAN_POINT('Ctrl Pts',(-0.218977648081212,0.00913598387302089,
-0.0104078383387266));
#38789=CARTESIAN_POINT('Ctrl Pts',(-0.218986343736269,0.0089407838193126,
-0.0104416741937123));
#38790=CARTESIAN_POINT('Ctrl Pts',(-0.218992197178124,0.00883386602501995,
-0.0104582986982075));
#38791=CARTESIAN_POINT('Ctrl Pts',(-0.219004132386565,0.00863515157903343,
-0.010486974430302));
#38792=CARTESIAN_POINT('Ctrl Pts',(-0.219030846027741,0.00825129593526508,
-0.010532248951195));
#38793=CARTESIAN_POINT('Ctrl Pts',(-0.219065518877002,0.00782491766491167,
-0.0105590987246595));
#38794=CARTESIAN_POINT('Ctrl Pts',(-0.219093932882599,0.00750191497004506,
-0.0105597757686429));
#38795=CARTESIAN_POINT('',(-0.21933444621923,0.00208165094137429,-0.00874770213447828));
#38796=CARTESIAN_POINT('Ctrl Pts',(-0.219093932790715,0.00750191392014267,
-0.0105597757668944));
#38797=CARTESIAN_POINT('Ctrl Pts',(-0.219091363943786,0.00747256155481735,
-0.0105597268780573));
#38798=CARTESIAN_POINT('Ctrl Pts',(-0.219083158892815,0.00737816662329933,
-0.0105590385569155));
#38799=CARTESIAN_POINT('Ctrl Pts',(-0.219070669665003,0.00723153191317315,
-0.0105557469627765));
#38800=CARTESIAN_POINT('Ctrl Pts',(-0.219049040320226,0.00697092841451702,
-0.0105453386377339));
#38801=CARTESIAN_POINT('Ctrl Pts',(-0.219023788904892,0.00664446839385532,
-0.0105197865549645));
#38802=CARTESIAN_POINT('Ctrl Pts',(-0.219004840951088,0.00636982416329366,
-0.0104876187300696));
#38803=CARTESIAN_POINT('Ctrl Pts',(-0.218993082147653,0.00617145191753081,
-0.0104591077909951));
#38804=CARTESIAN_POINT('Ctrl Pts',(-0.218987292078664,0.00606390321575527,
-0.0104424384360514));
#38805=CARTESIAN_POINT('Ctrl Pts',(-0.218978899048671,0.00587119292257413,
-0.0104091647811685));
#38806=CARTESIAN_POINT('Ctrl Pts',(-0.218971546712785,0.00564228014000307,
-0.0103643639674548));
#38807=CARTESIAN_POINT('Ctrl Pts',(-0.218964321547142,0.00522375765311925,
-0.010269771802408));
#38808=CARTESIAN_POINT('Ctrl Pts',(-0.218969821519855,0.00476695009836949,
-0.0101384745729358));
#38809=CARTESIAN_POINT('Ctrl Pts',(-0.218991661007704,0.00425642621369877,
-0.00995497442064813));
#38810=CARTESIAN_POINT('Ctrl Pts',(-0.219014980238518,0.00391149220966936,
-0.00981293822701731));
#38811=CARTESIAN_POINT('Ctrl Pts',(-0.219044445738678,0.0035938325504786,
-0.00966808189076132));
#38812=CARTESIAN_POINT('Ctrl Pts',(-0.219084102183354,0.0032795196513945,
-0.00950851937931829));
#38813=CARTESIAN_POINT('Ctrl Pts',(-0.219118245852969,0.00307177877162768,
-0.00939505134583221));
#38814=CARTESIAN_POINT('Ctrl Pts',(-0.219192630933237,0.00268000249045626,
-0.00916667015435901));
#38815=CARTESIAN_POINT('Ctrl Pts',(-0.219270936600666,0.00233524319353199,
-0.00893798766130989));
#38816=CARTESIAN_POINT('Ctrl Pts',(-0.21933444621923,0.00208165094137429,
-0.00874770213447828));
#38817=CARTESIAN_POINT('',(-0.220398889212142,0.00187262715651618,-0.00860768688447762));
#38818=CARTESIAN_POINT('Ctrl Pts',(-0.219334462389046,0.00208158637615524,
-0.00874765368687672));
#38819=CARTESIAN_POINT('Ctrl Pts',(-0.219425793438088,0.00202206306270178,
-0.00870462918406799));
#38820=CARTESIAN_POINT('Ctrl Pts',(-0.21952774431459,0.001966817344836,
-0.00866370750595934));
#38821=CARTESIAN_POINT('Ctrl Pts',(-0.219689244178597,0.0019182609466121,
-0.00862890993327191));
#38822=CARTESIAN_POINT('Ctrl Pts',(-0.219854580810695,0.00189027043079792,
-0.00861014656253604));
#38823=CARTESIAN_POINT('Ctrl Pts',(-0.219932302779978,0.00188400419581293,
-0.00860679425156521));
#38824=CARTESIAN_POINT('Ctrl Pts',(-0.220109564738917,0.00187347457135006,
-0.00860216273510668));
#38825=CARTESIAN_POINT('Ctrl Pts',(-0.220271782826522,0.00187187244955368,
-0.00860435257401022));
#38826=CARTESIAN_POINT('Ctrl Pts',(-0.220398889374219,0.00187262610998296,
-0.00860768604747057));
#38827=CARTESIAN_POINT('',(-0.220093675868021,0.00750238722497637,-0.0105812047033426));
#38828=CARTESIAN_POINT('Ctrl Pts',(-0.220398889212142,0.00187262715651618,
-0.00860768688447762));
#38829=CARTESIAN_POINT('Ctrl Pts',(-0.220325484304193,0.00213200728749386,
-0.00881442320912016));
#38830=CARTESIAN_POINT('Ctrl Pts',(-0.220234829353635,0.00248683546590626,
-0.00906356305457854));
#38831=CARTESIAN_POINT('Ctrl Pts',(-0.220148516910183,0.00289195962917674,
-0.00931277193349481));
#38832=CARTESIAN_POINT('Ctrl Pts',(-0.220108515163862,0.00310948370060873,
-0.00943785467178893));
#38833=CARTESIAN_POINT('Ctrl Pts',(-0.220062852968177,0.00343129554586821,
-0.00960968366812658));
#38834=CARTESIAN_POINT('Ctrl Pts',(-0.220028161092074,0.00375928956199721,
-0.00976693216495996));
#38835=CARTESIAN_POINT('Ctrl Pts',(-0.2200001950355,0.00411596320034711,
-0.00992117944275958));
#38836=CARTESIAN_POINT('Ctrl Pts',(-0.219972806906522,0.00464561758738128,
-0.0101209718218955));
#38837=CARTESIAN_POINT('Ctrl Pts',(-0.219963925723449,0.00512193290843601,
-0.0102645130809962));
#38838=CARTESIAN_POINT('Ctrl Pts',(-0.219969506458366,0.00555990563946997,
-0.010368087562553));
#38839=CARTESIAN_POINT('Ctrl Pts',(-0.219976339542357,0.00579963386232449,
-0.0104171404227165));
#38840=CARTESIAN_POINT('Ctrl Pts',(-0.219984587220457,0.00600242303326202,
-0.0104536932553516));
#38841=CARTESIAN_POINT('Ctrl Pts',(-0.219990333510819,0.00611399594757277,
-0.0104717372508179));
#38842=CARTESIAN_POINT('Ctrl Pts',(-0.22000218901098,0.00632132593880884,
-0.0105027872797225));
#38843=CARTESIAN_POINT('Ctrl Pts',(-0.22002126634217,0.00660537282155696,
-0.010537762376978));
#38844=CARTESIAN_POINT('Ctrl Pts',(-0.220047872899446,0.00695409209273236,
-0.0105655599657259));
#38845=CARTESIAN_POINT('Ctrl Pts',(-0.220071923105481,0.00724852275464313,
-0.010578454459571));
#38846=CARTESIAN_POINT('Ctrl Pts',(-0.220087753192226,0.00743405295678876,
-0.0105810960015779));
#38847=CARTESIAN_POINT('Ctrl Pts',(-0.220093675868021,0.00750238722497637,
-0.0105812047033426));
#38848=CARTESIAN_POINT('',(-0.220393499421047,0.0131406655980601,-0.00859683816125004));
#38849=CARTESIAN_POINT('Ctrl Pts',(-0.220093676024769,0.00750238903348299,
-0.0105812047062192));
#38850=CARTESIAN_POINT('Ctrl Pts',(-0.220064038609195,0.0078424228712658,
-0.0105804785346465));
#38851=CARTESIAN_POINT('Ctrl Pts',(-0.220028091034243,0.00829105610092071,
-0.0105507649732036));
#38852=CARTESIAN_POINT('Ctrl Pts',(-0.22000077939978,0.00869453830083411,
-0.0105006834495053));
#38853=CARTESIAN_POINT('Ctrl Pts',(-0.219988773478308,0.00890303838725181,
-0.0104690245340275));
#38854=CARTESIAN_POINT('Ctrl Pts',(-0.219982933523342,0.00901565479908935,
-0.0104505869356331));
#38855=CARTESIAN_POINT('Ctrl Pts',(-0.219974591645721,0.00921875156863704,
-0.0104135355837661));
#38856=CARTESIAN_POINT('Ctrl Pts',(-0.219967636443395,0.00945797102713633,
-0.010364072084006));
#38857=CARTESIAN_POINT('Ctrl Pts',(-0.21996180269844,0.00989499716700375,
-0.0102597121161312));
#38858=CARTESIAN_POINT('Ctrl Pts',(-0.21997008010861,0.0103646441858166,
-0.0101174395351826));
#38859=CARTESIAN_POINT('Ctrl Pts',(-0.219997251598277,0.0108961260692111,
-0.00991623904923765));
#38860=CARTESIAN_POINT('Ctrl Pts',(-0.220025403017237,0.011254696912044,
-0.00976046818541328));
#38861=CARTESIAN_POINT('Ctrl Pts',(-0.220060403203651,0.0115850292814646,
-0.00960142209635256));
#38862=CARTESIAN_POINT('Ctrl Pts',(-0.220107259625711,0.0119132768930959,
-0.00942506124254951));
#38863=CARTESIAN_POINT('Ctrl Pts',(-0.220146529462806,0.0121263777148836,
-0.0093016756523289));
#38864=CARTESIAN_POINT('Ctrl Pts',(-0.220231925495274,0.0125296319749163,
-0.00905236487169771));
#38865=CARTESIAN_POINT('Ctrl Pts',(-0.220321219690334,0.0128823887678109,
-0.00880352703074719));
#38866=CARTESIAN_POINT('Ctrl Pts',(-0.220393499421047,0.0131406655980601,
-0.00859683816125004));
#38867=CARTESIAN_POINT('Ctrl Pts',(-0.22039358407139,0.013140991540263,
-0.00859656588824042));
#38868=CARTESIAN_POINT('Ctrl Pts',(-0.220310157492514,0.0131540633141861,
-0.00858424110404083));
#38869=CARTESIAN_POINT('Ctrl Pts',(-0.220244794120044,0.0131619399905808,
-0.00857642714207583));
#38870=CARTESIAN_POINT('Ctrl Pts',(-0.220182610404876,0.0131636989800502,
-0.00857367424019087));
#38871=CARTESIAN_POINT('Ctrl Pts',(-0.220159268269797,0.0131643592585442,
-0.0085726408730547));
#38872=CARTESIAN_POINT('Ctrl Pts',(-0.220136422298581,0.0131641674296186,
-0.00857231223501343));
#38873=CARTESIAN_POINT('Ctrl Pts',(-0.220113443370469,0.0131632181340495,
-0.00857259438936373));
#38874=CARTESIAN_POINT('Ctrl Pts',(-0.220071345066223,0.0131614789870583,
-0.00857311130728197));
#38875=CARTESIAN_POINT('Ctrl Pts',(-0.220028530403874,0.013157319506211,
-0.0085755806678843));
#38876=CARTESIAN_POINT('Ctrl Pts',(-0.219979896985917,0.0131495411313915,
-0.00858081575979762));
#38877=CARTESIAN_POINT('Ctrl Pts',(-0.219946707664722,0.0131442328682444,
-0.00858438838854329));
#38878=CARTESIAN_POINT('Ctrl Pts',(-0.219910901437945,0.0131370141276404,
-0.0085894452325124));
#38879=CARTESIAN_POINT('Ctrl Pts',(-0.219879097881105,0.0131295674172822,
-0.00859475249655793));
#38880=CARTESIAN_POINT('Ctrl Pts',(-0.21986429862666,0.0131261022148859,
-0.0085972221433152));
#38881=CARTESIAN_POINT('Ctrl Pts',(-0.21985036403865,0.013122615979583,
-0.00859972378921321));
#38882=CARTESIAN_POINT('Ctrl Pts',(-0.219837954567319,0.0131193803823998,
-0.00860205524280899));
#38883=CARTESIAN_POINT('Ctrl Pts',(-0.219798877176445,0.0131091914958259,
-0.00860939698372875));
#38884=CARTESIAN_POINT('Ctrl Pts',(-0.219774519200556,0.0131019017584804,
-0.00861468504433669));
#38885=CARTESIAN_POINT('Ctrl Pts',(-0.219741730015257,0.0130915210697872,
-0.00862222162618131));
#38886=CARTESIAN_POINT('Ctrl Pts',(-0.219708940829959,0.0130811403810939,
-0.00862975820802594));
#38887=CARTESIAN_POINT('Ctrl Pts',(-0.219667972560944,0.0130672096099914,
-0.00863991639049878));
#38888=CARTESIAN_POINT('Ctrl Pts',(-0.219624658540191,0.0130511824119699,
-0.00865158596317062));
#38889=CARTESIAN_POINT('Ctrl Pts',(-0.219538033728064,0.0130191292108723,
-0.00867492423846189));
#38890=CARTESIAN_POINT('Ctrl Pts',(-0.219442025425284,0.0129787732466052,
-0.00870422485193976));
#38891=CARTESIAN_POINT('Ctrl Pts',(-0.21932971552655,0.0129301753163333,
-0.00873889027865428));
#38892=CARTESIAN_POINT('Origin',(-0.21760795824129,0.00750000466343435,
-0.0015071771812637));
#38893=CARTESIAN_POINT('',(-0.217213394097559,0.0124661280854866,-0.0090257192728346));
#38894=CARTESIAN_POINT('',(-0.217094603491324,0.00750113103643811,-0.0105144286907592));
#38895=CARTESIAN_POINT('Ctrl Pts',(-0.217213394097559,0.0124661280854866,
-0.0090257192728346));
#38896=CARTESIAN_POINT('Ctrl Pts',(-0.21717041116494,0.0122246593680101,
-0.00918417758179821));
#38897=CARTESIAN_POINT('Ctrl Pts',(-0.217117057284765,0.0119007341084134,
-0.0093732488499977));
#38898=CARTESIAN_POINT('Ctrl Pts',(-0.21706465598238,0.0115324288885954,
-0.00956270965111247));
#38899=CARTESIAN_POINT('Ctrl Pts',(-0.217040698371939,0.0113484579716673,
-0.00965206989281391));
#38900=CARTESIAN_POINT('Ctrl Pts',(-0.217007713187453,0.0110273071878711,
-0.00979619168030236));
#38901=CARTESIAN_POINT('Ctrl Pts',(-0.216979134587681,0.0106353061403178,
-0.00995398193963724));
#38902=CARTESIAN_POINT('Ctrl Pts',(-0.216960102400533,0.0100812880088519,
-0.0101420606778224));
#38903=CARTESIAN_POINT('Ctrl Pts',(-0.216964970234854,0.00960681098718408,
-0.0102666718666015));
#38904=CARTESIAN_POINT('Ctrl Pts',(-0.216978302680794,0.00921416448670835,
-0.0103486251961947));
#38905=CARTESIAN_POINT('Ctrl Pts',(-0.21698838211439,0.00899401757483317,
-0.01038817297612));
#38906=CARTESIAN_POINT('Ctrl Pts',(-0.216999139916386,0.00879594563401397,
-0.010419159692913));
#38907=CARTESIAN_POINT('Ctrl Pts',(-0.217004856243495,0.00870275409322374,
-0.0104320663215466));
#38908=CARTESIAN_POINT('Ctrl Pts',(-0.217016574597487,0.00851987098217247,
-0.0104557992732465));
#38909=CARTESIAN_POINT('Ctrl Pts',(-0.217040946256797,0.00817310207656308,
-0.0104923571850839));
#38910=CARTESIAN_POINT('Ctrl Pts',(-0.217070785262386,0.00778990612293632,
-0.0105138775080055));
#38911=CARTESIAN_POINT('Ctrl Pts',(-0.217094604240616,0.00750113159837561,
-0.010514428709891));
#38912=CARTESIAN_POINT('',(-0.217217196076401,0.00253915440696052,-0.00902927251451939));
#38913=CARTESIAN_POINT('Ctrl Pts',(-0.217094604204801,0.00750113097791163,
-0.0105144287091931));
#38914=CARTESIAN_POINT('Ctrl Pts',(-0.217084161848402,0.00737376523387638,
-0.0105142185903619));
#38915=CARTESIAN_POINT('Ctrl Pts',(-0.217060477387662,0.00707794301303083,
-0.01050688284421));
#38916=CARTESIAN_POINT('Ctrl Pts',(-0.217034564919892,0.00673221457752508,
-0.0104821172122667));
#38917=CARTESIAN_POINT('Ctrl Pts',(-0.217017123930288,0.00648242698557118,
-0.0104560964710192));
#38918=CARTESIAN_POINT('Ctrl Pts',(-0.217005554768794,0.00629995272480641,
-0.0104324364268733));
#38919=CARTESIAN_POINT('Ctrl Pts',(-0.216999885759004,0.00620651112707121,
-0.0104195265524636));
#38920=CARTESIAN_POINT('Ctrl Pts',(-0.216989325922178,0.00600939813741562,
-0.0103887567565715));
#38921=CARTESIAN_POINT('Ctrl Pts',(-0.216979430273025,0.00578936969628363,
-0.0103493264841639));
#38922=CARTESIAN_POINT('Ctrl Pts',(-0.216966473873743,0.00539729869136527,
-0.0102676831160186));
#38923=CARTESIAN_POINT('Ctrl Pts',(-0.216962156491798,0.00492156112687701,
-0.0101429282776497));
#38924=CARTESIAN_POINT('Ctrl Pts',(-0.216981833480707,0.00436966098887771,
-0.00995584505032058));
#38925=CARTESIAN_POINT('Ctrl Pts',(-0.217010842686626,0.00397750116182149,
-0.0097983012137332));
#38926=CARTESIAN_POINT('Ctrl Pts',(-0.217044214738291,0.00365555388525719,
-0.00965402891301301));
#38927=CARTESIAN_POINT('Ctrl Pts',(-0.217068262983783,0.00347186850781422,
-0.00956491767776186));
#38928=CARTESIAN_POINT('Ctrl Pts',(-0.21712081802361,0.00310386192693681,
-0.0093758711515526));
#38929=CARTESIAN_POINT('Ctrl Pts',(-0.217174218047225,0.00278029120291905,
-0.00918727068287094));
#38930=CARTESIAN_POINT('Ctrl Pts',(-0.217217196076401,0.00253915440696052,
-0.00902927251451939));
#38931=CARTESIAN_POINT('',(-0.218253133349592,0.00235141795600442,-0.00892454475911964));
#38932=CARTESIAN_POINT('Ctrl Pts',(-0.217217809477599,0.00253896772880568,
-0.0090293011698677));
#38933=CARTESIAN_POINT('Ctrl Pts',(-0.217290041369587,0.00250069176491746,
-0.00900556706915477));
#38934=CARTESIAN_POINT('Ctrl Pts',(-0.217368407052876,0.0024671494138073,
-0.00898467489825882));
#38935=CARTESIAN_POINT('Ctrl Pts',(-0.217450359266991,0.00244089398796864,
-0.00896864143762584));
#38936=CARTESIAN_POINT('Ctrl Pts',(-0.217491335374049,0.0024277662750493,
-0.00896062470730935));
#38937=CARTESIAN_POINT('Ctrl Pts',(-0.217533055849,0.00241628436709229,
-0.00895369982738143));
#38938=CARTESIAN_POINT('Ctrl Pts',(-0.217580470128854,0.00240565996459356,
-0.00894744657919007));
#38939=CARTESIAN_POINT('Ctrl Pts',(-0.217627884408709,0.00239503556209484,
-0.00894119333099871));
#38940=CARTESIAN_POINT('Ctrl Pts',(-0.21768122272973,0.00238589707961749,
-0.00893604813963404));
#38941=CARTESIAN_POINT('Ctrl Pts',(-0.217720667840838,0.00238036482543931,
-0.00893308565286313));
#38942=CARTESIAN_POINT('Ctrl Pts',(-0.21772785791221,0.00237935640383077,
-0.00893254564953383));
#38943=CARTESIAN_POINT('Ctrl Pts',(-0.217734589088163,0.00237845246471081,
-0.00893206729807201));
#38944=CARTESIAN_POINT('Ctrl Pts',(-0.217740992213186,0.00237762157144803,
-0.00893163189219981));
#38945=CARTESIAN_POINT('Ctrl Pts',(-0.217769716970056,0.00237389414040906,
-0.0089296786384724));
#38946=CARTESIAN_POINT('Ctrl Pts',(-0.217791731404344,0.00237149849359442,
-0.00892849060637797));
#38947=CARTESIAN_POINT('Ctrl Pts',(-0.217819659624921,0.00236886316801429,
-0.00892726140202061));
#38948=CARTESIAN_POINT('Ctrl Pts',(-0.217853813412136,0.0023656403938008,
-0.00892575819189133));
#38949=CARTESIAN_POINT('Ctrl Pts',(-0.21789677874394,0.00236237522790454,
-0.0089244180371867));
#38950=CARTESIAN_POINT('Ctrl Pts',(-0.217942798021502,0.00235987579789025,
-0.0089236782831972));
#38951=CARTESIAN_POINT('Ctrl Pts',(-0.218032838016481,0.00235498548500703,
-0.00892223090181643));
#38952=CARTESIAN_POINT('Ctrl Pts',(-0.218134518988832,0.00235293450087632,
-0.00892302018243319));
#38953=CARTESIAN_POINT('Ctrl Pts',(-0.218253133349592,0.00235141795600442,
-0.00892454475911964));
#38954=CARTESIAN_POINT('',(-0.218094235237686,0.00750143446742459,-0.0105360562554827));
#38955=CARTESIAN_POINT('Ctrl Pts',(-0.218253133066283,0.00235141263875458,
-0.00892455212338305));
#38956=CARTESIAN_POINT('Ctrl Pts',(-0.218214219872793,0.00253247183269533,
-0.00904968294283068));
#38957=CARTESIAN_POINT('Ctrl Pts',(-0.218179081459859,0.00271867387981424,
-0.00916861222376044));
#38958=CARTESIAN_POINT('Ctrl Pts',(-0.21803449218446,0.00360160792485018,
-0.00968787065959727));
#38959=CARTESIAN_POINT('Ctrl Pts',(-0.217972979168045,0.00434860675246558,
-0.0100034645917515));
#38960=CARTESIAN_POINT('Ctrl Pts',(-0.217957033748206,0.00590729686837615,
-0.0104276715988628));
#38961=CARTESIAN_POINT('Ctrl Pts',(-0.218001909352134,0.00670430387980213,
-0.0105340609659123));
#38962=CARTESIAN_POINT('Ctrl Pts',(-0.218097813131851,0.00750001270663325,
-0.0105361337811779));
#38963=CARTESIAN_POINT('',(-0.2182565110078,0.0126543573605341,-0.00892058764987726));
#38964=CARTESIAN_POINT('Ctrl Pts',(-0.218094235237686,0.00750143446742459,
-0.0105360562554827));
#38965=CARTESIAN_POINT('Ctrl Pts',(-0.218067105154875,0.00780677055571136,
-0.0105354203113047));
#38966=CARTESIAN_POINT('Ctrl Pts',(-0.218033831405312,0.00820961502316317,
-0.0105114742256329));
#38967=CARTESIAN_POINT('Ctrl Pts',(-0.218007882474728,0.00857238380872824,
-0.0104711475163477));
#38968=CARTESIAN_POINT('Ctrl Pts',(-0.217996152558159,0.00875980809131382,
-0.0104456876420246));
#38969=CARTESIAN_POINT('Ctrl Pts',(-0.217990313058703,0.00886144379089272,
-0.0104307972172058));
#38970=CARTESIAN_POINT('Ctrl Pts',(-0.217981597968648,0.00904302164651337,
-0.0104011947822263));
#38971=CARTESIAN_POINT('Ctrl Pts',(-0.217973528732665,0.00925803386380941,
-0.0103615120623033));
#38972=CARTESIAN_POINT('Ctrl Pts',(-0.217964102590318,0.0096505431499046,
-0.010278050687789));
#38973=CARTESIAN_POINT('Ctrl Pts',(-0.217965530958217,0.0101943339463829,
-0.0101316150791819));
#38974=CARTESIAN_POINT('Ctrl Pts',(-0.217989853133676,0.0107921989301394,
-0.00991655019287694));
#38975=CARTESIAN_POINT('Ctrl Pts',(-0.218020475341655,0.0111925938083483,
-0.0097457526023216));
#38976=CARTESIAN_POINT('Ctrl Pts',(-0.218052426173444,0.0114968851846426,
-0.00960217923509529));
#38977=CARTESIAN_POINT('Ctrl Pts',(-0.218079973263592,0.0116953987503668,
-0.00950129475060471));
#38978=CARTESIAN_POINT('Ctrl Pts',(-0.218140496279061,0.0120732358289631,
-0.00929682365052865));
#38979=CARTESIAN_POINT('Ctrl Pts',(-0.218204497408712,0.0124072068218569,
-0.00909170879414502));
#38980=CARTESIAN_POINT('Ctrl Pts',(-0.2182565110078,0.0126543573605341,
-0.00892058764987726));
#38981=CARTESIAN_POINT('Ctrl Pts',(-0.218256501705708,0.0126543585852145,
-0.00892058659399183));
#38982=CARTESIAN_POINT('Ctrl Pts',(-0.218154525997755,0.0126678026917317,
-0.00890901246260343));
#38983=CARTESIAN_POINT('Ctrl Pts',(-0.218078194794121,0.0126730947409307,
-0.00890364142665837));
#38984=CARTESIAN_POINT('Ctrl Pts',(-0.217909752747571,0.0126633106168309,
-0.00890684541098475));
#38985=CARTESIAN_POINT('Ctrl Pts',(-0.217821972872918,0.0126501072829163,
-0.00891420792415138));
#38986=CARTESIAN_POINT('Ctrl Pts',(-0.21754967081416,0.0125870145067814,
-0.00895194276125938));
#38987=CARTESIAN_POINT('Ctrl Pts',(-0.217380015618932,0.0125265412057645,
-0.00898944383847723));
#38988=CARTESIAN_POINT('Ctrl Pts',(-0.217213440148644,0.0124661800217875,
-0.009025685986326));
#38989=CARTESIAN_POINT('Origin',(-0.215572945664865,0.00750000047003143,
-0.00143236497997678));
#38990=CARTESIAN_POINT('',(-0.215184743945676,0.012323689646171,-0.00907719137595261));
#38991=CARTESIAN_POINT('',(-0.215095211258851,0.00750052176516078,-0.010469157777843));
#38992=CARTESIAN_POINT('Ctrl Pts',(-0.215184743945676,0.012323689646171,
-0.00907719137595261));
#38993=CARTESIAN_POINT('Ctrl Pts',(-0.21514648660725,0.0120862670790848,
-0.00922607274352441));
#38994=CARTESIAN_POINT('Ctrl Pts',(-0.215099018442826,0.0117687123887809,
-0.00940346464373393));
#38995=CARTESIAN_POINT('Ctrl Pts',(-0.215052369462544,0.0114082657322194,
-0.00958112131941231));
#38996=CARTESIAN_POINT('Ctrl Pts',(-0.215031100534081,0.0112292263444702,
-0.00966451563804252));
#38997=CARTESIAN_POINT('Ctrl Pts',(-0.21500151205561,0.0109134744577964,
-0.00980042007136559));
#38998=CARTESIAN_POINT('Ctrl Pts',(-0.214976322453243,0.0105309593786002,
-0.00994796510360923));
#38999=CARTESIAN_POINT('Ctrl Pts',(-0.214960394330003,0.00999902377695271,
-0.0101215370958852));
#39000=CARTESIAN_POINT('Ctrl Pts',(-0.214966324260738,0.00953215587950937,
-0.0102394787165332));
#39001=CARTESIAN_POINT('Ctrl Pts',(-0.214980033976025,0.00915301666182799,
-0.0103153885509512));
#39002=CARTESIAN_POINT('Ctrl Pts',(-0.214990161391655,0.00894081415800363,
-0.0103520081134918));
#39003=CARTESIAN_POINT('Ctrl Pts',(-0.215000843349877,0.0087507069385728,
-0.0103805993488392));
#39004=CARTESIAN_POINT('Ctrl Pts',(-0.215006529173423,0.00866069457107862,
-0.0103925976782496));
#39005=CARTESIAN_POINT('Ctrl Pts',(-0.215018149652307,0.00848438866324892,
-0.0104146108210603));
#39006=CARTESIAN_POINT('Ctrl Pts',(-0.215042272034264,0.00814969066011635,
-0.0104485878385499));
#39007=CARTESIAN_POINT('Ctrl Pts',(-0.215071730086938,0.00777959042738062,
-0.0104686311967555));
#39008=CARTESIAN_POINT('Ctrl Pts',(-0.215095211712589,0.00750052238910928,
-0.0104691577890294));
#39009=CARTESIAN_POINT('',(-0.215187317923645,0.00267870325034433,-0.00907875410590838));
#39010=CARTESIAN_POINT('Ctrl Pts',(-0.215095211657488,0.00750052173172372,
-0.0104691577878692));
#39011=CARTESIAN_POINT('Ctrl Pts',(-0.215093348816256,0.0074782969939577,
-0.0104691185637939));
#39012=CARTESIAN_POINT('Ctrl Pts',(-0.215086094585673,0.00739134142684377,
-0.0104685644526724));
#39013=CARTESIAN_POINT('Ctrl Pts',(-0.215075843703081,0.00726661667161012,
-0.0104660613626304));
#39014=CARTESIAN_POINT('Ctrl Pts',(-0.215057434122424,0.00703872552940382,
-0.0104581862817437));
#39015=CARTESIAN_POINT('Ctrl Pts',(-0.215035586165921,0.00675491463768686,
-0.0104388446803273));
#39016=CARTESIAN_POINT('Ctrl Pts',(-0.215018376650014,0.00651490499106983,
-0.0104145485250919));
#39017=CARTESIAN_POINT('Ctrl Pts',(-0.215006844975634,0.00633859231783919,
-0.01039251067607));
#39018=CARTESIAN_POINT('Ctrl Pts',(-0.215001196968655,0.00624840215077872,
-0.0103804808191619));
#39019=CARTESIAN_POINT('Ctrl Pts',(-0.214990660376026,0.00605883545559521,
-0.0103519593738021));
#39020=CARTESIAN_POINT('Ctrl Pts',(-0.214980672161886,0.00584665249207341,
-0.0103153399439608));
#39021=CARTESIAN_POINT('Ctrl Pts',(-0.214967245748183,0.00546782162430372,
-0.0102394950560305));
#39022=CARTESIAN_POINT('Ctrl Pts',(-0.214961732355427,0.00500012678372268,
-0.0101213055392285));
#39023=CARTESIAN_POINT('Ctrl Pts',(-0.214978156077839,0.00446989750802472,
-0.00994828915619471));
#39024=CARTESIAN_POINT('Ctrl Pts',(-0.215003681155038,0.00408735391033809,
-0.00980081329302173));
#39025=CARTESIAN_POINT('Ctrl Pts',(-0.215033590721385,0.00377091209053468,
-0.00966463271638572));
#39026=CARTESIAN_POINT('Ctrl Pts',(-0.215054895180567,0.00359250015699713,
-0.00958153380973349));
#39027=CARTESIAN_POINT('Ctrl Pts',(-0.215101625155304,0.00323264763109776,
-0.0094042312271201));
#39028=CARTESIAN_POINT('Ctrl Pts',(-0.21514908525396,0.00291571044311647,
-0.00922727046007243));
#39029=CARTESIAN_POINT('Ctrl Pts',(-0.215187317923645,0.00267870325034433,
-0.00907875410590838));
#39030=CARTESIAN_POINT('',(-0.216194991836357,0.00264076678978001,-0.00907662738373749));
#39031=CARTESIAN_POINT('Ctrl Pts',(-0.215187406628623,0.00267868409859472,
-0.00907874392743814));
#39032=CARTESIAN_POINT('Ctrl Pts',(-0.21552326791646,0.00266602963457283,
-0.00907807250913494));
#39033=CARTESIAN_POINT('Ctrl Pts',(-0.215859129663761,0.00265338920072677,
-0.0090773662716867));
#39034=CARTESIAN_POINT('Ctrl Pts',(-0.21619499193747,0.00264076476354384,
-0.00907662607383746));
#39035=CARTESIAN_POINT('',(-0.216094920727691,0.00750081535589013,-0.0104908925867836));
#39036=CARTESIAN_POINT('Ctrl Pts',(-0.216194991836357,0.00264076678978001,
-0.00907662738373749));
#39037=CARTESIAN_POINT('Ctrl Pts',(-0.216155366004592,0.00288037027759099,
-0.00922841667383286));
#39038=CARTESIAN_POINT('Ctrl Pts',(-0.216106174921698,0.00320114029982177,
-0.00940926923509961));
#39039=CARTESIAN_POINT('Ctrl Pts',(-0.216057819495052,0.00356499889891992,
-0.009590150528347));
#39040=CARTESIAN_POINT('Ctrl Pts',(-0.216035682401327,0.00374666276300005,
-0.00967541861388872));
#39041=CARTESIAN_POINT('Ctrl Pts',(-0.21600516202416,0.00406273234928654,
-0.0098125207512195));
#39042=CARTESIAN_POINT('Ctrl Pts',(-0.215978862788875,0.00444643562956339,
-0.00996170720449533));
#39043=CARTESIAN_POINT('Ctrl Pts',(-0.215961627981838,0.00497762456890586,
-0.0101366227379806));
#39044=CARTESIAN_POINT('Ctrl Pts',(-0.215966673091261,0.00544925004400758,
-0.0102570027663552));
#39045=CARTESIAN_POINT('Ctrl Pts',(-0.215979918232889,0.00583091044504249,
-0.010334140462034));
#39046=CARTESIAN_POINT('Ctrl Pts',(-0.21598984730753,0.00604476982194863,
-0.0103714130964631));
#39047=CARTESIAN_POINT('Ctrl Pts',(-0.216000365432515,0.00623593452875368,
-0.0104004595092437));
#39048=CARTESIAN_POINT('Ctrl Pts',(-0.216006025580804,0.00632705052741814,
-0.0104127398163461));
#39049=CARTESIAN_POINT('Ctrl Pts',(-0.216017604486095,0.00650523993901912,
-0.0104352082840549));
#39050=CARTESIAN_POINT('Ctrl Pts',(-0.21604165432455,0.00684284821730302,
-0.0104699298205827));
#39051=CARTESIAN_POINT('Ctrl Pts',(-0.216071599729952,0.00722182610486624,
-0.0104904107732437));
#39052=CARTESIAN_POINT('Ctrl Pts',(-0.216094920728811,0.00750081502625171,
-0.0104908925868377));
#39053=CARTESIAN_POINT('',(-0.216191681155669,0.0123629325401175,-0.00907419422952278));
#39054=CARTESIAN_POINT('Ctrl Pts',(-0.216094920727691,0.00750081535589013,
-0.0104908925867836));
#39055=CARTESIAN_POINT('Ctrl Pts',(-0.21607114795769,0.00778396749876566,
-0.0104903501412173));
#39056=CARTESIAN_POINT('Ctrl Pts',(-0.216041367011789,0.00815931797022712,
-0.0104697259238784));
#39057=CARTESIAN_POINT('Ctrl Pts',(-0.216017038090091,0.00849870004219069,
-0.0104347690624456));
#39058=CARTESIAN_POINT('Ctrl Pts',(-0.216005363149858,0.00867711965280929,
-0.0104121793506864));
#39059=CARTESIAN_POINT('Ctrl Pts',(-0.21599962253345,0.00876887272456124,
-0.0103997619303256));
#39060=CARTESIAN_POINT('Ctrl Pts',(-0.215989057163612,0.0089590976354752,
-0.0103707564576226));
#39061=CARTESIAN_POINT('Ctrl Pts',(-0.215979036512872,0.00917200431861489,
-0.0103335666094436));
#39062=CARTESIAN_POINT('Ctrl Pts',(-0.215965573411188,0.00955218224306641,
-0.01025658134513));
#39063=CARTESIAN_POINT('Ctrl Pts',(-0.215959983300432,0.0100198628373282,
-0.0101373332269741));
#39064=CARTESIAN_POINT('Ctrl Pts',(-0.215976608750281,0.0105552916003265,
-0.00996109009686354));
#39065=CARTESIAN_POINT('Ctrl Pts',(-0.216002575783096,0.0109398514635131,
-0.00981140744813802));
#39066=CARTESIAN_POINT('Ctrl Pts',(-0.216032886151583,0.0112567101897491,
-0.00967382351912691));
#39067=CARTESIAN_POINT('Ctrl Pts',(-0.216054884878806,0.0114382008550471,
-0.00958853634620765));
#39068=CARTESIAN_POINT('Ctrl Pts',(-0.216103051979017,0.0118022669367451,
-0.00940736798328436));
#39069=CARTESIAN_POINT('Ctrl Pts',(-0.216152125740651,0.0121231895976479,
-0.00922623781176936));
#39070=CARTESIAN_POINT('Ctrl Pts',(-0.216191681155669,0.0123629325401175,
-0.00907419422952278));
#39071=CARTESIAN_POINT('Ctrl Pts',(-0.216191679984792,0.0123629610678733,
-0.00907417531574932));
#39072=CARTESIAN_POINT('Ctrl Pts',(-0.215856063870635,0.0123498846849188,
-0.00907522003451906));
#39073=CARTESIAN_POINT('Ctrl Pts',(-0.215520448246673,0.0123367926637154,
-0.00907622680850737));
#39074=CARTESIAN_POINT('Ctrl Pts',(-0.215184833018176,0.0123236876257974,
-0.00907719458563817));
#39075=CARTESIAN_POINT('Origin',(-0.191548193502062,0.0075000009419683,
-0.000492621109443556));
#39076=CARTESIAN_POINT('',(-0.192104402373237,0.00750389176243192,-0.00994933158139058));
#39077=CARTESIAN_POINT('',(-0.192122530472206,0.0119802570120685,-0.00881815091622089));
#39078=CARTESIAN_POINT('Ctrl Pts',(-0.192108734077425,0.00750469088463491,
-0.00994879424709136));
#39079=CARTESIAN_POINT('Ctrl Pts',(-0.192103207711712,0.0075509068388887,
-0.00994865116432292));
#39080=CARTESIAN_POINT('Ctrl Pts',(-0.192097845739629,0.00759714834567246,
-0.00994817223080437));
#39081=CARTESIAN_POINT('Ctrl Pts',(-0.191980221684322,0.00864423060253309,
-0.00992970587840616));
#39082=CARTESIAN_POINT('Ctrl Pts',(-0.191946432880569,0.00963929255173959,
-0.00975446086017676));
#39083=CARTESIAN_POINT('Ctrl Pts',(-0.192015568180551,0.0110713112592102,
-0.00926000378799105));
#39084=CARTESIAN_POINT('Ctrl Pts',(-0.192059160699483,0.0115364242758858,
-0.00905610534302461));
#39085=CARTESIAN_POINT('Ctrl Pts',(-0.192122341662653,0.0119805125490225,
-0.00881800902404164));
#39086=CARTESIAN_POINT('',(-0.191053645153712,0.0113981655634775,-0.00908339543415031));
#39087=CARTESIAN_POINT('Ctrl Pts',(-0.192122530472206,0.0119802570120685,
-0.00881815091622089));
#39088=CARTESIAN_POINT('Ctrl Pts',(-0.19199161678884,0.0119322240752818,
-0.0088412067577884));
#39089=CARTESIAN_POINT('Ctrl Pts',(-0.191879939462572,0.0118894807233055,
-0.00886131310476818));
#39090=CARTESIAN_POINT('Ctrl Pts',(-0.191781985634829,0.0118492817294659,
-0.00888005248158014));
#39091=CARTESIAN_POINT('Ctrl Pts',(-0.191732121208329,0.011828818008753,
-0.00888959195848701));
#39092=CARTESIAN_POINT('Ctrl Pts',(-0.191685813361322,0.0118090078712822,
-0.00889876632261227));
#39093=CARTESIAN_POINT('Ctrl Pts',(-0.191648874008136,0.0117929042881476,
-0.00890618640190862));
#39094=CARTESIAN_POINT('Ctrl Pts',(-0.191611934654949,0.0117768007050129,
-0.00891360648120497));
#39095=CARTESIAN_POINT('Ctrl Pts',(-0.191584363162224,0.0117644186426757,
-0.00891930142696703));
#39096=CARTESIAN_POINT('Ctrl Pts',(-0.19154291056778,0.0117435795925307,
-0.00892888798659096));
#39097=CARTESIAN_POINT('Ctrl Pts',(-0.191501457973336,0.0117227405423857,
-0.00893847454621488));
#39098=CARTESIAN_POINT('Ctrl Pts',(-0.191446125407219,0.0116934182420501,
-0.00895190070791356));
#39099=CARTESIAN_POINT('Ctrl Pts',(-0.191397663363911,0.0116652096291388,
-0.00896471741532005));
#39100=CARTESIAN_POINT('Ctrl Pts',(-0.191349201320603,0.0116370010162275,
-0.00897753412272655));
#39101=CARTESIAN_POINT('Ctrl Pts',(-0.191307608992891,0.0116099242324839,
-0.0089897785286841));
#39102=CARTESIAN_POINT('Ctrl Pts',(-0.191267699831175,0.0115815575659545,
-0.00900251346495063));
#39103=CARTESIAN_POINT('Ctrl Pts',(-0.1911878850761,0.0115248267692159,
-0.00902798219882765));
#39104=CARTESIAN_POINT('Ctrl Pts',(-0.191114803398555,0.0114629153130397,
-0.00905536613897805));
#39105=CARTESIAN_POINT('Ctrl Pts',(-0.191053645153712,0.0113981655634775,
-0.00908339543415031));
#39106=CARTESIAN_POINT('',(-0.191102317990465,0.00750205528623176,-0.00992689696933848));
#39107=CARTESIAN_POINT('Ctrl Pts',(-0.191053667625411,0.0113981565442571,
-0.00908340001178101));
#39108=CARTESIAN_POINT('Ctrl Pts',(-0.191051193363694,0.0113718165320938,
-0.00909528900497808));
#39109=CARTESIAN_POINT('Ctrl Pts',(-0.191048779622539,0.0113454205791333,
-0.0091070587574167));
#39110=CARTESIAN_POINT('Ctrl Pts',(-0.190954175177597,0.0102820119819883,
-0.00957542619835343));
#39111=CARTESIAN_POINT('Ctrl Pts',(-0.190955921046233,0.00917583914081459,
-0.00984130463999999));
#39112=CARTESIAN_POINT('Ctrl Pts',(-0.191064314723308,0.0078705269708081,
-0.00992065058137066));
#39113=CARTESIAN_POINT('Ctrl Pts',(-0.191082145256522,0.00768562531559786,
-0.00992646114623245));
#39114=CARTESIAN_POINT('Ctrl Pts',(-0.191102363522027,0.00750132035680661,
-0.00992692622707289));
#39115=CARTESIAN_POINT('',(-0.191055938690558,0.00361094738279529,-0.00908764566835488));
#39116=CARTESIAN_POINT('Ctrl Pts',(-0.191104123278973,0.00750132061311004,
-0.00992696446771463));
#39117=CARTESIAN_POINT('Ctrl Pts',(-0.19106845003887,0.00717518850570648,
-0.00992623479437091));
#39118=CARTESIAN_POINT('Ctrl Pts',(-0.191040610403852,0.00685082501865862,
-0.0099087736553339));
#39119=CARTESIAN_POINT('Ctrl Pts',(-0.190956197985429,0.00550729994350422,
-0.0097680742307451));
#39120=CARTESIAN_POINT('Ctrl Pts',(-0.190969527586036,0.00452315153618091,
-0.00949802905279705));
#39121=CARTESIAN_POINT('Ctrl Pts',(-0.191054063007182,0.00361171883661926,
-0.00908787631838634));
#39122=CARTESIAN_POINT('',(-0.192132222592215,0.00302368985652182,-0.0088204938392334));
#39123=CARTESIAN_POINT('Ctrl Pts',(-0.191056694227376,0.00361001886952257,
-0.00908716487649774));
#39124=CARTESIAN_POINT('Ctrl Pts',(-0.191117646682474,0.00354507577298782,
-0.00905911829100523));
#39125=CARTESIAN_POINT('Ctrl Pts',(-0.191190576613973,0.003482977172259,
-0.00903171364009081));
#39126=CARTESIAN_POINT('Ctrl Pts',(-0.191270285221213,0.00342607672119435,
-0.00900622453480157));
#39127=CARTESIAN_POINT('Ctrl Pts',(-0.191310139525385,0.00339762649526841,
-0.00899347998198063));
#39128=CARTESIAN_POINT('Ctrl Pts',(-0.191351688242736,0.00337047038354003,
-0.00898122608515244));
#39129=CARTESIAN_POINT('Ctrl Pts',(-0.19140012564909,0.00334217558575491,
-0.0089683974383084));
#39130=CARTESIAN_POINT('Ctrl Pts',(-0.191448563055443,0.00331388078796979,
-0.00895556879146436));
#39131=CARTESIAN_POINT('Ctrl Pts',(-0.191503889964036,0.00328446553423945,
-0.00894212797770866));
#39132=CARTESIAN_POINT('Ctrl Pts',(-0.191545324948472,0.00326357080218557,
-0.00893253552891437));
#39133=CARTESIAN_POINT('Ctrl Pts',(-0.191586759932908,0.00324267607013168,
-0.00892294308012008));
#39134=CARTESIAN_POINT('Ctrl Pts',(-0.191614301855269,0.00323027547924158,
-0.00891725135146682));
#39135=CARTESIAN_POINT('Ctrl Pts',(-0.191651228210345,0.00321413808329353,
-0.00890983105241841));
#39136=CARTESIAN_POINT('Ctrl Pts',(-0.191688154565421,0.00319800068734548,
-0.00890241075337));
#39137=CARTESIAN_POINT('Ctrl Pts',(-0.1917344659906,0.00317814151164943,
-0.00889323255797904));
#39138=CARTESIAN_POINT('Ctrl Pts',(-0.191784343440197,0.00315762666347515,
-0.00888368869751462));
#39139=CARTESIAN_POINT('Ctrl Pts',(-0.19188409833939,0.0031165969671266,
-0.00886460097658579));
#39140=CARTESIAN_POINT('Ctrl Pts',(-0.191998116385108,0.00307292140876782,
-0.00884409435676829));
#39141=CARTESIAN_POINT('Ctrl Pts',(-0.192132222764199,0.00302369025826422,
-0.00882049405934325));
#39142=CARTESIAN_POINT('Ctrl Pts',(-0.192132222592215,0.00302368985652182,
-0.0088204938392334));
#39143=CARTESIAN_POINT('Ctrl Pts',(-0.192103791504356,0.00325082082607522,
-0.00894220488147181));
#39144=CARTESIAN_POINT('Ctrl Pts',(-0.192068646087494,0.00355203440365802,
-0.00908672318139968));
#39145=CARTESIAN_POINT('Ctrl Pts',(-0.192034396050521,0.00389166889704801,
-0.00923113586730494));
#39146=CARTESIAN_POINT('Ctrl Pts',(-0.19201895526882,0.00405874480199876,
-0.00929842428009787));
#39147=CARTESIAN_POINT('Ctrl Pts',(-0.191997619334613,0.0043567261598758,
-0.0094095168730219));
#39148=CARTESIAN_POINT('Ctrl Pts',(-0.191980450765341,0.00471410316628912,
-0.00952906101135592));
#39149=CARTESIAN_POINT('Ctrl Pts',(-0.191971848059539,0.00520369664809944,
-0.00966821105761361));
#39150=CARTESIAN_POINT('Ctrl Pts',(-0.191980537392393,0.00563814596492265,
-0.00976411773704245));
#39151=CARTESIAN_POINT('Ctrl Pts',(-0.191994962083258,0.00598633526148447,
-0.00982505229803761));
#39152=CARTESIAN_POINT('Ctrl Pts',(-0.192005079326421,0.00618120430706718,
-0.00985448438518454));
#39153=CARTESIAN_POINT('Ctrl Pts',(-0.192015400395759,0.00635425493589708,
-0.00987729266943201));
#39154=CARTESIAN_POINT('Ctrl Pts',(-0.19202086841947,0.00643706239649949,
-0.00988698789097493));
#39155=CARTESIAN_POINT('Ctrl Pts',(-0.192031975743343,0.0065989007730196,
-0.0099047027533171));
#39156=CARTESIAN_POINT('Ctrl Pts',(-0.192048185086397,0.00681719200235256,
-0.00992426365281129));
#39157=CARTESIAN_POINT('Ctrl Pts',(-0.192069332648122,0.0070838409743984,
-0.00993985662063671));
#39158=CARTESIAN_POINT('Ctrl Pts',(-0.192085638344594,0.00728158938794661,
-0.00994618972545213));
#39159=CARTESIAN_POINT('Ctrl Pts',(-0.192096778314419,0.00741407240370789,
-0.009948236681352));
#39160=CARTESIAN_POINT('Ctrl Pts',(-0.192100401188873,0.00745684365403462,
-0.00994862837396258));
#39161=CARTESIAN_POINT('Ctrl Pts',(-0.192104337739042,0.00750296369756609,
-0.00994869941298362));
#39162=CARTESIAN_POINT('Origin',(-0.22657497719928,0.0105076883533885,0.00733431533838148));
#39163=CARTESIAN_POINT('Ctrl Pts',(-0.225970553562738,0.0102603089488576,
0.0102745179149678));
#39164=CARTESIAN_POINT('Ctrl Pts',(-0.225969704710384,0.010270943438745,
0.0103064390545693));
#39165=CARTESIAN_POINT('Ctrl Pts',(-0.225968879295254,0.0102817420965276,
0.0103382186548783));
#39166=CARTESIAN_POINT('Ctrl Pts',(-0.225968077478529,0.0102926941256055,
0.0103698341560209));
#39167=CARTESIAN_POINT('Ctrl Pts',(-0.226088480400989,0.00749337594554441,
0.0108173434082515));
#39168=CARTESIAN_POINT('Ctrl Pts',(-0.226091023274651,0.00749377529304714,
0.0107836282080371));
#39169=CARTESIAN_POINT('Ctrl Pts',(-0.226093596038501,0.00749416765923866,
0.0107499145846004));
#39170=CARTESIAN_POINT('Ctrl Pts',(-0.226096198745771,0.00749455297790887,
0.0107162215195238));
#39171=CARTESIAN_POINT('Origin',(-0.226550254959384,0.00452042011638252,
0.00737614095179629));
#39172=CARTESIAN_POINT('Origin',(-0.203567794470365,0.00749999935701362,
0.000977046461186483));
#39173=CARTESIAN_POINT('',(-0.203099755569153,0.00751239992371187,0.0102033423261815));
#39174=CARTESIAN_POINT('',(-0.203180925911572,0.00274255958650594,0.00887885017805646));
#39175=CARTESIAN_POINT('Ctrl Pts',(-0.203180925911572,0.00274255958650594,
0.00887885017805646));
#39176=CARTESIAN_POINT('Ctrl Pts',(-0.203144430180515,0.00297855990713514,
0.00902006318418588));
#39177=CARTESIAN_POINT('Ctrl Pts',(-0.203099100468265,0.00329328958382362,
0.00918815539817035));
#39178=CARTESIAN_POINT('Ctrl Pts',(-0.203054332460607,0.00365027651704815,
0.00935661910300519));
#39179=CARTESIAN_POINT('Ctrl Pts',(-0.203033957671154,0.00382624548473899,
0.00943519574639222));
#39180=CARTESIAN_POINT('Ctrl Pts',(-0.203004894631343,0.0041419656001032,
0.00956548767658879));
#39181=CARTESIAN_POINT('Ctrl Pts',(-0.202980280894576,0.00452088750482505,
0.00970547640495058));
#39182=CARTESIAN_POINT('Ctrl Pts',(-0.202964648697527,0.00503857041836433,
0.00986783483593268));
#39183=CARTESIAN_POINT('Ctrl Pts',(-0.20297036150819,0.00550510267309646,
0.00998125540777899));
#39184=CARTESIAN_POINT('Ctrl Pts',(-0.202983860319937,0.00587653496273335,
0.0100526595036212));
#39185=CARTESIAN_POINT('Ctrl Pts',(-0.202993842688538,0.00608408581120754,
0.010087118293265));
#39186=CARTESIAN_POINT('Ctrl Pts',(-0.203004352694453,0.00626908343786698,
0.0101139235131616));
#39187=CARTESIAN_POINT('Ctrl Pts',(-0.203010023447602,0.00635758963013911,
0.0101253105115554));
#39188=CARTESIAN_POINT('Ctrl Pts',(-0.203021614388977,0.00653051337351625,
0.0101461407131562));
#39189=CARTESIAN_POINT('Ctrl Pts',(-0.203045798331806,0.00685963984035563,
0.0101784216117505));
#39190=CARTESIAN_POINT('Ctrl Pts',(-0.203075452970359,0.00722429942668557,
0.0101975556471434));
#39191=CARTESIAN_POINT('Ctrl Pts',(-0.203099127134863,0.00749962060040461,
0.0101980805626216));
#39192=CARTESIAN_POINT('',(-0.203173150554077,0.0122530887858704,0.00888129623516349));
#39193=CARTESIAN_POINT('Ctrl Pts',(-0.203103859230808,0.00751546179966354,
0.0101981702831522));
#39194=CARTESIAN_POINT('Ctrl Pts',(-0.203056775223463,0.00789820782417455,
0.0101965072528155));
#39195=CARTESIAN_POINT('Ctrl Pts',(-0.203021238778556,0.00828462825544898,
0.0101712805771079));
#39196=CARTESIAN_POINT('Ctrl Pts',(-0.202934392060027,0.00973750097566171,
0.00998326665784201));
#39197=CARTESIAN_POINT('Ctrl Pts',(-0.20296540424907,0.0107807607669583,
0.00966106303167944));
#39198=CARTESIAN_POINT('Ctrl Pts',(-0.203118299904493,0.0119203561347129,
0.00907304555521591));
#39199=CARTESIAN_POINT('Ctrl Pts',(-0.203144199565202,0.0120881563723461,
0.00897978675739302));
#39200=CARTESIAN_POINT('Ctrl Pts',(-0.203173149226216,0.0122530889570464,
0.00888129613151275));
#39201=CARTESIAN_POINT('',(-0.204179780874563,0.012253032433249,0.00890317356958328));
#39202=CARTESIAN_POINT('Ctrl Pts',(-0.203173153192913,0.0122530883967066,
0.00888129655433334));
#39203=CARTESIAN_POINT('Ctrl Pts',(-0.203511932509764,0.0122530694823888,
0.00888865928521167));
#39204=CARTESIAN_POINT('Ctrl Pts',(-0.203847729433473,0.0122530549450459,
0.00889595466893973));
#39205=CARTESIAN_POINT('Ctrl Pts',(-0.204179836434326,0.0122530445711258,
0.00890316748087414));
#39206=CARTESIAN_POINT('',(-0.204098748533723,0.00749980191224963,0.0102197690721754));
#39207=CARTESIAN_POINT('Ctrl Pts',(-0.204179780874563,0.012253032433249,
0.00890317356958328));
#39208=CARTESIAN_POINT('Ctrl Pts',(-0.204143461050771,0.0120171892546894,
0.00904411661106718));
#39209=CARTESIAN_POINT('Ctrl Pts',(-0.204098317379387,0.0117026096193404,
0.00921193526686398));
#39210=CARTESIAN_POINT('Ctrl Pts',(-0.204053625025722,0.011345447823741,
0.00938026087496657));
#39211=CARTESIAN_POINT('Ctrl Pts',(-0.204033257590342,0.011169438898885,
0.00945875526541203));
#39212=CARTESIAN_POINT('Ctrl Pts',(-0.20400400644035,0.0108526182110254,
0.0095892955380159));
#39213=CARTESIAN_POINT('Ctrl Pts',(-0.203979232931866,0.010473412739609,
0.00972905581782053));
#39214=CARTESIAN_POINT('Ctrl Pts',(-0.203963398504837,0.00995938769060063,
0.00989005736630761));
#39215=CARTESIAN_POINT('Ctrl Pts',(-0.203968966224995,0.00948972602499641,
0.0100040791989076));
#39216=CARTESIAN_POINT('Ctrl Pts',(-0.203982474968269,0.00911908695810915,
0.0100751001999791));
#39217=CARTESIAN_POINT('Ctrl Pts',(-0.203992485231315,0.00891210336567303,
0.0101093719543023));
#39218=CARTESIAN_POINT('Ctrl Pts',(-0.204003028710727,0.00872797162306478,
0.0101359840652107));
#39219=CARTESIAN_POINT('Ctrl Pts',(-0.20400874394351,0.00863961277180208,
0.0101473278130879));
#39220=CARTESIAN_POINT('Ctrl Pts',(-0.204020424813096,0.00846714164179978,
0.0101680546246225));
#39221=CARTESIAN_POINT('Ctrl Pts',(-0.204044836153723,0.00813870113222504,
0.0102001979821628));
#39222=CARTESIAN_POINT('Ctrl Pts',(-0.204074808586391,0.00777469146557797,
0.0102192556370909));
#39223=CARTESIAN_POINT('Ctrl Pts',(-0.204098748532138,0.00749980199044204,
0.0102197690721427));
#39224=CARTESIAN_POINT('',(-0.204181203653622,0.00274295112565268,0.00890078565278145));
#39225=CARTESIAN_POINT('Ctrl Pts',(-0.204098748533723,0.00749980191224963,
0.0102197690721754));
#39226=CARTESIAN_POINT('Ctrl Pts',(-0.204074880929372,0.00722376251075426,
0.0102192452129123));
#39227=CARTESIAN_POINT('Ctrl Pts',(-0.204045011657587,0.0068582828311219,
0.0102000235115584));
#39228=CARTESIAN_POINT('Ctrl Pts',(-0.204020697069231,0.00652849968391289,
0.0101676045847285));
#39229=CARTESIAN_POINT('Ctrl Pts',(-0.204009076078799,0.00635546295071101,
0.0101467226518613));
#39230=CARTESIAN_POINT('Ctrl Pts',(-0.204003375631308,0.00626651305530474,
0.0101352488071801));
#39231=CARTESIAN_POINT('Ctrl Pts',(-0.20399294897216,0.00608271596521517,
0.0101085755847959));
#39232=CARTESIAN_POINT('Ctrl Pts',(-0.203983037889796,0.00587591892958034,
0.0100742185056347));
#39233=CARTESIAN_POINT('Ctrl Pts',(-0.203969676391244,0.0055058961751446,
0.0100031125965096));
#39234=CARTESIAN_POINT('Ctrl Pts',(-0.203964190242521,0.00503729302673557,
0.00988910976652827));
#39235=CARTESIAN_POINT('Ctrl Pts',(-0.203979910998399,0.00452522540899178,
0.00972857991125269));
#39236=CARTESIAN_POINT('Ctrl Pts',(-0.204004528322486,0.00414749332803605,
0.00958931999877319));
#39237=CARTESIAN_POINT('Ctrl Pts',(-0.204033478477464,0.00383291015267278,
0.00945976525310406));
#39238=CARTESIAN_POINT('Ctrl Pts',(-0.204053978965976,0.00365549874924138,
0.00938071761359606));
#39239=CARTESIAN_POINT('Ctrl Pts',(-0.204098931566298,0.00329690411269798,
0.00921173427308648));
#39240=CARTESIAN_POINT('Ctrl Pts',(-0.204144505573565,0.00298031101002354,
0.00904279652424585));
#39241=CARTESIAN_POINT('Ctrl Pts',(-0.204181203653622,0.00274295112565268,
0.00890078565278145));
#39242=CARTESIAN_POINT('Ctrl Pts',(-0.204181260022187,0.00274294282639214,
0.00890078188239789));
#39243=CARTESIAN_POINT('Ctrl Pts',(-0.203847886509956,0.00274281850013204,
0.00889347492067281));
#39244=CARTESIAN_POINT('Ctrl Pts',(-0.203514399366426,0.00274269020994476,
0.00888616310506232));
#39245=CARTESIAN_POINT('Ctrl Pts',(-0.203181006275248,0.00274255803686494,
0.00887885098901425));
#39246=CARTESIAN_POINT('Origin',(-0.205569658041737,0.00749999947180197,
0.00105479137718579));
#39247=CARTESIAN_POINT('',(-0.205098436723926,0.00749984710325509,0.0102432567628741));
#39248=CARTESIAN_POINT('',(-0.205181476923035,0.00274471358820867,0.00891990256930596));
#39249=CARTESIAN_POINT('Ctrl Pts',(-0.205181476923035,0.00274471358820867,
0.00891990256930596));
#39250=CARTESIAN_POINT('Ctrl Pts',(-0.205144999435084,0.00298046276772295,
0.0090615603243642));
#39251=CARTESIAN_POINT('Ctrl Pts',(-0.205099653927717,0.00329494512090687,
0.00923020959913407));
#39252=CARTESIAN_POINT('Ctrl Pts',(-0.205054727115499,0.00365205955154019,
0.00939936791908314));
#39253=CARTESIAN_POINT('Ctrl Pts',(-0.205034265565039,0.00382779147629106,
0.00947814183092217));
#39254=CARTESIAN_POINT('Ctrl Pts',(-0.20500474207185,0.00414512155714752,
0.0096095461180496));
#39255=CARTESIAN_POINT('Ctrl Pts',(-0.204979716812682,0.00452455957091514,
0.00975004056260158));
#39256=CARTESIAN_POINT('Ctrl Pts',(-0.204963626367347,0.00503777155002916,
0.00991158317344809));
#39257=CARTESIAN_POINT('Ctrl Pts',(-0.204969004327107,0.00550889290724541,
0.0100265106819687));
#39258=CARTESIAN_POINT('Ctrl Pts',(-0.20498237769071,0.00587963241517032,
0.010097851465535));
#39259=CARTESIAN_POINT('Ctrl Pts',(-0.204992318269195,0.00608664949133323,
0.0101322804306265));
#39260=CARTESIAN_POINT('Ctrl Pts',(-0.20500279780342,0.00627066364792692,
0.010158996492799));
#39261=CARTESIAN_POINT('Ctrl Pts',(-0.205008498650806,0.00635916355663372,
0.0101704121841367));
#39262=CARTESIAN_POINT('Ctrl Pts',(-0.205020149004397,0.00653174744369742,
0.010191247580515));
#39263=CARTESIAN_POINT('Ctrl Pts',(-0.205044527128556,0.00686045861570371,
0.0102235677823509));
#39264=CARTESIAN_POINT('Ctrl Pts',(-0.20507449102882,0.00722474579493575,
0.010242732314049));
#39265=CARTESIAN_POINT('Ctrl Pts',(-0.205098436838663,0.00749984638114644,
0.0102432567656874));
#39266=CARTESIAN_POINT('',(-0.205180383787346,0.0122514622743969,0.0089221865607949));
#39267=CARTESIAN_POINT('Ctrl Pts',(-0.205098436789953,0.0074998471090431,
0.0102432567646418));
#39268=CARTESIAN_POINT('Ctrl Pts',(-0.205074354603187,0.00777471924233373,
0.0102427384211593));
#39269=CARTESIAN_POINT('Ctrl Pts',(-0.205044224088182,0.00813868908844073,
0.0102236143681364));
#39270=CARTESIAN_POINT('Ctrl Pts',(-0.205019718722386,0.00846712890458327,
0.0101913547215864));
#39271=CARTESIAN_POINT('Ctrl Pts',(-0.205008014898611,0.00863952563124892,
0.010170565224802));
#39272=CARTESIAN_POINT('Ctrl Pts',(-0.205002283639176,0.00872803405528101,
0.0101591583475927));
#39273=CARTESIAN_POINT('Ctrl Pts',(-0.204991783191973,0.00891153024400615,
0.0101325492799381));
#39274=CARTESIAN_POINT('Ctrl Pts',(-0.204981823379621,0.00911820648575059,
0.0100982161433639));
#39275=CARTESIAN_POINT('Ctrl Pts',(-0.204968402235169,0.00948813798704052,
0.0100272030886554));
#39276=CARTESIAN_POINT('Ctrl Pts',(-0.204963285734911,0.00996204771265651,
0.0099113204303612));
#39277=CARTESIAN_POINT('Ctrl Pts',(-0.204978679135674,0.0104671708457599,
0.0097533572650039));
#39278=CARTESIAN_POINT('Ctrl Pts',(-0.205001872942925,0.0108105532641061,
0.00962546665935062));
#39279=CARTESIAN_POINT('Ctrl Pts',(-0.205017674322944,0.0109985928831329,
0.00955044853206125));
#39280=CARTESIAN_POINT('Ctrl Pts',(-0.205033320565654,0.0111580504126392,
0.00948319462115217));
#39281=CARTESIAN_POINT('Ctrl Pts',(-0.20504249987871,0.0112415438927982,
0.00944652284227898));
#39282=CARTESIAN_POINT('Ctrl Pts',(-0.205060574645265,0.0113979299630055,
0.00937617119624099));
#39283=CARTESIAN_POINT('Ctrl Pts',(-0.205098289295843,0.0116949803514041,
0.00923470790117257));
#39284=CARTESIAN_POINT('Ctrl Pts',(-0.205144065972417,0.012015827840092,
0.00906362218301645));
#39285=CARTESIAN_POINT('Ctrl Pts',(-0.205180383787346,0.0122514622743969,
0.0089221865607949));
#39286=CARTESIAN_POINT('',(-0.206180937657661,0.0122515141026534,0.00894388147634254));
#39287=CARTESIAN_POINT('Ctrl Pts',(-0.205180453611888,0.0122514588177548,
0.00892219016333599));
#39288=CARTESIAN_POINT('Ctrl Pts',(-0.205511148871274,0.0122514771336389,
0.00892935988179134));
#39289=CARTESIAN_POINT('Ctrl Pts',(-0.205844866014664,0.0122514995001858,
0.00893659277298742));
#39290=CARTESIAN_POINT('Ctrl Pts',(-0.206180987661044,0.0122515260700969,
0.00894387533870355));
#39291=CARTESIAN_POINT('',(-0.206098158559683,0.00749989366550756,0.0102649624274855));
#39292=CARTESIAN_POINT('Ctrl Pts',(-0.206180937657661,0.0122515141026534,
0.00894388147634254));
#39293=CARTESIAN_POINT('Ctrl Pts',(-0.206144660866419,0.0120160183041278,
0.009085236259632));
#39294=CARTESIAN_POINT('Ctrl Pts',(-0.206098899870945,0.01169524993866,
0.00925629857313019));
#39295=CARTESIAN_POINT('Ctrl Pts',(-0.206061132361365,0.0113980780373007,
0.00939782966776102));
#39296=CARTESIAN_POINT('Ctrl Pts',(-0.20604299822031,0.0112415087259796,
0.00946826283096089));
#39297=CARTESIAN_POINT('Ctrl Pts',(-0.206033784421152,0.0111579602868827,
0.00950495948634835));
#39298=CARTESIAN_POINT('Ctrl Pts',(-0.20601801307969,0.0109979583047259,
0.00957243326902137));
#39299=CARTESIAN_POINT('Ctrl Pts',(-0.206002083351523,0.0108095769841854,
0.00964756592446938));
#39300=CARTESIAN_POINT('Ctrl Pts',(-0.205978663196826,0.0104657148947248,
0.0097755526521527));
#39301=CARTESIAN_POINT('Ctrl Pts',(-0.205962991007194,0.00996284049211284,
0.00993280311124859));
#39302=CARTESIAN_POINT('Ctrl Pts',(-0.205967866525693,0.00948672058736224,
0.010049230644559));
#39303=CARTESIAN_POINT('Ctrl Pts',(-0.205981177868757,0.00911719678861053,
0.0101200908184433));
#39304=CARTESIAN_POINT('Ctrl Pts',(-0.205991090210523,0.00891083408445435,
0.0101543521708114));
#39305=CARTESIAN_POINT('Ctrl Pts',(-0.206001553448915,0.00872784553293601,
0.010180878134153));
#39306=CARTESIAN_POINT('Ctrl Pts',(-0.206007285858683,0.0086394365338037,
0.0101922726253234));
#39307=CARTESIAN_POINT('Ctrl Pts',(-0.206019006109483,0.00846724868623852,
0.0102130367903869));
#39308=CARTESIAN_POINT('Ctrl Pts',(-0.206043602684669,0.00813897561664646,
0.0102452907826911));
#39309=CARTESIAN_POINT('Ctrl Pts',(-0.206073911555016,0.00777492913360827,
0.0102644392378273));
#39310=CARTESIAN_POINT('Ctrl Pts',(-0.206098158559595,0.00749989366551524,
0.0102649624274836));
#39311=CARTESIAN_POINT('',(-0.206181705500482,0.00274489174553523,0.00894172441120622));
#39312=CARTESIAN_POINT('Ctrl Pts',(-0.206098158559683,0.00749989366550756,
0.0102649624274855));
#39313=CARTESIAN_POINT('Ctrl Pts',(-0.206073959098662,0.00722364355886157,
0.0102644337474957));
#39314=CARTESIAN_POINT('Ctrl Pts',(-0.206043716980217,0.00685803736171764,
0.0102451182414761));
#39315=CARTESIAN_POINT('Ctrl Pts',(-0.206019177562163,0.00652833493064124,
0.0102125773260753));
#39316=CARTESIAN_POINT('Ctrl Pts',(-0.206007493409607,0.00635553275105125,
0.0101916493844423));
#39317=CARTESIAN_POINT('Ctrl Pts',(-0.206001762741477,0.00626650822424718,
0.010180120236742));
#39318=CARTESIAN_POINT('Ctrl Pts',(-0.205991386078031,0.00608379417233497,
0.0101535194432339));
#39319=CARTESIAN_POINT('Ctrl Pts',(-0.20598153359865,0.00587762722169114,
0.0101191755144898));
#39320=CARTESIAN_POINT('Ctrl Pts',(-0.205968325976292,0.00550849646880288,
0.0100481105257598));
#39321=CARTESIAN_POINT('Ctrl Pts',(-0.205963195332645,0.00503604973694923,
0.00993274520514876));
#39322=CARTESIAN_POINT('Ctrl Pts',(-0.205979390899299,0.00452804773636262,
0.00977287900430854));
#39323=CARTESIAN_POINT('Ctrl Pts',(-0.20600443701926,0.00414976611457223,
0.00963305573502386));
#39324=CARTESIAN_POINT('Ctrl Pts',(-0.20603386541523,0.0038335282789123,
0.00950233649648007));
#39325=CARTESIAN_POINT('Ctrl Pts',(-0.206054458420243,0.00365634684123214,
0.0094230617805734));
#39326=CARTESIAN_POINT('Ctrl Pts',(-0.20609954285163,0.00329779903994257,
0.00925341710486629));
#39327=CARTESIAN_POINT('Ctrl Pts',(-0.206145078217534,0.00298174438244053,
0.00908403851963943));
#39328=CARTESIAN_POINT('Ctrl Pts',(-0.206181705500482,0.00274489174553523,
0.00894172441120622));
#39329=CARTESIAN_POINT('Ctrl Pts',(-0.206181756662732,0.00274488347523256,
0.00894172052487549));
#39330=CARTESIAN_POINT('Ctrl Pts',(-0.205849126200276,0.00274483042692363,
0.00893446732041925));
#39331=CARTESIAN_POINT('Ctrl Pts',(-0.205515617123526,0.00274477344911426,
0.00892719266697236));
#39332=CARTESIAN_POINT('Ctrl Pts',(-0.205181550495496,0.00274471254920856,
0.00891990353869956));
#39333=CARTESIAN_POINT('Origin',(-0.207569521557474,0.00749999958288434,
0.00113169766824726));
#39334=CARTESIAN_POINT('',(-0.20709777676797,0.00750000074588895,0.0102884318050736));
#39335=CARTESIAN_POINT('',(-0.207182008644929,0.00274682078388386,0.0089610216724757));
#39336=CARTESIAN_POINT('Ctrl Pts',(-0.207182008644929,0.00274682078388386,
0.0089610216724757));
#39337=CARTESIAN_POINT('Ctrl Pts',(-0.207145575477217,0.00298221862702531,
0.00910305394454891));
#39338=CARTESIAN_POINT('Ctrl Pts',(-0.207114932447028,0.00319598750884428,
0.00921768338570113));
#39339=CARTESIAN_POINT('Ctrl Pts',(-0.20709026641563,0.00338043799469262,
0.00930998443979783));
#39340=CARTESIAN_POINT('Ctrl Pts',(-0.207077933399932,0.00347266323761681,
0.00935613496684619));
#39341=CARTESIAN_POINT('Ctrl Pts',(-0.207067094216487,0.0035575471412094,
0.0093967226125637));
#39342=CARTESIAN_POINT('Ctrl Pts',(-0.207057405036147,0.0036379865399805,
0.00943389841659064));
#39343=CARTESIAN_POINT('Ctrl Pts',(-0.207052560445977,0.00367820623936605,
0.00945248631860411));
#39344=CARTESIAN_POINT('Ctrl Pts',(-0.20704800397913,0.00371732864609859,
0.00947019260412138));
#39345=CARTESIAN_POINT('Ctrl Pts',(-0.20704418523739,0.00375081558048865,
0.00948512581363911));
#39346=CARTESIAN_POINT('Ctrl Pts',(-0.20704036649565,0.00378430251487872,
0.00950005902315684));
#39347=CARTESIAN_POINT('Ctrl Pts',(-0.207037283499954,0.00381211261975297,
0.00951231025313473));
#39348=CARTESIAN_POINT('Ctrl Pts',(-0.207033092445885,0.00385268931337077,
0.00952982555512431));
#39349=CARTESIAN_POINT('Ctrl Pts',(-0.207028901391817,0.00389326600698857,
0.0095473408571139));
#39350=CARTESIAN_POINT('Ctrl Pts',(-0.20702360583578,0.00394668069240661,
0.00956995652994313));
#39351=CARTESIAN_POINT('Ctrl Pts',(-0.207018954045241,0.00399696732814934,
0.00959066061121586));
#39352=CARTESIAN_POINT('Ctrl Pts',(-0.207014302254701,0.00404725396389208,
0.0096113646924886));
#39353=CARTESIAN_POINT('Ctrl Pts',(-0.207010291748562,0.00409436609404158,
0.00963027138650139));
#39354=CARTESIAN_POINT('Ctrl Pts',(-0.207006494295823,0.00414215515037163,
0.00964901097839348));
#39355=CARTESIAN_POINT('Ctrl Pts',(-0.206998899390345,0.00423773326303174,
0.00968649016217763));
#39356=CARTESIAN_POINT('Ctrl Pts',(-0.206992159164313,0.00433605953714399,
0.00972318743619733));
#39357=CARTESIAN_POINT('Ctrl Pts',(-0.206986611713382,0.00443508121932275,
0.00975821336343698));
#39358=CARTESIAN_POINT('Ctrl Pts',(-0.20697551681152,0.00463312458368026,
0.00982826521791629));
#39359=CARTESIAN_POINT('Ctrl Pts',(-0.206969194341382,0.00483399433937503,
0.00989157040197803));
#39360=CARTESIAN_POINT('Ctrl Pts',(-0.20696699998225,0.00502987816024672,
0.00994635944260401));
#39361=CARTESIAN_POINT('Ctrl Pts',(-0.206964805623117,0.00522576198111841,
0.01000114848323));
#39362=CARTESIAN_POINT('Ctrl Pts',(-0.206966726835597,0.0054164844159352,
0.0100479985563706));
#39363=CARTESIAN_POINT('Ctrl Pts',(-0.206972408255633,0.00562088128514229,
0.0100909504821526));
#39364=CARTESIAN_POINT('Ctrl Pts',(-0.206975248965651,0.00572307971974584,
0.0101124264450436));
#39365=CARTESIAN_POINT('Ctrl Pts',(-0.206979033308164,0.00582873120607272,
0.0101327630618226));
#39366=CARTESIAN_POINT('Ctrl Pts',(-0.206983588792974,0.00593280052031057,
0.0101509283408082));
#39367=CARTESIAN_POINT('Ctrl Pts',(-0.206985866535379,0.0059848351774295,
0.010160010980301));
#39368=CARTESIAN_POINT('Ctrl Pts',(-0.206988336095,0.00603646618332007,
0.0101685953570537));
#39369=CARTESIAN_POINT('Ctrl Pts',(-0.206991307383632,0.00609278624748642,
0.0101774134158557));
#39370=CARTESIAN_POINT('Ctrl Pts',(-0.206994278672263,0.00614910631165276,
0.0101862314746577));
#39371=CARTESIAN_POINT('Ctrl Pts',(-0.206997755000619,0.00621013982597531,
0.0101951308300653));
#39372=CARTESIAN_POINT('Ctrl Pts',(-0.207000448457267,0.00625541611911697,
0.0102013968217338));
#39373=CARTESIAN_POINT('Ctrl Pts',(-0.207003141913915,0.00630069241225863,
0.0102076628134023));
#39374=CARTESIAN_POINT('Ctrl Pts',(-0.207005047888527,0.00633018297254175,
0.0102115076445645));
#39375=CARTESIAN_POINT('Ctrl Pts',(-0.207007462395225,0.00636646234232639,
0.0102160830445708));
#39376=CARTESIAN_POINT('Ctrl Pts',(-0.207009876901922,0.00640274171211104,
0.0102206584445771));
#39377=CARTESIAN_POINT('Ctrl Pts',(-0.207012802402609,0.00644582342611286,
0.0102258510976829));
#39378=CARTESIAN_POINT('Ctrl Pts',(-0.207015923228053,0.00649018925995671,
0.0102308383765914));
#39379=CARTESIAN_POINT('Ctrl Pts',(-0.207022164878943,0.00657892092764439,
0.0102408129344084));
#39380=CARTESIAN_POINT('Ctrl Pts',(-0.207029184722482,0.00667277538880603,
0.0102501089745481));
#39381=CARTESIAN_POINT('Ctrl Pts',(-0.20703723126043,0.00677582274945741,
0.0102584537446242));
#39382=CARTESIAN_POINT('Ctrl Pts',(-0.207053324334665,0.00698191744947961,
0.010275143283053));
#39383=CARTESIAN_POINT('Ctrl Pts',(-0.20707352685292,0.00722478486283655,
0.0102879049777361));
#39384=CARTESIAN_POINT('Ctrl Pts',(-0.207097776722938,0.00749999991179089,
0.0102884318038818));
#39385=CARTESIAN_POINT('',(-0.20718151084421,0.0122499348362438,0.00896297700837428));
#39386=CARTESIAN_POINT('Ctrl Pts',(-0.207097776664925,0.00750000073675634,
0.0102884318026212));
#39387=CARTESIAN_POINT('Ctrl Pts',(-0.207073415449424,0.00777501615170926,
0.0102879024570678));
#39388=CARTESIAN_POINT('Ctrl Pts',(-0.207042984455933,0.00813902360000427,
0.0102686867749524));
#39389=CARTESIAN_POINT('Ctrl Pts',(-0.207018325616829,0.00846728489363423,
0.0102363188518694));
#39390=CARTESIAN_POINT('Ctrl Pts',(-0.207006597174583,0.00863941228212482,
0.0102154905383654));
#39391=CARTESIAN_POINT('Ctrl Pts',(-0.207000859433949,0.00872792628559308,
0.0102040402212881));
#39392=CARTESIAN_POINT('Ctrl Pts',(-0.206990444167153,0.00891044623298851,
0.0101774926917494));
#39393=CARTESIAN_POINT('Ctrl Pts',(-0.206980584381931,0.00911656578521641,
0.0101431628687521));
#39394=CARTESIAN_POINT('Ctrl Pts',(-0.206967386735522,0.00948571707073339,
0.0100721765704815));
#39395=CARTESIAN_POINT('Ctrl Pts',(-0.20696272620052,0.00996376203546202,
0.00995482693936122));
#39396=CARTESIAN_POINT('Ctrl Pts',(-0.206978636730251,0.0104642557690517,
0.00979773389759007));
#39397=CARTESIAN_POINT('Ctrl Pts',(-0.207002273125407,0.0108084189656327,
0.00966921478300733));
#39398=CARTESIAN_POINT('Ctrl Pts',(-0.207018324368728,0.0109970008490617,
0.00959372828534347));
#39399=CARTESIAN_POINT('Ctrl Pts',(-0.207034226461458,0.0111575074984121,
0.00952578095182555));
#39400=CARTESIAN_POINT('Ctrl Pts',(-0.207043446318233,0.0112407737564283,
0.00948906068501107));
#39401=CARTESIAN_POINT('Ctrl Pts',(-0.207061625861014,0.0113972450779469,
0.00941839667616617));
#39402=CARTESIAN_POINT('Ctrl Pts',(-0.207099440341916,0.0116941168274847,
0.00927644448342378));
#39403=CARTESIAN_POINT('Ctrl Pts',(-0.207145227178358,0.0120146497717542,
0.00910481081580588));
#39404=CARTESIAN_POINT('Ctrl Pts',(-0.20718151084421,0.0122499348362438,
0.00896297700837428));
#39405=CARTESIAN_POINT('',(-0.208182029839437,0.0122499766833686,0.0089846914473168));
#39406=CARTESIAN_POINT('Ctrl Pts',(-0.207181573897133,0.0122499313680481,
0.00896298048072855));
#39407=CARTESIAN_POINT('Ctrl Pts',(-0.207511997686088,0.0122499464756022,
0.00897015094572272));
#39408=CARTESIAN_POINT('Ctrl Pts',(-0.207845716051498,0.0122499654803498,
0.0089773906346182));
#39409=CARTESIAN_POINT('Ctrl Pts',(-0.208182074796062,0.0122499885499931,
0.00898468523090216));
#39410=CARTESIAN_POINT('',(-0.208097511648441,0.0075000000097323,0.0103101525084975));
#39411=CARTESIAN_POINT('Ctrl Pts',(-0.208182029839437,0.0122499766833686,
0.0089846914473168));
#39412=CARTESIAN_POINT('Ctrl Pts',(-0.208145792855726,0.0120148330456536,
0.00912644211787466));
#39413=CARTESIAN_POINT('Ctrl Pts',(-0.208115282833245,0.0118012225403462,
0.00924089818765459));
#39414=CARTESIAN_POINT('Ctrl Pts',(-0.208090691592793,0.0116168440875562,
0.0093330878093222));
#39415=CARTESIAN_POINT('Ctrl Pts',(-0.208078395972566,0.0115246548611613,
0.00937918262015601));
#39416=CARTESIAN_POINT('Ctrl Pts',(-0.208067579614742,0.01143978576553,
0.00941973075151924));
#39417=CARTESIAN_POINT('Ctrl Pts',(-0.208057894473467,0.0113593052267618,
0.00945689384554209));
#39418=CARTESIAN_POINT('Ctrl Pts',(-0.208053051902829,0.0113190649573777,
0.00947547539255351));
#39419=CARTESIAN_POINT('Ctrl Pts',(-0.208048492764793,0.0112799078747642,
0.00949318175625101));
#39420=CARTESIAN_POINT('Ctrl Pts',(-0.208044672538954,0.0112464177413264,
0.00950810304976068));
#39421=CARTESIAN_POINT('Ctrl Pts',(-0.208040852313116,0.0112129276078887,
0.00952302434327035));
#39422=CARTESIAN_POINT('Ctrl Pts',(-0.208037768998231,0.011185146207607,
0.0095352526709192));
#39423=CARTESIAN_POINT('Ctrl Pts',(-0.208033554813732,0.0111444421187781,
0.0095528062343153));
#39424=CARTESIAN_POINT('Ctrl Pts',(-0.208029340629233,0.0111037380299492,
0.00957035979771141));
#39425=CARTESIAN_POINT('Ctrl Pts',(-0.208023999188475,0.0110500387683215,
0.00959307229688317));
#39426=CARTESIAN_POINT('Ctrl Pts',(-0.20801930739809,0.0109995533354734,
0.00961383345579642));
#39427=CARTESIAN_POINT('Ctrl Pts',(-0.208014615607705,0.0109490679026253,
0.00963459461470967));
#39428=CARTESIAN_POINT('Ctrl Pts',(-0.208010570935794,0.0109018436683241,
0.00965352096117992));
#39429=CARTESIAN_POINT('Ctrl Pts',(-0.208006738138096,0.0108539525564452,
0.00967227472359561));
#39430=CARTESIAN_POINT('Ctrl Pts',(-0.207999072542699,0.0107581703326874,
0.009709782248427));
#39431=CARTESIAN_POINT('Ctrl Pts',(-0.207992257022405,0.0106596778635927,
0.00974648077505833));
#39432=CARTESIAN_POINT('Ctrl Pts',(-0.20798663414025,0.0105608119821825,
0.00978139682654719));
#39433=CARTESIAN_POINT('Ctrl Pts',(-0.207975388375939,0.0103630802193621,
0.00985122892952491));
#39434=CARTESIAN_POINT('Ctrl Pts',(-0.207968912875204,0.0101638391044602,
0.00991394443523984));
#39435=CARTESIAN_POINT('Ctrl Pts',(-0.207966563520788,0.00996813660690527,
0.00996863187517243));
#39436=CARTESIAN_POINT('Ctrl Pts',(-0.207964214166371,0.00977243410935032,
0.010023319315105));
#39437=CARTESIAN_POINT('Ctrl Pts',(-0.207965981064406,0.00958041158679767,
0.0100704340503291));
#39438=CARTESIAN_POINT('Ctrl Pts',(-0.207971550318033,0.00937594739075353,
0.0101133221912404));
#39439=CARTESIAN_POINT('Ctrl Pts',(-0.207974334944846,0.00927371529273146,
0.0101347662616961));
#39440=CARTESIAN_POINT('Ctrl Pts',(-0.207978073340098,0.00916834167558793,
0.0101550073443192));
#39441=CARTESIAN_POINT('Ctrl Pts',(-0.207982591228724,0.00906458569967766,
0.0101730864752584));
#39442=CARTESIAN_POINT('Ctrl Pts',(-0.207984850173036,0.00901270771172253,
0.010182126040728));
#39443=CARTESIAN_POINT('Ctrl Pts',(-0.207987303053134,0.0089612420508267,
0.0101906682698402));
#39444=CARTESIAN_POINT('Ctrl Pts',(-0.207990257022641,0.00890517318126005,
0.0101994339730368));
#39445=CARTESIAN_POINT('Ctrl Pts',(-0.207993210992147,0.0088491043116934,
0.0102081996762335));
#39446=CARTESIAN_POINT('Ctrl Pts',(-0.207996669304785,0.00878840827953629,
0.0102170390987288));
#39447=CARTESIAN_POINT('Ctrl Pts',(-0.20799935633465,0.00874331456968449,
0.0102232734971157));
#39448=CARTESIAN_POINT('Ctrl Pts',(-0.208002043364514,0.0086982208598327,
0.0102295078955026));
#39449=CARTESIAN_POINT('Ctrl Pts',(-0.208003954567205,0.00866875755870705,
0.0102333464296309));
#39450=CARTESIAN_POINT('Ctrl Pts',(-0.208006377063033,0.00863253933496215,
0.0102379103435317));
#39451=CARTESIAN_POINT('Ctrl Pts',(-0.208008799558861,0.00859632111121726,
0.0102424742574324));
#39452=CARTESIAN_POINT('Ctrl Pts',(-0.208011735782999,0.00855333458415877,
0.010247651469918));
#39453=CARTESIAN_POINT('Ctrl Pts',(-0.208014872254183,0.00850905162177827,
0.0102526261647438));
#39454=CARTESIAN_POINT('Ctrl Pts',(-0.208021145196552,0.00842048569701728,
0.0102625755543955));
#39455=CARTESIAN_POINT('Ctrl Pts',(-0.208028216050051,0.00832674758329316,
0.0102718564983692));
#39456=CARTESIAN_POINT('Ctrl Pts',(-0.208036331741941,0.00822380066238706,
0.0102801905377563));
#39457=CARTESIAN_POINT('Ctrl Pts',(-0.208052563125722,0.00801790682057488,
0.0102968586165304));
#39458=CARTESIAN_POINT('Ctrl Pts',(-0.208072976460898,0.00777517677190799,
0.01030961950719));
#39459=CARTESIAN_POINT('Ctrl Pts',(-0.208097511648349,0.0075000000097405,
0.0103101525084955));
#39460=CARTESIAN_POINT('',(-0.208182216877932,0.00274693029866322,0.00898281703864054));
#39461=CARTESIAN_POINT('Ctrl Pts',(-0.208097511648441,0.0075000000097323,
0.0103101525084975));
#39462=CARTESIAN_POINT('Ctrl Pts',(-0.208072993965045,0.00722356118992073,
0.0103096197641003));
#39463=CARTESIAN_POINT('Ctrl Pts',(-0.208042400274024,0.00685784507416209,
0.0102902147042539));
#39464=CARTESIAN_POINT('Ctrl Pts',(-0.208017662771516,0.00652823631150515,
0.0102575584516077));
#39465=CARTESIAN_POINT('Ctrl Pts',(-0.208005930920095,0.00635564877914102,
0.0102365846017781));
#39466=CARTESIAN_POINT('Ctrl Pts',(-0.208000182777587,0.00626659133857995,
0.0102250079709892));
#39467=CARTESIAN_POINT('Ctrl Pts',(-0.207989865689244,0.00608477119043111,
0.0101984552495345));
#39468=CARTESIAN_POINT('Ctrl Pts',(-0.20798008310499,0.00587913141808675,
0.0101641066168629));
#39469=CARTESIAN_POINT('Ctrl Pts',(-0.20796704329005,0.00551077955137498,
0.0100930537471372));
#39470=CARTESIAN_POINT('Ctrl Pts',(-0.207962271325726,0.00503494827512439,
0.00997642711268012));
#39471=CARTESIAN_POINT('Ctrl Pts',(-0.207978920836864,0.00453114766412443,
0.00981730821500114));
#39472=CARTESIAN_POINT('Ctrl Pts',(-0.208004383855489,0.00415229827421602,
0.00967694145303679));
#39473=CARTESIAN_POINT('Ctrl Pts',(-0.208034293916788,0.00383415769731894,
0.00954496308351629));
#39474=CARTESIAN_POINT('Ctrl Pts',(-0.208054940986263,0.00365745017531619,
0.00946557676160163));
#39475=CARTESIAN_POINT('Ctrl Pts',(-0.208100143499718,0.00329896113401496,
0.00929530510330588));
#39476=CARTESIAN_POINT('Ctrl Pts',(-0.208145646094477,0.00298337772013156,
0.00912547875455556));
#39477=CARTESIAN_POINT('Ctrl Pts',(-0.208182216877932,0.00274693029866322,
0.00898281703864054));
#39478=CARTESIAN_POINT('Ctrl Pts',(-0.208182263102175,0.00274692209240819,
0.00898281306397055));
#39479=CARTESIAN_POINT('Ctrl Pts',(-0.207850589804928,0.00274689181898717,
0.00897558929414468));
#39480=CARTESIAN_POINT('Ctrl Pts',(-0.207517041324408,0.00274685772814941,
0.00896832247078491));
#39481=CARTESIAN_POINT('Ctrl Pts',(-0.207182075713153,0.00274681975932118,
0.00896102250785583));
#39482=CARTESIAN_POINT('Origin',(-0.209569669966458,0.0074999996646916,
0.00120787420876588));
#39483=CARTESIAN_POINT('',(-0.209097173739288,0.00750003250879847,0.0103336083052934));
#39484=CARTESIAN_POINT('',(-0.209182480741977,0.00274873233260506,0.00900211047042567));
#39485=CARTESIAN_POINT('Ctrl Pts',(-0.209182480741977,0.00274873233260506,
0.00900211047042567));
#39486=CARTESIAN_POINT('Ctrl Pts',(-0.209146100632164,0.00298377716177745,
0.0091445129836625));
#39487=CARTESIAN_POINT('Ctrl Pts',(-0.209115469242561,0.00319733244281788,
0.00925948736122651));
#39488=CARTESIAN_POINT('Ctrl Pts',(-0.209090780763169,0.00338164312408276,
0.00935207775087));
#39489=CARTESIAN_POINT('Ctrl Pts',(-0.209078436523473,0.00347379846471521,
0.00939837294569175));
#39490=CARTESIAN_POINT('Ctrl Pts',(-0.209067577573349,0.00355863035290946,
0.00943909229052956));
#39491=CARTESIAN_POINT('Ctrl Pts',(-0.209057852718374,0.00363908113506117,
0.00947641386394267));
#39492=CARTESIAN_POINT('Ctrl Pts',(-0.209052990290886,0.00367930652613703,
0.00949507465064922));
#39493=CARTESIAN_POINT('Ctrl Pts',(-0.209048412020849,0.00371845076690064,
0.00951285684655249));
#39494=CARTESIAN_POINT('Ctrl Pts',(-0.209044577592333,0.00375191008281231,
0.00952783315673602));
#39495=CARTESIAN_POINT('Ctrl Pts',(-0.209040743163818,0.00378536939872397,
0.00954280946691956));
#39496=CARTESIAN_POINT('Ctrl Pts',(-0.209037650558984,0.00381310148600916,
0.0095550727096917));
#39497=CARTESIAN_POINT('Ctrl Pts',(-0.209033414786212,0.00385381876556008,
0.00957271270229389));
#39498=CARTESIAN_POINT('Ctrl Pts',(-0.209029179013441,0.00389453604511099,
0.00959035269489609));
#39499=CARTESIAN_POINT('Ctrl Pts',(-0.20902380372181,0.00394831201896141,
0.00961320158436462));
#39500=CARTESIAN_POINT('Ctrl Pts',(-0.209019083848898,0.00399885026944767,
0.00963407810398663));
#39501=CARTESIAN_POINT('Ctrl Pts',(-0.209014363975986,0.00404938851993394,
0.00965495462360864));
#39502=CARTESIAN_POINT('Ctrl Pts',(-0.209010296961274,0.00409664094942468,
0.00967397655360619));
#39503=CARTESIAN_POINT('Ctrl Pts',(-0.20900644299565,0.00414455930228565,
0.00969282408903857));
#39504=CARTESIAN_POINT('Ctrl Pts',(-0.208998735064402,0.00424039600800758,
0.00973051915990333));
#39505=CARTESIAN_POINT('Ctrl Pts',(-0.20899188194532,0.00433893998899708,
0.00976739632961011));
#39506=CARTESIAN_POINT('Ctrl Pts',(-0.208986231409264,0.00443780727573967,
0.00980246391163614));
#39507=CARTESIAN_POINT('Ctrl Pts',(-0.208974930337152,0.00463554184922485,
0.00987259907568821));
#39508=CARTESIAN_POINT('Ctrl Pts',(-0.208968439083203,0.00483458168125401,
0.00993551952661447));
#39509=CARTESIAN_POINT('Ctrl Pts',(-0.208966086654309,0.00503022581632468,
0.00999043002591778));
#39510=CARTESIAN_POINT('Ctrl Pts',(-0.208963734225416,0.00522586995139535,
0.0100453405252211));
#39511=CARTESIAN_POINT('Ctrl Pts',(-0.208965510899781,0.0054179784984252,
0.010092688255882));
#39512=CARTESIAN_POINT('Ctrl Pts',(-0.208971085353274,0.00562259743052403,
0.0101357952616566));
#39513=CARTESIAN_POINT('Ctrl Pts',(-0.208973872580021,0.00572490689657345,
0.0101573487645439));
#39514=CARTESIAN_POINT('Ctrl Pts',(-0.208977612437784,0.00583037530970805,
0.0101776955278211));
#39515=CARTESIAN_POINT('Ctrl Pts',(-0.208982132048375,0.005934240640779,
0.0101958705541318));
#39516=CARTESIAN_POINT('Ctrl Pts',(-0.208984391853671,0.00598617330631448,
0.0102049580672871));
#39517=CARTESIAN_POINT('Ctrl Pts',(-0.20898684565277,0.00603769719115068,
0.010213546086111));
#39518=CARTESIAN_POINT('Ctrl Pts',(-0.208989800847266,0.00609384162467977,
0.0102223601272953));
#39519=CARTESIAN_POINT('Ctrl Pts',(-0.208992756041762,0.00614998605820886,
0.0102311741684797));
#39520=CARTESIAN_POINT('Ctrl Pts',(-0.208996215912591,0.00621077528232891,
0.0102400633187187));
#39521=CARTESIAN_POINT('Ctrl Pts',(-0.208998903301093,0.00625592035494135,
0.0102463300512141));
#39522=CARTESIAN_POINT('Ctrl Pts',(-0.209001590689595,0.00630106542755378,
0.0102525967837096));
#39523=CARTESIAN_POINT('Ctrl Pts',(-0.209003501015202,0.00633053794223429,
0.0102564517903237));
#39524=CARTESIAN_POINT('Ctrl Pts',(-0.209005923797116,0.00636677733471289,
0.0102610367039119));
#39525=CARTESIAN_POINT('Ctrl Pts',(-0.209008346579031,0.00640301672719149,
0.0102656216175002));
#39526=CARTESIAN_POINT('Ctrl Pts',(-0.209011284270186,0.00644603652114672,
0.0102708236109892));
#39527=CARTESIAN_POINT('Ctrl Pts',(-0.209014422806348,0.00649035160598153,
0.0102758217619476));
#39528=CARTESIAN_POINT('Ctrl Pts',(-0.209020699878673,0.00657898177565117,
0.0102858180638643));
#39529=CARTESIAN_POINT('Ctrl Pts',(-0.209027777232078,0.00667277941439591,
0.0102951415368914));
#39530=CARTESIAN_POINT('Ctrl Pts',(-0.209035902314636,0.00677579123680547,
0.0103035135477044));
#39531=CARTESIAN_POINT('Ctrl Pts',(-0.209052152478095,0.00698181486062926,
0.0103202575676242));
#39532=CARTESIAN_POINT('Ctrl Pts',(-0.209072596182764,0.00722469622862829,
0.0103330749790414));
#39533=CARTESIAN_POINT('Ctrl Pts',(-0.209097173739288,0.00750003250879847,
0.0103336083052934));
#39534=CARTESIAN_POINT('',(-0.209182595670359,0.0122484553035031,0.00900382443876613));
#39535=CARTESIAN_POINT('Ctrl Pts',(-0.209097173663308,0.00750003352365617,
0.0103336083036377));
#39536=CARTESIAN_POINT('Ctrl Pts',(-0.209072487387346,0.0077752027295915,
0.0103330705552668));
#39537=CARTESIAN_POINT('Ctrl Pts',(-0.20904170611148,0.00813926656432189,
0.0103137660496164));
#39538=CARTESIAN_POINT('Ctrl Pts',(-0.209016870020302,0.00846736255900025,
0.0102812931650683));
#39539=CARTESIAN_POINT('Ctrl Pts',(-0.209005112436531,0.00863924123692276,
0.0102604258946952));
#39540=CARTESIAN_POINT('Ctrl Pts',(-0.208999371395027,0.00872773998646285,
0.0102489367160665));
#39541=CARTESIAN_POINT('Ctrl Pts',(-0.208989042716632,0.00890940175348926,
0.0102224367002035));
#39542=CARTESIAN_POINT('Ctrl Pts',(-0.208979287054889,0.00911503344528391,
0.0101880995138537));
#39543=CARTESIAN_POINT('Ctrl Pts',(-0.20896632173186,0.00948348192094728,
0.0101171239430875));
#39544=CARTESIAN_POINT('Ctrl Pts',(-0.208962145860431,0.00996543922381415,
0.00999835162461839));
#39545=CARTESIAN_POINT('Ctrl Pts',(-0.208978582898474,0.0104611459243631,
0.00984221246132182));
#39546=CARTESIAN_POINT('Ctrl Pts',(-0.209002670041753,0.010806151365008,
0.00971305719239442));
#39547=CARTESIAN_POINT('Ctrl Pts',(-0.209018974214673,0.0109953313838264,
0.00963708637988462));
#39548=CARTESIAN_POINT('Ctrl Pts',(-0.209035136938378,0.0111569767219068,
0.00956840910744746));
#39549=CARTESIAN_POINT('Ctrl Pts',(-0.2090443919497,0.0112400061477328,
0.00953164701243018));
#39550=CARTESIAN_POINT('Ctrl Pts',(-0.2090626715537,0.0113965822320191,
0.00946066576998285));
#39551=CARTESIAN_POINT('Ctrl Pts',(-0.209100573807665,0.0116932888722541,
0.00931822603645342));
#39552=CARTESIAN_POINT('Ctrl Pts',(-0.209146357132706,0.0120135168800619,
0.00914604905715582));
#39553=CARTESIAN_POINT('Ctrl Pts',(-0.209182595670359,0.0122484553035031,
0.00900382443876613));
#39554=CARTESIAN_POINT('',(-0.210183354865266,0.0122485335158607,0.00902553609473393));
#39555=CARTESIAN_POINT('Ctrl Pts',(-0.209182651576042,0.0122484518533258,
0.00900382775451287));
#39556=CARTESIAN_POINT('Ctrl Pts',(-0.209514352353559,0.0122484795677455,
0.00901102297423394));
#39557=CARTESIAN_POINT('Ctrl Pts',(-0.209848095210384,0.0122485111023429,
0.00901826026877957));
#39558=CARTESIAN_POINT('Ctrl Pts',(-0.210183395177975,0.0122485465320611,
0.00902552904778905));
#39559=CARTESIAN_POINT('',(-0.21009684684534,0.00750005508728801,0.0103553421922863));
#39560=CARTESIAN_POINT('Ctrl Pts',(-0.210183354865266,0.0122485335158607,
0.00902553609473393));
#39561=CARTESIAN_POINT('Ctrl Pts',(-0.21014698672904,0.0120127163893144,
0.00916829590243412));
#39562=CARTESIAN_POINT('Ctrl Pts',(-0.210116347665497,0.0117983968347776,
0.00928354689096572));
#39563=CARTESIAN_POINT('Ctrl Pts',(-0.210091629427547,0.0116133305266073,
0.00937637517010963));
#39564=CARTESIAN_POINT('Ctrl Pts',(-0.210079270308572,0.0115207973725221,
0.00942278930968159));
#39565=CARTESIAN_POINT('Ctrl Pts',(-0.210068390961519,0.0114355897376177,
0.0094636177544873));
#39566=CARTESIAN_POINT('Ctrl Pts',(-0.210058641871792,0.0113547868889098,
0.00950103016538221));
#39567=CARTESIAN_POINT('Ctrl Pts',(-0.210053767326929,0.0113143854645558,
0.00951973637082966));
#39568=CARTESIAN_POINT('Ctrl Pts',(-0.210049175979292,0.0112750711533674,
0.00953755945900945));
#39569=CARTESIAN_POINT('Ctrl Pts',(-0.210045325081173,0.0112414204036042,
0.00955258917223236));
#39570=CARTESIAN_POINT('Ctrl Pts',(-0.210041474183053,0.0112077696538411,
0.00956761888545526));
#39571=CARTESIAN_POINT('Ctrl Pts',(-0.210038361718855,0.0111798246297253,
0.00957994792756669));
#39572=CARTESIAN_POINT('Ctrl Pts',(-0.210034112592833,0.0111389858803094,
0.0095975987918489));
#39573=CARTESIAN_POINT('Ctrl Pts',(-0.21002986346681,0.0110981471308936,
0.00961524965613112));
#39574=CARTESIAN_POINT('Ctrl Pts',(-0.210024481319256,0.0110443415114109,
0.00963805491322707));
#39575=CARTESIAN_POINT('Ctrl Pts',(-0.210019750328922,0.0109937885568437,
0.00965888559117742));
#39576=CARTESIAN_POINT('Ctrl Pts',(-0.210015019338587,0.0109432356022766,
0.00967971626912777));
#39577=CARTESIAN_POINT('Ctrl Pts',(-0.210010936953547,0.010895983133197,
0.00969868974003685));
#39578=CARTESIAN_POINT('Ctrl Pts',(-0.210007065948202,0.0108480896648573,
0.00971747917026967));
#39579=CARTESIAN_POINT('Ctrl Pts',(-0.209999323937511,0.010752302728178,
0.00975505803073532));
#39580=CARTESIAN_POINT('Ctrl Pts',(-0.20999243008157,0.0106539077570024,
0.00979177949000212));
#39581=CARTESIAN_POINT('Ctrl Pts',(-0.209986729913038,0.0105554038508432,
0.00982662910691118));
#39582=CARTESIAN_POINT('Ctrl Pts',(-0.209975329575974,0.0103583960385248,
0.00989632834072931));
#39583=CARTESIAN_POINT('Ctrl Pts',(-0.20996870266948,0.0101609552771156,
0.00995860087647994));
#39584=CARTESIAN_POINT('Ctrl Pts',(-0.209966181083884,0.0099663565756417,
0.0100131324078234));
#39585=CARTESIAN_POINT('Ctrl Pts',(-0.209963659498287,0.0097717578741678,
0.010067663939167));
#39586=CARTESIAN_POINT('Ctrl Pts',(-0.20996523499344,0.0095801214325255,
0.0101148334644337));
#39587=CARTESIAN_POINT('Ctrl Pts',(-0.209970581938221,0.00937693500919795,
0.0101576234975028));
#39588=CARTESIAN_POINT('Ctrl Pts',(-0.209973255410611,0.00927534179753417,
0.0101790185140374));
#39589=CARTESIAN_POINT('Ctrl Pts',(-0.209976874657855,0.00917083217192017,
0.0101991847003489));
#39590=CARTESIAN_POINT('Ctrl Pts',(-0.209981275808507,0.00906791018342924,
0.0102172183293223));
#39591=CARTESIAN_POINT('Ctrl Pts',(-0.209983476383833,0.00901644918918377,
0.010226235143809));
#39592=CARTESIAN_POINT('Ctrl Pts',(-0.209985871541067,0.00896539272474216,
0.0102347599358926));
#39593=CARTESIAN_POINT('Ctrl Pts',(-0.209988753927672,0.00890990792081734,
0.0102434932168294));
#39594=CARTESIAN_POINT('Ctrl Pts',(-0.209991636314278,0.00885442311689252,
0.0102522264977662));
#39595=CARTESIAN_POINT('Ctrl Pts',(-0.209995009051587,0.00879448684103273,
0.0102610247017059));
#39596=CARTESIAN_POINT('Ctrl Pts',(-0.209997655872122,0.00874962140646036,
0.0102672801053472));
#39597=CARTESIAN_POINT('Ctrl Pts',(-0.210000302692657,0.00870475597188798,
0.0102735355089885));
#39598=CARTESIAN_POINT('Ctrl Pts',(-0.210002219201085,0.00867498878986495,
0.0102774502766726));
#39599=CARTESIAN_POINT('Ctrl Pts',(-0.210004644701109,0.00863857556372592,
0.0102820788410741));
#39600=CARTESIAN_POINT('Ctrl Pts',(-0.210007070201132,0.0086021623375869,
0.0102867074054757));
#39601=CARTESIAN_POINT('Ctrl Pts',(-0.210010007073723,0.00855908986493375,
0.0102919402530651));
#39602=CARTESIAN_POINT('Ctrl Pts',(-0.210013153594257,0.00851467298255937,
0.010296974800606));
#39603=CARTESIAN_POINT('Ctrl Pts',(-0.210019446635327,0.00842583921781061,
0.0103070438956879));
#39604=CARTESIAN_POINT('Ctrl Pts',(-0.210026575247729,0.00833164123919009,
0.0103164587172962));
#39605=CARTESIAN_POINT('Ctrl Pts',(-0.210034778165727,0.00822815474954129,
0.0103249153303143));
#39606=CARTESIAN_POINT('Ctrl Pts',(-0.210051184001722,0.00802118177024369,
0.0103418285563504));
#39607=CARTESIAN_POINT('Ctrl Pts',(-0.210071889472725,0.00777705421800207,
0.0103547979768471));
#39608=CARTESIAN_POINT('Ctrl Pts',(-0.210096846845341,0.00750005508730573,
0.0103553421922863));
#39609=CARTESIAN_POINT('',(-0.210182935446423,0.00274902832065848,0.0090240398964221));
#39610=CARTESIAN_POINT('Ctrl Pts',(-0.21009684684534,0.00750005508728801,
0.0103553421922863));
#39611=CARTESIAN_POINT('Ctrl Pts',(-0.210072031529707,0.00722345799301737,
0.0103548042976559));
#39612=CARTESIAN_POINT('Ctrl Pts',(-0.210051420859798,0.00697958369651794,
0.0103418734782538));
#39613=CARTESIAN_POINT('Ctrl Pts',(-0.210035067604621,0.00677277347393194,
0.0103249955737702));
#39614=CARTESIAN_POINT('Ctrl Pts',(-0.210026890977033,0.00666936836263893,
0.0103165566215284));
#39615=CARTESIAN_POINT('Ctrl Pts',(-0.210019778074828,0.00657522908219787,
0.0103071597973542));
#39616=CARTESIAN_POINT('Ctrl Pts',(-0.210013486125652,0.00648637336607246,
0.0102970986183953));
#39617=CARTESIAN_POINT('Ctrl Pts',(-0.210010340151064,0.00644194550800976,
0.0102920680289159));
#39618=CARTESIAN_POINT('Ctrl Pts',(-0.210007400180234,0.00639884193886295,
0.0102868361402636));
#39619=CARTESIAN_POINT('Ctrl Pts',(-0.210004973587317,0.00636245780845583,
0.0102822154131323));
#39620=CARTESIAN_POINT('Ctrl Pts',(-0.2100025469944,0.00632607367804871,
0.010277594686001));
#39621=CARTESIAN_POINT('Ctrl Pts',(-0.210000631361163,0.00629639559480933,
0.0102736963514528));
#39622=CARTESIAN_POINT('Ctrl Pts',(-0.209997964377369,0.00625135134602337,
0.0102674207308797));
#39623=CARTESIAN_POINT('Ctrl Pts',(-0.209995297393576,0.00620630709723741,
0.0102611451103067));
#39624=CARTESIAN_POINT('Ctrl Pts',(-0.209991883546243,0.00614592463301405,
0.0102522858149151));
#39625=CARTESIAN_POINT('Ctrl Pts',(-0.209988966602404,0.00609008632608619,
0.0102434964886858));
#39626=CARTESIAN_POINT('Ctrl Pts',(-0.209986049658564,0.00603424801915834,
0.0102347071624564));
#39627=CARTESIAN_POINT('Ctrl Pts',(-0.209983626420324,0.00598293016518101,
0.0102261348990641));
#39628=CARTESIAN_POINT('Ctrl Pts',(-0.209981397477455,0.00593121358005969,
0.010217067716942));
#39629=CARTESIAN_POINT('Ctrl Pts',(-0.209976939591716,0.00582778040981704,
0.0101989333526979));
#39630=CARTESIAN_POINT('Ctrl Pts',(-0.209973262537477,0.00572278351867268,
0.0101786514229577));
#39631=CARTESIAN_POINT('Ctrl Pts',(-0.209970535541532,0.00562077092014045,
0.0101571397893884));
#39632=CARTESIAN_POINT('Ctrl Pts',(-0.209965081549642,0.00541674572307599,
0.0101141165222497));
#39633=CARTESIAN_POINT('Ctrl Pts',(-0.209963416125406,0.00522454125933521,
0.0100667110234108));
#39634=CARTESIAN_POINT('Ctrl Pts',(-0.209965850832377,0.00502978892616377,
0.0100120423326667));
#39635=CARTESIAN_POINT('Ctrl Pts',(-0.209968285539348,0.00483503659299233,
0.00995737364192262));
#39636=CARTESIAN_POINT('Ctrl Pts',(-0.209974828395779,0.00463785411534847,
0.00989507293553626));
#39637=CARTESIAN_POINT('Ctrl Pts',(-0.209986151081867,0.00444115623501538,
0.00982539340942192));
#39638=CARTESIAN_POINT('Ctrl Pts',(-0.209991812424911,0.00434280729484884,
0.00979055364636475));
#39639=CARTESIAN_POINT('Ctrl Pts',(-0.209998669097466,0.00424458096669036,
0.00975385206320209));
#39640=CARTESIAN_POINT('Ctrl Pts',(-0.210006377134424,0.00414898659058324,
0.0097163102825907));
#39641=CARTESIAN_POINT('Ctrl Pts',(-0.210010231152903,0.00410118940252968,
0.009697539392285));
#39642=CARTESIAN_POINT('Ctrl Pts',(-0.210014297357555,0.00405403923554369,
0.00967858857821047));
#39643=CARTESIAN_POINT('Ctrl Pts',(-0.210019009898115,0.00400361901395296,
0.00965779428064045));
#39644=CARTESIAN_POINT('Ctrl Pts',(-0.210023722438676,0.00395319879236224,
0.00963699998307044));
#39645=CARTESIAN_POINT('Ctrl Pts',(-0.210029083843341,0.00389955594149032,
0.00961424590868889));
#39646=CARTESIAN_POINT('Ctrl Pts',(-0.210033322718555,0.00385880004226566,
0.00959661798140514));
#39647=CARTESIAN_POINT('Ctrl Pts',(-0.210037561593769,0.003818044143041,
0.00957899005412139));
#39648=CARTESIAN_POINT('Ctrl Pts',(-0.210040674328065,0.00379010257233756,
0.00956665439685066));
#39649=CARTESIAN_POINT('Ctrl Pts',(-0.21004452606445,0.00375646787301374,
0.00955162163910428));
#39650=CARTESIAN_POINT('Ctrl Pts',(-0.210048377800834,0.00372283317368993,
0.00953658888135791));
#39651=CARTESIAN_POINT('Ctrl Pts',(-0.210052970542858,0.00368354728906639,
0.00951876686204021));
#39652=CARTESIAN_POINT('Ctrl Pts',(-0.210057849482595,0.00364316443446752,
0.00950005720653822));
#39653=CARTESIAN_POINT('Ctrl Pts',(-0.210067607362068,0.00356239872526979,
0.00946263789553426));
#39654=CARTESIAN_POINT('Ctrl Pts',(-0.210078507512784,0.00347718902812302,
0.009421783939139));
#39655=CARTESIAN_POINT('Ctrl Pts',(-0.210090897724529,0.0033846321571345,
0.00937532941205294));
#39656=CARTESIAN_POINT('Ctrl Pts',(-0.210115678148019,0.00319951841515747,
0.00928242035788084));
#39657=CARTESIAN_POINT('Ctrl Pts',(-0.210146420514204,0.00298506387705781,
0.00916703088647436));
#39658=CARTESIAN_POINT('Ctrl Pts',(-0.210182935446423,0.00274902832065848,
0.0090240398964221));
#39659=CARTESIAN_POINT('Ctrl Pts',(-0.210182976903937,0.00274902032469847,
0.00902403592680517));
#39660=CARTESIAN_POINT('Ctrl Pts',(-0.20984954026572,0.00274892753071286,
0.00901673074474417));
#39661=CARTESIAN_POINT('Ctrl Pts',(-0.209515992344277,0.00274883116012269,
0.00900942096250049));
#39662=CARTESIAN_POINT('Ctrl Pts',(-0.209182541425264,0.00274873127424957,
0.00900211114486483));
#39663=CARTESIAN_POINT('Origin',(-0.193569723895743,0.00749999928673165,
0.000576601746083541));
#39664=CARTESIAN_POINT('',(-0.193103855785931,0.00749669634329043,0.00997223704509611));
#39665=CARTESIAN_POINT('',(-0.193177238560899,0.00273223379907955,0.00867522024057621));
#39666=CARTESIAN_POINT('Ctrl Pts',(-0.193177238560899,0.00273223379907955,
0.00867522024057621));
#39667=CARTESIAN_POINT('Ctrl Pts',(-0.193141338548451,0.00296984836335153,
0.00881424998266486));
#39668=CARTESIAN_POINT('Ctrl Pts',(-0.193096834920356,0.00328633988174973,
0.00897964130725951));
#39669=CARTESIAN_POINT('Ctrl Pts',(-0.193053183912405,0.00364435066138988,
0.00914510567071404));
#39670=CARTESIAN_POINT('Ctrl Pts',(-0.193033364102516,0.00382132177014467,
0.00922249602324718));
#39671=CARTESIAN_POINT('Ctrl Pts',(-0.193005741650242,0.00413502514833468,
0.00934940056504819));
#39672=CARTESIAN_POINT('Ctrl Pts',(-0.192982517471961,0.00451365419336154,
0.00948680984862821));
#39673=CARTESIAN_POINT('Ctrl Pts',(-0.192968455245345,0.00503817115554176,
0.00964815811736775));
#39674=CARTESIAN_POINT('Ctrl Pts',(-0.192975186509652,0.00549854166420586,
0.00975802728443494));
#39675=CARTESIAN_POINT('Ctrl Pts',(-0.19298920675885,0.00587143281971192,
0.00982864698119864));
#39676=CARTESIAN_POINT('Ctrl Pts',(-0.192999409086713,0.0060799974385049,
0.00986272641220591));
#39677=CARTESIAN_POINT('Ctrl Pts',(-0.193010093679397,0.00626674437952322,
0.00988934301760898));
#39678=CARTESIAN_POINT('Ctrl Pts',(-0.193015756303844,0.00635510160385565,
0.00990051431842612));
#39679=CARTESIAN_POINT('Ctrl Pts',(-0.193027331983661,0.00652836366928688,
0.00992104290850712));
#39680=CARTESIAN_POINT('Ctrl Pts',(-0.193051322868053,0.00685751684410879,
0.00995279515838206));
#39681=CARTESIAN_POINT('Ctrl Pts',(-0.193080570759728,0.00722182594281122,
0.00997163711061381));
#39682=CARTESIAN_POINT('Ctrl Pts',(-0.193103856303716,0.00749669585242133,
0.0099722370582992));
#39683=CARTESIAN_POINT('',(-0.193178778898313,0.0122641846768735,0.00867735780753799));
#39684=CARTESIAN_POINT('Ctrl Pts',(-0.193103856259104,0.00749669638308835,
0.00997223705752114));
#39685=CARTESIAN_POINT('Ctrl Pts',(-0.193080779856104,0.00777118576984942,
0.00997183458338455));
#39686=CARTESIAN_POINT('Ctrl Pts',(-0.193051800859628,0.00813509755822241,
0.0099533036309153));
#39687=CARTESIAN_POINT('Ctrl Pts',(-0.193028037317639,0.00846412037883092,
0.00992183479932284));
#39688=CARTESIAN_POINT('Ctrl Pts',(-0.193016578366468,0.00863735206193072,
0.00990145478660238));
#39689=CARTESIAN_POINT('Ctrl Pts',(-0.193010965599083,0.00872584131090312,
0.0098903385279732));
#39690=CARTESIAN_POINT('Ctrl Pts',(-0.193000420585326,0.00891232900027939,
0.00986391558070171));
#39691=CARTESIAN_POINT('Ctrl Pts',(-0.192990369106261,0.00912085072542072,
0.00983002353592887));
#39692=CARTESIAN_POINT('Ctrl Pts',(-0.192976617902903,0.00949374270917578,
0.00975975040781575));
#39693=CARTESIAN_POINT('Ctrl Pts',(-0.19297025631144,0.00995631925037694,
0.00964969128851549));
#39694=CARTESIAN_POINT('Ctrl Pts',(-0.192984612054924,0.010479251557637,
0.00948921247306322));
#39695=CARTESIAN_POINT('Ctrl Pts',(-0.193007926010543,0.0108584095631401,
0.00935197207317474));
#39696=CARTESIAN_POINT('Ctrl Pts',(-0.193035575544608,0.0111730562205009,
0.00922493533851728));
#39697=CARTESIAN_POINT('Ctrl Pts',(-0.193055315395668,0.0113502096335574,
0.00914759534273209));
#39698=CARTESIAN_POINT('Ctrl Pts',(-0.193098792555964,0.0117089358444973,
0.00898206393295022));
#39699=CARTESIAN_POINT('Ctrl Pts',(-0.193143069638179,0.0120260667690436,
0.00881654618530351));
#39700=CARTESIAN_POINT('Ctrl Pts',(-0.193178778898313,0.0122641846768735,
0.00867735780753799));
#39701=CARTESIAN_POINT('',(-0.194178078842629,0.0122641623067804,0.00869897679015584));
#39702=CARTESIAN_POINT('Ctrl Pts',(-0.193178864680093,0.0122641819069075,
0.00867736129034749));
#39703=CARTESIAN_POINT('Ctrl Pts',(-0.193463836609973,0.0122641761777926,
0.00868352602731349));
#39704=CARTESIAN_POINT('Ctrl Pts',(-0.193745328838661,0.0122641740469773,
0.0086896134147566));
#39705=CARTESIAN_POINT('Ctrl Pts',(-0.194074393693453,0.0122641754661562,
0.00869672728191949));
#39706=CARTESIAN_POINT('Ctrl Pts',(-0.194126196785175,0.0122641758053938,
0.00869784711561093));
#39707=CARTESIAN_POINT('Ctrl Pts',(-0.194178146257402,0.0122641762630964,
0.00869897004455999));
#39708=CARTESIAN_POINT('',(-0.194103293745545,0.00749642396384868,0.00999384323056315));
#39709=CARTESIAN_POINT('Ctrl Pts',(-0.194178078842629,0.0122641623067804,
0.00869897679015584));
#39710=CARTESIAN_POINT('Ctrl Pts',(-0.194141973426115,0.0120248709868358,
0.00883884524871636));
#39711=CARTESIAN_POINT('Ctrl Pts',(-0.194097233107932,0.0117060242318462,
0.00900513658754215));
#39712=CARTESIAN_POINT('Ctrl Pts',(-0.194053464891725,0.011345942522752,
0.00917111002034425));
#39713=CARTESIAN_POINT('Ctrl Pts',(-0.194033531058898,0.0111668482859879,
0.0092491326416897));
#39714=CARTESIAN_POINT('Ctrl Pts',(-0.19400626338759,0.0108549923204777,
0.00937482374371128));
#39715=CARTESIAN_POINT('Ctrl Pts',(-0.193983223778424,0.0104774717474761,
0.0095113892130402));
#39716=CARTESIAN_POINT('Ctrl Pts',(-0.193969272664656,0.00995468087707124,
0.00967167132788243));
#39717=CARTESIAN_POINT('Ctrl Pts',(-0.193975843094312,0.00949639281041089,
0.00978072143137081));
#39718=CARTESIAN_POINT('Ctrl Pts',(-0.193989589072645,0.00912520255875588,
0.00985085735588398));
#39719=CARTESIAN_POINT('Ctrl Pts',(-0.193999610986714,0.00891747787109268,
0.00988472745515668));
#39720=CARTESIAN_POINT('Ctrl Pts',(-0.194010085577249,0.00873187890670615,
0.00991114102178041));
#39721=CARTESIAN_POINT('Ctrl Pts',(-0.194015720554619,0.00864278840341037,
0.0099223937624794));
#39722=CARTESIAN_POINT('Ctrl Pts',(-0.1940271920793,0.00846906395058688,
0.0099429287560856));
#39723=CARTESIAN_POINT('Ctrl Pts',(-0.194051023711656,0.00813851336097762,
0.00997471124740048));
#39724=CARTESIAN_POINT('Ctrl Pts',(-0.194080113956685,0.00777260055205324,
0.00999344724325746));
#39725=CARTESIAN_POINT('Ctrl Pts',(-0.194103293745545,0.00749642396384868,
0.00999384323056315));
#39726=CARTESIAN_POINT('',(-0.194177625723629,0.0027323178355601,0.00869689395108569));
#39727=CARTESIAN_POINT('Ctrl Pts',(-0.194103293744492,0.00749642367320619,
0.00999384323042973));
#39728=CARTESIAN_POINT('Ctrl Pts',(-0.194079985850101,0.00722088152225355,
0.00999323445983037));
#39729=CARTESIAN_POINT('Ctrl Pts',(-0.194050722774099,0.0068557531252023,
0.00997429687100921));
#39730=CARTESIAN_POINT('Ctrl Pts',(-0.194026735405087,0.00652587479550234,
0.00994239080627125));
#39731=CARTESIAN_POINT('Ctrl Pts',(-0.194015177153977,0.00635238376057256,
0.00992178766320044));
#39732=CARTESIAN_POINT('Ctrl Pts',(-0.194009508832243,0.00626361512406841,
0.00991053211974325));
#39733=CARTESIAN_POINT('Ctrl Pts',(-0.193998907820037,0.00607757541380027,
0.00988395901128883));
#39734=CARTESIAN_POINT('Ctrl Pts',(-0.193988775979243,0.00586949907587681,
0.00984990969528716));
#39735=CARTESIAN_POINT('Ctrl Pts',(-0.193974870892261,0.00549767136340122,
0.00977943757151345));
#39736=CARTESIAN_POINT('Ctrl Pts',(-0.193968261065726,0.0050373352232251,
0.0096694859417466));
#39737=CARTESIAN_POINT('Ctrl Pts',(-0.193982282452568,0.00451653356420576,
0.00950934180685302));
#39738=CARTESIAN_POINT('Ctrl Pts',(-0.194005392087704,0.00413945225215935,
0.009372680210967));
#39739=CARTESIAN_POINT('Ctrl Pts',(-0.194032753971147,0.00382781295525132,
0.00924684759490062));
#39740=CARTESIAN_POINT('Ctrl Pts',(-0.194052709819781,0.00364922188115017,
0.00916891841726741));
#39741=CARTESIAN_POINT('Ctrl Pts',(-0.194096578993025,0.00328971244232934,
0.0090029756844143));
#39742=CARTESIAN_POINT('Ctrl Pts',(-0.194141428072699,0.00297131658783776,
0.00883672851200297));
#39743=CARTESIAN_POINT('Ctrl Pts',(-0.194177625723629,0.0027323178355601,
0.00869689395108569));
#39744=CARTESIAN_POINT('Ctrl Pts',(-0.194177692817492,0.00273230882489036,
0.00869689009986668));
#39745=CARTESIAN_POINT('Ctrl Pts',(-0.193847122383193,0.00273228814490392,
0.00868973235595818));
#39746=CARTESIAN_POINT('Ctrl Pts',(-0.193513460240482,0.00273226267284877,
0.00868250496244904));
#39747=CARTESIAN_POINT('Ctrl Pts',(-0.193177329099023,0.00273223222473439,
0.00867522127133823));
#39748=CARTESIAN_POINT('Origin',(-0.213570493936196,0.00749999991453831,
0.00135810061113277));
#39749=CARTESIAN_POINT('',(-0.213095879900848,0.00749981038892108,0.0104239596070259));
#39750=CARTESIAN_POINT('',(-0.213184217082503,0.00275309087589512,0.00908489825530902));
#39751=CARTESIAN_POINT('Ctrl Pts',(-0.213184217082503,0.00275309087589512,
0.00908489825530902));
#39752=CARTESIAN_POINT('Ctrl Pts',(-0.213147946013642,0.00298738821182737,
0.00922795940497672));
#39753=CARTESIAN_POINT('Ctrl Pts',(-0.213102043822126,0.00330706237473753,
0.00940128400476012));
#39754=CARTESIAN_POINT('Ctrl Pts',(-0.213063912983746,0.00360352093124194,
0.00954476365425644));
#39755=CARTESIAN_POINT('Ctrl Pts',(-0.213045438975613,0.00376028588544419,
0.00961638748972627));
#39756=CARTESIAN_POINT('Ctrl Pts',(-0.21303611057467,0.00384298953821337,
0.00965330164747907));
#39757=CARTESIAN_POINT('Ctrl Pts',(-0.213019519962499,0.00400641619864203,
0.0097232562400473));
#39758=CARTESIAN_POINT('Ctrl Pts',(-0.213002812612574,0.00419655873439527,
0.00980013519929093));
#39759=CARTESIAN_POINT('Ctrl Pts',(-0.212978040034831,0.00454275981693908,
0.00993049491628299));
#39760=CARTESIAN_POINT('Ctrl Pts',(-0.212960945692762,0.00503202112932064,
0.0100856322688812));
#39761=CARTESIAN_POINT('Ctrl Pts',(-0.212964569057503,0.00551635865886951,
0.0102060183120711));
#39762=CARTESIAN_POINT('Ctrl Pts',(-0.212977236919282,0.00588477353496685,
0.0102774366800835));
#39763=CARTESIAN_POINT('Ctrl Pts',(-0.212986849121923,0.00609047891122502,
0.0103120226917365));
#39764=CARTESIAN_POINT('Ctrl Pts',(-0.212997070713013,0.00627230341138433,
0.0103387200016791));
#39765=CARTESIAN_POINT('Ctrl Pts',(-0.213002759777912,0.00636041695190613,
0.0103502342952264));
#39766=CARTESIAN_POINT('Ctrl Pts',(-0.213014513644883,0.0065320872202858,
0.0103712237365575));
#39767=CARTESIAN_POINT('Ctrl Pts',(-0.213039521035394,0.00685995861526675,
0.0104039161017014));
#39768=CARTESIAN_POINT('Ctrl Pts',(-0.213070754183437,0.00722428790289929,
0.0104234068834067));
#39769=CARTESIAN_POINT('Ctrl Pts',(-0.213095879900848,0.00749981038892108,
0.0104239596070259));
#39770=CARTESIAN_POINT('',(-0.213185690986499,0.0122460699114039,0.00908544519816533));
#39771=CARTESIAN_POINT('Ctrl Pts',(-0.213095879800977,0.00749981164463391,
0.0104239596048778));
#39772=CARTESIAN_POINT('Ctrl Pts',(-0.21307066098287,0.00777532698194311,
0.0104234163142761));
#39773=CARTESIAN_POINT('Ctrl Pts',(-0.213039345087209,0.00813961477500167,
0.0104039423501419));
#39774=CARTESIAN_POINT('Ctrl Pts',(-0.213014332410071,0.00846746144496389,
0.0103712668864278));
#39775=CARTESIAN_POINT('Ctrl Pts',(-0.213002611006837,0.00863903521304472,
0.0103503010215217));
#39776=CARTESIAN_POINT('Ctrl Pts',(-0.212996938122665,0.00872728047684472,
0.0103387717522634));
#39777=CARTESIAN_POINT('Ctrl Pts',(-0.212986830556453,0.00890843702918285,
0.0103121890710692));
#39778=CARTESIAN_POINT('Ctrl Pts',(-0.212977345913122,0.00911377178123675,
0.0102776975483701));
#39779=CARTESIAN_POINT('Ctrl Pts',(-0.212964930987284,0.00948166907831092,
0.0102064767184181));
#39780=CARTESIAN_POINT('Ctrl Pts',(-0.212961762283236,0.00996812097797597,
0.0100856145356055));
#39781=CARTESIAN_POINT('Ctrl Pts',(-0.212979243563552,0.010455543907438,
0.00993109274363753));
#39782=CARTESIAN_POINT('Ctrl Pts',(-0.213004227851109,0.0108020944666052,
0.00980069536728062));
#39783=CARTESIAN_POINT('Ctrl Pts',(-0.213021034374403,0.010992458373273,
0.00972376062269633));
#39784=CARTESIAN_POINT('Ctrl Pts',(-0.213037712034966,0.0111563039303219,
0.00965364877306718));
#39785=CARTESIAN_POINT('Ctrl Pts',(-0.213047042089263,0.0112389114824525,
0.00961678452581526));
#39786=CARTESIAN_POINT('Ctrl Pts',(-0.213065532800899,0.011395719129502,
0.00954516055025792));
#39787=CARTESIAN_POINT('Ctrl Pts',(-0.213103648549054,0.011692151249117,
0.00940172652220947));
#39788=CARTESIAN_POINT('Ctrl Pts',(-0.213149487437096,0.0120118029750531,
0.00922845413600301));
#39789=CARTESIAN_POINT('Ctrl Pts',(-0.213185690986499,0.0122460699114039,
0.00908544519816533));
#39790=CARTESIAN_POINT('',(-0.21418640254952,0.0122466617247526,0.00910686742116922));
#39791=CARTESIAN_POINT('Ctrl Pts',(-0.2131857349772,0.0122460667524225,
0.00908544809488056));
#39792=CARTESIAN_POINT('Ctrl Pts',(-0.213519274711084,0.0122462654086515,
0.00909258732591442));
#39793=CARTESIAN_POINT('Ctrl Pts',(-0.213852910436955,0.0122464675875923,
0.00909972647388659));
#39794=CARTESIAN_POINT('Ctrl Pts',(-0.214186433624517,0.0122466731629066,
0.00910686107552119));
#39795=CARTESIAN_POINT('',(-0.214095609529152,0.00749962227619371,0.0104457232276635));
#39796=CARTESIAN_POINT('Ctrl Pts',(-0.21418640254952,0.0122466617247526,
0.00910686742116922));
#39797=CARTESIAN_POINT('Ctrl Pts',(-0.214150242333865,0.0120125218227116,
0.00924982396327141));
#39798=CARTESIAN_POINT('Ctrl Pts',(-0.214119695946351,0.0117994816513621,
0.00936540572011131));
#39799=CARTESIAN_POINT('Ctrl Pts',(-0.214094978666479,0.0116154403154175,
0.00945854637191276));
#39800=CARTESIAN_POINT('Ctrl Pts',(-0.214082620026543,0.0115234196474453,
0.00950511669781349));
#39801=CARTESIAN_POINT('Ctrl Pts',(-0.214071718166771,0.0114386625650815,
0.00954609956536755));
#39802=CARTESIAN_POINT('Ctrl Pts',(-0.214061901531328,0.0113580994422348,
0.00958373978635917));
#39803=CARTESIAN_POINT('Ctrl Pts',(-0.214056993213607,0.0113178178808115,
0.00960255989685498));
#39804=CARTESIAN_POINT('Ctrl Pts',(-0.214052356864697,0.0112785699444597,
0.00962051390331013));
#39805=CARTESIAN_POINT('Ctrl Pts',(-0.214048480156471,0.011245138655905,
0.00963558167760563));
#39806=CARTESIAN_POINT('Ctrl Pts',(-0.214044603448246,0.0112117073673503,
0.00965064945190114));
#39807=CARTESIAN_POINT('Ctrl Pts',(-0.214041484259469,0.0111841374694742,
0.00966292843300825));
#39808=CARTESIAN_POINT('Ctrl Pts',(-0.214037123296481,0.0111429803313046,
0.00968087903102329));
#39809=CARTESIAN_POINT('Ctrl Pts',(-0.214032762333493,0.0111018231931349,
0.00969882962903835));
#39810=CARTESIAN_POINT('Ctrl Pts',(-0.2140271634979,0.0110469997465657,
0.00972227262366574));
#39811=CARTESIAN_POINT('Ctrl Pts',(-0.214022249173218,0.0109957218446917,
0.00974357751472393));
#39812=CARTESIAN_POINT('Ctrl Pts',(-0.214017334848535,0.0109444439428178,
0.00976488240578211));
#39813=CARTESIAN_POINT('Ctrl Pts',(-0.21401310225623,0.0108967640800364,
0.00978417682540769));
#39814=CARTESIAN_POINT('Ctrl Pts',(-0.214009080069515,0.0108484579449649,
0.00980327310576939));
#39815=CARTESIAN_POINT('Ctrl Pts',(-0.214001035696085,0.0107518456748219,
0.00984146566649278));
#39816=CARTESIAN_POINT('Ctrl Pts',(-0.213993835957383,0.0106526766076716,
0.00987872729674494));
#39817=CARTESIAN_POINT('Ctrl Pts',(-0.213987853556733,0.0105541854242721,
0.00991381013011468));
#39818=CARTESIAN_POINT('Ctrl Pts',(-0.213975888755433,0.0103572030574731,
0.00998397579685417));
#39819=CARTESIAN_POINT('Ctrl Pts',(-0.213968788113749,0.0101630030187667,
0.0100456647992242));
#39820=CARTESIAN_POINT('Ctrl Pts',(-0.213965822435937,0.00996845937459876,
0.0101006100729016));
#39821=CARTESIAN_POINT('Ctrl Pts',(-0.213962856758125,0.00977391573043078,
0.010155555346579));
#39822=CARTESIAN_POINT('Ctrl Pts',(-0.213964023065156,0.00957908264351894,
0.0102038937335934));
#39823=CARTESIAN_POINT('Ctrl Pts',(-0.21396908446874,0.00937400127475314,
0.0102473014551026));
#39824=CARTESIAN_POINT('Ctrl Pts',(-0.213971615170531,0.00927146059037024,
0.0102690053158571));
#39825=CARTESIAN_POINT('Ctrl Pts',(-0.213975121956478,0.00916633323749196,
0.0102893703986903));
#39826=CARTESIAN_POINT('Ctrl Pts',(-0.213979431254745,0.0090628082995213,
0.010307568910536));
#39827=CARTESIAN_POINT('Ctrl Pts',(-0.213981585903878,0.00901104583053597,
0.0103166681664589));
#39828=CARTESIAN_POINT('Ctrl Pts',(-0.213983940282687,0.00895969182533451,
0.0103252670482856));
#39829=CARTESIAN_POINT('Ctrl Pts',(-0.213986791258972,0.00890381663198042,
0.0103340808021143));
#39830=CARTESIAN_POINT('Ctrl Pts',(-0.213989642235257,0.00884794143862632,
0.010342894555943));
#39831=CARTESIAN_POINT('Ctrl Pts',(-0.213992993054109,0.00878752094369971,
0.0103517741168447));
#39832=CARTESIAN_POINT('Ctrl Pts',(-0.213995611973794,0.00874260648517612,
0.0103580417152856));
#39833=CARTESIAN_POINT('Ctrl Pts',(-0.213998230893478,0.00869769202665253,
0.0103643093137265));
#39834=CARTESIAN_POINT('Ctrl Pts',(-0.214000113365021,0.00866831195366434,
0.0103681739093432));
#39835=CARTESIAN_POINT('Ctrl Pts',(-0.214002517474644,0.00863218386042468,
0.0103727705888645));
#39836=CARTESIAN_POINT('Ctrl Pts',(-0.214004921584266,0.00859605576718503,
0.0103773672683857));
#39837=CARTESIAN_POINT('Ctrl Pts',(-0.214007849777381,0.00855316610357289,
0.0103825837003049));
#39838=CARTESIAN_POINT('Ctrl Pts',(-0.214010995703821,0.00850896144170923,
0.0103875992331155));
#39839=CARTESIAN_POINT('Ctrl Pts',(-0.214017287556701,0.00842055211798191,
0.0103976302987366));
#39840=CARTESIAN_POINT('Ctrl Pts',(-0.214024447245813,0.00832689656229679,
0.010407000033626));
#39841=CARTESIAN_POINT('Ctrl Pts',(-0.214032716845087,0.00822397462738881,
0.0104154199196861));
#39842=CARTESIAN_POINT('Ctrl Pts',(-0.214049256043635,0.00801813075757284,
0.0104322596918063));
#39843=CARTESIAN_POINT('Ctrl Pts',(-0.214070237444844,0.00777522053581388,
0.0104451823806317));
#39844=CARTESIAN_POINT('Ctrl Pts',(-0.214095609529044,0.00749962227620365,
0.0104457232276612));
#39845=CARTESIAN_POINT('',(-0.214184674208418,0.00275297203288764,0.00910660423566295));
#39846=CARTESIAN_POINT('Ctrl Pts',(-0.214095609529152,0.00749962227619371,
0.0104457232276635));
#39847=CARTESIAN_POINT('Ctrl Pts',(-0.214070225361772,0.00722287809655221,
0.0104451590880677));
#39848=CARTESIAN_POINT('Ctrl Pts',(-0.214049220380385,0.00697896534568404,
0.0104321129966427));
#39849=CARTESIAN_POINT('Ctrl Pts',(-0.21403264326934,0.00677222587095417,
0.0104151132536551));
#39850=CARTESIAN_POINT('Ctrl Pts',(-0.214024354713817,0.00666885613358923,
0.0104066133821613));
#39851=CARTESIAN_POINT('Ctrl Pts',(-0.214017172498679,0.00657477953844181,
0.0103971539088115));
#39852=CARTESIAN_POINT('Ctrl Pts',(-0.214010855799684,0.0064860163185143,
0.0103870326191949));
#39853=CARTESIAN_POINT('Ctrl Pts',(-0.214007697450186,0.00644163470855054,
0.0103819719743867));
#39854=CARTESIAN_POINT('Ctrl Pts',(-0.214004756250064,0.00639858488273828,
0.0103767104892244));
#39855=CARTESIAN_POINT('Ctrl Pts',(-0.214002336625303,0.00636225692718804,
0.0103720655349163));
#39856=CARTESIAN_POINT('Ctrl Pts',(-0.213999917000542,0.0063259289716378,
0.0103674205806083));
#39857=CARTESIAN_POINT('Ctrl Pts',(-0.213998016520098,0.00629630934580017,
0.0103635038297016));
#39858=CARTESIAN_POINT('Ctrl Pts',(-0.213995384865398,0.00625134630123713,
0.010357198392522));
#39859=CARTESIAN_POINT('Ctrl Pts',(-0.213992753210698,0.00620638325667409,
0.0103508929553423));
#39860=CARTESIAN_POINT('Ctrl Pts',(-0.213989394888805,0.00614610502882649,
0.0103419917952826));
#39861=CARTESIAN_POINT('Ctrl Pts',(-0.21398653156378,0.00609034800684164,
0.0103331590792549));
#39862=CARTESIAN_POINT('Ctrl Pts',(-0.213983668238756,0.00603459098485678,
0.0103243263632272));
#39863=CARTESIAN_POINT('Ctrl Pts',(-0.213981296702793,0.00598333124078719,
0.0103157094453065));
#39864=CARTESIAN_POINT('Ctrl Pts',(-0.213979122749828,0.00593168239145384,
0.0103065968143388));
#39865=CARTESIAN_POINT('Ctrl Pts',(-0.213974774843896,0.00582838469278714,
0.0102883715524033));
#39866=CARTESIAN_POINT('Ctrl Pts',(-0.213971220854217,0.00572356184595577,
0.0102679987910534));
#39867=CARTESIAN_POINT('Ctrl Pts',(-0.213968629170881,0.0056214786218438,
0.0102463358658497));
#39868=CARTESIAN_POINT('Ctrl Pts',(-0.213963445804209,0.00541731217361988,
0.0102030100154425));
#39869=CARTESIAN_POINT('Ctrl Pts',(-0.213962101745618,0.00522400033366578,
0.0101549790725054));
#39870=CARTESIAN_POINT('Ctrl Pts',(-0.213964873552575,0.00503030005499574,
0.01010023830303));
#39871=CARTESIAN_POINT('Ctrl Pts',(-0.213967645359531,0.0048365997763257,
0.0100454975335545));
#39872=CARTESIAN_POINT('Ctrl Pts',(-0.213974537218841,0.00464258063418668,
0.00998385461054552));
#39873=CARTESIAN_POINT('Ctrl Pts',(-0.213986279184264,0.00444636027725606,
0.00991397063797153));
#39874=CARTESIAN_POINT('Ctrl Pts',(-0.213992150166976,0.00434825009879075,
0.00987902865168454));
#39875=CARTESIAN_POINT('Ctrl Pts',(-0.2139992347739,0.0042496038046692,
0.00984197597949799));
#39876=CARTESIAN_POINT('Ctrl Pts',(-0.214007169132657,0.00415347647942909,
0.00980399912099018));
#39877=CARTESIAN_POINT('Ctrl Pts',(-0.214011136312036,0.00410541281680903,
0.00978501069173628));
#39878=CARTESIAN_POINT('Ctrl Pts',(-0.214015315205515,0.00405796652499624,
0.00976582446738269));
#39879=CARTESIAN_POINT('Ctrl Pts',(-0.214020163647885,0.00400702271758286,
0.00974467724691843));
#39880=CARTESIAN_POINT('Ctrl Pts',(-0.214025012090255,0.00395607891016948,
0.00972353002645416));
#39881=CARTESIAN_POINT('Ctrl Pts',(-0.214030532775055,0.00390168841775467,
0.00970029807802345));
#39882=CARTESIAN_POINT('Ctrl Pts',(-0.214034858845576,0.00386064793818244,
0.00968241922088636));
#39883=CARTESIAN_POINT('Ctrl Pts',(-0.214039184916098,0.00381960745861021,
0.00966454036374926));
#39884=CARTESIAN_POINT('Ctrl Pts',(-0.214042312567376,0.00379183998995763,
0.0096521893849458));
#39885=CARTESIAN_POINT('Ctrl Pts',(-0.214046191819162,0.00375827537784855,
0.00963707794241496));
#39886=CARTESIAN_POINT('Ctrl Pts',(-0.214050071070949,0.00372471076573947,
0.00962196649988412));
#39887=CARTESIAN_POINT('Ctrl Pts',(-0.214054704007104,0.00368539291187765,
0.00960399886809182));
#39888=CARTESIAN_POINT('Ctrl Pts',(-0.214059615038916,0.00364501315118274,
0.00958515134653227));
#39889=CARTESIAN_POINT('Ctrl Pts',(-0.214069437102542,0.00356425362979292,
0.00954745630341316));
#39890=CARTESIAN_POINT('Ctrl Pts',(-0.21408036893767,0.00347918796641314,
0.00950636164773408));
#39891=CARTESIAN_POINT('Ctrl Pts',(-0.214092773485727,0.00338681699209809,
0.0094596464485715));
#39892=CARTESIAN_POINT('Ctrl Pts',(-0.214117582581841,0.00320207504346799,
0.00936621605024635));
#39893=CARTESIAN_POINT('Ctrl Pts',(-0.214148284403255,0.00298816452839985,
0.00925021741124221));
#39894=CARTESIAN_POINT('Ctrl Pts',(-0.214184674208418,0.00275297203288764,
0.00910660423566295));
#39895=CARTESIAN_POINT('Ctrl Pts',(-0.214184706718132,0.00275296401068821,
0.0091066000178277));
#39896=CARTESIAN_POINT('Ctrl Pts',(-0.213850325206826,0.00275300942663134,
0.00909934875292539));
#39897=CARTESIAN_POINT('Ctrl Pts',(-0.213516724599567,0.00275305138100511,
0.00909211236159907));
#39898=CARTESIAN_POINT('Ctrl Pts',(-0.213184266201433,0.00275308988725477,
0.0090848987175866));
#39899=CARTESIAN_POINT('Origin',(-0.223676757797681,0.00749999628416647,
0.00172570651533405));
#39900=CARTESIAN_POINT('',(-0.22309284651216,0.00749584998232693,0.0106501221268793));
#39901=CARTESIAN_POINT('',(-0.223392296011988,0.00186204391920834,0.00865271087646174));
#39902=CARTESIAN_POINT('Ctrl Pts',(-0.223392296011988,0.00186204391920834,
0.00865271087646174));
#39903=CARTESIAN_POINT('Ctrl Pts',(-0.223319871060027,0.00211980418497422,
0.00886086131836836));
#39904=CARTESIAN_POINT('Ctrl Pts',(-0.223230417685778,0.00247217783692335,
0.00911151291301624));
#39905=CARTESIAN_POINT('Ctrl Pts',(-0.223144978048942,0.00287497601905299,
0.00936251343998583));
#39906=CARTESIAN_POINT('Ctrl Pts',(-0.22310564727859,0.00308846183391502,
0.00948703711985114));
#39907=CARTESIAN_POINT('Ctrl Pts',(-0.22305914643883,0.00341474467215678,
0.00966364610365276));
#39908=CARTESIAN_POINT('Ctrl Pts',(-0.223024306677471,0.00374403882274536,
0.00982342475701909));
#39909=CARTESIAN_POINT('Ctrl Pts',(-0.222996283861068,0.0041018555788969,
0.00998004297101686));
#39910=CARTESIAN_POINT('Ctrl Pts',(-0.222969194008887,0.00463196501065476,
0.0101823328381467));
#39911=CARTESIAN_POINT('Ctrl Pts',(-0.22296083527953,0.00510571723112372,
0.0103269540955497));
#39912=CARTESIAN_POINT('Ctrl Pts',(-0.222966830172775,0.00554467492095415,
0.010432283226809));
#39913=CARTESIAN_POINT('Ctrl Pts',(-0.222973890152792,0.00578493801794152,
0.0104821858289615));
#39914=CARTESIAN_POINT('Ctrl Pts',(-0.222982369849644,0.00598932331249166,
0.0105195922928726));
#39915=CARTESIAN_POINT('Ctrl Pts',(-0.222988213034318,0.00610111321959354,
0.0105379385005546));
#39916=CARTESIAN_POINT('Ctrl Pts',(-0.223000242325119,0.00630906110798175,
0.0105696138144231));
#39917=CARTESIAN_POINT('Ctrl Pts',(-0.223027517337247,0.00671085691261999,
0.0106196318321823));
#39918=CARTESIAN_POINT('Ctrl Pts',(-0.223063339697324,0.00715748003617067,
0.0106493315311508));
#39919=CARTESIAN_POINT('Ctrl Pts',(-0.22309284651216,0.00749584998232693,
0.0106501221268793));
#39920=CARTESIAN_POINT('',(-0.2233982585897,0.013123285512218,0.00866473942159963));
#39921=CARTESIAN_POINT('Ctrl Pts',(-0.223092846396494,0.00749585131677931,
0.0106501221250134));
#39922=CARTESIAN_POINT('Ctrl Pts',(-0.223063630887188,0.00783291331843735,
0.0106496508010981));
#39923=CARTESIAN_POINT('Ctrl Pts',(-0.223028200638697,0.00827785100296254,
0.0106205981598599));
#39924=CARTESIAN_POINT('Ctrl Pts',(-0.223001293631607,0.00867832292771731,
0.0105713108445289));
#39925=CARTESIAN_POINT('Ctrl Pts',(-0.222989468933273,0.00888549981070341,
0.0105400738724192));
#39926=CARTESIAN_POINT('Ctrl Pts',(-0.222983723480319,0.00899722891238163,
0.0105219073079855));
#39927=CARTESIAN_POINT('Ctrl Pts',(-0.222975502745266,0.00919991606191928,
0.0104851529915839));
#39928=CARTESIAN_POINT('Ctrl Pts',(-0.222968716597595,0.00943907010756142,
0.0104359371442604));
#39929=CARTESIAN_POINT('Ctrl Pts',(-0.22296319930633,0.00987692923929947,
0.0103317776510189));
#39930=CARTESIAN_POINT('Ctrl Pts',(-0.222972029344618,0.0103524546158386,
0.0101877530993365));
#39931=CARTESIAN_POINT('Ctrl Pts',(-0.222999554069768,0.0108861515781492,
0.0099850487725875));
#39932=CARTESIAN_POINT('Ctrl Pts',(-0.223027657018532,0.0112442757284449,
0.00982888868406289));
#39933=CARTESIAN_POINT('Ctrl Pts',(-0.223062483445131,0.0115730293585616,
0.00966992388725343));
#39934=CARTESIAN_POINT('Ctrl Pts',(-0.223108468347194,0.0118955673702011,
0.00949610299343309));
#39935=CARTESIAN_POINT('Ctrl Pts',(-0.223148241664016,0.0121105250457455,
0.00937134181568169));
#39936=CARTESIAN_POINT('Ctrl Pts',(-0.223234432572955,0.012513148459596,
0.00912151309303764));
#39937=CARTESIAN_POINT('Ctrl Pts',(-0.223324944071789,0.0128655990519436,
0.0088719056596678));
#39938=CARTESIAN_POINT('Ctrl Pts',(-0.2233982585897,0.013123285512218,0.00866473942159963));
#39939=CARTESIAN_POINT('',(-0.224398127361235,0.0131227913316661,0.0086866275128953));
#39940=CARTESIAN_POINT('Ctrl Pts',(-0.223398249886961,0.0131232867503721,
0.00866473823159148));
#39941=CARTESIAN_POINT('Ctrl Pts',(-0.223731523675107,0.0131231213967512,
0.00867203444050197));
#39942=CARTESIAN_POINT('Ctrl Pts',(-0.22406487360808,0.0131229619290297,
0.00867932750749511));
#39943=CARTESIAN_POINT('Ctrl Pts',(-0.224398096141527,0.013122808446012,
0.00868661298034067));
#39944=CARTESIAN_POINT('',(-0.224092572998184,0.00749536846703943,0.0106715944441166));
#39945=CARTESIAN_POINT('Ctrl Pts',(-0.224398127361235,0.0131227913316661,
0.0086866275128953));
#39946=CARTESIAN_POINT('Ctrl Pts',(-0.224325062414434,0.012865842986752,
0.00889316997404273));
#39947=CARTESIAN_POINT('Ctrl Pts',(-0.224234820704135,0.0125144219497046,
0.00914211665554571));
#39948=CARTESIAN_POINT('Ctrl Pts',(-0.224148755853197,0.0121126796310063,
0.00939153056882088));
#39949=CARTESIAN_POINT('Ctrl Pts',(-0.224109017097858,0.0118984407581323,
0.00951597785856116));
#39950=CARTESIAN_POINT('Ctrl Pts',(-0.224062783214931,0.0115753502059685,
0.0096902410433109));
#39951=CARTESIAN_POINT('Ctrl Pts',(-0.224027819291741,0.0112462212233988,
0.00984947839760243));
#39952=CARTESIAN_POINT('Ctrl Pts',(-0.22399959162762,0.0108878152232127,
0.010005881088725));
#39953=CARTESIAN_POINT('Ctrl Pts',(-0.223971919420138,0.0103523511641684,
0.0102092626278178));
#39954=CARTESIAN_POINT('Ctrl Pts',(-0.223963160381509,0.00988219899480068,
0.0103516928623865));
#39955=CARTESIAN_POINT('Ctrl Pts',(-0.223968441757534,0.0094464451478849,
0.0104557627503415));
#39956=CARTESIAN_POINT('Ctrl Pts',(-0.223975077093011,0.00920839189318166,
0.010504967431807));
#39957=CARTESIAN_POINT('Ctrl Pts',(-0.223983110990325,0.00900703426964022,
0.0105417005683667));
#39958=CARTESIAN_POINT('Ctrl Pts',(-0.223988835346065,0.0088942902955332,
0.0105601622854623));
#39959=CARTESIAN_POINT('Ctrl Pts',(-0.224000615907753,0.00868625901717492,
0.0105917267871887));
#39960=CARTESIAN_POINT('Ctrl Pts',(-0.22402755697167,0.0082832671038718,
0.010641668948832));
#39961=CARTESIAN_POINT('Ctrl Pts',(-0.224063163807534,0.00783511181037311,
0.0106711391391908));
#39962=CARTESIAN_POINT('Ctrl Pts',(-0.224092572998184,0.00749536846703943,
0.0106715944441166));
#39963=CARTESIAN_POINT('',(-0.224391698001265,0.00186171520950775,0.0086738967910923));
#39964=CARTESIAN_POINT('Ctrl Pts',(-0.224092573136878,0.00749536686481965,
0.0106715944462637));
#39965=CARTESIAN_POINT('Ctrl Pts',(-0.224063181659026,0.00715789448494786,
0.0106707879238547));
#39966=CARTESIAN_POINT('Ctrl Pts',(-0.224027485085123,0.00671245635685632,
0.0106412153002841));
#39967=CARTESIAN_POINT('Ctrl Pts',(-0.224000282681402,0.00631182732071981,
0.0105914571765522));
#39968=CARTESIAN_POINT('Ctrl Pts',(-0.223988268398574,0.00610438871051628,
0.0105599315069899));
#39969=CARTESIAN_POINT('Ctrl Pts',(-0.223982438964663,0.00599317088837536,
0.0105417285207031));
#39970=CARTESIAN_POINT('Ctrl Pts',(-0.223973911582342,0.0057884503761421,
0.0105043511524616));
#39971=CARTESIAN_POINT('Ctrl Pts',(-0.223966812223066,0.00554799671714812,
0.0104545007048094));
#39972=CARTESIAN_POINT('Ctrl Pts',(-0.223960725771381,0.00510876621667219,
0.0103493125263479));
#39973=CARTESIAN_POINT('Ctrl Pts',(-0.223969092055907,0.00463281516023792,
0.0102040504815577));
#39974=CARTESIAN_POINT('Ctrl Pts',(-0.223995910584984,0.00410544707731089,
0.0100029403064932));
#39975=CARTESIAN_POINT('Ctrl Pts',(-0.224023629066248,0.00374891304215397,
0.00984712705576497));
#39976=CARTESIAN_POINT('Ctrl Pts',(-0.224058140037829,0.00342059928890112,
0.00968806171234968));
#39977=CARTESIAN_POINT('Ctrl Pts',(-0.224103946844588,0.00309637190744777,
0.00951295535214167));
#39978=CARTESIAN_POINT('Ctrl Pts',(-0.224143508176959,0.00288006695304061,
0.00938706853711633));
#39979=CARTESIAN_POINT('Ctrl Pts',(-0.224229127635015,0.00247511074954968,
0.00913501513009971));
#39980=CARTESIAN_POINT('Ctrl Pts',(-0.224318956776766,0.00212070098651109,
0.00888305882592809));
#39981=CARTESIAN_POINT('Ctrl Pts',(-0.224391698001265,0.00186171520950775,
0.0086738967910923));
#39982=CARTESIAN_POINT('Ctrl Pts',(-0.224391663297086,0.00186170374604395,
0.0086738867188744));
#39983=CARTESIAN_POINT('Ctrl Pts',(-0.224058368109329,0.00186182240933105,
0.00866682869105414));
#39984=CARTESIAN_POINT('Ctrl Pts',(-0.223725161158108,0.00186193524227883,
0.0086597678079791));
#39985=CARTESIAN_POINT('Ctrl Pts',(-0.223392285411273,0.00186204218687632,
0.00865270923953699));
#39986=CARTESIAN_POINT('Origin',(-0.211568383091034,0.00749999976424864,
0.00128327533895461));
#39987=CARTESIAN_POINT('',(-0.2110965359026,0.00749997454127243,0.0103787827909976));
#39988=CARTESIAN_POINT('',(-0.211183402636931,0.00275068069530849,0.00904332274846592));
#39989=CARTESIAN_POINT('Ctrl Pts',(-0.211183402636931,0.00275068069530849,
0.00904332274846592));
#39990=CARTESIAN_POINT('Ctrl Pts',(-0.211147095219407,0.00298515572002027,
0.00918594988314655));
#39991=CARTESIAN_POINT('Ctrl Pts',(-0.211101192602613,0.00330488634667183,
0.00935868020099563));
#39992=CARTESIAN_POINT('Ctrl Pts',(-0.211063143045044,0.00360117936401887,
0.00950160180870966));
#39993=CARTESIAN_POINT('Ctrl Pts',(-0.21104475417619,0.0037577018790529,
0.00957289220178136));
#39994=CARTESIAN_POINT('Ctrl Pts',(-0.211035467150038,0.00384039342259991,
0.00960968445757509));
#39995=CARTESIAN_POINT('Ctrl Pts',(-0.211019066687301,0.0040029883061291,
0.00967908598737613));
#39996=CARTESIAN_POINT('Ctrl Pts',(-0.211002549970838,0.00419272029530249,
0.00975560521859346));
#39997=CARTESIAN_POINT('Ctrl Pts',(-0.210978116351287,0.00453848546937588,
0.00988555577385184));
#39998=CARTESIAN_POINT('Ctrl Pts',(-0.210961424663072,0.00503260509810232,
0.0100417888938481));
#39999=CARTESIAN_POINT('Ctrl Pts',(-0.210965443153373,0.00551404341866351,
0.0101610108572086));
#40000=CARTESIAN_POINT('Ctrl Pts',(-0.210978272865404,0.00588224623587764,
0.0102322905439714));
#40001=CARTESIAN_POINT('Ctrl Pts',(-0.210987956400489,0.00608781575055283,
0.0102667980265165));
#40002=CARTESIAN_POINT('Ctrl Pts',(-0.210998218524945,0.00626946825961742,
0.0102934418192037));
#40003=CARTESIAN_POINT('Ctrl Pts',(-0.211003938107319,0.00635797387487456,
0.0103049979326545));
#40004=CARTESIAN_POINT('Ctrl Pts',(-0.211015693571684,0.00653001085820023,
0.010326006931539));
#40005=CARTESIAN_POINT('Ctrl Pts',(-0.211040617677658,0.0068586970342682,
0.0103587408428194));
#40006=CARTESIAN_POINT('Ctrl Pts',(-0.211071626779655,0.00722383932448257,
0.0103782401381245));
#40007=CARTESIAN_POINT('Ctrl Pts',(-0.2110965359026,0.00749997454127243,
0.0103787827909976));
#40008=CARTESIAN_POINT('',(-0.21118417804845,0.0122471792256319,0.009044647334993));
#40009=CARTESIAN_POINT('Ctrl Pts',(-0.211096535799883,0.00749997567494527,
0.010378782788766));
#40010=CARTESIAN_POINT('Ctrl Pts',(-0.211071573366554,0.00777549325047854,
0.0103782404346483));
#40011=CARTESIAN_POINT('Ctrl Pts',(-0.211040513267916,0.00813985761538285,
0.0103588270763272));
#40012=CARTESIAN_POINT('Ctrl Pts',(-0.211015576714647,0.00846798462518059,
0.0103262153638346));
#40013=CARTESIAN_POINT('Ctrl Pts',(-0.211003834816079,0.00863970531938501,
0.0103052888750913));
#40014=CARTESIAN_POINT('Ctrl Pts',(-0.210998116574614,0.00872823661427716,
0.0102937495397744));
#40015=CARTESIAN_POINT('Ctrl Pts',(-0.210987925682693,0.00890910709332001,
0.0102672755357513));
#40016=CARTESIAN_POINT('Ctrl Pts',(-0.210978321795415,0.00911419488984098,
0.010232927644559));
#40017=CARTESIAN_POINT('Ctrl Pts',(-0.21096565564001,0.00948174160645032,
0.0101619632965175));
#40018=CARTESIAN_POINT('Ctrl Pts',(-0.210961963015379,0.00996543783438438,
0.0100423573285345));
#40019=CARTESIAN_POINT('Ctrl Pts',(-0.210978912084468,0.0104576617459814,
0.0098868796580418));
#40020=CARTESIAN_POINT('Ctrl Pts',(-0.211003457455194,0.0108036566335765,
0.00975703895053704));
#40021=CARTESIAN_POINT('Ctrl Pts',(-0.211020020345204,0.0109935540978411,
0.00968054497958633));
#40022=CARTESIAN_POINT('Ctrl Pts',(-0.211036452134397,0.0111564247405211,
0.00961110274277066));
#40023=CARTESIAN_POINT('Ctrl Pts',(-0.211045742641945,0.0112392207523565,
0.00957430044553631));
#40024=CARTESIAN_POINT('Ctrl Pts',(-0.211064129984168,0.0113959395659256,
0.00950298930486255));
#40025=CARTESIAN_POINT('Ctrl Pts',(-0.211102140859678,0.0116925422723936,
0.00936004108598765));
#40026=CARTESIAN_POINT('Ctrl Pts',(-0.211147954901023,0.0120125365367652,
0.00918728999384757));
#40027=CARTESIAN_POINT('Ctrl Pts',(-0.21118417804845,0.0122471792256319,
0.009044647334993));
#40028=CARTESIAN_POINT('',(-0.212184953537621,0.0122473744306414,0.00906630151341282));
#40029=CARTESIAN_POINT('Ctrl Pts',(-0.21118422788918,0.0122471764791729,
0.00904465009819522));
#40030=CARTESIAN_POINT('Ctrl Pts',(-0.211517519859832,0.0122472431453679,
0.00905186065814718));
#40031=CARTESIAN_POINT('Ctrl Pts',(-0.211851190949066,0.0122473134521283,
0.00905907723991485));
#40032=CARTESIAN_POINT('Ctrl Pts',(-0.212184989270622,0.0122473873638838,
0.00906629438464372));
#40033=CARTESIAN_POINT('',(-0.212096216935387,0.00749993309271591,0.010400531159228));
#40034=CARTESIAN_POINT('Ctrl Pts',(-0.212184953537621,0.0122473744306414,
0.00906630151341282));
#40035=CARTESIAN_POINT('Ctrl Pts',(-0.212148608862081,0.0120119705243528,
0.00920941487666883));
#40036=CARTESIAN_POINT('Ctrl Pts',(-0.212117954036947,0.0117979090212747,
0.00932500833085451));
#40037=CARTESIAN_POINT('Ctrl Pts',(-0.212093189286655,0.0116130124708475,
0.00941812959134124));
#40038=CARTESIAN_POINT('Ctrl Pts',(-0.212080806911509,0.0115205641956338,
0.0094646902215846));
#40039=CARTESIAN_POINT('Ctrl Pts',(-0.212069896597886,0.0114354199872055,
0.00950565381710398));
#40040=CARTESIAN_POINT('Ctrl Pts',(-0.212060100467986,0.0113546092190502,
0.00954321884104617));
#40041=CARTESIAN_POINT('Ctrl Pts',(-0.212055202403036,0.0113142038349725,
0.00956200135301727));
#40042=CARTESIAN_POINT('Ctrl Pts',(-0.212050583528796,0.0112748674132463,
0.00957990458571435));
#40043=CARTESIAN_POINT('Ctrl Pts',(-0.212046712568544,0.0112412478030318,
0.00959497929731873));
#40044=CARTESIAN_POINT('Ctrl Pts',(-0.212042841608291,0.0112076281928174,
0.00961005400892311));
#40045=CARTESIAN_POINT('Ctrl Pts',(-0.212039716504683,0.0111797685814931,
0.0096223947625136));
#40046=CARTESIAN_POINT('Ctrl Pts',(-0.212035415305258,0.0111387765475974,
0.00964018017975509));
#40047=CARTESIAN_POINT('Ctrl Pts',(-0.212031114105832,0.0110977845137017,
0.00965796559699658));
#40048=CARTESIAN_POINT('Ctrl Pts',(-0.212025640550936,0.0110435846392935,
0.00968102375737418));
#40049=CARTESIAN_POINT('Ctrl Pts',(-0.212020830685943,0.0109927516904921,
0.0097020431984729));
#40050=CARTESIAN_POINT('Ctrl Pts',(-0.212016020820949,0.0109419187416906,
0.00972306263957162));
#40051=CARTESIAN_POINT('Ctrl Pts',(-0.212011872008556,0.010894502303713,
0.00974216458214745));
#40052=CARTESIAN_POINT('Ctrl Pts',(-0.212007934174403,0.0108464578821206,
0.00976107397304423));
#40053=CARTESIAN_POINT('Ctrl Pts',(-0.212000058506097,0.0107503690389357,
0.00979889275483778));
#40054=CARTESIAN_POINT('Ctrl Pts',(-0.211993029531615,0.010651721257402,
0.00983581351009456));
#40055=CARTESIAN_POINT('Ctrl Pts',(-0.211987203427364,0.0105533047573211,
0.00987073287076495));
#40056=CARTESIAN_POINT('Ctrl Pts',(-0.211975551218862,0.0103564717571592,
0.00994057159210573));
#40057=CARTESIAN_POINT('Ctrl Pts',(-0.211968707612936,0.0101605940883872,
0.0100025370378822));
#40058=CARTESIAN_POINT('Ctrl Pts',(-0.211965975423112,0.0099663576093433,
0.0100571576241214));
#40059=CARTESIAN_POINT('Ctrl Pts',(-0.211963243233289,0.00977212113029945,
0.0101117782103606));
#40060=CARTESIAN_POINT('Ctrl Pts',(-0.211964616403369,0.0095796185691958,
0.0101593323058388));
#40061=CARTESIAN_POINT('Ctrl Pts',(-0.211969788366012,0.00937629259852591,
0.01020228070507));
#40062=CARTESIAN_POINT('Ctrl Pts',(-0.211972374347333,0.00927462961319097,
0.0102237549046856));
#40063=CARTESIAN_POINT('Ctrl Pts',(-0.211975912663703,0.0091702339273998,
0.0102439564753252));
#40064=CARTESIAN_POINT('Ctrl Pts',(-0.21198024063847,0.00906742206628467,
0.0102620249393407));
#40065=CARTESIAN_POINT('Ctrl Pts',(-0.211982404625853,0.00901601613572711,
0.0102710591713484));
#40066=CARTESIAN_POINT('Ctrl Pts',(-0.211984765148223,0.00896501374588465,
0.0102796005580246));
#40067=CARTESIAN_POINT('Ctrl Pts',(-0.211987610756156,0.00890961963149956,
0.0102883465429082));
#40068=CARTESIAN_POINT('Ctrl Pts',(-0.211990456364088,0.00885422551711447,
0.0102970925277919));
#40069=CARTESIAN_POINT('Ctrl Pts',(-0.21199379016818,0.00879441655146242,
0.0103059001321234));
#40070=CARTESIAN_POINT('Ctrl Pts',(-0.211996413112179,0.00874961583566324,
0.0103121670340523));
#40071=CARTESIAN_POINT('Ctrl Pts',(-0.211999036056178,0.00870481511986407,
0.0103184339359812));
#40072=CARTESIAN_POINT('Ctrl Pts',(-0.212000943752514,0.00867505009895193,
0.0103223618108506));
#40073=CARTESIAN_POINT('Ctrl Pts',(-0.212003363382826,0.0086386498772624,
0.0103270043852339));
#40074=CARTESIAN_POINT('Ctrl Pts',(-0.212005783013139,0.00860224965557287,
0.0103316469596172));
#40075=CARTESIAN_POINT('Ctrl Pts',(-0.21200871695817,0.00855920099241481,
0.0103368948021386));
#40076=CARTESIAN_POINT('Ctrl Pts',(-0.212011866469682,0.00851480072693946,
0.0103419449315219));
#40077=CARTESIAN_POINT('Ctrl Pts',(-0.212018165492707,0.00842600019598875,
0.0103520451902885));
#40078=CARTESIAN_POINT('Ctrl Pts',(-0.212025323759104,0.00833180673148592,
0.0103614935292938));
#40079=CARTESIAN_POINT('Ctrl Pts',(-0.212033577950091,0.00822830849881047,
0.0103699817552531));
#40080=CARTESIAN_POINT('Ctrl Pts',(-0.212050086332064,0.00802131203345956,
0.0103869582071715));
#40081=CARTESIAN_POINT('Ctrl Pts',(-0.212070980805244,0.00777709603119313,
0.0103999842177033));
#40082=CARTESIAN_POINT('Ctrl Pts',(-0.212096216935389,0.00749993309273471,
0.0104005311592281));
#40083=CARTESIAN_POINT('',(-0.212183765169463,0.00275128401172433,0.00906545360362375));
#40084=CARTESIAN_POINT('Ctrl Pts',(-0.212096216935387,0.00749993309271591,
0.010400531159228));
#40085=CARTESIAN_POINT('Ctrl Pts',(-0.212071126307345,0.00722322961499376,
0.0103999832300892));
#40086=CARTESIAN_POINT('Ctrl Pts',(-0.212050323820085,0.00697932624712693,
0.0103869945506515));
#40087=CARTESIAN_POINT('Ctrl Pts',(-0.212033859878558,0.00677255811334454,
0.0103700572244492));
#40088=CARTESIAN_POINT('Ctrl Pts',(-0.212025627907794,0.00666917404645334,
0.0103615885613481));
#40089=CARTESIAN_POINT('Ctrl Pts',(-0.212018479948959,0.00657507361336468,
0.010352161442409));
#40090=CARTESIAN_POINT('Ctrl Pts',(-0.212012174388185,0.00648628210784819,
0.0103420727979329));
#40091=CARTESIAN_POINT('Ctrl Pts',(-0.212009021607799,0.00644188635508995,
0.0103370284756949));
#40092=CARTESIAN_POINT('Ctrl Pts',(-0.212006080193597,0.00639882124771468,
0.0103317835311436));
#40093=CARTESIAN_POINT('Ctrl Pts',(-0.212003655779862,0.00636247064645391,
0.010327151684048));
#40094=CARTESIAN_POINT('Ctrl Pts',(-0.212001231366128,0.00632612004519314,
0.0103225198369524));
#40095=CARTESIAN_POINT('Ctrl Pts',(-0.211999321532852,0.0062964705099328,
0.0103186123262797));
#40096=CARTESIAN_POINT('Ctrl Pts',(-0.211996671040146,0.00625149580262887,
0.010312326350296));
#40097=CARTESIAN_POINT('Ctrl Pts',(-0.211994020547439,0.00620652109532495,
0.0103060403743122));
#40098=CARTESIAN_POINT('Ctrl Pts',(-0.211990633880624,0.00614624923462854,
0.0102971697588912));
#40099=CARTESIAN_POINT('Ctrl Pts',(-0.21198774295475,0.00609049435275109,
0.0102883669432379));
#40100=CARTESIAN_POINT('Ctrl Pts',(-0.211984852028876,0.00603473947087364,
0.0102795641275845));
#40101=CARTESIAN_POINT('Ctrl Pts',(-0.211982453651153,0.00598347782917449,
0.0102709758732188));
#40102=CARTESIAN_POINT('Ctrl Pts',(-0.211980251215045,0.00593181943961855,
0.0102618921530657));
#40103=CARTESIAN_POINT('Ctrl Pts',(-0.211975846342829,0.00582850266050667,
0.0102437247127595));
#40104=CARTESIAN_POINT('Ctrl Pts',(-0.21197222883814,0.00572363000883807,
0.0102234098804427));
#40105=CARTESIAN_POINT('Ctrl Pts',(-0.21196956741466,0.00562157793695026,
0.010201826560603));
#40106=CARTESIAN_POINT('Ctrl Pts',(-0.2119642445677,0.00541747379317463,
0.0101586599209237));
#40107=CARTESIAN_POINT('Ctrl Pts',(-0.211962735409498,0.00522454320374596,
0.010110908237939));
#40108=CARTESIAN_POINT('Ctrl Pts',(-0.211965334255942,0.00503024391291162,
0.0100561856635299));
#40109=CARTESIAN_POINT('Ctrl Pts',(-0.211967933102386,0.00483594462207727,
0.0100014630891208));
#40110=CARTESIAN_POINT('Ctrl Pts',(-0.211974645886691,0.00464036808754224,
0.00993949688927384));
#40111=CARTESIAN_POINT('Ctrl Pts',(-0.211986174288779,0.0044439250258746,
0.00986972273612033));
#40112=CARTESIAN_POINT('Ctrl Pts',(-0.211991938489823,0.00434570349504078,
0.00983483565954358));
#40113=CARTESIAN_POINT('Ctrl Pts',(-0.211998907343389,0.00424727340981272,
0.00979796220794339));
#40114=CARTESIAN_POINT('Ctrl Pts',(-0.212006726980613,0.00415142401522088,
0.00976020909830612));
#40115=CARTESIAN_POINT('Ctrl Pts',(-0.212010636799224,0.00410349931792496,
0.00974133254348749));
#40116=CARTESIAN_POINT('Ctrl Pts',(-0.212014758624468,0.00405620812295089,
0.00972226775875776));
#40117=CARTESIAN_POINT('Ctrl Pts',(-0.212019538220643,0.00400553612295486,
0.00970130241315875));
#40118=CARTESIAN_POINT('Ctrl Pts',(-0.212024317816818,0.00395486412295883,
0.00968033706755973));
#40119=CARTESIAN_POINT('Ctrl Pts',(-0.212029757792179,0.00390086039173556,
0.00965735126569874));
#40120=CARTESIAN_POINT('Ctrl Pts',(-0.212034039987089,0.00385996834286666,
0.00963960170087009));
#40121=CARTESIAN_POINT('Ctrl Pts',(-0.212038322181999,0.00381907629399776,
0.00962185213604143));
#40122=CARTESIAN_POINT('Ctrl Pts',(-0.212041442891325,0.00379122118675441,
0.00960950912507693));
#40123=CARTESIAN_POINT('Ctrl Pts',(-0.212045308742462,0.00375762262362403,
0.00959443826985068));
#40124=CARTESIAN_POINT('Ctrl Pts',(-0.2120491745936,0.00372402406049364,
0.00957936741462442));
#40125=CARTESIAN_POINT('Ctrl Pts',(-0.21205378762908,0.0036847249345285,
0.00956147482426794));
#40126=CARTESIAN_POINT('Ctrl Pts',(-0.212058682884334,0.00364434597571046,
0.00954269834621542));
#40127=CARTESIAN_POINT('Ctrl Pts',(-0.212068473394842,0.00356358805807439,
0.00950514539011038));
#40128=CARTESIAN_POINT('Ctrl Pts',(-0.212079390220398,0.00347845353315219,
0.00946417474742));
#40129=CARTESIAN_POINT('Ctrl Pts',(-0.212091788556574,0.00338599268517819,
0.00941759379839564));
#40130=CARTESIAN_POINT('Ctrl Pts',(-0.212116585228927,0.00320107098923018,
0.00932443190034691));
#40131=CARTESIAN_POINT('Ctrl Pts',(-0.212147309727277,0.00298689421470239,
0.00920874679129024));
#40132=CARTESIAN_POINT('Ctrl Pts',(-0.212183765169463,0.00275128401172433,
0.00906545360362375));
#40133=CARTESIAN_POINT('Ctrl Pts',(-0.212183802162308,0.00275127625620254,
0.00906544966550962));
#40134=CARTESIAN_POINT('Ctrl Pts',(-0.211850395705467,0.00275108062549403,
0.00905807711035799));
#40135=CARTESIAN_POINT('Ctrl Pts',(-0.211516878203266,0.00275088152870816,
0.00905070000977781));
#40136=CARTESIAN_POINT('Ctrl Pts',(-0.211183457783125,0.0027506790911641,
0.00904332296693787));
#40137=CARTESIAN_POINT('Origin',(-0.201568052764461,0.00749999926826592,
0.000898602350899668));
#40138=CARTESIAN_POINT('',(-0.201099819882141,0.00749914619770346,0.0101529062582246));
#40139=CARTESIAN_POINT('',(-0.201180426584977,0.0027404758504493,0.00883792993396412));
#40140=CARTESIAN_POINT('Ctrl Pts',(-0.201180426584977,0.0027404758504493,
0.00883792993396412));
#40141=CARTESIAN_POINT('Ctrl Pts',(-0.201143782776895,0.00297687352666821,
0.00897876952690809));
#40142=CARTESIAN_POINT('Ctrl Pts',(-0.201098326821028,0.00329208064462831,
0.00914639237872595));
#40143=CARTESIAN_POINT('Ctrl Pts',(-0.201053656234426,0.00364905443742606,
0.00931418085756173));
#40144=CARTESIAN_POINT('Ctrl Pts',(-0.2010333398498,0.00382564426305905,
0.00939269762319622));
#40145=CARTESIAN_POINT('Ctrl Pts',(-0.201004911345248,0.0041388485598608,
0.00952147497706033));
#40146=CARTESIAN_POINT('Ctrl Pts',(-0.200980856006014,0.00451692057273125,
0.00966086163852431));
#40147=CARTESIAN_POINT('Ctrl Pts',(-0.200965882884491,0.00504039570807835,
0.00982439009474785));
#40148=CARTESIAN_POINT('Ctrl Pts',(-0.200972067968975,0.00550094059850311,
0.0099359440718681));
#40149=CARTESIAN_POINT('Ctrl Pts',(-0.200985770459153,0.00587373777427713,
0.010007547779862));
#40150=CARTESIAN_POINT('Ctrl Pts',(-0.200995828352292,0.00608227698546498,
0.0100420971753329));
#40151=CARTESIAN_POINT('Ctrl Pts',(-0.201006404478933,0.0062689806201438,
0.0100690695042997));
#40152=CARTESIAN_POINT('Ctrl Pts',(-0.201012027549101,0.00635736976848426,
0.0100803938087593));
#40153=CARTESIAN_POINT('Ctrl Pts',(-0.201023530642222,0.0065306602030437,
0.0101011948342447));
#40154=CARTESIAN_POINT('Ctrl Pts',(-0.2010474121427,0.0068598642396664,
0.0101333483495882));
#40155=CARTESIAN_POINT('Ctrl Pts',(-0.201076578870104,0.0072242446465652,
0.0101523770736324));
#40156=CARTESIAN_POINT('Ctrl Pts',(-0.201099819882141,0.00749914619770346,
0.0101529062582246));
#40157=CARTESIAN_POINT('',(-0.201177053601335,0.0122550060276839,0.00884070721774072));
#40158=CARTESIAN_POINT('Ctrl Pts',(-0.201099415026176,0.00749913299764412,
0.0101528974791025));
#40159=CARTESIAN_POINT('Ctrl Pts',(-0.201096555619577,0.00753150741933934,
0.0101528385065419));
#40160=CARTESIAN_POINT('Ctrl Pts',(-0.201093736994948,0.00756388495100858,
0.0101526106398872));
#40161=CARTESIAN_POINT('Ctrl Pts',(-0.201087666450416,0.00763453987982649,
0.0101517444674804));
#40162=CARTESIAN_POINT('Ctrl Pts',(-0.201084429222973,0.00767281663265906,
0.010151038985735));
#40163=CARTESIAN_POINT('Ctrl Pts',(-0.201080801334986,0.0077163098527908,
0.0101499685939465));
#40164=CARTESIAN_POINT('Ctrl Pts',(-0.201080366927711,0.00772152768394031,
0.0101498357845174));
#40165=CARTESIAN_POINT('Ctrl Pts',(-0.201079462914577,0.00773240637854102,
0.0101495497227957));
#40166=CARTESIAN_POINT('Ctrl Pts',(-0.201078993452857,0.0077380672302977,
0.0101493956923408));
#40167=CARTESIAN_POINT('Ctrl Pts',(-0.201077400593704,0.00775731229740116,
0.0101488544418675));
#40168=CARTESIAN_POINT('Ctrl Pts',(-0.201076281646611,0.00777089616598205,
0.0101484426009006));
#40169=CARTESIAN_POINT('Ctrl Pts',(-0.201071551307129,0.00782858173595134,
0.0101465670310501));
#40170=CARTESIAN_POINT('Ctrl Pts',(-0.201067988458377,0.007872677626471,
0.0101448189497164));
#40171=CARTESIAN_POINT('Ctrl Pts',(-0.201053871077008,0.00804952410981167,
0.010136545542321));
#40172=CARTESIAN_POINT('Ctrl Pts',(-0.201043541456728,0.0081825036848605,
0.0101274548226958));
#40173=CARTESIAN_POINT('Ctrl Pts',(-0.201032352560321,0.00833284176583748,
0.0101139327363592));
#40174=CARTESIAN_POINT('Ctrl Pts',(-0.201031018431873,0.00835090027672925,
0.0101122552185723));
#40175=CARTESIAN_POINT('Ctrl Pts',(-0.201022652850357,0.00846509755040904,
0.0101013102262794));
#40176=CARTESIAN_POINT('Ctrl Pts',(-0.201015937700995,0.00856111993260325,
0.0100905968298343));
#40177=CARTESIAN_POINT('Ctrl Pts',(-0.201001522417578,0.00878472981437558,
0.0100621250456051));
#40178=CARTESIAN_POINT('Ctrl Pts',(-0.200994315161741,0.00891158178381539,
0.0100433010725122));
#40179=CARTESIAN_POINT('Ctrl Pts',(-0.200984966053877,0.00910857513732452,
0.0100099106717903));
#40180=CARTESIAN_POINT('Ctrl Pts',(-0.200982001710847,0.00917864056758256,
0.00999721021346039));
#40181=CARTESIAN_POINT('Ctrl Pts',(-0.200976604379606,0.00932560861946987,
0.00996883327826301));
#40182=CARTESIAN_POINT('Ctrl Pts',(-0.200974256328178,0.00940247516841393,
0.00995298677241071));
#40183=CARTESIAN_POINT('Ctrl Pts',(-0.200968526789994,0.00964294760988883,
0.0099002516080076));
#40184=CARTESIAN_POINT('Ctrl Pts',(-0.200967003526247,0.00980579664254104,
0.00985992759696585));
#40185=CARTESIAN_POINT('Ctrl Pts',(-0.20096903863634,0.0100680083654313,
0.00978748245514171));
#40186=CARTESIAN_POINT('Ctrl Pts',(-0.200970898955289,0.0101677912935188,
0.00975811362521028));
#40187=CARTESIAN_POINT('Ctrl Pts',(-0.200979011841939,0.0104409498990722,
0.00967275625057537));
#40188=CARTESIAN_POINT('Ctrl Pts',(-0.200987498960234,0.0106129719117605,
0.00961344672677827));
#40189=CARTESIAN_POINT('Ctrl Pts',(-0.201017172577816,0.0110403688905056,
0.00945204240146106));
#40190=CARTESIAN_POINT('Ctrl Pts',(-0.201042813248034,0.0112880111477272,
0.00934589777805525));
#40191=CARTESIAN_POINT('Ctrl Pts',(-0.201075293812801,0.0115421151804829,
0.00922361425713881));
#40192=CARTESIAN_POINT('Ctrl Pts',(-0.201076280881285,0.011549797704654,
0.00921990414749716));
#40193=CARTESIAN_POINT('Ctrl Pts',(-0.201079194491396,0.011572363930971,
0.00920896798108764));
#40194=CARTESIAN_POINT('Ctrl Pts',(-0.201081132455913,0.0115872323483612,
0.00920171333031922));
#40195=CARTESIAN_POINT('Ctrl Pts',(-0.201097568219318,0.0117122511540107,
0.00914030016243677));
#40196=CARTESIAN_POINT('Ctrl Pts',(-0.201112835939432,0.0118218912000811,
0.00908371368776426));
#40197=CARTESIAN_POINT('Ctrl Pts',(-0.201133528613954,0.011965820847289,
0.00900576141837299));
#40198=CARTESIAN_POINT('Ctrl Pts',(-0.201138749565774,0.0120016723198076,
0.00898603600794796));
#40199=CARTESIAN_POINT('Ctrl Pts',(-0.201147172122991,0.0120587248794593,
0.00895415204620798));
#40200=CARTESIAN_POINT('Ctrl Pts',(-0.201150340696306,0.0120800145739369,
0.0089421434805461));
#40201=CARTESIAN_POINT('Ctrl Pts',(-0.201155474346223,0.0121142184060044,
0.00892267196211884));
#40202=CARTESIAN_POINT('Ctrl Pts',(-0.201157427314594,0.0121271638790092,
0.00891526094768469));
#40203=CARTESIAN_POINT('Ctrl Pts',(-0.201159756324221,0.0121425212968394,
0.0089064198753503));
#40204=CARTESIAN_POINT('Ctrl Pts',(-0.20116012521612,0.0121449513662034,
0.00890501944645919));
#40205=CARTESIAN_POINT('Ctrl Pts',(-0.201165961618878,0.0121833606018225,
0.00888286129962451));
#40206=CARTESIAN_POINT('Ctrl Pts',(-0.201171486576948,0.0122191939011565,
0.00886186694378061));
#40207=CARTESIAN_POINT('Ctrl Pts',(-0.201177074329032,0.0122548777933217,
0.00884063698486466));
#40208=CARTESIAN_POINT('',(-0.202178357934375,0.0122547990652915,0.00886239654148025));
#40209=CARTESIAN_POINT('Ctrl Pts',(-0.201177075042786,0.0122548774470157,
0.00884063720755112));
#40210=CARTESIAN_POINT('Ctrl Pts',(-0.201513398686541,0.0122548513903108,
0.00884794584758545));
#40211=CARTESIAN_POINT('Ctrl Pts',(-0.201847382617857,0.0122548298057659,
0.00885520107578513));
#40212=CARTESIAN_POINT('Ctrl Pts',(-0.202178423329881,0.0122548125338768,
0.00886238990093067));
#40213=CARTESIAN_POINT('',(-0.20209947962974,0.0074995037887144,0.0101745804416663));
#40214=CARTESIAN_POINT('Ctrl Pts',(-0.202178357934375,0.0122547990652915,
0.00886239654148025));
#40215=CARTESIAN_POINT('Ctrl Pts',(-0.202141594099432,0.0120170628854501,
0.0090038431709906));
#40216=CARTESIAN_POINT('Ctrl Pts',(-0.202096005540814,0.0116999888925394,
0.0091720983007729));
#40217=CARTESIAN_POINT('Ctrl Pts',(-0.202051299589304,0.0113413832046676,
0.00934019418830925));
#40218=CARTESIAN_POINT('Ctrl Pts',(-0.202030922651275,0.0111631559854859,
0.00941915423537262));
#40219=CARTESIAN_POINT('Ctrl Pts',(-0.202002813441514,0.0108513628693672,
0.00954689664555636));
#40220=CARTESIAN_POINT('Ctrl Pts',(-0.201978982212522,0.0104745530127929,
0.00968535788947888));
#40221=CARTESIAN_POINT('Ctrl Pts',(-0.201964231695163,0.00995451013132065,
0.00984735855643358));
#40222=CARTESIAN_POINT('Ctrl Pts',(-0.201970487645389,0.00949571672073084,
0.00995827983118732));
#40223=CARTESIAN_POINT('Ctrl Pts',(-0.20198422225347,0.00912548553395714,
0.0100293214390935));
#40224=CARTESIAN_POINT('Ctrl Pts',(-0.201994298073442,0.0089183090129626,
0.01006364374664));
#40225=CARTESIAN_POINT('Ctrl Pts',(-0.202004853442309,0.00873340615709544,
0.0100903924612634));
#40226=CARTESIAN_POINT('Ctrl Pts',(-0.202010564769062,0.00864432102944395,
0.0101018364537206));
#40227=CARTESIAN_POINT('Ctrl Pts',(-0.202022184353771,0.0084708735187532,
0.0101226862224682));
#40228=CARTESIAN_POINT('Ctrl Pts',(-0.202046363769246,0.00814074718404573,
0.0101549882276266));
#40229=CARTESIAN_POINT('Ctrl Pts',(-0.202075916750842,0.00777532058791057,
0.0101740844248864));
#40230=CARTESIAN_POINT('Ctrl Pts',(-0.202099479627945,0.00749950405175959,
0.0101745804416416));
#40231=CARTESIAN_POINT('',(-0.202180663785047,0.00274072929799762,0.0088597653691895));
#40232=CARTESIAN_POINT('Ctrl Pts',(-0.20209947962974,0.0074995037887144,
0.0101745804416663));
#40233=CARTESIAN_POINT('Ctrl Pts',(-0.202076131298968,0.00722392201477745,
0.0101740593562675));
#40234=CARTESIAN_POINT('Ctrl Pts',(-0.20204684427521,0.00685873434784241,
0.0101549564340284));
#40235=CARTESIAN_POINT('Ctrl Pts',(-0.202022880675394,0.00652881578934848,
0.0101226689516121));
#40236=CARTESIAN_POINT('Ctrl Pts',(-0.202011355028604,0.00635531779374554,
0.010101806581237));
#40237=CARTESIAN_POINT('Ctrl Pts',(-0.202005706364736,0.00626652087781374,
0.0100904032799156));
#40238=CARTESIAN_POINT('Ctrl Pts',(-0.201995177744416,0.00608055260618936,
0.0100634924125636));
#40239=CARTESIAN_POINT('Ctrl Pts',(-0.201985156071195,0.00587249572156429,
0.0100289878141918));
#40240=CARTESIAN_POINT('Ctrl Pts',(-0.201971520984681,0.00550072819479208,
0.00995755927342406));
#40241=CARTESIAN_POINT('Ctrl Pts',(-0.20196544994584,0.00503969878565304,
0.00984581157874883));
#40242=CARTESIAN_POINT('Ctrl Pts',(-0.201980400836738,0.00452026663623846,
0.00968362153215009));
#40243=CARTESIAN_POINT('Ctrl Pts',(-0.202004357630176,0.00414366225519954,
0.00954499266392052));
#40244=CARTESIAN_POINT('Ctrl Pts',(-0.202032546032405,0.00383236089516692,
0.00941725161945248));
#40245=CARTESIAN_POINT('Ctrl Pts',(-0.202053003952958,0.00365417172245642,
0.00933820187402095));
#40246=CARTESIAN_POINT('Ctrl Pts',(-0.202097905643997,0.00329565767648496,
0.00916992114684366));
#40247=CARTESIAN_POINT('Ctrl Pts',(-0.202143715934825,0.00297852659698653,
0.0090014268340662));
#40248=CARTESIAN_POINT('Ctrl Pts',(-0.202180663785047,0.00274072929799762,
0.0088597653691895));
#40249=CARTESIAN_POINT('Ctrl Pts',(-0.202180730245087,0.00274072081434495,
0.00885976172744631));
#40250=CARTESIAN_POINT('Ctrl Pts',(-0.201847614367768,0.002740642783753,
0.00885249354413258));
#40251=CARTESIAN_POINT('Ctrl Pts',(-0.201514127092812,0.00274056060342704,
0.00884521482192548));
#40252=CARTESIAN_POINT('Ctrl Pts',(-0.201180516431429,0.00274047431825838,
0.00883793096370741));
#40253=CARTESIAN_POINT('Origin',(-0.199568033794847,0.00749999923595005,
0.000819344953990154));
#40254=CARTESIAN_POINT('',(-0.1991008326205,0.00749816128270665,0.0101077386020297));
#40255=CARTESIAN_POINT('',(-0.199179696503545,0.00273822610415434,0.00879699955640872));
#40256=CARTESIAN_POINT('Ctrl Pts',(-0.199179696503545,0.00273822610415434,
0.00879699955640872));
#40257=CARTESIAN_POINT('Ctrl Pts',(-0.199143244354989,0.00297491563473041,
0.00893740460207546));
#40258=CARTESIAN_POINT('Ctrl Pts',(-0.199098034288274,0.00329043121711526,
0.00910449277330028));
#40259=CARTESIAN_POINT('Ctrl Pts',(-0.199053629766553,0.00364764361753438,
0.00927172156032095));
#40260=CARTESIAN_POINT('Ctrl Pts',(-0.199033441682036,0.00382433767861057,
0.00934997449065479));
#40261=CARTESIAN_POINT('Ctrl Pts',(-0.199005233009131,0.0041375930335457,
0.00947827794999704));
#40262=CARTESIAN_POINT('Ctrl Pts',(-0.198981402060209,0.00451576736201145,
0.00961718934348785));
#40263=CARTESIAN_POINT('Ctrl Pts',(-0.198966678315752,0.0050396146973732,
0.00978024084154024));
#40264=CARTESIAN_POINT('Ctrl Pts',(-0.198973006624955,0.00549995157901586,
0.00989136011088092));
#40265=CARTESIAN_POINT('Ctrl Pts',(-0.198986778545821,0.00587279695417407,
0.00996274653281332));
#40266=CARTESIAN_POINT('Ctrl Pts',(-0.198996863774921,0.00608136231939041,
0.00999719312649999));
#40267=CARTESIAN_POINT('Ctrl Pts',(-0.199007457649552,0.00626811792143402,
0.0100240914954152));
#40268=CARTESIAN_POINT('Ctrl Pts',(-0.199013083248747,0.00635648831399133,
0.0100353799134243));
#40269=CARTESIAN_POINT('Ctrl Pts',(-0.199024590483033,0.00652977437477116,
0.0100561209067557));
#40270=CARTESIAN_POINT('Ctrl Pts',(-0.199048467492299,0.00685894990481282,
0.0100881861616881));
#40271=CARTESIAN_POINT('Ctrl Pts',(-0.199077613823705,0.00722329121805871,
0.0101071812274239));
#40272=CARTESIAN_POINT('Ctrl Pts',(-0.1991008326205,0.00749816128270665,
0.0101077386020297));
#40273=CARTESIAN_POINT('',(-0.199174846040548,0.0122573379664025,0.00879984889793131));
#40274=CARTESIAN_POINT('Ctrl Pts',(-0.199100423117724,0.00749814796091967,
0.0101077297270977));
#40275=CARTESIAN_POINT('Ctrl Pts',(-0.19909756555931,0.0075305462084152,
0.0101076742637468));
#40276=CARTESIAN_POINT('Ctrl Pts',(-0.199094748669567,0.00756294756525031,
0.0101074502765084));
#40277=CARTESIAN_POINT('Ctrl Pts',(-0.199088680122758,0.00763367215169112,
0.0101065931641555));
#40278=CARTESIAN_POINT('Ctrl Pts',(-0.199085443155413,0.00767199473866375,
0.0101058927930515));
#40279=CARTESIAN_POINT('Ctrl Pts',(-0.199081815402933,0.0077155398050165,
0.0101048285564554));
#40280=CARTESIAN_POINT('Ctrl Pts',(-0.199081381028702,0.00772076361829315,
0.0101046964973235));
#40281=CARTESIAN_POINT('Ctrl Pts',(-0.199080477068572,0.00773165489864521,
0.0101044120095616));
#40282=CARTESIAN_POINT('Ctrl Pts',(-0.199080007626291,0.0077373223541118,
0.0101042588036328));
#40283=CARTESIAN_POINT('Ctrl Pts',(-0.199078414782293,0.00775659033516524,
0.0101037203668784));
#40284=CARTESIAN_POINT('Ctrl Pts',(-0.199077295813301,0.00777019051735651,
0.0101033105458919));
#40285=CARTESIAN_POINT('Ctrl Pts',(-0.199072564471858,0.00782795529984388,
0.010101443394002));
#40286=CARTESIAN_POINT('Ctrl Pts',(-0.199069000449091,0.00787211412832768,
0.0100997019290571));
#40287=CARTESIAN_POINT('Ctrl Pts',(-0.199054876294354,0.00804922540293602,
0.0100914555228068));
#40288=CARTESIAN_POINT('Ctrl Pts',(-0.19904453897387,0.00818240784315175,
0.0100823868562197));
#40289=CARTESIAN_POINT('Ctrl Pts',(-0.199033337016503,0.00833297925678125,
0.0100688913142093));
#40290=CARTESIAN_POINT('Ctrl Pts',(-0.199032001445838,0.00835106298428525,
0.0100672172864517));
#40291=CARTESIAN_POINT('Ctrl Pts',(-0.199023626091707,0.00846542043988094,
0.0100562946091264));
#40292=CARTESIAN_POINT('Ctrl Pts',(-0.199016899990595,0.00856157817146482,
0.0100456013004476));
#40293=CARTESIAN_POINT('Ctrl Pts',(-0.199002448107951,0.00878551065801579,
0.0100171786105707));
#40294=CARTESIAN_POINT('Ctrl Pts',(-0.198995210202229,0.00891256346882149,
0.00999838210039725));
#40295=CARTESIAN_POINT('Ctrl Pts',(-0.19898579937427,0.00910984027578994,
0.00996504196596855));
#40296=CARTESIAN_POINT('Ctrl Pts',(-0.198982810425363,0.00917999713999155,
0.00995236200383042));
#40297=CARTESIAN_POINT('Ctrl Pts',(-0.198977354128857,0.00932718349070731,
0.00992402518089048));
#40298=CARTESIAN_POINT('Ctrl Pts',(-0.198974971381639,0.00940417699397456,
0.00990819783379226));
#40299=CARTESIAN_POINT('Ctrl Pts',(-0.198969144880626,0.00964414837341371,
0.00985572112873346));
#40300=CARTESIAN_POINT('Ctrl Pts',(-0.198967522050789,0.00980638347769885,
0.00981568579315269));
#40301=CARTESIAN_POINT('Ctrl Pts',(-0.198969324601282,0.0100680598402537,
0.00974366898222702));
#40302=CARTESIAN_POINT('Ctrl Pts',(-0.198971089194015,0.0101679091427984,
0.0097143946132173));
#40303=CARTESIAN_POINT('Ctrl Pts',(-0.198978917886141,0.010441256588431,
0.00962930961412696));
#40304=CARTESIAN_POINT('Ctrl Pts',(-0.198987201313106,0.0106134127355314,
0.0095701851250402));
#40305=CARTESIAN_POINT('Ctrl Pts',(-0.199016321440205,0.0110411790868304,
0.00940927412525473));
#40306=CARTESIAN_POINT('Ctrl Pts',(-0.199041597438575,0.0112890619670433,
0.00930344946960165));
#40307=CARTESIAN_POINT('Ctrl Pts',(-0.19907660436805,0.0115666451139836,
0.00917040760605046));
#40308=CARTESIAN_POINT('Ctrl Pts',(-0.199080566717778,0.0115974228045342,
0.00915544770808169));
#40309=CARTESIAN_POINT('Ctrl Pts',(-0.199098466915732,0.0117341340684825,
0.00908806532924535));
#40310=CARTESIAN_POINT('Ctrl Pts',(-0.199113021702264,0.0118396876158331,
0.00903351829961953));
#40311=CARTESIAN_POINT('Ctrl Pts',(-0.199132696289241,0.0119779176994999,
0.0089587005678997));
#40312=CARTESIAN_POINT('Ctrl Pts',(-0.199137603313996,0.0120119720702286,
0.00893999160482358));
#40313=CARTESIAN_POINT('Ctrl Pts',(-0.199145564734414,0.0120665080077619,
0.00890958426378745));
#40314=CARTESIAN_POINT('Ctrl Pts',(-0.19914858987286,0.01208706755771,0.00889801824544057));
#40315=CARTESIAN_POINT('Ctrl Pts',(-0.199155380000627,0.0121328394308257,
0.00887203916099361));
#40316=CARTESIAN_POINT('Ctrl Pts',(-0.199159154233648,0.0121580277333056,
0.00885758650169327));
#40317=CARTESIAN_POINT('Ctrl Pts',(-0.199166705696621,0.0122079000416094,
0.00882865950851265));
#40318=CARTESIAN_POINT('Ctrl Pts',(-0.19917048206159,0.0122325858177661,
0.00881418863909818));
#40319=CARTESIAN_POINT('Ctrl Pts',(-0.199174288103971,0.0122572011081367,
0.00879960620353417));
#40320=CARTESIAN_POINT('',(-0.200176262520899,0.012256855145248,0.0088215241666907));
#40321=CARTESIAN_POINT('Ctrl Pts',(-0.199174569563385,0.0122572006783931,
0.00879961255852584));
#40322=CARTESIAN_POINT('Ctrl Pts',(-0.199508459486052,0.0122570856871889,
0.00880691615277684));
#40323=CARTESIAN_POINT('Ctrl Pts',(-0.199842448484061,0.0122569750175065,
0.0088142193158282));
#40324=CARTESIAN_POINT('Ctrl Pts',(-0.200176327292855,0.012256868740326,
0.00882151747157252));
#40325=CARTESIAN_POINT('',(-0.200100338986871,0.00749890820710971,0.0101293940320589));
#40326=CARTESIAN_POINT('Ctrl Pts',(-0.200176262520899,0.012256855145248,
0.0088215241666907));
#40327=CARTESIAN_POINT('Ctrl Pts',(-0.200139848831246,0.0120187427182138,
0.00896257979280764));
#40328=CARTESIAN_POINT('Ctrl Pts',(-0.200094704254856,0.0117012524516469,
0.0091303434798315));
#40329=CARTESIAN_POINT('Ctrl Pts',(-0.20005045695783,0.0113422735683314,
0.00929792076866446));
#40330=CARTESIAN_POINT('Ctrl Pts',(-0.200030300865821,0.0111639202596685,
0.00937661504422539));
#40331=CARTESIAN_POINT('Ctrl Pts',(-0.200002516361759,0.0108518407830771,
0.00950396043743957));
#40332=CARTESIAN_POINT('Ctrl Pts',(-0.199979012211579,0.0104747794652236,
0.00964195956351153));
#40333=CARTESIAN_POINT('Ctrl Pts',(-0.199964586451688,0.00995464152162186,
0.00980336058488574));
#40334=CARTESIAN_POINT('Ctrl Pts',(-0.199971015201619,0.00949550037894515,
0.00991393870179615));
#40335=CARTESIAN_POINT('Ctrl Pts',(-0.199984854194566,0.0091251855923606,
0.00998471643871501));
#40336=CARTESIAN_POINT('Ctrl Pts',(-0.199994977020821,0.00891797369328077,
0.0100189096450406));
#40337=CARTESIAN_POINT('Ctrl Pts',(-0.20000556647705,0.00873306695781704,
0.0100455533980267));
#40338=CARTESIAN_POINT('Ctrl Pts',(-0.200011293457012,0.00864395082942657,
0.0100569561025451));
#40339=CARTESIAN_POINT('Ctrl Pts',(-0.200022940128602,0.00847046801670082,
0.0100777265959388));
#40340=CARTESIAN_POINT('Ctrl Pts',(-0.200047163314547,0.00814026979588536,
0.0101099034239855));
#40341=CARTESIAN_POINT('Ctrl Pts',(-0.200076753172813,0.00777477572470487,
0.0101289155097155));
#40342=CARTESIAN_POINT('Ctrl Pts',(-0.200100338983303,0.0074989084716685,
0.0101293940320128));
#40343=CARTESIAN_POINT('',(-0.200180004805387,0.00273845846940322,0.00881880778057919));
#40344=CARTESIAN_POINT('Ctrl Pts',(-0.200100338986871,0.00749890820710971,
0.0101293940320589));
#40345=CARTESIAN_POINT('Ctrl Pts',(-0.200077055880268,0.007223317195962,
0.0101288571167368));
#40346=CARTESIAN_POINT('Ctrl Pts',(-0.200047843901506,0.00685811476510037,
0.0101097990374615));
#40347=CARTESIAN_POINT('Ctrl Pts',(-0.200023930105906,0.00652817936751469,
0.0100776062887231));
#40348=CARTESIAN_POINT('Ctrl Pts',(-0.200012422102254,0.006354660368642,
0.0100568059955802));
#40349=CARTESIAN_POINT('Ctrl Pts',(-0.200006781974207,0.0062658760601037,
0.0100454406027125));
#40350=CARTESIAN_POINT('Ctrl Pts',(-0.199996254518662,0.00607981053317545,
0.010018601506999));
#40351=CARTESIAN_POINT('Ctrl Pts',(-0.199986224309984,0.00587169694792907,
0.00998419872280633));
#40352=CARTESIAN_POINT('Ctrl Pts',(-0.199972547223942,0.00549983639015558,
0.009912982695534));
#40353=CARTESIAN_POINT('Ctrl Pts',(-0.199966345220014,0.00503915807743746,
0.00980171648677967));
#40354=CARTESIAN_POINT('Ctrl Pts',(-0.199981045250382,0.00451916422140907,
0.0096399511092111));
#40355=CARTESIAN_POINT('Ctrl Pts',(-0.200004772849193,0.00414244958212928,
0.0095017911578116));
#40356=CARTESIAN_POINT('Ctrl Pts',(-0.200032732117133,0.00383113331162465,
0.00937453733845435));
#40357=CARTESIAN_POINT('Ctrl Pts',(-0.200053059983703,0.00365281023225859,
0.00929574219517862));
#40358=CARTESIAN_POINT('Ctrl Pts',(-0.200097690354166,0.00329403452386807,
0.00912801389820296));
#40359=CARTESIAN_POINT('Ctrl Pts',(-0.200143251201405,0.00297656720641742,
0.00896004372071677));
#40360=CARTESIAN_POINT('Ctrl Pts',(-0.200180004805387,0.00273845846940322,
0.00881880778057919));
#40361=CARTESIAN_POINT('Ctrl Pts',(-0.200180071690563,0.00273844985852019,
0.00881880409310063));
#40362=CARTESIAN_POINT('Ctrl Pts',(-0.199847123138668,0.00273837907375333,
0.00881154922699135));
#40363=CARTESIAN_POINT('Ctrl Pts',(-0.199513602268475,0.00273830396530483,
0.00880427938248978));
#40364=CARTESIAN_POINT('Ctrl Pts',(-0.199179786681636,0.00273822456479632,
0.00879700059164244));
#40365=CARTESIAN_POINT('Origin',(-0.19756813490279,0.0074999991336252,0.000739267166499619));
#40366=CARTESIAN_POINT('',(-0.197101856029946,0.00749734564313153,0.0100625711830282));
#40367=CARTESIAN_POINT('',(-0.197178881546705,0.00273601310122549,0.00875618433461763));
#40368=CARTESIAN_POINT('Ctrl Pts',(-0.197178881546705,0.00273601310122549,
0.00875618433461763));
#40369=CARTESIAN_POINT('Ctrl Pts',(-0.197142626964537,0.00297299673492067,
0.00889614308672296));
#40370=CARTESIAN_POINT('Ctrl Pts',(-0.197097670535042,0.00328882261774284,
0.00906268248965719));
#40371=CARTESIAN_POINT('Ctrl Pts',(-0.197053541172525,0.00364627238000341,
0.00922933666434974));
#40372=CARTESIAN_POINT('Ctrl Pts',(-0.197033485692237,0.00382307290229682,
0.00930731998477126));
#40373=CARTESIAN_POINT('Ctrl Pts',(-0.197005506268391,0.00413636603733711,
0.00943513380611822));
#40374=CARTESIAN_POINT('Ctrl Pts',(-0.196981909916078,0.00451463585616606,
0.00957355710978556));
#40375=CARTESIAN_POINT('Ctrl Pts',(-0.196967449184374,0.00503887642033483,
0.00973612429519158));
#40376=CARTESIAN_POINT('Ctrl Pts',(-0.196973930017077,0.00549897094200798,
0.00984679224998308));
#40377=CARTESIAN_POINT('Ctrl Pts',(-0.196987776644517,0.00587186549873816,
0.00991795678216301));
#40378=CARTESIAN_POINT('Ctrl Pts',(-0.19699789164315,0.00608045844290354,
0.0099522983150153));
#40379=CARTESIAN_POINT('Ctrl Pts',(-0.197008505217262,0.00626727125993394,
0.00997912139989793));
#40380=CARTESIAN_POINT('Ctrl Pts',(-0.197014133781209,0.00635562038557536,
0.00999037271097673));
#40381=CARTESIAN_POINT('Ctrl Pts',(-0.197025646063537,0.00652890076404714,
0.0100110519118934));
#40382=CARTESIAN_POINT('Ctrl Pts',(-0.197049522384861,0.00685808246893175,
0.0100430297163264));
#40383=CARTESIAN_POINT('Ctrl Pts',(-0.197078653753898,0.00722244105207463,
0.0100619906974236));
#40384=CARTESIAN_POINT('Ctrl Pts',(-0.197101856530647,0.00749734560084308,
0.0100625711961792));
#40385=CARTESIAN_POINT('',(-0.197176217067543,0.0122591131058223,0.00875901669782422));
#40386=CARTESIAN_POINT('Ctrl Pts',(-0.19710185655348,0.00749734587138656,
0.0100625711967505));
#40387=CARTESIAN_POINT('Ctrl Pts',(-0.197078523516818,0.00777162104014169,
0.0100621439902365));
#40388=CARTESIAN_POINT('Ctrl Pts',(-0.197049199366131,0.00813529702223795,
0.0100434664523806));
#40389=CARTESIAN_POINT('Ctrl Pts',(-0.197025114401905,0.00846412790914781,
0.0100117657915565));
#40390=CARTESIAN_POINT('Ctrl Pts',(-0.197013477905477,0.00863733646442351,
0.00999122542111019));
#40391=CARTESIAN_POINT('Ctrl Pts',(-0.197007781021792,0.00872568364978063,
0.00998004160952768));
#40392=CARTESIAN_POINT('Ctrl Pts',(-0.196997012427155,0.00891259409020632,
0.00995334571824261));
#40393=CARTESIAN_POINT('Ctrl Pts',(-0.19698672575335,0.00912127329859086,
0.00991914668186268));
#40394=CARTESIAN_POINT('Ctrl Pts',(-0.1969725724387,0.00949430522202776,
0.00984823772706428));
#40395=CARTESIAN_POINT('Ctrl Pts',(-0.196965699496595,0.00995460126870586,
0.0097378606524851));
#40396=CARTESIAN_POINT('Ctrl Pts',(-0.196979759716268,0.010478671284573,
0.00957576289904584));
#40397=CARTESIAN_POINT('Ctrl Pts',(-0.197003135124178,0.0108570185538505,
0.00943763320894697));
#40398=CARTESIAN_POINT('Ctrl Pts',(-0.197030958275967,0.0111703409896189,
0.00931008407709414));
#40399=CARTESIAN_POINT('Ctrl Pts',(-0.197050972536751,0.011347427828458,
0.00923213571472623));
#40400=CARTESIAN_POINT('Ctrl Pts',(-0.197095032095316,0.0117053572034986,
0.00906557221068337));
#40401=CARTESIAN_POINT('Ctrl Pts',(-0.197139967387252,0.0120217156630974,
0.00889902627611354));
#40402=CARTESIAN_POINT('Ctrl Pts',(-0.197176217067543,0.0122591131058223,
0.00875901669782422));
#40403=CARTESIAN_POINT('',(-0.198173992730521,0.0122590030744015,0.00878068750897002));
#40404=CARTESIAN_POINT('Ctrl Pts',(-0.197176307469774,0.012259110245449,
0.00875902035178441));
#40405=CARTESIAN_POINT('Ctrl Pts',(-0.197510848228027,0.0122590743715548,
0.00876628567977086));
#40406=CARTESIAN_POINT('Ctrl Pts',(-0.19784360274998,0.0122590432302266,
0.0087735095219768));
#40407=CARTESIAN_POINT('Ctrl Pts',(-0.198174057214716,0.012259016706353,
0.00878068082077123));
#40408=CARTESIAN_POINT('',(-0.198101353816547,0.00749782534027133,0.0100842108241173));
#40409=CARTESIAN_POINT('Ctrl Pts',(-0.198173992730521,0.0122590030744015,
0.00878068750897002));
#40410=CARTESIAN_POINT('Ctrl Pts',(-0.198138004888705,0.0120204746132674,
0.00892136889022891));
#40411=CARTESIAN_POINT('Ctrl Pts',(-0.198093401335538,0.0117025124533415,
0.00908865958938337));
#40412=CARTESIAN_POINT('Ctrl Pts',(-0.198049719256268,0.0113431216479256,
0.00925572482570341));
#40413=CARTESIAN_POINT('Ctrl Pts',(-0.198029831826993,0.0111645836672768,
0.00933417156341316));
#40414=CARTESIAN_POINT('Ctrl Pts',(-0.198002470389522,0.0108523209073434,
0.00946106760549989));
#40415=CARTESIAN_POINT('Ctrl Pts',(-0.197979387062072,0.0104750174531497,
0.00959859870239481));
#40416=CARTESIAN_POINT('Ctrl Pts',(-0.197965389781622,0.00995446908941076,
0.00975947656779084));
#40417=CARTESIAN_POINT('Ctrl Pts',(-0.197972030645853,0.00949520601411241,
0.00986963753715952));
#40418=CARTESIAN_POINT('Ctrl Pts',(-0.19798596221564,0.00912470398287173,
0.00994016293552026));
#40419=CARTESIAN_POINT('Ctrl Pts',(-0.197996115677719,0.00891738945160544,
0.00997423054978755));
#40420=CARTESIAN_POINT('Ctrl Pts',(-0.198006719249522,0.00873237689330112,
0.0100007756142138));
#40421=CARTESIAN_POINT('Ctrl Pts',(-0.198012445790112,0.00864323678034072,
0.0100121312968828));
#40422=CARTESIAN_POINT('Ctrl Pts',(-0.1980240882512,0.00846968835882415,
0.0100328176107757));
#40423=CARTESIAN_POINT('Ctrl Pts',(-0.198048284245988,0.00813937985693941,
0.0100648555245894));
#40424=CARTESIAN_POINT('Ctrl Pts',(-0.198077819417979,0.00777377379615927,
0.0100837657093142));
#40425=CARTESIAN_POINT('Ctrl Pts',(-0.198101353812703,0.00749782560887336,
0.0100842108240968));
#40426=CARTESIAN_POINT('',(-0.198179277467544,0.00273626767412241,0.00877799114281851));
#40427=CARTESIAN_POINT('Ctrl Pts',(-0.198101353816547,0.00749782534027133,
0.0100842108241173));
#40428=CARTESIAN_POINT('Ctrl Pts',(-0.198078088183822,0.00722225737258161,
0.0100836427809772));
#40429=CARTESIAN_POINT('Ctrl Pts',(-0.198048890875069,0.00685708620871131,
0.0100646149235419));
#40430=CARTESIAN_POINT('Ctrl Pts',(-0.19802497722664,0.00652717554366646,
0.0100325082639782));
#40431=CARTESIAN_POINT('Ctrl Pts',(-0.19801346332886,0.00635366308942737,
0.0100117676259961));
#40432=CARTESIAN_POINT('Ctrl Pts',(-0.198007819566227,0.00626489379443579,
0.0100004373772158));
#40433=CARTESIAN_POINT('Ctrl Pts',(-0.197997274071363,0.00607879754285442,
0.00997367463662727));
#40434=CARTESIAN_POINT('Ctrl Pts',(-0.197987215946941,0.00587067685471771,
0.00993937790394548));
#40435=CARTESIAN_POINT('Ctrl Pts',(-0.197973468852053,0.00549880245195572,
0.00986838680752163));
#40436=CARTESIAN_POINT('Ctrl Pts',(-0.197967122562937,0.00503838759263585,
0.00975757572268468));
#40437=CARTESIAN_POINT('Ctrl Pts',(-0.197981576098232,0.0045180222909139,
0.00959629573797476));
#40438=CARTESIAN_POINT('Ctrl Pts',(-0.198005082771862,0.00414121672263879,
0.00945862266623302));
#40439=CARTESIAN_POINT('Ctrl Pts',(-0.198032826989652,0.00382985614807151,
0.00933185115640346));
#40440=CARTESIAN_POINT('Ctrl Pts',(-0.198053027382874,0.0036514357600232,
0.00925333145484234));
#40441=CARTESIAN_POINT('Ctrl Pts',(-0.198097395119529,0.00329243200436169,
0.00908618421763473));
#40442=CARTESIAN_POINT('Ctrl Pts',(-0.198142713099356,0.00297466421302015,
0.00891877230038998));
#40443=CARTESIAN_POINT('Ctrl Pts',(-0.198179277467544,0.00273626767412241,
0.00877799114281851));
#40444=CARTESIAN_POINT('Ctrl Pts',(-0.19817934460266,0.00273625896376666,
0.0087779874234125));
#40445=CARTESIAN_POINT('Ctrl Pts',(-0.197846274705172,0.00273618093672907,
0.00877073110479899));
#40446=CARTESIAN_POINT('Ctrl Pts',(-0.197512729366218,0.00273609845023171,
0.0087634618445431));
#40447=CARTESIAN_POINT('Ctrl Pts',(-0.197178972113877,0.00273601154455744,
0.00875618537063138));
#40448=CARTESIAN_POINT('Origin',(-0.195568703024637,0.00749999923833712,
0.000658360812067055));
#40449=CARTESIAN_POINT('',(-0.195102854699168,0.00749647351839117,0.0100174036757887));
#40450=CARTESIAN_POINT('',(-0.195178081382383,0.00273409965744036,0.00871564145407736));
#40451=CARTESIAN_POINT('Ctrl Pts',(-0.195178081382383,0.00273409965744036,
0.00871564145407736));
#40452=CARTESIAN_POINT('Ctrl Pts',(-0.195142003031606,0.00297137204920274,
0.00885512670497663));
#40453=CARTESIAN_POINT('Ctrl Pts',(-0.195097271567982,0.00328749493151492,
0.00902108304563917));
#40454=CARTESIAN_POINT('Ctrl Pts',(-0.195053379669963,0.00364518457110896,
0.00918713546639911));
#40455=CARTESIAN_POINT('Ctrl Pts',(-0.195033441180626,0.00382205047526963,
0.00926481961242654));
#40456=CARTESIAN_POINT('Ctrl Pts',(-0.195005638551936,0.00413551272222303,
0.009392175608848));
#40457=CARTESIAN_POINT('Ctrl Pts',(-0.194982225913951,0.00451392049931529,
0.00953009104539298));
#40458=CARTESIAN_POINT('Ctrl Pts',(-0.194967960467318,0.00503823275189329,
0.00969205034835313));
#40459=CARTESIAN_POINT('Ctrl Pts',(-0.194974562672158,0.00549844324011582,
0.00980233354848123));
#40460=CARTESIAN_POINT('Ctrl Pts',(-0.194988493479225,0.00587128826194149,
0.00987323309250545));
#40461=CARTESIAN_POINT('Ctrl Pts',(-0.194998650748219,0.00607983838954741,
0.0099074486869859));
#40462=CARTESIAN_POINT('Ctrl Pts',(-0.195009298503175,0.00626658803704918,
0.0099341733993258));
#40463=CARTESIAN_POINT('Ctrl Pts',(-0.195014943861307,0.00635493196350272,
0.00994538806277399));
#40464=CARTESIAN_POINT('Ctrl Pts',(-0.195026487338825,0.00652818220539433,
0.00996599834821625));
#40465=CARTESIAN_POINT('Ctrl Pts',(-0.195050420612355,0.00685731380746718,
0.0099978773710621));
#40466=CARTESIAN_POINT('Ctrl Pts',(-0.195079610558799,0.00722161145123598,
0.0100167973575665));
#40467=CARTESIAN_POINT('Ctrl Pts',(-0.195102855210816,0.00749647347509058,
0.0100174036899749));
#40468=CARTESIAN_POINT('',(-0.19517793622571,0.0122618594502722,0.00871802364175171));
#40469=CARTESIAN_POINT('Ctrl Pts',(-0.195102855229775,0.00749647369925886,
0.0100174036904694));
#40470=CARTESIAN_POINT('Ctrl Pts',(-0.195079650033701,0.0077708960107351,
0.0100170049335787));
#40471=CARTESIAN_POINT('Ctrl Pts',(-0.195050492730399,0.00813475203583469,
0.00999841538572308));
#40472=CARTESIAN_POINT('Ctrl Pts',(-0.195026555120156,0.00846373126034199,
0.0099668392959626));
#40473=CARTESIAN_POINT('Ctrl Pts',(-0.195014995306788,0.00863700065608847,
0.00994637890650517));
#40474=CARTESIAN_POINT('Ctrl Pts',(-0.195009336160461,0.00872539617663902,
0.00993523552157287));
#40475=CARTESIAN_POINT('Ctrl Pts',(-0.194998651227084,0.00891229649891521,
0.00990865196002218));
#40476=CARTESIAN_POINT('Ctrl Pts',(-0.194988450243687,0.0091210211909995,
0.00987458746983198));
#40477=CARTESIAN_POINT('Ctrl Pts',(-0.194974434565974,0.00949420365260338,
0.00980394105343129));
#40478=CARTESIAN_POINT('Ctrl Pts',(-0.194967699416777,0.00995492489130331,
0.0096939165698559));
#40479=CARTESIAN_POINT('Ctrl Pts',(-0.19498181283275,0.0104798102273614,
0.0095321912702417));
#40480=CARTESIAN_POINT('Ctrl Pts',(-0.195005149570046,0.0108583756108732,
0.00939450978445774));
#40481=CARTESIAN_POINT('Ctrl Pts',(-0.195032878840536,0.0111716458058373,
0.00926749369434052));
#40482=CARTESIAN_POINT('Ctrl Pts',(-0.195052857418986,0.0113489620203353,
0.00918976770636426));
#40483=CARTESIAN_POINT('Ctrl Pts',(-0.195096844479162,0.01170725645881,
0.00902372410857468));
#40484=CARTESIAN_POINT('Ctrl Pts',(-0.195141725801382,0.0120240670219162,
0.00885765266532079));
#40485=CARTESIAN_POINT('Ctrl Pts',(-0.19517793622571,0.0122618594502722,
0.00871802364175171));
#40486=CARTESIAN_POINT('',(-0.19617749360186,0.0122611495956684,0.00874007044956493));
#40487=CARTESIAN_POINT('Ctrl Pts',(-0.195178027888241,0.0122618562493937,
0.00871802751514387));
#40488=CARTESIAN_POINT('Ctrl Pts',(-0.195511176940293,0.0122616207531416,
0.0087253750077405));
#40489=CARTESIAN_POINT('Ctrl Pts',(-0.195844424120966,0.01226138980123,
0.00873272192611785));
#40490=CARTESIAN_POINT('Ctrl Pts',(-0.196177561574348,0.0122611635394136,
0.00874006368840159));
#40491=CARTESIAN_POINT('',(-0.19610247501614,0.00749683809102515,0.0100390300519628));
#40492=CARTESIAN_POINT('Ctrl Pts',(-0.19617749360186,0.0122611495956684,
0.00874007044956493));
#40493=CARTESIAN_POINT('Ctrl Pts',(-0.196141014853573,0.0120222633487051,
0.00888031100537719));
#40494=CARTESIAN_POINT('Ctrl Pts',(-0.19609580872818,0.0117038769497799,
0.00904706732867685));
#40495=CARTESIAN_POINT('Ctrl Pts',(-0.196051579746205,0.011344201623836,
0.00921353755448672));
#40496=CARTESIAN_POINT('Ctrl Pts',(-0.196031434794024,0.0111652973544448,
0.00929179681903197));
#40497=CARTESIAN_POINT('Ctrl Pts',(-0.196003872188682,0.0108536221626497,
0.00941792065964247));
#40498=CARTESIAN_POINT('Ctrl Pts',(-0.195980602663577,0.0104763472727013,
0.00955493379103075));
#40499=CARTESIAN_POINT('Ctrl Pts',(-0.195966554994754,0.00995393571634196,
0.00971572130618377));
#40500=CARTESIAN_POINT('Ctrl Pts',(-0.195973267353857,0.00949586692018786,
0.00982513937332992));
#40501=CARTESIAN_POINT('Ctrl Pts',(-0.195987224807208,0.00912487364769354,
0.00989550872314588));
#40502=CARTESIAN_POINT('Ctrl Pts',(-0.195997392390853,0.00891725362595259,
0.00992949377263191));
#40503=CARTESIAN_POINT('Ctrl Pts',(-0.196008014235276,0.00873175598500685,
0.00995599726309419));
#40504=CARTESIAN_POINT('Ctrl Pts',(-0.196013728479012,0.00864268846028022,
0.00996729220581992));
#40505=CARTESIAN_POINT('Ctrl Pts',(-0.196025358475374,0.00846903577183134,
0.009987901148687));
#40506=CARTESIAN_POINT('Ctrl Pts',(-0.196049514119745,0.00813862434607263,
0.0100198011636422));
#40507=CARTESIAN_POINT('Ctrl Pts',(-0.196078991315259,0.00777288071169348,
0.0100386152787338));
#40508=CARTESIAN_POINT('Ctrl Pts',(-0.19610247501614,0.00749683809102515,
0.0100390300519628));
#40509=CARTESIAN_POINT('',(-0.196178471694746,0.00273416910722515,0.00873732259680264));
#40510=CARTESIAN_POINT('Ctrl Pts',(-0.196102475015075,0.00749683779606065,
0.01003903005184));
#40511=CARTESIAN_POINT('Ctrl Pts',(-0.196079179883013,0.00722129154127866,
0.0100384329494739));
#40512=CARTESIAN_POINT('Ctrl Pts',(-0.196049938683409,0.00685615343993873,
0.010019439305117));
#40513=CARTESIAN_POINT('Ctrl Pts',(-0.196025978348201,0.00652626866424729,
0.00998742334664808));
#40514=CARTESIAN_POINT('Ctrl Pts',(-0.19601443718888,0.00635277195028409,
0.00996674647638142));
#40515=CARTESIAN_POINT('Ctrl Pts',(-0.196008778514743,0.00626400469010116,
0.00995545091588954));
#40516=CARTESIAN_POINT('Ctrl Pts',(-0.195998200063883,0.0060779436700094,
0.00992877795260165));
#40517=CARTESIAN_POINT('Ctrl Pts',(-0.195988099405926,0.00586985213365078,
0.00989459928016789));
#40518=CARTESIAN_POINT('Ctrl Pts',(-0.195974263559204,0.00549801481097926,
0.0098238581958861));
#40519=CARTESIAN_POINT('Ctrl Pts',(-0.195967774730541,0.00503764505177799,
0.00971346212967491));
#40520=CARTESIAN_POINT('Ctrl Pts',(-0.195982000966316,0.00451710683680645,
0.0095527459791788));
#40521=CARTESIAN_POINT('Ctrl Pts',(-0.19600530088904,0.00414017154598768,
0.00941556906216487));
#40522=CARTESIAN_POINT('Ctrl Pts',(-0.196032847971522,0.00382866522289246,
0.00928925272084666));
#40523=CARTESIAN_POINT('Ctrl Pts',(-0.19605292051857,0.00365017065488466,
0.0092110260323459));
#40524=CARTESIAN_POINT('Ctrl Pts',(-0.196097027755299,0.00329092584867731,
0.00904447216382486));
#40525=CARTESIAN_POINT('Ctrl Pts',(-0.196142099821149,0.00297285698814056,
0.00887763569320788));
#40526=CARTESIAN_POINT('Ctrl Pts',(-0.196178471694746,0.00273416910722515,
0.00873732259680264));
#40527=CARTESIAN_POINT('Ctrl Pts',(-0.196178538776777,0.00273416018332472,
0.0087373187725441));
#40528=CARTESIAN_POINT('Ctrl Pts',(-0.195848366636187,0.00273414417116084,
0.00873016714070241));
#40529=CARTESIAN_POINT('Ctrl Pts',(-0.195514684660614,0.00273412355097259,
0.00872293686128152));
#40530=CARTESIAN_POINT('Ctrl Pts',(-0.195178171724056,0.00273409810905456,
0.00871564249297404));
#40531=CARTESIAN_POINT('Origin',(-0.221676747656307,0.00749999656668326,
0.0016542281911168));
#40532=CARTESIAN_POINT('',(-0.221093368579246,0.00749707905428301,0.0106049493394889));
#40533=CARTESIAN_POINT('',(-0.221393324273061,0.00186012453844665,0.0086135531677188));
#40534=CARTESIAN_POINT('Ctrl Pts',(-0.221393324273061,0.00186012453844665,
0.0086135531677188));
#40535=CARTESIAN_POINT('Ctrl Pts',(-0.221320882289907,0.00211836443593635,
0.00882119182016569));
#40536=CARTESIAN_POINT('Ctrl Pts',(-0.221231403465256,0.00247125386688205,
0.00907118054582986));
#40537=CARTESIAN_POINT('Ctrl Pts',(-0.221145920712544,0.00287451696712188,
0.0093214834214468));
#40538=CARTESIAN_POINT('Ctrl Pts',(-0.221106573265363,0.00308812820272732,
0.00944560427206486));
#40539=CARTESIAN_POINT('Ctrl Pts',(-0.221059991603806,0.00341486099713401,
0.0096217897422861));
#40540=CARTESIAN_POINT('Ctrl Pts',(-0.221025097040765,0.00374441410818285,
0.00978109693071447));
#40541=CARTESIAN_POINT('Ctrl Pts',(-0.220997020866922,0.00410243999479013,
0.00993723070964949));
#40542=CARTESIAN_POINT('Ctrl Pts',(-0.220969869674211,0.00463263526782197,
0.0101388265080547));
#40543=CARTESIAN_POINT('Ctrl Pts',(-0.220961461135514,0.0051065827707716,
0.0102830013236984));
#40544=CARTESIAN_POINT('Ctrl Pts',(-0.22096742412538,0.00554565041247079,
0.0103879784709596));
#40545=CARTESIAN_POINT('Ctrl Pts',(-0.22097446939084,0.00578597401251634,
0.0104377123773018));
#40546=CARTESIAN_POINT('Ctrl Pts',(-0.22098293893607,0.00599041622708282,
0.0104749903919));
#40547=CARTESIAN_POINT('Ctrl Pts',(-0.220988776572196,0.00610221416093042,
0.0104932684418798));
#40548=CARTESIAN_POINT('Ctrl Pts',(-0.221000797352358,0.00631019098849533,
0.0105248268975094));
#40549=CARTESIAN_POINT('Ctrl Pts',(-0.221028058933879,0.00671202962450896,
0.0105746498724072));
#40550=CARTESIAN_POINT('Ctrl Pts',(-0.221063870013657,0.00715868680504821,
0.0106042063475681));
#40551=CARTESIAN_POINT('Ctrl Pts',(-0.221093368579246,0.00749707905428301,
0.0106049493394889));
#40552=CARTESIAN_POINT('',(-0.22139901452729,0.0131263848813722,0.0086245734578183));
#40553=CARTESIAN_POINT('Ctrl Pts',(-0.221093368511532,0.00749707983574417,
0.0106049493382898));
#40554=CARTESIAN_POINT('Ctrl Pts',(-0.221064138632359,0.00783440526382265,
0.0106044317127623));
#40555=CARTESIAN_POINT('Ctrl Pts',(-0.221028690283817,0.00827968401694266,
0.0105753564148156));
#40556=CARTESIAN_POINT('Ctrl Pts',(-0.221001771034026,0.00868043883058296,
0.0105260869185151));
#40557=CARTESIAN_POINT('Ctrl Pts',(-0.220989940522154,0.00888778115969991,
0.0104948644318784));
#40558=CARTESIAN_POINT('Ctrl Pts',(-0.220984195526036,0.00899953416961957,
0.0104767199871332));
#40559=CARTESIAN_POINT('Ctrl Pts',(-0.220975962958393,0.00920256216542126,
0.0104399565249176));
#40560=CARTESIAN_POINT('Ctrl Pts',(-0.220969173569176,0.00944187368631053,
0.010390779029624));
#40561=CARTESIAN_POINT('Ctrl Pts',(-0.220963664948118,0.00987968825111028,
0.0102868015301267));
#40562=CARTESIAN_POINT('Ctrl Pts',(-0.220972537969122,0.0103543468070456,
0.0101433091098129));
#40563=CARTESIAN_POINT('Ctrl Pts',(-0.22100014605577,0.0108863043563923,
0.00994189923874667));
#40564=CARTESIAN_POINT('Ctrl Pts',(-0.221028400357267,0.0112443083842731,
0.0097863495839049));
#40565=CARTESIAN_POINT('Ctrl Pts',(-0.221063406650245,0.011573393629629,
0.00962781935203964));
#40566=CARTESIAN_POINT('Ctrl Pts',(-0.221109786986603,0.0118977656332968,
0.00945360557205793));
#40567=CARTESIAN_POINT('Ctrl Pts',(-0.221149495808629,0.0121123070321511,
0.00932948385688051));
#40568=CARTESIAN_POINT('Ctrl Pts',(-0.221235610859116,0.012515396777809,
0.00908025727666793));
#40569=CARTESIAN_POINT('Ctrl Pts',(-0.221325901145816,0.0128682488917034,
0.00883128630788534));
#40570=CARTESIAN_POINT('Ctrl Pts',(-0.22139901452729,0.0131263848813722,
0.0086245734578183));
#40571=CARTESIAN_POINT('',(-0.222398584008074,0.0131269370004452,0.00864558885643978));
#40572=CARTESIAN_POINT('Ctrl Pts',(-0.221399005354199,0.0131263862088147,
0.00862457218979462));
#40573=CARTESIAN_POINT('Ctrl Pts',(-0.22173218058233,0.0131265693374647,
0.00863157775568907));
#40574=CARTESIAN_POINT('Ctrl Pts',(-0.222065430958852,0.0131267587198589,
0.00863857987776453));
#40575=CARTESIAN_POINT('Ctrl Pts',(-0.222398552886268,0.0131269542394213,
0.00864557427637836));
#40576=CARTESIAN_POINT('',(-0.222093143437656,0.00749648534996505,0.0106264030851718));
#40577=CARTESIAN_POINT('Ctrl Pts',(-0.222398584008074,0.0131269370004452,
0.00864558885643978));
#40578=CARTESIAN_POINT('Ctrl Pts',(-0.222325641082348,0.0128695208609679,
0.00885175731756058));
#40579=CARTESIAN_POINT('Ctrl Pts',(-0.222235540235227,0.0125176000581379,
0.00910020560792411));
#40580=CARTESIAN_POINT('Ctrl Pts',(-0.222149564294992,0.0121153707119367,
0.00934910793309511));
#40581=CARTESIAN_POINT('Ctrl Pts',(-0.222109873160673,0.0119010991654769,
0.00947318891730329));
#40582=CARTESIAN_POINT('Ctrl Pts',(-0.222063547308976,0.0115772555261176,
0.00964731674420564));
#40583=CARTESIAN_POINT('Ctrl Pts',(-0.222028542068434,0.0112478469047188,
0.00980619275617348));
#40584=CARTESIAN_POINT('Ctrl Pts',(-0.222000270545164,0.0108892810765668,
0.0099621912896326));
#40585=CARTESIAN_POINT('Ctrl Pts',(-0.221972560495376,0.01035418756447,
0.0101648683784779));
#40586=CARTESIAN_POINT('Ctrl Pts',(-0.22196374637383,0.00988361918379579,
0.0103070820085407));
#40587=CARTESIAN_POINT('Ctrl Pts',(-0.22196900595078,0.00944781271840059,
0.0104109088339609));
#40588=CARTESIAN_POINT('Ctrl Pts',(-0.221975632337354,0.00920971477057703,
0.0104600109800392));
#40589=CARTESIAN_POINT('Ctrl Pts',(-0.221983661532872,0.00900833042423417,
0.0104966686439572));
#40590=CARTESIAN_POINT('Ctrl Pts',(-0.221989384785992,0.00889557040884757,
0.0105150945176128));
#40591=CARTESIAN_POINT('Ctrl Pts',(-0.222001164804074,0.00868751157232488,
0.0105465995258684));
#40592=CARTESIAN_POINT('Ctrl Pts',(-0.222028109563492,0.00828446961210274,
0.0105964575047171));
#40593=CARTESIAN_POINT('Ctrl Pts',(-0.22206372594124,0.00783626729013152,
0.0106259053127712));
#40594=CARTESIAN_POINT('Ctrl Pts',(-0.222093143437656,0.00749648534996505,
0.0106264030851718));
#40595=CARTESIAN_POINT('',(-0.222392855892362,0.00185977364761083,0.00863470624003947));
#40596=CARTESIAN_POINT('Ctrl Pts',(-0.222093143598432,0.0074964834929572,
0.0106264030878921));
#40597=CARTESIAN_POINT('Ctrl Pts',(-0.22206375015713,0.00715897485979281,
0.0106256396722468));
#40598=CARTESIAN_POINT('Ctrl Pts',(-0.222028050253872,0.00671348063535476,
0.010596200751429));
#40599=CARTESIAN_POINT('Ctrl Pts',(-0.222000846841533,0.00631280356028926,
0.0105466293505842));
#40600=CARTESIAN_POINT('Ctrl Pts',(-0.221988831912577,0.00610531304827131,
0.0105152119148758));
#40601=CARTESIAN_POINT('Ctrl Pts',(-0.22198300522171,0.00599413078537288,
0.0104970825394779));
#40602=CARTESIAN_POINT('Ctrl Pts',(-0.221974470768666,0.00578916799523837,
0.0104597946922141));
#40603=CARTESIAN_POINT('Ctrl Pts',(-0.221967372630738,0.00554854776043954,
0.0104100791661046));
#40604=CARTESIAN_POINT('Ctrl Pts',(-0.221961300260906,0.00510911991771959,
0.0103051978930735));
#40605=CARTESIAN_POINT('Ctrl Pts',(-0.221969719400783,0.00463309356998036,
0.0101603737211353));
#40606=CARTESIAN_POINT('Ctrl Pts',(-0.221996612877404,0.00410625701407935,
0.0099601894605402));
#40607=CARTESIAN_POINT('Ctrl Pts',(-0.222024427583076,0.00374960296769934,
0.00980491605246754));
#40608=CARTESIAN_POINT('Ctrl Pts',(-0.222059048888332,0.00342099857771816,
0.00964632710519627));
#40609=CARTESIAN_POINT('Ctrl Pts',(-0.22210506112296,0.00309585054480878,
0.00947138795878032));
#40610=CARTESIAN_POINT('Ctrl Pts',(-0.222144630451831,0.0028796076224462,
0.00934600847256188));
#40611=CARTESIAN_POINT('Ctrl Pts',(-0.222230300116289,0.00247416995600222,
0.00909464993907419));
#40612=CARTESIAN_POINT('Ctrl Pts',(-0.222320125851231,0.00211925508531268,
0.00884336697495338));
#40613=CARTESIAN_POINT('Ctrl Pts',(-0.222392855892362,0.00185977364761083,
0.00863470624003947));
#40614=CARTESIAN_POINT('Ctrl Pts',(-0.22239282131095,0.00185976173076948,
0.00863469584383406));
#40615=CARTESIAN_POINT('Ctrl Pts',(-0.222059512049327,0.00185988814640051,
0.00862764965075787));
#40616=CARTESIAN_POINT('Ctrl Pts',(-0.221726263388519,0.00186000852650555,
0.0086205998615492));
#40617=CARTESIAN_POINT('Ctrl Pts',(-0.221393313500158,0.00186012280700108,
0.00861355153407611));
#40618=CARTESIAN_POINT('Origin',(-0.21967833919211,0.00750000224638511,
0.0015821781795227));
#40619=CARTESIAN_POINT('',(-0.219093931424061,0.00749805713493659,0.0105597809184262));
#40620=CARTESIAN_POINT('',(-0.219329675491582,0.00207001641050771,0.00873878981654981));
#40621=CARTESIAN_POINT('Ctrl Pts',(-0.219329675491582,0.00207001641050771,
0.0087387898165498));
#40622=CARTESIAN_POINT('Ctrl Pts',(-0.21926673218781,0.00232397546437185,
0.00893001603366529));
#40623=CARTESIAN_POINT('Ctrl Pts',(-0.21918910173417,0.00266911277428291,
0.0091597253869842));
#40624=CARTESIAN_POINT('Ctrl Pts',(-0.219115197421065,0.00306172087601469,
0.00938926825850818));
#40625=CARTESIAN_POINT('Ctrl Pts',(-0.219081341420747,0.00326851581087775,
0.00950267558687953));
#40626=CARTESIAN_POINT('Ctrl Pts',(-0.219041428682301,0.00358655944730087,
0.00966440155326771));
#40627=CARTESIAN_POINT('Ctrl Pts',(-0.219002234332528,0.00400670339074093,
0.00985725686767314));
#40628=CARTESIAN_POINT('Ctrl Pts',(-0.218968686763695,0.0046367188189223,
0.0101006623712429));
#40629=CARTESIAN_POINT('Ctrl Pts',(-0.218962333710723,0.00521465726012983,
0.0102673885531289));
#40630=CARTESIAN_POINT('Ctrl Pts',(-0.218970025383219,0.00563368217517905,
0.0103625206402003));
#40631=CARTESIAN_POINT('Ctrl Pts',(-0.21897762636222,0.00586348838946524,
0.0104077368567593));
#40632=CARTESIAN_POINT('Ctrl Pts',(-0.218986309443235,0.00605854847551105,
0.0104415635341072));
#40633=CARTESIAN_POINT('Ctrl Pts',(-0.218992164333208,0.00616555763761863,
0.0104582113469295));
#40634=CARTESIAN_POINT('Ctrl Pts',(-0.219004098923365,0.00636432765538068,
0.010486908383612));
#40635=CARTESIAN_POINT('Ctrl Pts',(-0.219030818498434,0.00674834748173606,
0.0105322256424722));
#40636=CARTESIAN_POINT('Ctrl Pts',(-0.219065504441556,0.00717490747545383,
0.010559101519801));
#40637=CARTESIAN_POINT('Ctrl Pts',(-0.219093931424061,0.00749805713493659,
0.0105597809184262));
#40638=CARTESIAN_POINT('',(-0.219334449421015,0.0129184051342887,0.00874766341044521));
#40639=CARTESIAN_POINT('Ctrl Pts',(-0.219093931309954,0.00749805843864198,
0.0105597809162631));
#40640=CARTESIAN_POINT('Ctrl Pts',(-0.219065711408738,0.00782047596527625,
0.010559245912387));
#40641=CARTESIAN_POINT('Ctrl Pts',(-0.219031316520399,0.00824607622127998,
0.0105326831954569));
#40642=CARTESIAN_POINT('Ctrl Pts',(-0.219004889515743,0.00862937329987748,
0.010487720905152));
#40643=CARTESIAN_POINT('Ctrl Pts',(-0.218993127081861,0.00882766146147039,
0.0104592502874459));
#40644=CARTESIAN_POINT('Ctrl Pts',(-0.218987354155981,0.00893476683096917,
0.0104426666457267));
#40645=CARTESIAN_POINT('Ctrl Pts',(-0.218978909341311,0.00912836382219906,
0.0104092624073532));
#40646=CARTESIAN_POINT('Ctrl Pts',(-0.218971559602137,0.00935720765481112,
0.0103644753266291));
#40647=CARTESIAN_POINT('Ctrl Pts',(-0.218964305057173,0.00977503223623715,
0.0102701201291484));
#40648=CARTESIAN_POINT('Ctrl Pts',(-0.218971244168002,0.0103548699408352,
0.0101036237942178));
#40649=CARTESIAN_POINT('Ctrl Pts',(-0.219005168265794,0.0109862554488166,
0.0098602839683849));
#40650=CARTESIAN_POINT('Ctrl Pts',(-0.219044409430049,0.0114052096208588,
0.00966840150914399));
#40651=CARTESIAN_POINT('Ctrl Pts',(-0.219084036732671,0.0117202529412656,
0.00950870094055952));
#40652=CARTESIAN_POINT('Ctrl Pts',(-0.219118190408138,0.0119278693536131,
0.00939524877450844));
#40653=CARTESIAN_POINT('Ctrl Pts',(-0.21919260264818,0.0123199329036179,
0.00916673739389008));
#40654=CARTESIAN_POINT('Ctrl Pts',(-0.219270925812016,0.0126647568293119,
0.0089379970943531));
#40655=CARTESIAN_POINT('Ctrl Pts',(-0.219334449421015,0.0129184051342887,
0.00874766341044521));
#40656=CARTESIAN_POINT('',(-0.220398875414435,0.013127345180933,0.00860767229782415));
#40657=CARTESIAN_POINT('Ctrl Pts',(-0.2193344482324,0.0129185235189919,
0.00874777258268191));
#40658=CARTESIAN_POINT('Ctrl Pts',(-0.219446892856324,0.0129669566534953,
0.00871338003143611));
#40659=CARTESIAN_POINT('Ctrl Pts',(-0.219543061237216,0.0130071173503667,
0.00868434426531221));
#40660=CARTESIAN_POINT('Ctrl Pts',(-0.21962977665937,0.0130390459589621,
0.00866119629744851));
#40661=CARTESIAN_POINT('Ctrl Pts',(-0.219673135892507,0.0130550108236821,
0.00864962190721527));
#40662=CARTESIAN_POINT('Ctrl Pts',(-0.219714134616583,0.0130688951516554,
0.00863954132345271));
#40663=CARTESIAN_POINT('Ctrl Pts',(-0.219746959307074,0.0130792506280983,
0.00863205556330531));
#40664=CARTESIAN_POINT('Ctrl Pts',(-0.219779783997565,0.0130896061045412,
0.00862456980315791));
#40665=CARTESIAN_POINT('Ctrl Pts',(-0.219804185483759,0.0130968868605942,
0.00861931110782013));
#40666=CARTESIAN_POINT('Ctrl Pts',(-0.219843260685388,0.0131070498458526,
0.00861201982549279));
#40667=CARTESIAN_POINT('Ctrl Pts',(-0.219855710948212,0.0131102880079675,
0.00860969665433781));
#40668=CARTESIAN_POINT('Ctrl Pts',(-0.219869697085274,0.0131137784499516,
0.00860720288149674));
#40669=CARTESIAN_POINT('Ctrl Pts',(-0.219884547633558,0.0131172460352354,
0.00860474250115293));
#40670=CARTESIAN_POINT('Ctrl Pts',(-0.219916305592798,0.0131246614807796,
0.00859948096755987));
#40671=CARTESIAN_POINT('Ctrl Pts',(-0.219952020187925,0.013131841676374,
0.00859447424251011));
#40672=CARTESIAN_POINT('Ctrl Pts',(-0.219985174108256,0.0131371095774531,
0.00859094902561431));
#40673=CARTESIAN_POINT('Ctrl Pts',(-0.220033831351422,0.0131448408364181,
0.00858577535885028));
#40674=CARTESIAN_POINT('Ctrl Pts',(-0.220076741916514,0.0131489240309038,
0.00858338293662867));
#40675=CARTESIAN_POINT('Ctrl Pts',(-0.220118876196711,0.0131505486997066,
0.00858296642564705));
#40676=CARTESIAN_POINT('Ctrl Pts',(-0.220141481026886,0.0131514203263775,
0.00858274296959271));
#40677=CARTESIAN_POINT('Ctrl Pts',(-0.220163923963669,0.0131515501294491,
0.00858311495808394));
#40678=CARTESIAN_POINT('Ctrl Pts',(-0.220186832211857,0.013150858495987,
0.00858416347060276));
#40679=CARTESIAN_POINT('Ctrl Pts',(-0.220249322385183,0.0131489718264098,
0.00858702365128946));
#40680=CARTESIAN_POINT('Ctrl Pts',(-0.22031494630866,0.0131409425340114,
0.00859494515751143));
#40681=CARTESIAN_POINT('Ctrl Pts',(-0.220398951901741,0.0131276350205432,
0.00860743104837679));
#40682=CARTESIAN_POINT('',(-0.220093673496084,0.00749758231473663,0.0105812097663496));
#40683=CARTESIAN_POINT('Ctrl Pts',(-0.220398875414435,0.013127345180933,
0.00860767229782415));
#40684=CARTESIAN_POINT('Ctrl Pts',(-0.220325934104189,0.0128696007310759,
0.00881311000494965));
#40685=CARTESIAN_POINT('Ctrl Pts',(-0.220235832151988,0.012517380154814,
0.00906064802695024));
#40686=CARTESIAN_POINT('Ctrl Pts',(-0.22014983518567,0.0121148742622212,
0.00930865312239604));
#40687=CARTESIAN_POINT('Ctrl Pts',(-0.220110148563968,0.0119006189294791,
0.00943221399864835));
#40688=CARTESIAN_POINT('Ctrl Pts',(-0.220063730000698,0.0115762317761984,
0.00960591985594359));
#40689=CARTESIAN_POINT('Ctrl Pts',(-0.220028700288234,0.011246729617028,
0.0097641926164711));
#40690=CARTESIAN_POINT('Ctrl Pts',(-0.220000425693391,0.0108882511595183,
0.00991953869054433));
#40691=CARTESIAN_POINT('Ctrl Pts',(-0.21997276242715,0.0103537426143642,
0.0101212364943754));
#40692=CARTESIAN_POINT('Ctrl Pts',(-0.219964019306003,0.00988381931694247,
0.0102628033818167));
#40693=CARTESIAN_POINT('Ctrl Pts',(-0.219969349684687,0.00944806796185167,
0.010366308027579));
#40694=CARTESIAN_POINT('Ctrl Pts',(-0.219976017534628,0.00920993945947005,
0.0104152726707589));
#40695=CARTESIAN_POINT('Ctrl Pts',(-0.219984088108219,0.00900837540122992,
0.0104518536356056));
#40696=CARTESIAN_POINT('Ctrl Pts',(-0.219989822314319,0.00889575753165797,
0.0104702005507611));
#40697=CARTESIAN_POINT('Ctrl Pts',(-0.220001626212636,0.00868779787530209,
0.0105016013492101));
#40698=CARTESIAN_POINT('Ctrl Pts',(-0.220028604724524,0.00828502755883445,
0.0105512922085914));
#40699=CARTESIAN_POINT('Ctrl Pts',(-0.220064244947719,0.00783712777332673,
0.0105806702055769));
#40700=CARTESIAN_POINT('Ctrl Pts',(-0.220093673496084,0.00749758231473663,
0.0105812097663496));
#40701=CARTESIAN_POINT('',(-0.220393469212935,0.00185932807944966,0.00859684197992795));
#40702=CARTESIAN_POINT('Ctrl Pts',(-0.220093673613352,0.00749758096170686,
0.0105812097684996));
#40703=CARTESIAN_POINT('Ctrl Pts',(-0.220064263129577,0.00716015337126071,
0.0105804886629416));
#40704=CARTESIAN_POINT('Ctrl Pts',(-0.220028538804154,0.00671475847876594,
0.010551204008513));
#40705=CARTESIAN_POINT('Ctrl Pts',(-0.220001313267265,0.00631415782065367,
0.0105018520462385));
#40706=CARTESIAN_POINT('Ctrl Pts',(-0.219989286579143,0.00610669204075673,
0.0104705664657165));
#40707=CARTESIAN_POINT('Ctrl Pts',(-0.219983455094469,0.00599554664686926,
0.0104525162872843));
#40708=CARTESIAN_POINT('Ctrl Pts',(-0.219974905590976,0.00579052816249508,
0.0104153681588899));
#40709=CARTESIAN_POINT('Ctrl Pts',(-0.219967795508928,0.00554977942667081,
0.0103658112243735));
#40710=CARTESIAN_POINT('Ctrl Pts',(-0.219961695456283,0.00511134405379829,
0.0102616067514142));
#40711=CARTESIAN_POINT('Ctrl Pts',(-0.219972297213109,0.00450814141055009,
0.0100789890536557));
#40712=CARTESIAN_POINT('Ctrl Pts',(-0.22001334899915,0.00385700754459336,
0.0098147555328663));
#40713=CARTESIAN_POINT('Ctrl Pts',(-0.220059518713161,0.00342300351096295,
0.00960528627718777));
#40714=CARTESIAN_POINT('Ctrl Pts',(-0.220105621826452,0.00309650561112459,
0.00943058591199622));
#40715=CARTESIAN_POINT('Ctrl Pts',(-0.220145194571405,0.00288044200687532,
0.0093057716638572));
#40716=CARTESIAN_POINT('Ctrl Pts',(-0.220230894847921,0.00247454997032606,
0.00905526038955808));
#40717=CARTESIAN_POINT('Ctrl Pts',(-0.220320732206519,0.00211923598389529,
0.00880483474782587));
#40718=CARTESIAN_POINT('Ctrl Pts',(-0.220393469212935,0.00185932807944966,
0.00859684197992795));
#40719=CARTESIAN_POINT('Ctrl Pts',(-0.220393469326552,0.00185932703395312,
0.00859684113942577));
#40720=CARTESIAN_POINT('Ctrl Pts',(-0.220266240041375,0.00185875869807335,
0.00859365486146192));
#40721=CARTESIAN_POINT('Ctrl Pts',(-0.220103936772937,0.0018605882269132,
0.00859165532427359));
#40722=CARTESIAN_POINT('Ctrl Pts',(-0.219926730734395,0.00187135174347915,
0.00859651152760235));
#40723=CARTESIAN_POINT('Ctrl Pts',(-0.219849192249158,0.00187769702112859,
0.00859995165438822));
#40724=CARTESIAN_POINT('Ctrl Pts',(-0.219683953461115,0.00190591750515629,
0.00861898651311973));
#40725=CARTESIAN_POINT('Ctrl Pts',(-0.219522447796733,0.00195479415049073,
0.0086541771714266));
#40726=CARTESIAN_POINT('Ctrl Pts',(-0.219420848743358,0.00201019267767576,
0.00869537988459834));
#40727=CARTESIAN_POINT('Ctrl Pts',(-0.219329691282643,0.00206995189687594,
0.00873874123435077));
#40728=CARTESIAN_POINT('Origin',(-0.21760795179008,0.00750000191208944,
0.00150723219269739));
#40729=CARTESIAN_POINT('',(-0.217094603861694,0.00749884707608177,0.0105144330567323));
#40730=CARTESIAN_POINT('',(-0.217213232792442,0.00253460675136436,0.0090261857131641));
#40731=CARTESIAN_POINT('Ctrl Pts',(-0.217213232792442,0.00253460675136436,
0.00902618571316409));
#40732=CARTESIAN_POINT('Ctrl Pts',(-0.217170309351211,0.00277579295122344,
0.00918442809411469));
#40733=CARTESIAN_POINT('Ctrl Pts',(-0.217117004028407,0.00309947496425187,
0.00937334421669727));
#40734=CARTESIAN_POINT('Ctrl Pts',(-0.21706463523819,0.00346758551596026,
0.0095627049050888));
#40735=CARTESIAN_POINT('Ctrl Pts',(-0.217040687245035,0.00365149899647496,
0.00965203925472441));
#40736=CARTESIAN_POINT('Ctrl Pts',(-0.217007699799833,0.00397270993102743,
0.00979619091369355));
#40737=CARTESIAN_POINT('Ctrl Pts',(-0.216979123906403,0.00436472477058794,
0.00995398513378322));
#40738=CARTESIAN_POINT('Ctrl Pts',(-0.216960097915139,0.00491864701878528,
0.0101420370266245));
#40739=CARTESIAN_POINT('Ctrl Pts',(-0.21696496840512,0.00539322729827493,
0.010266679263318));
#40740=CARTESIAN_POINT('Ctrl Pts',(-0.216978301352722,0.00578584987535544,
0.0103486271386283));
#40741=CARTESIAN_POINT('Ctrl Pts',(-0.216988380938197,0.0060059828310731,
0.0103881729924593));
#40742=CARTESIAN_POINT('Ctrl Pts',(-0.216999137729455,0.00620401844451835,
0.010419155240653));
#40743=CARTESIAN_POINT('Ctrl Pts',(-0.21700485626558,0.00629724070264874,
0.0104320669469113));
#40744=CARTESIAN_POINT('Ctrl Pts',(-0.217016575872302,0.00648013407847732,
0.0104558017273798));
#40745=CARTESIAN_POINT('Ctrl Pts',(-0.217040949115086,0.00682691734809784,
0.0104923617788424));
#40746=CARTESIAN_POINT('Ctrl Pts',(-0.217070787207733,0.00721009507694088,
0.0105138806616736));
#40747=CARTESIAN_POINT('Ctrl Pts',(-0.217094604615836,0.00749884651657513,
0.0105144330760153));
#40748=CARTESIAN_POINT('',(-0.217217320966152,0.0124615983754921,0.00902878263841572));
#40749=CARTESIAN_POINT('Ctrl Pts',(-0.217094604580183,0.00749884713502375,
0.0105144330753234));
#40750=CARTESIAN_POINT('Ctrl Pts',(-0.217070937522513,0.00778749281737824,
0.01051395809991));
#40751=CARTESIAN_POINT('Ctrl Pts',(-0.217041312684742,0.00817050093947764,
0.0104925590483005));
#40752=CARTESIAN_POINT('Ctrl Pts',(-0.217017156529758,0.00851709921734971,
0.0104561284919407));
#40753=CARTESIAN_POINT('Ctrl Pts',(-0.217005563781867,0.00869984918082267,
0.0104324752847162));
#40754=CARTESIAN_POINT('Ctrl Pts',(-0.216999909235435,0.00879305702910093,
0.0104195962148299));
#40755=CARTESIAN_POINT('Ctrl Pts',(-0.216989318519438,0.00899071226752479,
0.0103887488120621));
#40756=CARTESIAN_POINT('Ctrl Pts',(-0.216979434680228,0.00921060200406897,
0.0103493316559271));
#40757=CARTESIAN_POINT('Ctrl Pts',(-0.216966443804416,0.00960257895555559,
0.0102677731436431));
#40758=CARTESIAN_POINT('Ctrl Pts',(-0.216962353786427,0.0100798262263821,
0.0101422226623979));
#40759=CARTESIAN_POINT('Ctrl Pts',(-0.216981259047774,0.0106259713240169,
0.00995801306633485));
#40760=CARTESIAN_POINT('Ctrl Pts',(-0.217008015270036,0.0109796849032678,
0.00981495279359965));
#40761=CARTESIAN_POINT('Ctrl Pts',(-0.217026124783938,0.0111726831205931,
0.00973148164241474));
#40762=CARTESIAN_POINT('Ctrl Pts',(-0.217043798305059,0.0113336323415438,
0.00965791312087231));
#40763=CARTESIAN_POINT('Ctrl Pts',(-0.217054626933635,0.011421252747556,
0.00961622526465953));
#40764=CARTESIAN_POINT('Ctrl Pts',(-0.217075748242504,0.0115827300577152,
0.00953743738321973));
#40765=CARTESIAN_POINT('Ctrl Pts',(-0.217120156049393,0.0118899261409953,
0.00937864862166455));
#40766=CARTESIAN_POINT('Ctrl Pts',(-0.217174287324889,0.0122201761123988,
0.0091870018582681));
#40767=CARTESIAN_POINT('Ctrl Pts',(-0.217217320966152,0.0124615983754921,
0.00902878263841572));
#40768=CARTESIAN_POINT('',(-0.218253210572638,0.0126493218644601,0.00892398112026186));
#40769=CARTESIAN_POINT('Ctrl Pts',(-0.217217407969934,0.012461760044758,
0.00902867794239265));
#40770=CARTESIAN_POINT('Ctrl Pts',(-0.217390176156768,0.0125240868152205,
0.00899132591420084));
#40771=CARTESIAN_POINT('Ctrl Pts',(-0.217559211504655,0.0125854878241809,
0.00895315310690254));
#40772=CARTESIAN_POINT('Ctrl Pts',(-0.217872840726586,0.0126523647125971,
0.00891377523936488));
#40773=CARTESIAN_POINT('Ctrl Pts',(-0.218037719196302,0.0126678617041626,
0.00890646877918805));
#40774=CARTESIAN_POINT('Ctrl Pts',(-0.218252689489813,0.0126468959037447,
0.00892569856217048));
#40775=CARTESIAN_POINT('',(-0.218094234747031,0.00749853993277985,0.0105360606597374));
#40776=CARTESIAN_POINT('Ctrl Pts',(-0.21825294850133,0.0126481187356084,
0.00892485362262281));
#40777=CARTESIAN_POINT('Ctrl Pts',(-0.218213614101177,0.0124649627842807,
0.00905141958171181));
#40778=CARTESIAN_POINT('Ctrl Pts',(-0.218178110563308,0.0122764066318995,
0.00917173521317051));
#40779=CARTESIAN_POINT('Ctrl Pts',(-0.218033008484456,0.0113863756832155,
0.00969402331777485));
#40780=CARTESIAN_POINT('Ctrl Pts',(-0.217971681763306,0.010633235009572,
0.0100108663882326));
#40781=CARTESIAN_POINT('Ctrl Pts',(-0.217958148745726,0.00907579362155081,
0.0104298068455017));
#40782=CARTESIAN_POINT('Ctrl Pts',(-0.218002961139097,0.00828768224388102,
0.0105340872225598));
#40783=CARTESIAN_POINT('Ctrl Pts',(-0.218097863485635,0.00749998147943064,
0.0105361392872622));
#40784=CARTESIAN_POINT('',(-0.218256592144584,0.00234509828687441,0.00892021730379066));
#40785=CARTESIAN_POINT('Ctrl Pts',(-0.218094234747031,0.00749853993277985,
0.0105360606597374));
#40786=CARTESIAN_POINT('Ctrl Pts',(-0.218067229862006,0.00719461363377097,
0.0105354273206674));
#40787=CARTESIAN_POINT('Ctrl Pts',(-0.218034080490654,0.00679346748207321,
0.0105116869301656));
#40788=CARTESIAN_POINT('Ctrl Pts',(-0.21800818493669,0.00643215822152021,
0.0104716988671063));
#40789=CARTESIAN_POINT('Ctrl Pts',(-0.21799644503754,0.00624516791030783,
0.0104463965071334));
#40790=CARTESIAN_POINT('Ctrl Pts',(-0.217990618901119,0.00614435829544673,
0.0104316969225262));
#40791=CARTESIAN_POINT('Ctrl Pts',(-0.217981770592061,0.00596124495709672,
0.0104019555911123));
#40792=CARTESIAN_POINT('Ctrl Pts',(-0.217973610494308,0.00574494251941056,
0.0103621182566814));
#40793=CARTESIAN_POINT('Ctrl Pts',(-0.217964050770803,0.00535017373709659,
0.010278344750214));
#40794=CARTESIAN_POINT('Ctrl Pts',(-0.217965654179541,0.0047997316957265,
0.0101297502965913));
#40795=CARTESIAN_POINT('Ctrl Pts',(-0.217989855945059,0.0042083269497704,
0.0099166719695582));
#40796=CARTESIAN_POINT('Ctrl Pts',(-0.218020294338235,0.00380946035749678,
0.00974665422212974));
#40797=CARTESIAN_POINT('Ctrl Pts',(-0.218051893437689,0.00350742154534804,
0.00960429012063944));
#40798=CARTESIAN_POINT('Ctrl Pts',(-0.218079557608433,0.00330729544536573,
0.00950272759445357));
#40799=CARTESIAN_POINT('Ctrl Pts',(-0.218140179572864,0.00292838976944255,
0.00929780698585744));
#40800=CARTESIAN_POINT('Ctrl Pts',(-0.218204388361096,0.00259313741219679,
0.00909197882225042));
#40801=CARTESIAN_POINT('Ctrl Pts',(-0.218256592144584,0.00234509828687441,
0.00892021730379066));
#40802=CARTESIAN_POINT('Ctrl Pts',(-0.218256590177538,0.00234471180662227,
0.00891993757141349));
#40803=CARTESIAN_POINT('Ctrl Pts',(-0.218134550040916,0.00234639978140227,
0.00891846142581766));
#40804=CARTESIAN_POINT('Ctrl Pts',(-0.218030331307428,0.00234857254097845,
0.00891770527303425));
#40805=CARTESIAN_POINT('Ctrl Pts',(-0.217938284843155,0.00235370353966548,
0.00891928351630347));
#40806=CARTESIAN_POINT('Ctrl Pts',(-0.21789226158873,0.00235626904025144,
0.00892007263832024));
#40807=CARTESIAN_POINT('Ctrl Pts',(-0.217849294553891,0.00235959837297097,
0.00892146168011855));
#40808=CARTESIAN_POINT('Ctrl Pts',(-0.217815141143007,0.00236287402990444,
0.00892300578397156));
#40809=CARTESIAN_POINT('Ctrl Pts',(-0.217787234278518,0.00236555057997048,
0.00892426747631409));
#40810=CARTESIAN_POINT('Ctrl Pts',(-0.21776523359559,0.00236797977945377,
0.00892548211417782));
#40811=CARTESIAN_POINT('Ctrl Pts',(-0.217736542858525,0.00237174995177,
0.00892747026727036));
#40812=CARTESIAN_POINT('Ctrl Pts',(-0.217730120853637,0.00237259385009819,
0.00892791528647114));
#40813=CARTESIAN_POINT('Ctrl Pts',(-0.217723369119116,0.00237351184464279,
0.00892840402086493));
#40814=CARTESIAN_POINT('Ctrl Pts',(-0.217716155559666,0.00237453595774939,
0.00892895558766939));
#40815=CARTESIAN_POINT('Ctrl Pts',(-0.217676714940117,0.00238013536476782,
0.00893197131612372));
#40816=CARTESIAN_POINT('Ctrl Pts',(-0.217623386945995,0.00238937088151384,
0.00893719459845315));
#40817=CARTESIAN_POINT('Ctrl Pts',(-0.217575997502252,0.0024000928055468,
0.00894352742526225));
#40818=CARTESIAN_POINT('Ctrl Pts',(-0.217528608058509,0.00241081472957976,
0.00894986025207134));
#40819=CARTESIAN_POINT('Ctrl Pts',(-0.21748692365309,0.00242239208269951,
0.00895686377608915));
#40820=CARTESIAN_POINT('Ctrl Pts',(-0.217445993783405,0.00243562190843874,
0.00896496838443612));
#40821=CARTESIAN_POINT('Ctrl Pts',(-0.217364134044035,0.00246208155991719,
0.00898117760113005));
#40822=CARTESIAN_POINT('Ctrl Pts',(-0.217285909895761,0.00249586793471726,
0.009002268401476));
#40823=CARTESIAN_POINT('Ctrl Pts',(-0.217213846553127,0.00253441541015326,
0.00902621814787699));
#40824=CARTESIAN_POINT('Origin',(-0.215573530857847,0.00749999953571053,
0.00143242725109262));
#40825=CARTESIAN_POINT('',(-0.215095212480479,0.0074994624607262,0.0104691619874357));
#40826=CARTESIAN_POINT('',(-0.215184718243368,0.00267629428099901,0.00907717660912712));
#40827=CARTESIAN_POINT('Ctrl Pts',(-0.215184718243368,0.00267629428099901,
0.00907717660912712));
#40828=CARTESIAN_POINT('Ctrl Pts',(-0.215146525718128,0.00291333324471743,
0.00922581923697571));
#40829=CARTESIAN_POINT('Ctrl Pts',(-0.215099132128048,0.00323035142786572,
0.00940295055899245));
#40830=CARTESIAN_POINT('Ctrl Pts',(-0.215052529840506,0.00359027095313646,
0.0095804179996351));
#40831=CARTESIAN_POINT('Ctrl Pts',(-0.215031287815733,0.00376889701897786,
0.00966366879374054));
#40832=CARTESIAN_POINT('Ctrl Pts',(-0.215001646638346,0.00408470068498395,
0.00979968054158577));
#40833=CARTESIAN_POINT('Ctrl Pts',(-0.214976411300077,0.00446709191320605,
0.00994727203699884));
#40834=CARTESIAN_POINT('Ctrl Pts',(-0.214960404393782,0.00499883510574172,
0.0101209196609526));
#40835=CARTESIAN_POINT('Ctrl Pts',(-0.21496627361394,0.00546556789926266,
0.0102389566418329));
#40836=CARTESIAN_POINT('Ctrl Pts',(-0.214979945130265,0.00584476958512956,
0.0103149788292726));
#40837=CARTESIAN_POINT('Ctrl Pts',(-0.214990053470249,0.00605703382503594,
0.0103516623791654));
#40838=CARTESIAN_POINT('Ctrl Pts',(-0.215000719830354,0.00624722516962262,
0.0103803117380582));
#40839=CARTESIAN_POINT('Ctrl Pts',(-0.21500639948341,0.00633726586564142,
0.0103923346962857));
#40840=CARTESIAN_POINT('Ctrl Pts',(-0.2150180188578,0.00651372661228292,
0.0104144070541134));
#40841=CARTESIAN_POINT('Ctrl Pts',(-0.21504216176965,0.00684888162182612,
0.0104484989408323));
#40842=CARTESIAN_POINT('Ctrl Pts',(-0.215071675719688,0.00721973594776213,
0.0104686336712516));
#40843=CARTESIAN_POINT('Ctrl Pts',(-0.215095212937786,0.00749946183679744,
0.010469161998726));
#40844=CARTESIAN_POINT('',(-0.215187306909941,0.0123212872974831,0.00907875575671606));
#40845=CARTESIAN_POINT('Ctrl Pts',(-0.21509521288266,0.00749946249445561,
0.0104691619975665));
#40846=CARTESIAN_POINT('Ctrl Pts',(-0.215071829072947,0.00777843220526683,
0.0104686701414006));
#40847=CARTESIAN_POINT('Ctrl Pts',(-0.215042508186161,0.00814840410898096,
0.0104486874756129));
#40848=CARTESIAN_POINT('Ctrl Pts',(-0.215018521912491,0.00848302265137899,
0.010414771019284));
#40849=CARTESIAN_POINT('Ctrl Pts',(-0.215006981087804,0.00865925893055341,
0.0103927968298261));
#40850=CARTESIAN_POINT('Ctrl Pts',(-0.215001332092595,0.00874932749581215,
0.0103808046216084));
#40851=CARTESIAN_POINT('Ctrl Pts',(-0.214990761677216,0.00893910554359824,
0.0103522978628875));
#40852=CARTESIAN_POINT('Ctrl Pts',(-0.214980760303275,0.00915110651643444,
0.0103157592549189));
#40853=CARTESIAN_POINT('Ctrl Pts',(-0.214967291189273,0.00952991578169268,
0.0102400211047526));
#40854=CARTESIAN_POINT('Ctrl Pts',(-0.214961715433187,0.00999770202566206,
0.0101219354144702));
#40855=CARTESIAN_POINT('Ctrl Pts',(-0.21497805603957,0.0105281712554395,
0.00994897805687468));
#40856=CARTESIAN_POINT('Ctrl Pts',(-0.215003530828357,0.0109108254011088,
0.00980155134947677));
#40857=CARTESIAN_POINT('Ctrl Pts',(-0.215033385682381,0.0112272328548644,
0.00966546816384362));
#40858=CARTESIAN_POINT('Ctrl Pts',(-0.215054708220528,0.0114059998732139,
0.00958225194620914));
#40859=CARTESIAN_POINT('Ctrl Pts',(-0.215101483573991,0.0117664187103973,
0.00940474035128169));
#40860=CARTESIAN_POINT('Ctrl Pts',(-0.215149013018853,0.0120838921330146,
0.00922751589232591));
#40861=CARTESIAN_POINT('Ctrl Pts',(-0.215187306909941,0.0123212872974831,
0.00907875575671606));
#40862=CARTESIAN_POINT('',(-0.21619498111519,0.0123592223745629,0.00907662987181358));
#40863=CARTESIAN_POINT('Ctrl Pts',(-0.215187395634347,0.0123213065775708,
0.00907874549728632));
#40864=CARTESIAN_POINT('Ctrl Pts',(-0.215523256950413,0.0123339606047753,
0.00907807433826628));
#40865=CARTESIAN_POINT('Ctrl Pts',(-0.215859118725865,0.0123466006041971,
0.00907736836098088));
#40866=CARTESIAN_POINT('Ctrl Pts',(-0.216194981027653,0.0123592246090725,
0.00907662842429546));
#40867=CARTESIAN_POINT('',(-0.216094921541195,0.00749916570422793,0.0104908968200396));
#40868=CARTESIAN_POINT('Ctrl Pts',(-0.21619498111519,0.0123592223745629,
0.00907662987181358));
#40869=CARTESIAN_POINT('Ctrl Pts',(-0.216155362015906,0.0121196513974751,
0.00922839918985609));
#40870=CARTESIAN_POINT('Ctrl Pts',(-0.216106178511469,0.0117989338970978,
0.00940923223843171));
#40871=CARTESIAN_POINT('Ctrl Pts',(-0.216057811341763,0.0114349409820479,
0.00959017566794329));
#40872=CARTESIAN_POINT('Ctrl Pts',(-0.216035688926043,0.0112534767903711,
0.00967536323588877));
#40873=CARTESIAN_POINT('Ctrl Pts',(-0.216005069337273,0.010936292214568,
0.00981293044007726));
#40874=CARTESIAN_POINT('Ctrl Pts',(-0.215978741304516,0.0105517099265693,
0.00996241119423929));
#40875=CARTESIAN_POINT('Ctrl Pts',(-0.215961582825803,0.0100173646530297,
0.0101380807976369));
#40876=CARTESIAN_POINT('Ctrl Pts',(-0.21596673159867,0.0095493024043187,
0.0102572803569698));
#40877=CARTESIAN_POINT('Ctrl Pts',(-0.215979905520899,0.00916939986895247,
0.0103340767317814));
#40878=CARTESIAN_POINT('Ctrl Pts',(-0.215989775607879,0.00895666797254574,
0.0103711720214632));
#40879=CARTESIAN_POINT('Ctrl Pts',(-0.216000215681289,0.0087666271555183,
0.0104000960510575));
#40880=CARTESIAN_POINT('Ctrl Pts',(-0.216005897736623,0.00867501258808179,
0.0104124712062286));
#40881=CARTESIAN_POINT('Ctrl Pts',(-0.216017469984678,0.00849676060675789,
0.0104349965087626));
#40882=CARTESIAN_POINT('Ctrl Pts',(-0.216041627508878,0.00815759916772721,
0.0104698569176309));
#40883=CARTESIAN_POINT('Ctrl Pts',(-0.216071253207282,0.00778232161320312,
0.0104904084248528));
#40884=CARTESIAN_POINT('Ctrl Pts',(-0.216094921542323,0.00749916603381114,
0.0104908968200947));
#40885=CARTESIAN_POINT('',(-0.216191654426503,0.00263704645852275,0.00907417602083059));
#40886=CARTESIAN_POINT('Ctrl Pts',(-0.216094921541195,0.00749916570422794,
0.0104908968200396));
#40887=CARTESIAN_POINT('Ctrl Pts',(-0.216071192372307,0.00721653565110898,
0.0104903547759566));
#40888=CARTESIAN_POINT('Ctrl Pts',(-0.216041458964601,0.00684184722529076,
0.0104697980736088));
#40889=CARTESIAN_POINT('Ctrl Pts',(-0.216017167701719,0.00650321518860178,
0.0104349873050386));
#40890=CARTESIAN_POINT('Ctrl Pts',(-0.216005495918259,0.00632499391538343,
0.0104124603199507));
#40891=CARTESIAN_POINT('Ctrl Pts',(-0.215999785556795,0.00623389233782072,
0.0104001638087242));
#40892=CARTESIAN_POINT('Ctrl Pts',(-0.215989126899373,0.00604229502726595,
0.0103709986123811));
#40893=CARTESIAN_POINT('Ctrl Pts',(-0.215979049981255,0.00582832919195152,
0.0103336406317383));
#40894=CARTESIAN_POINT('Ctrl Pts',(-0.215965509745345,0.00544633154702591,
0.0102563020723301));
#40895=CARTESIAN_POINT('Ctrl Pts',(-0.215960018296731,0.00497512481975459,
0.0101358767402293));
#40896=CARTESIAN_POINT('Ctrl Pts',(-0.215976719095431,0.00444282320964421,
0.00996037719921713));
#40897=CARTESIAN_POINT('Ctrl Pts',(-0.2160026550059,0.0040591388957791,
0.00981098396273215));
#40898=CARTESIAN_POINT('Ctrl Pts',(-0.216032864044917,0.00374339550357232,
0.00967386268571153));
#40899=CARTESIAN_POINT('Ctrl Pts',(-0.21605487584295,0.00356169862545164,
0.00958848969233502));
#40900=CARTESIAN_POINT('Ctrl Pts',(-0.216103025180366,0.00319777204921344,
0.00940738142590156));
#40901=CARTESIAN_POINT('Ctrl Pts',(-0.216152098903379,0.00287680952339826,
0.00922623444225587));
#40902=CARTESIAN_POINT('Ctrl Pts',(-0.216191654426503,0.00263704645852275,
0.00907417602083059));
#40903=CARTESIAN_POINT('Ctrl Pts',(-0.216191653441714,0.00263701806743481,
0.0090741571960286));
#40904=CARTESIAN_POINT('Ctrl Pts',(-0.215856037597591,0.0026500960872135,
0.00907520307043243));
#40905=CARTESIAN_POINT('Ctrl Pts',(-0.215520422243746,0.00266318974959057,
0.0090762109895145));
#40906=CARTESIAN_POINT('Ctrl Pts',(-0.215184807285386,0.00267629643176575,
0.00907717990060014));
#40907=CARTESIAN_POINT('Origin',(-0.191547395567967,0.00749999908856939,
0.000492597042041278));
#40908=CARTESIAN_POINT('',(-0.192132144845555,0.0119762408965025,0.00882053073189916));
#40909=CARTESIAN_POINT('',(-0.191055849854836,0.0113889510484509,0.00908769145233091));
#40910=CARTESIAN_POINT('Ctrl Pts',(-0.191056614430799,0.0113898867221809,
0.0090872068420641));
#40911=CARTESIAN_POINT('Ctrl Pts',(-0.191117574310851,0.0114548399350986,
0.00905915673004499));
#40912=CARTESIAN_POINT('Ctrl Pts',(-0.191190506743783,0.0115169438727942,
0.00903175032826067));
#40913=CARTESIAN_POINT('Ctrl Pts',(-0.191270216528898,0.0115738470715757,
0.00900626058658664));
#40914=CARTESIAN_POINT('Ctrl Pts',(-0.191310071421455,0.0116022986709664,
0.00899351571574962));
#40915=CARTESIAN_POINT('Ctrl Pts',(-0.191351620396497,0.0116294555035853,
0.00898126176834248));
#40916=CARTESIAN_POINT('Ctrl Pts',(-0.191400054122322,0.011657748330379,
0.00896843433727955));
#40917=CARTESIAN_POINT('Ctrl Pts',(-0.191448487848146,0.0116860411571727,
0.00895560690621663));
#40918=CARTESIAN_POINT('Ctrl Pts',(-0.191503807137231,0.0117154517655055,
0.00894216860952244));
#40919=CARTESIAN_POINT('Ctrl Pts',(-0.191545244991808,0.0117363473659623,
0.00893257605113595));
#40920=CARTESIAN_POINT('Ctrl Pts',(-0.191586682846384,0.0117572429664192,
0.00892298349274945));
#40921=CARTESIAN_POINT('Ctrl Pts',(-0.191614238129345,0.0117696499199227,
0.00891728899045274));
#40922=CARTESIAN_POINT('Ctrl Pts',(-0.191651171850599,0.0117857911134441,
0.00890986709567738));
#40923=CARTESIAN_POINT('Ctrl Pts',(-0.191688105571854,0.0118019323069654,
0.00890244520090202));
#40924=CARTESIAN_POINT('Ctrl Pts',(-0.191734418368519,0.0118217927219441,
0.00889326660022605));
#40925=CARTESIAN_POINT('Ctrl Pts',(-0.191784295315848,0.0118423082724498,
0.00888372257736298));
#40926=CARTESIAN_POINT('Ctrl Pts',(-0.191884049210506,0.011883339373461,
0.00886463453163682));
#40927=CARTESIAN_POINT('Ctrl Pts',(-0.191998058757268,0.0119270141737984,
0.00884412853116881));
#40928=CARTESIAN_POINT('Ctrl Pts',(-0.192132145017542,0.0119762404947695,
0.00882053095199951));
#40929=CARTESIAN_POINT('',(-0.192104389150085,0.00749606093322131,0.00994933148053198));
#40930=CARTESIAN_POINT('Ctrl Pts',(-0.192132144845555,0.0119762408965025,
0.00882053073189916));
#40931=CARTESIAN_POINT('Ctrl Pts',(-0.192103715169681,0.0117490897743726,
0.00894225010388478));
#40932=CARTESIAN_POINT('Ctrl Pts',(-0.192068573234184,0.0114478633967073,
0.00908676981991131));
#40933=CARTESIAN_POINT('Ctrl Pts',(-0.192034329267438,0.0111082303760389,
0.00923117662410021));
#40934=CARTESIAN_POINT('Ctrl Pts',(-0.19201889600854,0.0109412049797955,
0.00929844365315326));
#40935=CARTESIAN_POINT('Ctrl Pts',(-0.191997561428072,0.0106431647032832,
0.00940955553695104));
#40936=CARTESIAN_POINT('Ctrl Pts',(-0.191980397858888,0.010285777696736,
0.00952909690683793));
#40937=CARTESIAN_POINT('Ctrl Pts',(-0.191971805248502,0.00979625382147503,
0.00966822026083504));
#40938=CARTESIAN_POINT('Ctrl Pts',(-0.191980496803262,0.0093617963463922,
0.00976413432443437));
#40939=CARTESIAN_POINT('Ctrl Pts',(-0.19199493540629,0.00901347121364747,
0.00982508008438882));
#40940=CARTESIAN_POINT('Ctrl Pts',(-0.192005038620267,0.00881887992917666,
0.00985447421971926));
#40941=CARTESIAN_POINT('Ctrl Pts',(-0.192015409865108,0.00864506423045702,
0.00987737947917409));
#40942=CARTESIAN_POINT('Ctrl Pts',(-0.192020861696104,0.00856256927112993,
0.00988702574005904));
#40943=CARTESIAN_POINT('Ctrl Pts',(-0.192031955449212,0.00840095045736884,
0.00990472890594345));
#40944=CARTESIAN_POINT('Ctrl Pts',(-0.192054786510697,0.00809374315339341,
0.00993211432591152));
#40945=CARTESIAN_POINT('Ctrl Pts',(-0.192082412664333,0.00775366058309626,
0.00994830547279376));
#40946=CARTESIAN_POINT('Ctrl Pts',(-0.192104324882764,0.00749698449310426,
0.00994869951306347));
#40947=CARTESIAN_POINT('',(-0.192122489455637,0.00301997722274325,0.00881827773461044));
#40948=CARTESIAN_POINT('Ctrl Pts',(-0.192108700682526,0.00749526582339488,
0.0099487938961807));
#40949=CARTESIAN_POINT('Ctrl Pts',(-0.192103230217472,0.00744949681047625,
0.00994865204056603));
#40950=CARTESIAN_POINT('Ctrl Pts',(-0.192097918522563,0.00740368269194635,
0.00994818073646005));
#40951=CARTESIAN_POINT('Ctrl Pts',(-0.191981016723199,0.00636317794369435,
0.00992996660640991));
#40952=CARTESIAN_POINT('Ctrl Pts',(-0.191946332157474,0.00536896481747056,
0.00975679744953434));
#40953=CARTESIAN_POINT('Ctrl Pts',(-0.192015267591331,0.00393288153336258,
0.00926171219322835));
#40954=CARTESIAN_POINT('Ctrl Pts',(-0.192058801228599,0.00346626441370585,
0.00905753219206862));
#40955=CARTESIAN_POINT('Ctrl Pts',(-0.192122301842675,0.00301972304784883,
0.00881813661224312));
#40956=CARTESIAN_POINT('',(-0.191053639265561,0.00360252014973371,0.0090841498220513));
#40957=CARTESIAN_POINT('Ctrl Pts',(-0.192122489455637,0.00301997722274325,
0.00881827773461044));
#40958=CARTESIAN_POINT('Ctrl Pts',(-0.191991549101578,0.00306796965600734,
0.00884130847560521));
#40959=CARTESIAN_POINT('Ctrl Pts',(-0.191879858919587,0.00311067479627433,
0.00886139413752867));
#40960=CARTESIAN_POINT('Ctrl Pts',(-0.191781902301749,0.00315083974748719,
0.00888011500123793));
#40961=CARTESIAN_POINT('Ctrl Pts',(-0.191732037727987,0.00317128561645069,
0.00888964481055488));
#40962=CARTESIAN_POINT('Ctrl Pts',(-0.191685732156451,0.00319107891156394,
0.00889881027145093));
#40963=CARTESIAN_POINT('Ctrl Pts',(-0.191648801068625,0.00320716638729363,
0.00890622211943673));
#40964=CARTESIAN_POINT('Ctrl Pts',(-0.191611869980799,0.00322325386302332,
0.00891363396742254));
#40965=CARTESIAN_POINT('Ctrl Pts',(-0.191584312743833,0.00323562056547369,
0.00891932133001983));
#40966=CARTESIAN_POINT('Ctrl Pts',(-0.191542866130379,0.00325644619026458,
0.00892890116478443));
#40967=CARTESIAN_POINT('Ctrl Pts',(-0.191501419516925,0.00327727181505547,
0.00893848099954903));
#40968=CARTESIAN_POINT('Ctrl Pts',(-0.191446084656406,0.00330658260963377,
0.00895190132394306));
#40969=CARTESIAN_POINT('Ctrl Pts',(-0.19139762533046,0.0033347802690586,
0.00896471272346431));
#40970=CARTESIAN_POINT('Ctrl Pts',(-0.191349166004514,0.00336297792848342,
0.00897752412298555));
#40971=CARTESIAN_POINT('Ctrl Pts',(-0.191307581406187,0.00339004431685584,
0.00898976373818474));
#40972=CARTESIAN_POINT('Ctrl Pts',(-0.191267681664384,0.00341840149675534,
0.0090024944772828));
#40973=CARTESIAN_POINT('Ctrl Pts',(-0.19118788218078,0.00347511585655432,
0.00902795595547893));
#40974=CARTESIAN_POINT('Ctrl Pts',(-0.191114823138575,0.00353701496799355,
0.00905533519994708));
#40975=CARTESIAN_POINT('Ctrl Pts',(-0.191053698914977,0.00360175590961342,
0.00908336191387111));
#40976=CARTESIAN_POINT('',(-0.191108184220926,0.00749768564093594,0.00992694022012107));
#40977=CARTESIAN_POINT('Ctrl Pts',(-0.191051632810295,0.00360221947727921,
0.0090835271983084));
#40978=CARTESIAN_POINT('Ctrl Pts',(-0.191021186878507,0.00392206635238341,
0.00922786958441169));
#40979=CARTESIAN_POINT('Ctrl Pts',(-0.190999811324095,0.00425072879523787,
0.00935489154048301));
#40980=CARTESIAN_POINT('Ctrl Pts',(-0.19095367527545,0.00553194090199199,
0.00976957032772443));
#40981=CARTESIAN_POINT('Ctrl Pts',(-0.190993468703091,0.0065152661879122,
0.0099245060075464));
#40982=CARTESIAN_POINT('Ctrl Pts',(-0.191104699967524,0.00749947736827617,
0.00992697735777636));
#40983=CARTESIAN_POINT('Ctrl Pts',(-0.191108093501586,0.00749933750016912,
0.00992705109316002));
#40984=CARTESIAN_POINT('Ctrl Pts',(-0.191061680806587,0.00790407504383842,
0.00992607079981439));
#40985=CARTESIAN_POINT('Ctrl Pts',(-0.191027478698722,0.0083095718978316,
0.00989932465622092));
#40986=CARTESIAN_POINT('Ctrl Pts',(-0.190955876152719,0.00964018279270969,
0.00972531409106423));
#40987=CARTESIAN_POINT('Ctrl Pts',(-0.190972448810475,0.0105416572289866,
0.00946878822548761));
#40988=CARTESIAN_POINT('Ctrl Pts',(-0.191053991198766,0.0113881984379763,
0.00908791315351825));
#40989=CARTESIAN_POINT('Origin',(-0.228243019758013,0.0143258968887991,
-0.00627376866199084));
#40990=CARTESIAN_POINT('Origin',(-0.228011089022205,0.0141214482232033,
0.00627054897881623));
#40991=CARTESIAN_POINT('Ctrl Pts',(-0.204265073067,0.0127803686690591,-0.00856007647208766));
#40992=CARTESIAN_POINT('Ctrl Pts',(-0.204262729393093,0.0128387107088317,
-0.00864367908736358));
#40993=CARTESIAN_POINT('Ctrl Pts',(-0.204363894126176,0.0128284728860937,
-0.00865137065812417));
#40994=CARTESIAN_POINT('Ctrl Pts',(-0.204128064700356,0.0119492725903312,
-0.00913958927820265));
#40995=CARTESIAN_POINT('Ctrl Pts',(-0.204125477102728,0.011998566632778,
-0.00922956161310565));
#40996=CARTESIAN_POINT('Ctrl Pts',(-0.204226296468488,0.0119847835364124,
-0.00923756796894809));
#40997=CARTESIAN_POINT('Ctrl Pts',(-0.20384472208749,0.0100688601319156,
-0.0100298347632221));
#40998=CARTESIAN_POINT('Ctrl Pts',(-0.203841777898438,0.0100970878860094,
-0.0101297217092875));
#40999=CARTESIAN_POINT('Ctrl Pts',(-0.203944562018244,0.0100968720882839,
-0.010127895382756));
#41000=CARTESIAN_POINT('Ctrl Pts',(-0.20405840592736,0.00799378812699186,
-0.0102626707868758));
#41001=CARTESIAN_POINT('Ctrl Pts',(-0.204055334959227,0.00799938949731187,
-0.0103650911256359));
#41002=CARTESIAN_POINT('Ctrl Pts',(-0.204156746755187,0.00800979415998372,
-0.0103656374081853));
#41003=CARTESIAN_POINT('Ctrl Pts',(-0.204143725320899,0.00697638819353669,
-0.0102055690374362));
#41004=CARTESIAN_POINT('Ctrl Pts',(-0.204140678288162,0.00697055492621437,
-0.0103073359394314));
#41005=CARTESIAN_POINT('Ctrl Pts',(-0.204242317153123,0.00697890273577786,
-0.0103088949221699));
#41006=CARTESIAN_POINT('Ctrl Pts',(-0.204098738700262,0.00750019395234659,
-0.0102204142510564));
#41007=CARTESIAN_POINT('Ctrl Pts',(-0.204098590806404,0.00750019416653296,
-0.0102269583017623));
#41008=CARTESIAN_POINT('Ctrl Pts',(-0.204099088227802,0.00750019418365599,
-0.0102335006756741));
#41009=CARTESIAN_POINT('Ctrl Pts',(-0.204101430857704,0.00750019381893088,
-0.0102468030395632));
#41010=CARTESIAN_POINT('Ctrl Pts',(-0.204103353066049,0.00750019341260105,
-0.0102535132046417));
#41011=CARTESIAN_POINT('Ctrl Pts',(-0.204110778163236,0.00750019166647608,
-0.0102719147849014));
#41012=CARTESIAN_POINT('Ctrl Pts',(-0.204117865186854,0.00750018983664796,
-0.0102828141944625));
#41013=CARTESIAN_POINT('Ctrl Pts',(-0.204135782840589,0.0075001851440154,
-0.0103013364231896));
#41014=CARTESIAN_POINT('Ctrl Pts',(-0.204146447502616,0.00750018224294542,
-0.0103087848563091));
#41015=CARTESIAN_POINT('Ctrl Pts',(-0.204168356804244,0.00750017719045867,
-0.0103185177811627));
#41016=CARTESIAN_POINT('Ctrl Pts',(-0.204179152845045,0.0075001616685909,
-0.0103213085170776));
#41017=CARTESIAN_POINT('Ctrl Pts',(-0.204192375920369,0.00750018573349939,
-0.010322485851024));
#41018=CARTESIAN_POINT('Ctrl Pts',(-0.204194617299677,0.00750016630405051,
-0.0103226107361709));
#41019=CARTESIAN_POINT('Ctrl Pts',(-0.204196829921526,0.00750016559189676,
-0.0103226607415403));
#41020=CARTESIAN_POINT('Ctrl Pts',(-0.204181325032408,0.012257065641656,
-0.0089007774107484));
#41021=CARTESIAN_POINT('Ctrl Pts',(-0.204181296960589,0.0122609820637786,
-0.00890705005018559));
#41022=CARTESIAN_POINT('Ctrl Pts',(-0.204182202033119,0.0122655230269731,
-0.0089127959082597));
#41023=CARTESIAN_POINT('Ctrl Pts',(-0.204186011734323,0.0122765363438471,
-0.00892409037649733));
#41024=CARTESIAN_POINT('Ctrl Pts',(-0.204189199583018,0.0122830325026838,
-0.00892921331103979));
#41025=CARTESIAN_POINT('Ctrl Pts',(-0.204199541926441,0.0123005310075908,
-0.00894012819848833));
#41026=CARTESIAN_POINT('Ctrl Pts',(-0.204208309649517,0.0123124975679202,
-0.00894480621639041));
#41027=CARTESIAN_POINT('Ctrl Pts',(-0.204229550306519,0.0123373226808868,
-0.00894949032305491));
#41028=CARTESIAN_POINT('Ctrl Pts',(-0.204241261291575,0.0123493418130815,
-0.00894941000383247));
#41029=CARTESIAN_POINT('Ctrl Pts',(-0.204270868303184,0.0123769117862931,
-0.00894476547705386));
#41030=CARTESIAN_POINT('Ctrl Pts',(-0.204285432901854,0.0123881214336822,
-0.00893862798591079));
#41031=CARTESIAN_POINT('Ctrl Pts',(-0.204290480284829,0.0123917113386855,
-0.00893668244562294));
#41032=CARTESIAN_POINT('Ctrl Pts',(-0.204291371857698,0.012392496384385,
-0.0089362358274016));
#41033=CARTESIAN_POINT('Ctrl Pts',(-0.20429256803976,0.0123935448586381,
-0.00893563119921439));
#41034=CARTESIAN_POINT('Ctrl Pts',(-0.20429352351428,0.0123942615368791,
-0.00893520764733819));
#41035=CARTESIAN_POINT('Origin',(-0.204344423434958,0.012341683860884,-0.00885114476085288));
#41036=CARTESIAN_POINT('Ctrl Pts',(-0.203181004915558,0.0122576992722632,
-0.00887926075513702));
#41037=CARTESIAN_POINT('Ctrl Pts',(-0.203180880319866,0.0122616709335099,
-0.00888578894591877));
#41038=CARTESIAN_POINT('Ctrl Pts',(-0.203179990406391,0.0122663403805014,
-0.00889176162511392));
#41039=CARTESIAN_POINT('Ctrl Pts',(-0.203176628181342,0.012277395470525,
-0.00890301597230118));
#41040=CARTESIAN_POINT('Ctrl Pts',(-0.203174034602288,0.0122837777646263,
-0.00890801287099688));
#41041=CARTESIAN_POINT('Ctrl Pts',(-0.203165609250051,0.0123012757963656,
-0.00891867551477168));
#41042=CARTESIAN_POINT('Ctrl Pts',(-0.2031586136738,0.0123132348356185,
-0.00892310403449977));
#41043=CARTESIAN_POINT('Ctrl Pts',(-0.203142310649237,0.0123374075395989,
-0.00892703668417647));
#41044=CARTESIAN_POINT('Ctrl Pts',(-0.20313364719466,0.0123488884750934,
-0.00892677050332955));
#41045=CARTESIAN_POINT('Ctrl Pts',(-0.203113574189725,0.0123732482306594,
-0.00892228087227181));
#41046=CARTESIAN_POINT('Ctrl Pts',(-0.20310390248531,0.0123834505968482,
-0.00891756729833953));
#41047=CARTESIAN_POINT('Ctrl Pts',(-0.203096855974668,0.0123907471432063,
-0.00891357268518451));
#41048=CARTESIAN_POINT('Ctrl Pts',(-0.203094724720638,0.0123928548299233,
-0.00891238941300899));
#41049=CARTESIAN_POINT('Ctrl Pts',(-0.203092585205556,0.012394904002844,
-0.00891112094646253));
#41050=CARTESIAN_POINT('Ctrl Pts',(-0.203091800754282,0.0123956724650861,
-0.00891063229697375));
#41051=CARTESIAN_POINT('Ctrl Pts',(-0.204143997496444,0.00802323628381861,
-0.010205565063399));
#41052=CARTESIAN_POINT('Ctrl Pts',(-0.204140860611556,0.00802908085166497,
-0.0103074831625607));
#41053=CARTESIAN_POINT('Ctrl Pts',(-0.204242648149941,0.00802065830824136,
-0.0103089801716569));
#41054=CARTESIAN_POINT('Ctrl Pts',(-0.204058120672358,0.0070071871206502,
-0.0102622885094666));
#41055=CARTESIAN_POINT('Ctrl Pts',(-0.204054960205719,0.00700159695666881,
-0.0103648577443184));
#41056=CARTESIAN_POINT('Ctrl Pts',(-0.204156519163295,0.00699110367585506,
-0.0103653309638915));
#41057=CARTESIAN_POINT('Ctrl Pts',(-0.203843718954951,0.00493709923159828,
-0.0100315643925817));
#41058=CARTESIAN_POINT('Ctrl Pts',(-0.203840683456935,0.00490889608674471,
-0.0101316222849361));
#41059=CARTESIAN_POINT('Ctrl Pts',(-0.20394362305939,0.00490914794716083,
-0.0101297299846125));
#41060=CARTESIAN_POINT('Ctrl Pts',(-0.204127350940855,0.00305239049180689,
-0.00914022524378526));
#41061=CARTESIAN_POINT('Ctrl Pts',(-0.204124674731928,0.0030030291564167,
-0.00923033259386805));
#41062=CARTESIAN_POINT('Ctrl Pts',(-0.204225653522232,0.00301681463646749,
-0.00923826204389967));
#41063=CARTESIAN_POINT('Ctrl Pts',(-0.204263087479502,0.00222512775952759,
-0.00856364933328716));
#41064=CARTESIAN_POINT('Ctrl Pts',(-0.204260654022477,0.00216675058638386,
-0.00864741054064513));
#41065=CARTESIAN_POINT('Ctrl Pts',(-0.204361977315468,0.00217701080273715,
-0.00865502494961599));
#41066=CARTESIAN_POINT('Ctrl Pts',(-0.204292070928345,0.00260973041950684,
-0.00893764167137754));
#41067=CARTESIAN_POINT('Ctrl Pts',(-0.204291025482645,0.0026105155431871,
-0.00893810511839575));
#41068=CARTESIAN_POINT('Ctrl Pts',(-0.204288291638048,0.00261253468312918,
-0.00893925983789712));
#41069=CARTESIAN_POINT('Ctrl Pts',(-0.204285564855784,0.00261461434218402,
-0.00894033431311169));
#41070=CARTESIAN_POINT('Ctrl Pts',(-0.204276064531964,0.00262215153202754,
-0.00894413460675116));
#41071=CARTESIAN_POINT('Ctrl Pts',(-0.204263487933207,0.00263243098352953,
-0.0089483423375052));
#41072=CARTESIAN_POINT('Ctrl Pts',(-0.204238165020081,0.00265635914450468,
-0.00895184060040076));
#41073=CARTESIAN_POINT('Ctrl Pts',(-0.204227085909756,0.00266784811865962,
-0.00895174571839484));
#41074=CARTESIAN_POINT('Ctrl Pts',(-0.204206485960734,0.00269205167398984,
-0.00894702757360248));
#41075=CARTESIAN_POINT('Ctrl Pts',(-0.204197817017632,0.00270394972816067,
-0.00894230284157555));
#41076=CARTESIAN_POINT('Ctrl Pts',(-0.204187634236843,0.00272129696193903,
-0.00893136919571814));
#41077=CARTESIAN_POINT('Ctrl Pts',(-0.204184510539432,0.00272771010242592,
-0.00892627211040956));
#41078=CARTESIAN_POINT('Ctrl Pts',(-0.204180778308437,0.00273858477453516,
-0.00891506519824069));
#41079=CARTESIAN_POINT('Ctrl Pts',(-0.204179892226625,0.00274307102426783,
-0.00890937100289297));
#41080=CARTESIAN_POINT('Ctrl Pts',(-0.204179919702534,0.0027469445005241,
-0.00890316186212408));
#41081=CARTESIAN_POINT('Ctrl Pts',(-0.203143271812693,0.00698365837066073,
-0.0101836772736148));
#41082=CARTESIAN_POINT('Ctrl Pts',(-0.203141490914464,0.00697759707409294,
-0.0102900221295829));
#41083=CARTESIAN_POINT('Ctrl Pts',(-0.203035646026025,0.00696931019329735,
-0.0102810055802145));
#41084=CARTESIAN_POINT('Ctrl Pts',(-0.203057844304204,0.0080065505568688,
-0.0102395474721513));
#41085=CARTESIAN_POINT('Ctrl Pts',(-0.203056046122935,0.00801244156714122,
-0.0103465781511104));
#41086=CARTESIAN_POINT('Ctrl Pts',(-0.202950428971978,0.0080013749484015,
-0.0103385156607444));
#41087=CARTESIAN_POINT('Ctrl Pts',(-0.202848075368191,0.0100621302750322,
-0.0100051837092143));
#41088=CARTESIAN_POINT('Ctrl Pts',(-0.20284637539565,0.0100914860875319,
-0.0101095507090941));
#41089=CARTESIAN_POINT('Ctrl Pts',(-0.202739297675281,0.0100893700411261,
-0.0101043269775615));
#41090=CARTESIAN_POINT('Ctrl Pts',(-0.20312348077053,0.0119264298985161,
-0.00913154104380249));
#41091=CARTESIAN_POINT('Ctrl Pts',(-0.203122192521676,0.0119776612356224,
-0.00922571207633984));
#41092=CARTESIAN_POINT('Ctrl Pts',(-0.20301715666529,0.0119884333075752,
-0.0092108489932237));
#41093=CARTESIAN_POINT('Ctrl Pts',(-0.203261844553021,0.0127629120170625,
-0.00855350135677558));
#41094=CARTESIAN_POINT('Ctrl Pts',(-0.203260802723471,0.0128236026115707,
-0.00864104139382898));
#41095=CARTESIAN_POINT('Ctrl Pts',(-0.203155408062606,0.0128300897901739,
-0.00862693568704257));
#41096=CARTESIAN_POINT('Ctrl Pts',(-0.203101179356735,0.00746966964796713,
-0.0102067046864171));
#41097=CARTESIAN_POINT('Ctrl Pts',(-0.203099854724934,0.00747070927761228,
-0.0102176727827858));
#41098=CARTESIAN_POINT('Ctrl Pts',(-0.203096735385425,0.00747151343855428,
-0.0102283717733987));
#41099=CARTESIAN_POINT('Ctrl Pts',(-0.203086474952352,0.00747277282275856,
-0.010249734057713));
#41100=CARTESIAN_POINT('Ctrl Pts',(-0.203078924411847,0.00747318532340408,
-0.0102599911857472));
#41101=CARTESIAN_POINT('Ctrl Pts',(-0.203060454056968,0.00747281561145981,
-0.0102772439408748));
#41102=CARTESIAN_POINT('Ctrl Pts',(-0.203050700793186,0.00747201479849369,
-0.010283086345843));
#41103=CARTESIAN_POINT('Ctrl Pts',(-0.203036935787999,0.00746867281090778,
-0.0102893158064833));
#41104=CARTESIAN_POINT('Ctrl Pts',(-0.203031522359902,0.00746676460049837,
-0.0102911830158309));
#41105=CARTESIAN_POINT('Ctrl Pts',(-0.203026437789923,0.00746335128295609,
-0.0102925387461303));
#41106=CARTESIAN_POINT('Ctrl Pts',(-0.203025927392644,0.00746299355861727,
-0.0102926715115178));
#41107=CARTESIAN_POINT('Origin',(-0.203018630792398,0.0026610259015663,
-0.00882665770830219));
#41108=CARTESIAN_POINT('Ctrl Pts',(-0.20317320031072,0.00274689768611898,
-0.00888128997470166));
#41109=CARTESIAN_POINT('Ctrl Pts',(-0.203173025615196,0.00274389089988737,
-0.00888629384615075));
#41110=CARTESIAN_POINT('Ctrl Pts',(-0.203172429950494,0.00274045322122823,
-0.00889101255376211));
#41111=CARTESIAN_POINT('Ctrl Pts',(-0.20316959601839,0.00272971614503562,
-0.0089033005435487));
#41112=CARTESIAN_POINT('Ctrl Pts',(-0.203166494707998,0.00272180664330849,
-0.00890980481065451));
#41113=CARTESIAN_POINT('Ctrl Pts',(-0.203157477023721,0.00270296534417372,
-0.00892114361452894));
#41114=CARTESIAN_POINT('Ctrl Pts',(-0.2031511876556,0.00269197143508385,
-0.00892515254381942));
#41115=CARTESIAN_POINT('Ctrl Pts',(-0.203133615926001,0.00266420206416287,
-0.00893042371830774));
#41116=CARTESIAN_POINT('Ctrl Pts',(-0.203122454277358,0.00264914254816469,
-0.00892877786070083));
#41117=CARTESIAN_POINT('Ctrl Pts',(-0.203109312459774,0.00263034302082137,
-0.00892395358816016));
#41118=CARTESIAN_POINT('Ctrl Pts',(-0.203104868123276,0.00262369280401741,
-0.00892137703935346));
#41119=CARTESIAN_POINT('Ctrl Pts',(-0.203101838781183,0.00261554887056482,
-0.00891742625592927));
#41120=CARTESIAN_POINT('Ctrl Pts',(-0.203101402755506,0.00261337739142643,
-0.0089162616978424));
#41121=CARTESIAN_POINT('Ctrl Pts',(-0.203101377855557,0.00261069939040457,
-0.00891472500874586));
#41122=CARTESIAN_POINT('Ctrl Pts',(-0.203101415214044,0.0026100532038125,
-0.00891434527384206));
#41123=CARTESIAN_POINT('Ctrl Pts',(-0.203101497042113,0.00260941164989306,
-0.00891395940072847));
#41124=CARTESIAN_POINT('Origin',(-0.206699882182129,0.00706535101846166,
-0.00270713639773735));
#41125=CARTESIAN_POINT('Ctrl Pts',(-0.206265373707575,0.0127777966478479,
-0.00859997364655191));
#41126=CARTESIAN_POINT('Ctrl Pts',(-0.20626304639632,0.012836204592148,
-0.00868330038990975));
#41127=CARTESIAN_POINT('Ctrl Pts',(-0.206364024979952,0.0128261001065475,
-0.00869114028853961));
#41128=CARTESIAN_POINT('Ctrl Pts',(-0.206129048262261,0.011947813807502,
-0.00918129811142922));
#41129=CARTESIAN_POINT('Ctrl Pts',(-0.206126478296519,0.0119971744172948,
-0.00927102308516758));
#41130=CARTESIAN_POINT('Ctrl Pts',(-0.206227111583568,0.0119835677514146,
-0.00927917721234948));
#41131=CARTESIAN_POINT('Ctrl Pts',(-0.205843113708995,0.0100692150364398,
-0.0100742796343862));
#41132=CARTESIAN_POINT('Ctrl Pts',(-0.205840189802564,0.0100974870119682,
-0.0101739681899843));
#41133=CARTESIAN_POINT('Ctrl Pts',(-0.205942785236712,0.0100970730771734,
-0.0101723622736461));
#41134=CARTESIAN_POINT('Ctrl Pts',(-0.206056905618493,0.00799330463484866,
-0.010308040249357));
#41135=CARTESIAN_POINT('Ctrl Pts',(-0.206053854566429,0.00799891449469382,
-0.0104102754427349));
#41136=CARTESIAN_POINT('Ctrl Pts',(-0.206155065185868,0.00800948684235285,
-0.0104109713944681));
#41137=CARTESIAN_POINT('Ctrl Pts',(-0.206143839207489,0.00697634899411554,
-0.0102507166129379));
#41138=CARTESIAN_POINT('Ctrl Pts',(-0.206140812015937,0.0069705060182345,
-0.0103522948486019));
#41139=CARTESIAN_POINT('Ctrl Pts',(-0.206242251803155,0.00697892476553575,
-0.0103540372485459));
#41140=CARTESIAN_POINT('Ctrl Pts',(-0.206098147225107,0.00750010495671034,
-0.0102656023871143));
#41141=CARTESIAN_POINT('Ctrl Pts',(-0.20609799932479,0.00750010511644564,
-0.0102721467492724));
#41142=CARTESIAN_POINT('Ctrl Pts',(-0.206098496860782,0.00750010510170206,
-0.0102786894234506));
#41143=CARTESIAN_POINT('Ctrl Pts',(-0.206100839967226,0.00750010471944094,
-0.010291992420886));
#41144=CARTESIAN_POINT('Ctrl Pts',(-0.20610276255874,0.0075001043305413,
-0.0102987028842377));
#41145=CARTESIAN_POINT('Ctrl Pts',(-0.20611018892991,0.00750010270993599,
-0.010317104869771));
#41146=CARTESIAN_POINT('Ctrl Pts',(-0.206117276936597,0.00750010105092799,
-0.0103280041761893));
#41147=CARTESIAN_POINT('Ctrl Pts',(-0.206135196697436,0.00750009687187179,
-0.0103465261516109));
#41148=CARTESIAN_POINT('Ctrl Pts',(-0.206145862546723,0.00750009430132802,
-0.0103539743426226));
#41149=CARTESIAN_POINT('Ctrl Pts',(-0.206167775052211,0.00750009006200001,
-0.0103637073224297));
#41150=CARTESIAN_POINT('Ctrl Pts',(-0.206178571379276,0.00750007378825076,
-0.0103664970753006));
#41151=CARTESIAN_POINT('Ctrl Pts',(-0.206191789970321,0.00750010082790921,
-0.0103676740516232));
#41152=CARTESIAN_POINT('Ctrl Pts',(-0.206194036900753,0.00750007978106561,
-0.0103677992460968));
#41153=CARTESIAN_POINT('Ctrl Pts',(-0.206196247266376,0.00750007914373993,
-0.0103678492117139));
#41154=CARTESIAN_POINT('Ctrl Pts',(-0.206181817694621,0.0122551267607735,
-0.00894171598702609));
#41155=CARTESIAN_POINT('Ctrl Pts',(-0.20618178860154,0.0122590539690899,
-0.00894798079528798));
#41156=CARTESIAN_POINT('Ctrl Pts',(-0.206182692488116,0.0122636047879427,
-0.00895371774478208));
#41157=CARTESIAN_POINT('Ctrl Pts',(-0.206186498221275,0.0122746343758503,
-0.00896498778296844));
#41158=CARTESIAN_POINT('Ctrl Pts',(-0.206189682130124,0.0122811357191452,
-0.00897009628597565));
#41159=CARTESIAN_POINT('Ctrl Pts',(-0.206200014724264,0.0122986475116484,
-0.00898097783826835));
#41160=CARTESIAN_POINT('Ctrl Pts',(-0.206208776639363,0.0123106204169374,
-0.00898563506172976));
#41161=CARTESIAN_POINT('Ctrl Pts',(-0.206229865025598,0.0123352875681986,
-0.00899024734596498));
#41162=CARTESIAN_POINT('Ctrl Pts',(-0.206241398738038,0.0123471495980202,
-0.0089901803069501));
#41163=CARTESIAN_POINT('Ctrl Pts',(-0.206270681041155,0.0123744968585233,
-0.00898565892481136));
#41164=CARTESIAN_POINT('Ctrl Pts',(-0.206285145158284,0.0123856175724812,
-0.00897964283157976));
#41165=CARTESIAN_POINT('Ctrl Pts',(-0.206290134239438,0.012389286123914,
-0.00897768187932079));
#41166=CARTESIAN_POINT('Ctrl Pts',(-0.206291280718472,0.0123902435954362,
-0.00897714552013086));
#41167=CARTESIAN_POINT('Ctrl Pts',(-0.206292817844583,0.0123915197022351,
-0.00897641524707116));
#41168=CARTESIAN_POINT('Ctrl Pts',(-0.206294013519307,0.0123924158224524,
-0.00897588334166704));
#41169=CARTESIAN_POINT('Origin',(-0.206344964115316,0.0123396857707647,
-0.0088919177026923));
#41170=CARTESIAN_POINT('Ctrl Pts',(-0.205181552286433,0.0122555409350824,
-0.00892029894995692));
#41171=CARTESIAN_POINT('Ctrl Pts',(-0.205181427582414,0.0122595243991831,
-0.00892681884907278));
#41172=CARTESIAN_POINT('Ctrl Pts',(-0.205180537761043,0.012264204315227,
-0.00893278217335894));
#41173=CARTESIAN_POINT('Ctrl Pts',(-0.205177176102581,0.01227527836818,
-0.00894401489787914));
#41174=CARTESIAN_POINT('Ctrl Pts',(-0.205174583048941,0.0122816686296184,
-0.0089489997063002));
#41175=CARTESIAN_POINT('Ctrl Pts',(-0.20516615887642,0.0122991836084092,
-0.00895963048145717));
#41176=CARTESIAN_POINT('Ctrl Pts',(-0.205159163971388,0.012311149055828,
-0.008964037697506));
#41177=CARTESIAN_POINT('Ctrl Pts',(-0.205142860944653,0.0123353268288297,
-0.008967928075468));
#41178=CARTESIAN_POINT('Ctrl Pts',(-0.205134196499638,0.0123468070286007,
-0.00896764154323951));
#41179=CARTESIAN_POINT('Ctrl Pts',(-0.205114342718288,0.0123708879580858,
-0.00896315819011513));
#41180=CARTESIAN_POINT('Ctrl Pts',(-0.205104622989719,0.0123811700400964,
-0.00895847447913059));
#41181=CARTESIAN_POINT('Ctrl Pts',(-0.205097384650215,0.0123886506823329,
-0.00895436076088045));
#41182=CARTESIAN_POINT('Ctrl Pts',(-0.205095267860903,0.0123907425138203,
-0.00895318017659277));
#41183=CARTESIAN_POINT('Ctrl Pts',(-0.205093143040606,0.0123927769598421,
-0.00895191630922259));
#41184=CARTESIAN_POINT('Ctrl Pts',(-0.205092344163379,0.0123935584157556,
-0.00895141728292034));
#41185=CARTESIAN_POINT('Ctrl Pts',(-0.206144103513576,0.00802320152732896,
-0.0102507274525613));
#41186=CARTESIAN_POINT('Ctrl Pts',(-0.206140997950459,0.00802904586778321,
-0.010352306059325));
#41187=CARTESIAN_POINT('Ctrl Pts',(-0.206242434213696,0.00802058399184559,
-0.0103541294277887));
#41188=CARTESIAN_POINT('Ctrl Pts',(-0.206056579512448,0.00700735013193967,
-0.0103076580428027));
#41189=CARTESIAN_POINT('Ctrl Pts',(-0.206053450453671,0.00700175551739084,
-0.0104098901160137));
#41190=CARTESIAN_POINT('Ctrl Pts',(-0.206154656804463,0.00699109309901565,
-0.0104106529954126));
#41191=CARTESIAN_POINT('Ctrl Pts',(-0.205842609607531,0.00493647513741988,
-0.0100759677680453));
#41192=CARTESIAN_POINT('Ctrl Pts',(-0.205839605792459,0.00490826674460647,
-0.0101756783187804));
#41193=CARTESIAN_POINT('Ctrl Pts',(-0.205942200979761,0.00490877422186876,
-0.0101741790754591));
#41194=CARTESIAN_POINT('Ctrl Pts',(-0.206129004920361,0.00305341025745715,
-0.00918172589817647));
#41195=CARTESIAN_POINT('Ctrl Pts',(-0.206126357176411,0.00300405160961498,
-0.00927145037743672));
#41196=CARTESIAN_POINT('Ctrl Pts',(-0.206226999266609,0.00301755440218435,
-0.00927963958615716));
#41197=CARTESIAN_POINT('Ctrl Pts',(-0.206264033249047,0.0022273051379683,
-0.00860330356791341));
#41198=CARTESIAN_POINT('Ctrl Pts',(-0.206261626670221,0.00216894495741129,
-0.00868666242678945));
#41199=CARTESIAN_POINT('Ctrl Pts',(-0.206362612710959,0.00217897942055083,
-0.00869453476898776));
#41200=CARTESIAN_POINT('Ctrl Pts',(-0.206293209986791,0.00261116835746199,
-0.0089780881565586));
#41201=CARTESIAN_POINT('Ctrl Pts',(-0.206292152439964,0.00261196180857207,
-0.00897855861405994));
#41202=CARTESIAN_POINT('Ctrl Pts',(-0.206289430497985,0.00261397171563914,
-0.00897971274745204));
#41203=CARTESIAN_POINT('Ctrl Pts',(-0.206286715821411,0.00261604111206668,
-0.00898078772033416));
#41204=CARTESIAN_POINT('Ctrl Pts',(-0.206277145814662,0.00262362445694192,
-0.00898462953548511));
#41205=CARTESIAN_POINT('Ctrl Pts',(-0.206264610353204,0.0026338711059093,
-0.0089888332769248));
#41206=CARTESIAN_POINT('Ctrl Pts',(-0.206239352438,0.00265772908183957,
-0.00899237788634536));
#41207=CARTESIAN_POINT('Ctrl Pts',(-0.206228282712326,0.00266920622605173,
-0.00899231142454711));
#41208=CARTESIAN_POINT('Ctrl Pts',(-0.206207676314294,0.00269341580046527,
-0.0089876600294395));
#41209=CARTESIAN_POINT('Ctrl Pts',(-0.206198995732441,0.0027053325979369,
-0.0089829638682279));
#41210=CARTESIAN_POINT('Ctrl Pts',(-0.206188794293892,0.00272272036421045,
-0.00897206573525393));
#41211=CARTESIAN_POINT('Ctrl Pts',(-0.206185663094497,0.00272915354208732,
-0.00896697788736482));
#41212=CARTESIAN_POINT('Ctrl Pts',(-0.206181921166814,0.00274006870319551,
-0.00895577915139813));
#41213=CARTESIAN_POINT('Ctrl Pts',(-0.206181032892529,0.00274457413552852,
-0.00895008469635413));
#41214=CARTESIAN_POINT('Ctrl Pts',(-0.206181061337296,0.00274846569215316,
-0.00894387223338268));
#41215=CARTESIAN_POINT('Ctrl Pts',(-0.205142482088579,0.00699220996088759,
-0.0102293438807348));
#41216=CARTESIAN_POINT('Ctrl Pts',(-0.205140639337482,0.00698620356045466,
-0.0103359908107351));
#41217=CARTESIAN_POINT('Ctrl Pts',(-0.205034537097864,0.00697779962238244,
-0.0103265903532839));
#41218=CARTESIAN_POINT('Ctrl Pts',(-0.205055686601309,0.00801208405484312,
-0.0102842507443711));
#41219=CARTESIAN_POINT('Ctrl Pts',(-0.205053827163856,0.00801807257933057,
-0.0103915774312491));
#41220=CARTESIAN_POINT('Ctrl Pts',(-0.204947949614617,0.00800680784218544,
-0.0103831666819726));
#41221=CARTESIAN_POINT('Ctrl Pts',(-0.204846824706544,0.01006416746964,
-0.0100486295602955));
#41222=CARTESIAN_POINT('Ctrl Pts',(-0.204845062847581,0.0100937289998733,
-0.0101532635178354));
#41223=CARTESIAN_POINT('Ctrl Pts',(-0.204737712388477,0.0100917772942086,
-0.0101476164771957));
#41224=CARTESIAN_POINT('Ctrl Pts',(-0.205124477129889,0.0119248241379215,
-0.00917343580602142));
#41225=CARTESIAN_POINT('Ctrl Pts',(-0.20512312749823,0.011976373863991,
-0.00926778133092942));
#41226=CARTESIAN_POINT('Ctrl Pts',(-0.205017823077147,0.0119869252156459,
-0.00925255879414128));
#41227=CARTESIAN_POINT('Ctrl Pts',(-0.205262235724447,0.012760158868421,
-0.00859356109315354));
#41228=CARTESIAN_POINT('Ctrl Pts',(-0.205261132004666,0.0128212089278307,
-0.00868121456209581));
#41229=CARTESIAN_POINT('Ctrl Pts',(-0.205155466933443,0.0128274850701372,
-0.00866676438333058));
#41230=CARTESIAN_POINT('Ctrl Pts',(-0.205098440011371,0.00750015035561199,
-0.0102432542980132));
#41231=CARTESIAN_POINT('Ctrl Pts',(-0.205098278016604,0.00750015055076414,
-0.0102497158135366));
#41232=CARTESIAN_POINT('Ctrl Pts',(-0.205097487561935,0.00750015091686855,
-0.0102561461143775));
#41233=CARTESIAN_POINT('Ctrl Pts',(-0.205094563933792,0.00750015203413857,
-0.0102692494005583));
#41234=CARTESIAN_POINT('Ctrl Pts',(-0.205092340334007,0.00750015280942587,
-0.0102758660159279));
#41235=CARTESIAN_POINT('Ctrl Pts',(-0.205084090834935,0.00750015556900989,
-0.0102939134832974));
#41236=CARTESIAN_POINT('Ctrl Pts',(-0.205076518175416,0.0075001579817565,
-0.0103044814708938));
#41237=CARTESIAN_POINT('Ctrl Pts',(-0.205057781000493,0.00750016407237376,
-0.0103221751119802));
#41238=CARTESIAN_POINT('Ctrl Pts',(-0.205046790114734,0.00750016753939868,
-0.0103291339882119));
#41239=CARTESIAN_POINT('Ctrl Pts',(-0.205023489197286,0.00750017683211112,
-0.0103382475058349));
#41240=CARTESIAN_POINT('Ctrl Pts',(-0.205012454789772,0.00750016099293299,
-0.0103402131205683));
#41241=CARTESIAN_POINT('Ctrl Pts',(-0.205000340687757,0.00750021268667578,
-0.0103407434268609));
#41242=CARTESIAN_POINT('Ctrl Pts',(-0.204998015689761,0.00750017802011827,
-0.0103407682740367));
#41243=CARTESIAN_POINT('Ctrl Pts',(-0.204995840626232,0.00750017862353099,
-0.010340719315994));
#41244=CARTESIAN_POINT('Origin',(-0.20501976771991,0.00266278717579714,
-0.00886724406818112));
#41245=CARTESIAN_POINT('Ctrl Pts',(-0.205180471484369,0.00274828496058784,
-0.00892259092201156));
#41246=CARTESIAN_POINT('Ctrl Pts',(-0.205180344443188,0.00274423647563211,
-0.00892922577511845));
#41247=CARTESIAN_POINT('Ctrl Pts',(-0.205179425306355,0.0027394680149155,
-0.00893528377307584));
#41248=CARTESIAN_POINT('Ctrl Pts',(-0.20517595033189,0.00272816290128792,
-0.00894667609632815));
#41249=CARTESIAN_POINT('Ctrl Pts',(-0.205173267608394,0.00272163074259415,
-0.00895171169464386));
#41250=CARTESIAN_POINT('Ctrl Pts',(-0.205164629939474,0.00270387175476733,
-0.00896230741493743));
#41251=CARTESIAN_POINT('Ctrl Pts',(-0.205157518531435,0.00269181197528201,
-0.0089666338369735));
#41252=CARTESIAN_POINT('Ctrl Pts',(-0.205140876756943,0.00266732113900677,
-0.00897034072357252));
#41253=CARTESIAN_POINT('Ctrl Pts',(-0.205131972362909,0.00265562604229162,
-0.00896989952403503));
#41254=CARTESIAN_POINT('Ctrl Pts',(-0.205109001760081,0.00262806363961682,
-0.00896432066061317));
#41255=CARTESIAN_POINT('Ctrl Pts',(-0.205097770882948,0.00261689896753867,
-0.00895770506605427));
#41256=CARTESIAN_POINT('Ctrl Pts',(-0.205093772027569,0.00261306844039898,
-0.00895550370242417));
#41257=CARTESIAN_POINT('Ctrl Pts',(-0.205092571930731,0.00261162363512667,
-0.00895462460683516));
#41258=CARTESIAN_POINT('Ctrl Pts',(-0.205091223366067,0.00261030520999543,
-0.00895378355642604));
#41259=CARTESIAN_POINT('Ctrl Pts',(-0.205260955479136,0.00224264774500391,
-0.0085954366889458));
#41260=CARTESIAN_POINT('Ctrl Pts',(-0.20526001140994,0.00218180944454979,
-0.00868289007491256));
#41261=CARTESIAN_POINT('Ctrl Pts',(-0.205154592360999,0.00217532007259305,
-0.00866886906021484));
#41262=CARTESIAN_POINT('Ctrl Pts',(-0.205123528174581,0.00308109440095735,
-0.00917641256757719));
#41263=CARTESIAN_POINT('Ctrl Pts',(-0.205122337805058,0.00302977228761021,
-0.00927055314944947));
#41264=CARTESIAN_POINT('Ctrl Pts',(-0.205017275753863,0.00301909471955522,
-0.00925579939875452));
#41265=CARTESIAN_POINT('Ctrl Pts',(-0.20484613965658,0.00493748613428339,
-0.0100487096525008));
#41266=CARTESIAN_POINT('Ctrl Pts',(-0.204844542660311,0.0049080243327645,
-0.0101530627638109));
#41267=CARTESIAN_POINT('Ctrl Pts',(-0.204737444299667,0.00490974190000643,
-0.0101478430648011));
#41268=CARTESIAN_POINT('Ctrl Pts',(-0.205055811865902,0.00699451686999224,
-0.0102849389073442));
#41269=CARTESIAN_POINT('Ctrl Pts',(-0.205054115345084,0.00698860532580391,
-0.0103919880796032));
#41270=CARTESIAN_POINT('Ctrl Pts',(-0.204948496773928,0.00699993329614755,
-0.0103840506703114));
#41271=CARTESIAN_POINT('Ctrl Pts',(-0.205143562118305,0.00801654945543371,
-0.0102286679529194));
#41272=CARTESIAN_POINT('Ctrl Pts',(-0.205141882892494,0.00802262912478596,
-0.0103350243606254));
#41273=CARTESIAN_POINT('Ctrl Pts',(-0.20503603371479,0.00803106429285927,
-0.0103260782815921));
#41274=CARTESIAN_POINT('Ctrl Pts',(-0.208254443206528,0.0127067297690959,
-0.00868853043591179));
#41275=CARTESIAN_POINT('Ctrl Pts',(-0.208252817177365,0.0127639831859331,
-0.00877159573976323));
#41276=CARTESIAN_POINT('Ctrl Pts',(-0.208352886496751,0.0127538205857698,
-0.00877954740891872));
#41277=CARTESIAN_POINT('Ctrl Pts',(-0.208122153160708,0.0118948116780756,
-0.00924830039922951));
#41278=CARTESIAN_POINT('Ctrl Pts',(-0.208120294425605,0.0119432213060983,
-0.00933749997466366));
#41279=CARTESIAN_POINT('Ctrl Pts',(-0.208220100686766,0.0119302505900155,
-0.00934548024255124));
#41280=CARTESIAN_POINT('Ctrl Pts',(-0.207848482421744,0.0100670043687399,
-0.010110433671947));
#41281=CARTESIAN_POINT('Ctrl Pts',(-0.207846300193864,0.0100950982407419,
-0.0102091369504758));
#41282=CARTESIAN_POINT('Ctrl Pts',(-0.207947953070991,0.0100944347762669,
-0.0102079379981602));
#41283=CARTESIAN_POINT('Ctrl Pts',(-0.208049545050965,0.00805000192234531,
-0.0103475054232749));
#41284=CARTESIAN_POINT('Ctrl Pts',(-0.208047228055695,0.00805628014436581,
-0.0104487912651243));
#41285=CARTESIAN_POINT('Ctrl Pts',(-0.208147577167768,0.00806662809390711,
-0.0104495775820796));
#41286=CARTESIAN_POINT('Ctrl Pts',(-0.208136501793819,0.00706036444276593,
-0.0103009087163086));
#41287=CARTESIAN_POINT('Ctrl Pts',(-0.208134205125068,0.00705555198922157,
-0.0104016678523864));
#41288=CARTESIAN_POINT('Ctrl Pts',(-0.208234728401044,0.00706414444257922,
-0.0104034975501504));
#41289=CARTESIAN_POINT('Ctrl Pts',(-0.208097499489004,0.00749999845002932,
-0.0103107892565932));
#41290=CARTESIAN_POINT('Ctrl Pts',(-0.208097351583086,0.00749999854583129,
-0.0103173339068719));
#41291=CARTESIAN_POINT('Ctrl Pts',(-0.208097849227417,0.00749999849669942,
-0.0103238768584556));
#41292=CARTESIAN_POINT('Ctrl Pts',(-0.20810019278319,0.00749999810609638,
-0.0103371804420943));
#41293=CARTESIAN_POINT('Ctrl Pts',(-0.208102115735706,0.00749999774723053,
-0.0103438911809762));
#41294=CARTESIAN_POINT('Ctrl Pts',(-0.20810954331178,0.00749999630993762,
-0.0103622935486121));
#41295=CARTESIAN_POINT('Ctrl Pts',(-0.208116632253359,0.00749999488489928,
-0.0103731927605778));
#41296=CARTESIAN_POINT('Ctrl Pts',(-0.20813455402164,0.00749999139152034,
-0.0103917145053224));
#41297=CARTESIAN_POINT('Ctrl Pts',(-0.208145221004457,0.00749998925827104,
-0.0103991624716254));
#41298=CARTESIAN_POINT('Ctrl Pts',(-0.208167136994736,0.00749998606736913,
-0.0104088957045982));
#41299=CARTESIAN_POINT('Ctrl Pts',(-0.208177933625618,0.00749996906351887,
-0.0104116843695746));
#41300=CARTESIAN_POINT('Ctrl Pts',(-0.208191146848798,0.00749999943002881,
-0.0104128609239724));
#41301=CARTESIAN_POINT('Ctrl Pts',(-0.208193400306433,0.00749997664853401,
-0.0104129864827718));
#41302=CARTESIAN_POINT('Ctrl Pts',(-0.208195607948066,0.00749997611037837,
-0.0104130363984175));
#41303=CARTESIAN_POINT('Ctrl Pts',(-0.208182322531234,0.0122530850694677,
-0.00898281054933035));
#41304=CARTESIAN_POINT('Ctrl Pts',(-0.20818229260496,0.012257023594431,
-0.00898906876229917));
#41305=CARTESIAN_POINT('Ctrl Pts',(-0.208183195803744,0.0122615849103819,
-0.00899479795224621));
#41306=CARTESIAN_POINT('Ctrl Pts',(-0.208186999470675,0.0122726329544399,
-0.00900604646900106));
#41307=CARTESIAN_POINT('Ctrl Pts',(-0.208190181165405,0.0122791411220139,
-0.00901114196751426));
#41308=CARTESIAN_POINT('Ctrl Pts',(-0.208200508351318,0.0122966686441179,
-0.00902199162142199));
#41309=CARTESIAN_POINT('Ctrl Pts',(-0.208209267046805,0.0123086484551155,
-0.0090266281316795));
#41310=CARTESIAN_POINT('Ctrl Pts',(-0.208230283270831,0.0123332452203376,
-0.00903118464895189));
#41311=CARTESIAN_POINT('Ctrl Pts',(-0.208241733956362,0.0123450335003312,
-0.00903111298954677));
#41312=CARTESIAN_POINT('Ctrl Pts',(-0.208265092839061,0.0123668754193094,
-0.00902751311489447));
#41313=CARTESIAN_POINT('Ctrl Pts',(-0.208277074431209,0.0123772611298929,
-0.00902388967657451));
#41314=CARTESIAN_POINT('Ctrl Pts',(-0.208291136593539,0.0123877056522628,
-0.00901833269169697));
#41315=CARTESIAN_POINT('Ctrl Pts',(-0.208292766707618,0.012389140227029,
-0.00901750873668517));
#41316=CARTESIAN_POINT('Ctrl Pts',(-0.208294512702006,0.0123904475468134,
-0.00901672948361178));
#41317=CARTESIAN_POINT('Origin',(-0.208345496545884,0.0123375625807303,
-0.00893286285957864));
#41318=CARTESIAN_POINT('Ctrl Pts',(-0.207182081101986,0.0122534241571154,
-0.00896140352867932));
#41319=CARTESIAN_POINT('Ctrl Pts',(-0.207181956278481,0.0122574195556349,
-0.00896791580190798));
#41320=CARTESIAN_POINT('Ctrl Pts',(-0.207181066392585,0.012262110300776,
-0.0089738702636863));
#41321=CARTESIAN_POINT('Ctrl Pts',(-0.207177704706269,0.0122732045720034,
-0.0089850821673224));
#41322=CARTESIAN_POINT('Ctrl Pts',(-0.20717511169926,0.0122796037032122,
-0.00899005505969755));
#41323=CARTESIAN_POINT('Ctrl Pts',(-0.207166687657127,0.0122971375010644,
-0.00900065342756414));
#41324=CARTESIAN_POINT('Ctrl Pts',(-0.207159692854611,0.0123091105651382,
-0.00900503864248638));
#41325=CARTESIAN_POINT('Ctrl Pts',(-0.207143389299496,0.0123332953216799,
-0.00900888483866729));
#41326=CARTESIAN_POINT('Ctrl Pts',(-0.207134724148054,0.0123447752724386,
-0.00900857713229437));
#41327=CARTESIAN_POINT('Ctrl Pts',(-0.207114897742302,0.0123688127376833,
-0.00900405570779137));
#41328=CARTESIAN_POINT('Ctrl Pts',(-0.207105192569871,0.0123790762651988,
-0.00899937093567547));
#41329=CARTESIAN_POINT('Ctrl Pts',(-0.207097899951547,0.0123866015335837,
-0.00899521430276797));
#41330=CARTESIAN_POINT('Ctrl Pts',(-0.207095791256553,0.0123886836581939,
-0.00899403346105137));
#41331=CARTESIAN_POINT('Ctrl Pts',(-0.207093674671486,0.0123907089793412,
-0.0089927704541225));
#41332=CARTESIAN_POINT('Ctrl Pts',(-0.207092867603371,0.0123914974180721,
-0.0089922648645807));
#41333=CARTESIAN_POINT('Ctrl Pts',(-0.208143344830797,0.00801431535345852,
-0.0102963203625224));
#41334=CARTESIAN_POINT('Ctrl Pts',(-0.208140201657287,0.00802007540567886,
-0.010397751642749));
#41335=CARTESIAN_POINT('Ctrl Pts',(-0.208241474571592,0.00801153714660289,
-0.0103997680387923));
#41336=CARTESIAN_POINT('Ctrl Pts',(-0.208054400162267,0.00700150192641365,
-0.0103522839259218));
#41337=CARTESIAN_POINT('Ctrl Pts',(-0.208051234145549,0.00699583305844126,
-0.0104543596381036));
#41338=CARTESIAN_POINT('Ctrl Pts',(-0.208152281685006,0.00698503643943993,
-0.010455282128268));
#41339=CARTESIAN_POINT('Ctrl Pts',(-0.207845968693388,0.00497123137684409,
-0.0101233193244587));
#41340=CARTESIAN_POINT('Ctrl Pts',(-0.207842924905438,0.00494334863064471,
-0.0102228997512816));
#41341=CARTESIAN_POINT('Ctrl Pts',(-0.207945339089887,0.00494393007860572,
-0.0102217144919219));
#41342=CARTESIAN_POINT('Ctrl Pts',(-0.208120104371585,0.00312365367681334,
-0.00925598171762431));
#41343=CARTESIAN_POINT('Ctrl Pts',(-0.208117403181981,0.00307499116185933,
-0.00934585701471216));
#41344=CARTESIAN_POINT('Ctrl Pts',(-0.208217967734135,0.00308783281510984,
-0.00935385714742386));
#41345=CARTESIAN_POINT('Ctrl Pts',(-0.208250100050302,0.0023208742329109,
-0.00870641445993126));
#41346=CARTESIAN_POINT('Ctrl Pts',(-0.208247627110399,0.00226341898325691,
-0.00879022115099646));
#41347=CARTESIAN_POINT('Ctrl Pts',(-0.20834843066501,0.00227365595662788,
-0.0087982762741702));
#41348=CARTESIAN_POINT('Ctrl Pts',(-0.208294284391964,0.0026126423899481,
-0.00901864750601907));
#41349=CARTESIAN_POINT('Ctrl Pts',(-0.208293221456411,0.00261343900871228,
-0.00901912190356573));
#41350=CARTESIAN_POINT('Ctrl Pts',(-0.208290504841601,0.0026154435033703,
-0.00902027778717965));
#41351=CARTESIAN_POINT('Ctrl Pts',(-0.208287795713521,0.00261750700095301,
-0.00902135499508675));
#41352=CARTESIAN_POINT('Ctrl Pts',(-0.20827819847105,0.00262510339882467,
-0.00902522144578501));
#41353=CARTESIAN_POINT('Ctrl Pts',(-0.208265689525886,0.00263532392112371,
-0.00902943085794375));
#41354=CARTESIAN_POINT('Ctrl Pts',(-0.208240476225512,0.0026591282377444,
-0.00903302185679735));
#41355=CARTESIAN_POINT('Ctrl Pts',(-0.208229416121853,0.0026705920051928,
-0.0090329825727401));
#41356=CARTESIAN_POINT('Ctrl Pts',(-0.208208803468976,0.00269480468142731,
-0.00902839576330975));
#41357=CARTESIAN_POINT('Ctrl Pts',(-0.208200111195092,0.00270673906414479,
-0.00902372721040564));
#41358=CARTESIAN_POINT('Ctrl Pts',(-0.208189890950813,0.00272416595776656,
-0.00901286328082817));
#41359=CARTESIAN_POINT('Ctrl Pts',(-0.208186752219044,0.00273061869531979,
-0.00900778421126741));
#41360=CARTESIAN_POINT('Ctrl Pts',(-0.208183000720674,0.00274157311829964,
-0.008996593520968));
#41361=CARTESIAN_POINT('Ctrl Pts',(-0.208182110252984,0.00274609707774618,
-0.00899089919268803));
#41362=CARTESIAN_POINT('Ctrl Pts',(-0.208182139477677,0.00275000626856638,
-0.00898468398557736));
#41363=CARTESIAN_POINT('Ctrl Pts',(-0.207142447083897,0.006992183093808,
-0.0102750218786083));
#41364=CARTESIAN_POINT('Ctrl Pts',(-0.20714006707363,0.00698616230337856,
-0.0103806840105263));
#41365=CARTESIAN_POINT('Ctrl Pts',(-0.207034905932455,0.00697771837226714,
-0.0103717631079065));
#41366=CARTESIAN_POINT('Ctrl Pts',(-0.207054100312034,0.00801199116278463,
-0.01033007892178));
#41367=CARTESIAN_POINT('Ctrl Pts',(-0.207051705141398,0.00801788788449221,
-0.0104364247901112));
#41368=CARTESIAN_POINT('Ctrl Pts',(-0.206946768666599,0.00800656573091688,
-0.0104285255622565));
#41369=CARTESIAN_POINT('Ctrl Pts',(-0.20684533708077,0.0100638006421552,
-0.0100937633659248));
#41370=CARTESIAN_POINT('Ctrl Pts',(-0.206843030517134,0.0100931862263171,
-0.0101974378781082));
#41371=CARTESIAN_POINT('Ctrl Pts',(-0.206736620206684,0.010091652693392,
-0.0101921840430576));
#41372=CARTESIAN_POINT('Ctrl Pts',(-0.207125466271094,0.0119235866362789,
-0.00921573185060216));
#41373=CARTESIAN_POINT('Ctrl Pts',(-0.207123577691201,0.0119749030496809,
-0.00930908688655247));
#41374=CARTESIAN_POINT('Ctrl Pts',(-0.207019198536868,0.0119854727335022,
-0.00929435969050802));
#41375=CARTESIAN_POINT('Ctrl Pts',(-0.207262576286763,0.0127576794032243,
-0.00863412005073474));
#41376=CARTESIAN_POINT('Ctrl Pts',(-0.207260928577023,0.0128184051686157,
-0.00872080512210846));
#41377=CARTESIAN_POINT('Ctrl Pts',(-0.207156193086846,0.012824836055491,
-0.00870680606209627));
#41378=CARTESIAN_POINT('Ctrl Pts',(-0.207097778634823,0.0074999984041968,
-0.0102884291162079));
#41379=CARTESIAN_POINT('Ctrl Pts',(-0.207097617294887,0.00749999849305758,
-0.0102948949871889));
#41380=CARTESIAN_POINT('Ctrl Pts',(-0.207096826594071,0.00749999872193563,
-0.0103013296439083));
#41381=CARTESIAN_POINT('Ctrl Pts',(-0.20709390155598,0.00749999949493435,
-0.0103144375318467));
#41382=CARTESIAN_POINT('Ctrl Pts',(-0.207091677519774,0.00750000005938463,
-0.0103210545038764));
#41383=CARTESIAN_POINT('Ctrl Pts',(-0.207083426652751,0.00750000213865603,
-0.010339102345941));
#41384=CARTESIAN_POINT('Ctrl Pts',(-0.207075853009443,0.00750000401966211,
-0.0103496701497808));
#41385=CARTESIAN_POINT('Ctrl Pts',(-0.207057113766972,0.00750000895351662,
-0.0103673633379332));
#41386=CARTESIAN_POINT('Ctrl Pts',(-0.207046121745384,0.00750001179091493,
-0.010374321862266));
#41387=CARTESIAN_POINT('Ctrl Pts',(-0.207022667760621,0.00750002009313667,
-0.0103834937529816));
#41388=CARTESIAN_POINT('Ctrl Pts',(-0.207011610188164,0.007500002533942,
-0.010385407470795));
#41389=CARTESIAN_POINT('Ctrl Pts',(-0.206999679808045,0.00750005757307741,
-0.0103859295033157));
#41390=CARTESIAN_POINT('Ctrl Pts',(-0.206997334122852,0.00750001932399001,
-0.0103859545510466));
#41391=CARTESIAN_POINT('Ctrl Pts',(-0.206995169267356,0.00750001981683416,
-0.0103859057989294));
#41392=CARTESIAN_POINT('Origin',(-0.207020862424657,0.00266442695171015,
-0.0089078479286756));
#41393=CARTESIAN_POINT('Ctrl Pts',(-0.207181588037537,0.00274982395495244,
-0.00896336710976845));
#41394=CARTESIAN_POINT('Ctrl Pts',(-0.207181460885151,0.00274576262790076,
-0.00896999422727271));
#41395=CARTESIAN_POINT('Ctrl Pts',(-0.207180541651928,0.00274098238846861,
-0.00897604305378098));
#41396=CARTESIAN_POINT('Ctrl Pts',(-0.207177066510391,0.0027296549790865,
-0.00898741356184911));
#41397=CARTESIAN_POINT('Ctrl Pts',(-0.207174383711823,0.0027231128678696,
-0.00899243649753085));
#41398=CARTESIAN_POINT('Ctrl Pts',(-0.207165746028982,0.00270533301997872,
-0.00900299747571993));
#41399=CARTESIAN_POINT('Ctrl Pts',(-0.207158634768288,0.0026932646575399,
-0.00900730024230634));
#41400=CARTESIAN_POINT('Ctrl Pts',(-0.207142021128562,0.00266880706469116,
-0.00901095287902417));
#41401=CARTESIAN_POINT('Ctrl Pts',(-0.207133150573149,0.0026571524192198,
-0.00901049789236432));
#41402=CARTESIAN_POINT('Ctrl Pts',(-0.207115076418399,0.00263545890743936,
-0.00900608900771923));
#41403=CARTESIAN_POINT('Ctrl Pts',(-0.207105920485487,0.00262514686178307,
-0.0090021126094672));
#41404=CARTESIAN_POINT('Ctrl Pts',(-0.207095016218406,0.00261465333045586,
-0.008996083770829));
#41405=CARTESIAN_POINT('Ctrl Pts',(-0.207093747453505,0.00261315504859148,
-0.00899517016771365));
#41406=CARTESIAN_POINT('Ctrl Pts',(-0.207092338322616,0.00261177910282465,
-0.00899428861609635));
#41407=CARTESIAN_POINT('Ctrl Pts',(-0.207261911557155,0.00224487504033121,
-0.00863509602890071));
#41408=CARTESIAN_POINT('Ctrl Pts',(-0.207261061333487,0.00218403251266008,
-0.00872217940345594));
#41409=CARTESIAN_POINT('Ctrl Pts',(-0.207155912480172,0.0021773545685175,
-0.00870850348120737));
#41410=CARTESIAN_POINT('Ctrl Pts',(-0.20712510668135,0.00308209641683207,
-0.0092178996899935));
#41411=CARTESIAN_POINT('Ctrl Pts',(-0.20712401154892,0.00303076155080782,
-0.0093116937851499));
#41412=CARTESIAN_POINT('Ctrl Pts',(-0.20701921751319,0.0030200107749622,
-0.00929732600181945));
#41413=CARTESIAN_POINT('Ctrl Pts',(-0.206845115742223,0.00493737975183436,
-0.0100931217449419));
#41414=CARTESIAN_POINT('Ctrl Pts',(-0.206843618048967,0.00490790247082884,
-0.0101971639881759));
#41415=CARTESIAN_POINT('Ctrl Pts',(-0.206736790651225,0.00490918313827814,
-0.0101922763693325));
#41416=CARTESIAN_POINT('Ctrl Pts',(-0.207054261772577,0.0069945228288837,
-0.0103301552766145));
#41417=CARTESIAN_POINT('Ctrl Pts',(-0.207052663899309,0.00698859617030293,
-0.0104369057642559));
#41418=CARTESIAN_POINT('Ctrl Pts',(-0.206947324401705,0.00700004890355841,
-0.0104294130005563));
#41419=CARTESIAN_POINT('Ctrl Pts',(-0.207143517855953,0.00801628664541418,
-0.0102737391026986));
#41420=CARTESIAN_POINT('Ctrl Pts',(-0.207141937229774,0.0080223612876047,
-0.0103797952379834));
#41421=CARTESIAN_POINT('Ctrl Pts',(-0.207036365988693,0.00803087655515608,
-0.0103712544502575));
#41422=CARTESIAN_POINT('Ctrl Pts',(-0.210235470212884,0.0125831962427011,
-0.00881114272403701));
#41423=CARTESIAN_POINT('Ctrl Pts',(-0.210233811792169,0.0126392072517556,
-0.00889487396476536));
#41424=CARTESIAN_POINT('Ctrl Pts',(-0.210333701636679,0.0126288133946314,
-0.00890292617772176));
#41425=CARTESIAN_POINT('Ctrl Pts',(-0.210109914640351,0.0118029254008048,
-0.00933261880976109));
#41426=CARTESIAN_POINT('Ctrl Pts',(-0.210108040881823,0.0118503934809046,
-0.00942208249800212));
#41427=CARTESIAN_POINT('Ctrl Pts',(-0.2102077892993,0.0118381776955304,
-0.00942974108211226));
#41428=CARTESIAN_POINT('Ctrl Pts',(-0.209858863349157,0.0100626309432614,
-0.0101397859379606));
#41429=CARTESIAN_POINT('Ctrl Pts',(-0.209856688792772,0.0100907353699573,
-0.010238163383176));
#41430=CARTESIAN_POINT('Ctrl Pts',(-0.209958115064439,0.0100898245173313,
-0.0102374345613252));
#41431=CARTESIAN_POINT('Ctrl Pts',(-0.210038384794055,0.00814902869092786,
-0.0103806956142887));
#41432=CARTESIAN_POINT('Ctrl Pts',(-0.210036077908365,0.00815640672945998,
-0.0104816997027483));
#41433=CARTESIAN_POINT('Ctrl Pts',(-0.210136329087176,0.00816633140866834,
-0.0104825258559512));
#41434=CARTESIAN_POINT('Ctrl Pts',(-0.210123208037224,0.00720701508233023,
-0.0103517770571818));
#41435=CARTESIAN_POINT('Ctrl Pts',(-0.210120913424717,0.00720383758858374,
-0.0104524503373305));
#41436=CARTESIAN_POINT('Ctrl Pts',(-0.21022125585175,0.0072127173421066,
-0.0104542782118082));
#41437=CARTESIAN_POINT('Ctrl Pts',(-0.210096834544416,0.00749994081583322,
-0.0103559757400411));
#41438=CARTESIAN_POINT('Ctrl Pts',(-0.210096686633433,0.00749994088263926,
-0.0103625206548424));
#41439=CARTESIAN_POINT('Ctrl Pts',(-0.210097184378745,0.00749994083320546,
-0.0103690638608643));
#41440=CARTESIAN_POINT('Ctrl Pts',(-0.210099528352888,0.00749994050181511,
-0.0103823679829186));
#41441=CARTESIAN_POINT('Ctrl Pts',(-0.21010145164146,0.00749994020608678,
-0.0103890789745933));
#41442=CARTESIAN_POINT('Ctrl Pts',(-0.21010888034258,0.0074999390400106,
-0.0104074816985564));
#41443=CARTESIAN_POINT('Ctrl Pts',(-0.210115970160806,0.00749993789742544,
-0.0104183808246853));
#41444=CARTESIAN_POINT('Ctrl Pts',(-0.210133893814439,0.00749993516413654,
-0.0104369023611447));
#41445=CARTESIAN_POINT('Ctrl Pts',(-0.210144561863844,0.0074999334935551,
-0.0104443501210892));
#41446=CARTESIAN_POINT('Ctrl Pts',(-0.210166481412328,0.00749993137224817,
-0.0104540837252773));
#41447=CARTESIAN_POINT('Ctrl Pts',(-0.210177278352322,0.00749991366139868,
-0.0104568712710575));
#41448=CARTESIAN_POINT('Ctrl Pts',(-0.210190485815975,0.00749994729335911,
-0.0104580473756483));
#41449=CARTESIAN_POINT('Ctrl Pts',(-0.210192746196891,0.00749992280800758,
-0.0104581733219418));
#41450=CARTESIAN_POINT('Ctrl Pts',(-0.210194950898968,0.00749992236667074,
-0.0104582231832109));
#41451=CARTESIAN_POINT('Ctrl Pts',(-0.210183035273252,0.0122509820678714,
-0.00902403648976699));
#41452=CARTESIAN_POINT('Ctrl Pts',(-0.210183004474919,0.0122549334919774,
-0.00903029130710398));
#41453=CARTESIAN_POINT('Ctrl Pts',(-0.210183907816865,0.0122595072821419,
-0.00903601560526435));
#41454=CARTESIAN_POINT('Ctrl Pts',(-0.210187712856156,0.0122705785956896,
-0.00904724790522209));
#41455=CARTESIAN_POINT('Ctrl Pts',(-0.210190895163352,0.0122770963799046,
-0.00905233251787761));
#41456=CARTESIAN_POINT('Ctrl Pts',(-0.210201224090118,0.0122946438148163,
-0.00906315213064524));
#41457=CARTESIAN_POINT('Ctrl Pts',(-0.210209983860423,0.0123066314588125,
-0.0090677677614427));
#41458=CARTESIAN_POINT('Ctrl Pts',(-0.210231026129084,0.0123312626491986,
-0.00907228628335188));
#41459=CARTESIAN_POINT('Ctrl Pts',(-0.210242507315303,0.01234307663651,
-0.00907218824628096));
#41460=CARTESIAN_POINT('Ctrl Pts',(-0.210272325114507,0.012370930810171,
-0.0090675228065052));
#41461=CARTESIAN_POINT('Ctrl Pts',(-0.210287216580575,0.0123822262288944,
-0.00906117162122654));
#41462=CARTESIAN_POINT('Ctrl Pts',(-0.210291961848719,0.0123857329846465,
-0.00905929124963881));
#41463=CARTESIAN_POINT('Ctrl Pts',(-0.21029352851447,0.0123871255042076,
-0.00905848601124937));
#41464=CARTESIAN_POINT('Ctrl Pts',(-0.210295216002383,0.012388387453904,
-0.00905773072421305));
#41465=CARTESIAN_POINT('Origin',(-0.210345973362526,0.0123353396224193,
-0.00897396358652427));
#41466=CARTESIAN_POINT('Ctrl Pts',(-0.209182549309909,0.0122515014451553,
-0.00900247968906914));
#41467=CARTESIAN_POINT('Ctrl Pts',(-0.209182424357049,0.0122555091588162,
-0.00900898508945461));
#41468=CARTESIAN_POINT('Ctrl Pts',(-0.209181534228362,0.0122602114412656,
-0.00901493115388496));
#41469=CARTESIAN_POINT('Ctrl Pts',(-0.209178171837601,0.0122713281354332,
-0.00902612282222287));
#41470=CARTESIAN_POINT('Ctrl Pts',(-0.209175578325821,0.0122777376353018,
-0.00903108372130858));
#41471=CARTESIAN_POINT('Ctrl Pts',(-0.209167153320636,0.012295293505668,
-0.00904164807624254));
#41472=CARTESIAN_POINT('Ctrl Pts',(-0.20916015810978,0.0123072763124866,
-0.00904600973000227));
#41473=CARTESIAN_POINT('Ctrl Pts',(-0.209143853782949,0.0123314717979331,
-0.00904980789329348));
#41474=CARTESIAN_POINT('Ctrl Pts',(-0.209135188499717,0.0123429527526135,
-0.00904947723024575));
#41475=CARTESIAN_POINT('Ctrl Pts',(-0.209115354906058,0.0123669938598687,
-0.00904490615931702));
#41476=CARTESIAN_POINT('Ctrl Pts',(-0.209105645668148,0.0123772529746108,
-0.00904019631515971));
#41477=CARTESIAN_POINT('Ctrl Pts',(-0.209098365777995,0.0123847593086512,
-0.00903603151450798));
#41478=CARTESIAN_POINT('Ctrl Pts',(-0.209096254901744,0.012386841541812,
-0.00903484552833635));
#41479=CARTESIAN_POINT('Ctrl Pts',(-0.209094136097871,0.0123888666300359,
-0.00903357723246944));
#41480=CARTESIAN_POINT('Ctrl Pts',(-0.209093330965559,0.0123896523666189,
-0.00903307128651946));
#41481=CARTESIAN_POINT('Ctrl Pts',(-0.210122790867358,0.00778687461044981,
-0.010351991928395));
#41482=CARTESIAN_POINT('Ctrl Pts',(-0.210120509030329,0.00778997965051194,
-0.0104525808922906));
#41483=CARTESIAN_POINT('Ctrl Pts',(-0.210220759666774,0.00778106815290546,
-0.0104544784162097));
#41484=CARTESIAN_POINT('Ctrl Pts',(-0.21003771958249,0.00684739648040692,
-0.0103800502715855));
#41485=CARTESIAN_POINT('Ctrl Pts',(-0.210035425847737,0.00683998407859043,
-0.0104809600904831));
#41486=CARTESIAN_POINT('Ctrl Pts',(-0.210135588276038,0.00683002917116009,
-0.0104818514875396));
#41487=CARTESIAN_POINT('Ctrl Pts',(-0.209859680423329,0.00494226274913538,
-0.0101407557752523));
#41488=CARTESIAN_POINT('Ctrl Pts',(-0.209857518240127,0.00491423839445973,
-0.0102390594248941));
#41489=CARTESIAN_POINT('Ctrl Pts',(-0.209958850344826,0.00491528136435581,
-0.0102384592310678));
#41490=CARTESIAN_POINT('Ctrl Pts',(-0.210110442658573,0.00320097165849752,
-0.00933430005928662));
#41491=CARTESIAN_POINT('Ctrl Pts',(-0.210108580826121,0.00315358902991755,
-0.00942370536723907));
#41492=CARTESIAN_POINT('Ctrl Pts',(-0.210208251154881,0.00316568454937026,
-0.00943138424087661));
#41493=CARTESIAN_POINT('Ctrl Pts',(-0.210234851606964,0.00242463804919971,
-0.00881636542139056));
#41494=CARTESIAN_POINT('Ctrl Pts',(-0.210233203468192,0.0023687621720114,
-0.00890008212730693));
#41495=CARTESIAN_POINT('Ctrl Pts',(-0.210333010304818,0.00237908946436521,
-0.00890816439708428));
#41496=CARTESIAN_POINT('Ctrl Pts',(-0.210295598600257,0.00261401462196279,
-0.0090592390136268));
#41497=CARTESIAN_POINT('Ctrl Pts',(-0.210294527757695,0.00261481630216766,
-0.00905971848287953));
#41498=CARTESIAN_POINT('Ctrl Pts',(-0.210291818773028,0.00261681405859242,
-0.0090608751759147));
#41499=CARTESIAN_POINT('Ctrl Pts',(-0.210289117458866,0.00261887013661076,
-0.00906195389803063));
#41500=CARTESIAN_POINT('Ctrl Pts',(-0.210279475839446,0.00262649256331565,
-0.0090658514781019));
#41501=CARTESIAN_POINT('Ctrl Pts',(-0.210266998510554,0.00263668469064512,
-0.00907006215183289));
#41502=CARTESIAN_POINT('Ctrl Pts',(-0.210241838214722,0.00266042729560625,
-0.00907369833425217));
#41503=CARTESIAN_POINT('Ctrl Pts',(-0.210230787403518,0.00267187783814618,
-0.00907368640849252));
#41504=CARTESIAN_POINT('Ctrl Pts',(-0.210210167289941,0.00269609427310657,
-0.00906916472948773));
#41505=CARTESIAN_POINT('Ctrl Pts',(-0.210201462620991,0.00270804669853119,
-0.00906452399287538));
#41506=CARTESIAN_POINT('Ctrl Pts',(-0.210191222605049,0.00272551333019873,
-0.00905369442458548));
#41507=CARTESIAN_POINT('Ctrl Pts',(-0.210188075958288,0.00273198594347644,
-0.00904862407492236));
#41508=CARTESIAN_POINT('Ctrl Pts',(-0.210184314434985,0.00274298004307225,
-0.009037441123476));
#41509=CARTESIAN_POINT('Ctrl Pts',(-0.21018342165608,0.00274752263533853,
-0.00903174675206267));
#41510=CARTESIAN_POINT('Ctrl Pts',(-0.210183451653278,0.00275144948649388,
-0.00902552855343153));
#41511=CARTESIAN_POINT('Ctrl Pts',(-0.209142530989361,0.00699231287835271,
-0.0103201859233318));
#41512=CARTESIAN_POINT('Ctrl Pts',(-0.209140159029996,0.00698629063188217,
-0.0104254976026752));
#41513=CARTESIAN_POINT('Ctrl Pts',(-0.209035328768285,0.00697775411075113,
-0.0104169399852814));
#41514=CARTESIAN_POINT('Ctrl Pts',(-0.209052501584123,0.00801199897977874,
-0.0103753688499246));
#41515=CARTESIAN_POINT('Ctrl Pts',(-0.209050114754894,0.00801789659276563,
-0.0104813665305186));
#41516=CARTESIAN_POINT('Ctrl Pts',(-0.208945510592866,0.0080064387339923,
-0.0104738696299997));
#41517=CARTESIAN_POINT('Ctrl Pts',(-0.208843911922949,0.0100634291810789,
-0.0101383603557189));
#41518=CARTESIAN_POINT('Ctrl Pts',(-0.208841612864033,0.010092810496628,
-0.0102416789156079));
#41519=CARTESIAN_POINT('Ctrl Pts',(-0.208735524411325,0.0100916723284601,
-0.0102367238690831));
#41520=CARTESIAN_POINT('Ctrl Pts',(-0.20912641034549,0.0119222931217929,
-0.00925753171213683));
#41521=CARTESIAN_POINT('Ctrl Pts',(-0.209124526741439,0.011973601805003,
-0.00935049411365509));
#41522=CARTESIAN_POINT('Ctrl Pts',(-0.209020465657013,0.011984218099799,
-0.00933612171575852));
#41523=CARTESIAN_POINT('Ctrl Pts',(-0.209262852149274,0.012755138999478,
-0.00867419623553459));
#41524=CARTESIAN_POINT('Ctrl Pts',(-0.209261207617309,0.0128158403474571,
-0.00876047032963096));
#41525=CARTESIAN_POINT('Ctrl Pts',(-0.209156792369228,0.0128224261641587,
-0.00874678973944371));
#41526=CARTESIAN_POINT('Ctrl Pts',(-0.209097174394345,0.00749996481452615,
-0.0103336053964147));
#41527=CARTESIAN_POINT('Ctrl Pts',(-0.209097013698476,0.00749996488422219,
-0.0103400756121614));
#41528=CARTESIAN_POINT('Ctrl Pts',(-0.209096222734907,0.00749996508674242,
-0.0103465146116718));
#41529=CARTESIAN_POINT('Ctrl Pts',(-0.209093296226861,0.00749996579190134,
-0.0103596271412186));
#41530=CARTESIAN_POINT('Ctrl Pts',(-0.209091071696894,0.00749996631386664,
-0.0103662445158202));
#41531=CARTESIAN_POINT('Ctrl Pts',(-0.209082819281554,0.00749996825608746,
-0.0103842927814137));
#41532=CARTESIAN_POINT('Ctrl Pts',(-0.209075244524087,0.00749997002888941,
-0.0103948603774847));
#41533=CARTESIAN_POINT('Ctrl Pts',(-0.209056502939813,0.00749997474929252,
-0.0104125530535077));
#41534=CARTESIAN_POINT('Ctrl Pts',(-0.209045509631471,0.00749997746681514,
-0.0104195111797564));
#41535=CARTESIAN_POINT('Ctrl Pts',(-0.209021616726638,0.00749998590382376,
-0.0104288529900601));
#41536=CARTESIAN_POINT('Ctrl Pts',(-0.20901043096659,0.00749996892955642,
-0.0104306201858471));
#41537=CARTESIAN_POINT('Ctrl Pts',(-0.208999076760909,0.00750002603475989,
-0.0104311167615857));
#41538=CARTESIAN_POINT('Ctrl Pts',(-0.208996706540869,0.00749998403251248,
-0.010431142048249));
#41539=CARTESIAN_POINT('Ctrl Pts',(-0.208994553794872,0.00749998449679488,
-0.0104310935426435));
#41540=CARTESIAN_POINT('Origin',(-0.209022200231755,0.00266602605730765,
-0.00894852322668744));
#41541=CARTESIAN_POINT('Ctrl Pts',(-0.209182662289348,0.00275131519549864,
-0.00900420129328437));
#41542=CARTESIAN_POINT('Ctrl Pts',(-0.209182535027075,0.00274724125113172,
-0.00901082072251512));
#41543=CARTESIAN_POINT('Ctrl Pts',(-0.209181615672769,0.00274244949160901,
-0.00901686048171236));
#41544=CARTESIAN_POINT('Ctrl Pts',(-0.209178140260104,0.00273110039458304,
-0.00902820949029176));
#41545=CARTESIAN_POINT('Ctrl Pts',(-0.209175457304311,0.00272454867617604,
-0.00903321999133582));
#41546=CARTESIAN_POINT('Ctrl Pts',(-0.209166819295205,0.00270674881741965,
-0.00904374696922658));
#41547=CARTESIAN_POINT('Ctrl Pts',(-0.209159707896966,0.00269467240680358,
-0.00904802664813589));
#41548=CARTESIAN_POINT('Ctrl Pts',(-0.209143133038255,0.00267026580891761,
-0.00905162397869498));
#41549=CARTESIAN_POINT('Ctrl Pts',(-0.209134309594035,0.00265866825396765,
-0.00905115969568957));
#41550=CARTESIAN_POINT('Ctrl Pts',(-0.209112873661121,0.00263292743671442,
-0.00904592097808777));
#41551=CARTESIAN_POINT('Ctrl Pts',(-0.209102711421051,0.00262248317195225,
-0.00904033396457725));
#41552=CARTESIAN_POINT('Ctrl Pts',(-0.209096266044791,0.00261624347336712,
-0.0090367573419262));
#41553=CARTESIAN_POINT('Ctrl Pts',(-0.209094901489963,0.00261466852848538,
-0.00903579591927314));
#41554=CARTESIAN_POINT('Ctrl Pts',(-0.209093406978092,0.0026132111295408,
-0.00903485819588743));
#41555=CARTESIAN_POINT('Ctrl Pts',(-0.209262801112433,0.00224697126424917,
-0.00867490866995627));
#41556=CARTESIAN_POINT('Ctrl Pts',(-0.209261929283104,0.00218608218935967,
-0.00876166481462779));
#41557=CARTESIAN_POINT('Ctrl Pts',(-0.20915700285995,0.00217931463768635,
-0.00874818364093454));
#41558=CARTESIAN_POINT('Ctrl Pts',(-0.20912666223509,0.00308301714484159,
-0.00925954111540404));
#41559=CARTESIAN_POINT('Ctrl Pts',(-0.209125547091583,0.00303162849784595,
-0.0093530344837294));
#41560=CARTESIAN_POINT('Ctrl Pts',(-0.209020973849429,0.00302089220559985,
-0.00933889224512626));
#41561=CARTESIAN_POINT('Ctrl Pts',(-0.20884410193955,0.00493732213256617,
-0.0101376857974969));
#41562=CARTESIAN_POINT('Ctrl Pts',(-0.20884258581963,0.00490781537082798,
-0.0102414789789533));
#41563=CARTESIAN_POINT('Ctrl Pts',(-0.208735982101809,0.00490868367757524,
-0.0102367410833359));
#41564=CARTESIAN_POINT('Ctrl Pts',(-0.209052616298212,0.00699464150726956,
-0.0103754833052408));
#41565=CARTESIAN_POINT('Ctrl Pts',(-0.209051000912337,0.0069887103865453,
-0.0104819951718267));
#41566=CARTESIAN_POINT('Ctrl Pts',(-0.208945896242155,0.00700032634036486,
-0.0104747676946981));
#41567=CARTESIAN_POINT('Ctrl Pts',(-0.209143633401348,0.00801615107495887,
-0.0103189165970082));
#41568=CARTESIAN_POINT('Ctrl Pts',(-0.209142034971987,0.00802223475741889,
-0.010424730840755));
#41569=CARTESIAN_POINT('Ctrl Pts',(-0.209036696922337,0.00803083836422602,
-0.0104164124237201));
#41570=CARTESIAN_POINT('Ctrl Pts',(-0.194260566397066,0.0127940739393323,
-0.00836181481645916));
#41571=CARTESIAN_POINT('Ctrl Pts',(-0.194258157740366,0.0128520362452587,
-0.00844683908739088));
#41572=CARTESIAN_POINT('Ctrl Pts',(-0.19436029261288,0.0128412877828854,
-0.00845361523486277));
#41573=CARTESIAN_POINT('Ctrl Pts',(-0.194124314813594,0.0119569377977277,
-0.00893191938984265));
#41574=CARTESIAN_POINT('Ctrl Pts',(-0.194121655647109,0.0120058535938877,
-0.00902316064089455));
#41575=CARTESIAN_POINT('Ctrl Pts',(-0.194223452297076,0.0119915226494169,
-0.00903023491578875));
#41576=CARTESIAN_POINT('Ctrl Pts',(-0.193851105984685,0.0100693098681627,
-0.0098070233056107));
#41577=CARTESIAN_POINT('Ctrl Pts',(-0.193848076892825,0.010097302393308,
-0.00990791370737201));
#41578=CARTESIAN_POINT('Ctrl Pts',(-0.193951811020719,0.0100975879788375,
-0.00990507857556678));
#41579=CARTESIAN_POINT('Ctrl Pts',(-0.194064486196732,0.00799786398926628,
-0.0100356162055956));
#41580=CARTESIAN_POINT('Ctrl Pts',(-0.194061330849289,0.00800343965044749,
-0.0101389739286565));
#41581=CARTESIAN_POINT('Ctrl Pts',(-0.194163719819071,0.00801353727066376,
-0.0101386725304691));
#41582=CARTESIAN_POINT('Ctrl Pts',(-0.194147069647878,0.00697986904195666,
-0.00998010224803608));
#41583=CARTESIAN_POINT('Ctrl Pts',(-0.19414393857776,0.00697412920907708,
-0.0100828290181077));
#41584=CARTESIAN_POINT('Ctrl Pts',(-0.194246550098368,0.00698246049660227,
-0.0100834655870346));
#41585=CARTESIAN_POINT('Ctrl Pts',(-0.194103280095705,0.00750354479393001,
-0.00999450817382853));
#41586=CARTESIAN_POINT('Ctrl Pts',(-0.194103132213932,0.0075035473081524,
-0.0100010515017158));
#41587=CARTESIAN_POINT('Ctrl Pts',(-0.194103629370271,0.007503550039466,
-0.0100075931783246));
#41588=CARTESIAN_POINT('Ctrl Pts',(-0.194105970904067,0.00750355604164788,
-0.0100208940754098));
#41589=CARTESIAN_POINT('Ctrl Pts',(-0.194107892233365,0.00750355931897568,
-0.0100276035503664));
#41590=CARTESIAN_POINT('Ctrl Pts',(-0.194115314414744,0.0075035690321051,
-0.0100460041977227));
#41591=CARTESIAN_POINT('Ctrl Pts',(-0.194122399194833,0.00750357569145501,
-0.0100569038408753));
#41592=CARTESIAN_POINT('Ctrl Pts',(-0.19414031206282,0.00750358897799523,
-0.010075426673766));
#41593=CARTESIAN_POINT('Ctrl Pts',(-0.194150974046746,0.00750359548610248,
-0.010082875676867));
#41594=CARTESIAN_POINT('Ctrl Pts',(-0.194174603735767,0.00750360748583984,
-0.0100933762285736));
#41595=CARTESIAN_POINT('Ctrl Pts',(-0.194187730336832,0.00750377794946251,
-0.0100963594926318));
#41596=CARTESIAN_POINT('Ctrl Pts',(-0.194200912520396,0.00750360613312389,
-0.0100967433641591));
#41597=CARTESIAN_POINT('Ctrl Pts',(-0.194201350069792,0.00750361803291018,
-0.0100967539594273));
#41598=CARTESIAN_POINT('Ctrl Pts',(-0.194177780472304,0.0122674979892277,
-0.00869700656513734));
#41599=CARTESIAN_POINT('Ctrl Pts',(-0.194177756405024,0.0122713482585029,
-0.00870330565303864));
#41600=CARTESIAN_POINT('Ctrl Pts',(-0.194178660379777,0.0122758265372359,
-0.00870908561487317));
#41601=CARTESIAN_POINT('Ctrl Pts',(-0.194182462390553,0.012286723987401,
-0.00872048033693503));
#41602=CARTESIAN_POINT('Ctrl Pts',(-0.194185646336855,0.0122931733460766,
-0.00872566746126095));
#41603=CARTESIAN_POINT('Ctrl Pts',(-0.194195975107812,0.0123105730084261,
-0.00873675093606282));
#41604=CARTESIAN_POINT('Ctrl Pts',(-0.194204729183099,0.0123224980676776,
-0.00874154210222169));
#41605=CARTESIAN_POINT('Ctrl Pts',(-0.194226094161862,0.0123474717938464,
-0.00874649591046643));
#41606=CARTESIAN_POINT('Ctrl Pts',(-0.194237980625125,0.0123596746544839,
-0.00874649211843202));
#41607=CARTESIAN_POINT('Ctrl Pts',(-0.194268231716554,0.0123878641057918,
-0.00874186420697733));
#41608=CARTESIAN_POINT('Ctrl Pts',(-0.194283072567502,0.0123993606550317,
-0.00873548089790034));
#41609=CARTESIAN_POINT('Ctrl Pts',(-0.194287649953457,0.0124023998296309,
-0.00873384454996397));
#41610=CARTESIAN_POINT('Ctrl Pts',(-0.194288254848304,0.0124030132709194,
-0.00873349488248058));
#41611=CARTESIAN_POINT('Ctrl Pts',(-0.194289068674857,0.0124038353634868,
-0.00873302410067472));
#41612=CARTESIAN_POINT('Ctrl Pts',(-0.194289765313071,0.0124043621676603,
-0.00873271973491913));
#41613=CARTESIAN_POINT('Origin',(-0.194340688401695,0.0123526500534516,
-0.00864811707722939));
#41614=CARTESIAN_POINT('Ctrl Pts',(-0.193177319689981,0.0122679027418712,
-0.00867581562949272));
#41615=CARTESIAN_POINT('Ctrl Pts',(-0.193177195620142,0.0122718100036639,
-0.0086823850364032));
#41616=CARTESIAN_POINT('Ctrl Pts',(-0.193176303901968,0.0122764204768761,
-0.00868840561290754));
#41617=CARTESIAN_POINT('Ctrl Pts',(-0.193172933398585,0.0122873646022273,
-0.00869977330013174));
#41618=CARTESIAN_POINT('Ctrl Pts',(-0.19317033287057,0.0122936974996128,
-0.00870483499014074));
#41619=CARTESIAN_POINT('Ctrl Pts',(-0.193161886206775,0.0123110865119641,
-0.00871567327260089));
#41620=CARTESIAN_POINT('Ctrl Pts',(-0.193154873080797,0.0123229982296,-0.00872022208136985));
#41621=CARTESIAN_POINT('Ctrl Pts',(-0.193138530834182,0.0123471213424915,
-0.00872439825343486));
#41622=CARTESIAN_POINT('Ctrl Pts',(-0.193129848577642,0.0123585969399349,
-0.00872424886387294));
#41623=CARTESIAN_POINT('Ctrl Pts',(-0.193109605516503,0.0123831387994624,
-0.00871998396816283));
#41624=CARTESIAN_POINT('Ctrl Pts',(-0.193099863516187,0.0123934072473534,
-0.008715308331385));
#41625=CARTESIAN_POINT('Ctrl Pts',(-0.193093015200619,0.0124005273651118,
-0.00871150359471354));
#41626=CARTESIAN_POINT('Ctrl Pts',(-0.193090844328643,0.0124026776594429,
-0.00871032730139874));
#41627=CARTESIAN_POINT('Ctrl Pts',(-0.193088664937624,0.0124047671675376,
-0.00870906101126539));
#41628=CARTESIAN_POINT('Ctrl Pts',(-0.19308791289601,0.0124055064406691,
-0.00870860142875256));
#41629=CARTESIAN_POINT('Ctrl Pts',(-0.194360584264707,0.0021615829798264,
-0.00845557112034835));
#41630=CARTESIAN_POINT('Ctrl Pts',(-0.194258178150358,0.00215079489622151,
-0.00844888158936903));
#41631=CARTESIAN_POINT('Ctrl Pts',(-0.19426077173291,0.00220889260676681,
-0.00836363109027858));
#41632=CARTESIAN_POINT('Ctrl Pts',(-0.194224163205224,0.00301216227742662,
-0.00903230161285869));
#41633=CARTESIAN_POINT('Ctrl Pts',(-0.194122092678868,0.00299780557649061,
-0.00902532321450204));
#41634=CARTESIAN_POINT('Ctrl Pts',(-0.194124936884012,0.00304683006696333,
-0.00893383915952295));
#41635=CARTESIAN_POINT('Ctrl Pts',(-0.193953562027494,0.00490777775727108,
-0.00990682227567009));
#41636=CARTESIAN_POINT('Ctrl Pts',(-0.193849566274215,0.0049080439579958,
-0.00990973779496289));
#41637=CARTESIAN_POINT('Ctrl Pts',(-0.193852785118349,0.00493605141346052,
-0.00980856626502038));
#41638=CARTESIAN_POINT('Ctrl Pts',(-0.19416412360165,0.00699334436810937,
-0.0101391368498539));
#41639=CARTESIAN_POINT('Ctrl Pts',(-0.194061460165267,0.00700338018321717,
-0.0101395152380399));
#41640=CARTESIAN_POINT('Ctrl Pts',(-0.194064801952071,0.00700887609067415,
-0.0100358889677675));
#41641=CARTESIAN_POINT('Ctrl Pts',(-0.194246312133847,0.00802513287488578,
-0.0100830358876897));
#41642=CARTESIAN_POINT('Ctrl Pts',(-0.19414342831192,0.00803342503477834,
-0.0100824839740061));
#41643=CARTESIAN_POINT('Ctrl Pts',(-0.194146745965864,0.00802757386687429,
-0.00997950098896328));
#41644=CARTESIAN_POINT('Ctrl Pts',(-0.194290187104405,0.00259891113253263,
-0.00873470281275794));
#41645=CARTESIAN_POINT('Ctrl Pts',(-0.194289196087415,0.00259966116357646,
-0.00873513572158582));
#41646=CARTESIAN_POINT('Ctrl Pts',(-0.194286416940508,0.00260172379996549,
-0.008736291057404));
#41647=CARTESIAN_POINT('Ctrl Pts',(-0.194283643828663,0.00260385112950153,
-0.00873736128103573));
#41648=CARTESIAN_POINT('Ctrl Pts',(-0.194274462771107,0.00261119741567337,
-0.00874097761404353));
#41649=CARTESIAN_POINT('Ctrl Pts',(-0.194261757867021,0.00262161302243235,
-0.00874518598693824));
#41650=CARTESIAN_POINT('Ctrl Pts',(-0.19423621646237,0.00264584978012857,
-0.00874846049076316));
#41651=CARTESIAN_POINT('Ctrl Pts',(-0.194225125971027,0.0026573860669246,
-0.00874823380164047));
#41652=CARTESIAN_POINT('Ctrl Pts',(-0.194204592913332,0.00268156106677389,
-0.00874321412099836));
#41653=CARTESIAN_POINT('Ctrl Pts',(-0.194195984267789,0.00269338088257152,
-0.00873835693792421));
#41654=CARTESIAN_POINT('Ctrl Pts',(-0.194185890787921,0.00271055428582041,
-0.00872725214657669));
#41655=CARTESIAN_POINT('Ctrl Pts',(-0.194182801590003,0.00271688086249955,
-0.00872210658747948));
#41656=CARTESIAN_POINT('Ctrl Pts',(-0.194179113423095,0.00272757690945129,
-0.00871084654768075));
#41657=CARTESIAN_POINT('Ctrl Pts',(-0.194178237417962,0.00273197723860756,
-0.00870514428252823));
#41658=CARTESIAN_POINT('Ctrl Pts',(-0.194178261015029,0.00273576742350967,
-0.00869894006840107));
#41659=CARTESIAN_POINT('Ctrl Pts',(-0.193150275258269,0.0128441169814804,
-0.00842880923135799));
#41660=CARTESIAN_POINT('Ctrl Pts',(-0.193256325284946,0.0128379311470973,
-0.00844320696924679));
#41661=CARTESIAN_POINT('Ctrl Pts',(-0.193257206366102,0.0127778410782848,
-0.00835443734984138));
#41662=CARTESIAN_POINT('Ctrl Pts',(-0.193012927796993,0.0119927115204579,
-0.00900510709243607));
#41663=CARTESIAN_POINT('Ctrl Pts',(-0.193118624042428,0.0119821209508065,
-0.0090203118718904));
#41664=CARTESIAN_POINT('Ctrl Pts',(-0.193119759931369,0.0119315097041858,
-0.00892506728326148));
#41665=CARTESIAN_POINT('Ctrl Pts',(-0.192744917262978,0.0100930204918921,
-0.00988017938288733));
#41666=CARTESIAN_POINT('Ctrl Pts',(-0.192852605833001,0.010095868904492,
-0.00988588636415747));
#41667=CARTESIAN_POINT('Ctrl Pts',(-0.192854157456687,0.0100668059221215,
-0.00978080952480875));
#41668=CARTESIAN_POINT('Ctrl Pts',(-0.192955684307683,0.00800473900327279,
-0.0101117489985091));
#41669=CARTESIAN_POINT('Ctrl Pts',(-0.193061940873377,0.00801563509081901,
-0.0101204188260094));
#41670=CARTESIAN_POINT('Ctrl Pts',(-0.193063595677509,0.00800977514437518,
-0.0100127299449779));
#41671=CARTESIAN_POINT('Ctrl Pts',(-0.193039136173225,0.00697204692880732,
-0.0100554625058695));
#41672=CARTESIAN_POINT('Ctrl Pts',(-0.193145616630949,0.00698026662548628,
-0.0100650217034591));
#41673=CARTESIAN_POINT('Ctrl Pts',(-0.193147252943133,0.00698620175694981,
-0.00995799541934645));
#41674=CARTESIAN_POINT('Ctrl Pts',(-0.193103862234772,0.00750326159826634,
-0.00997223502421426));
#41675=CARTESIAN_POINT('Ctrl Pts',(-0.193103696428452,0.00750326382091886,
-0.00997867241877183));
#41676=CARTESIAN_POINT('Ctrl Pts',(-0.19310290699438,0.00750326582245723,
-0.00998507854929882));
#41677=CARTESIAN_POINT('Ctrl Pts',(-0.193099989901722,0.00750326946960355,
-0.00999815742026939));
#41678=CARTESIAN_POINT('Ctrl Pts',(-0.193097767534269,0.0075032710631149,
-0.0100047730394995));
#41679=CARTESIAN_POINT('Ctrl Pts',(-0.193089521905136,0.00750327467609872,
-0.0100228194487802));
#41680=CARTESIAN_POINT('Ctrl Pts',(-0.193081952036663,0.00750327586985883,
-0.0100333879480974));
#41681=CARTESIAN_POINT('Ctrl Pts',(-0.193063220755058,0.0075032758439836,
-0.0100510828272992));
#41682=CARTESIAN_POINT('Ctrl Pts',(-0.193052233129148,0.0075032746140179,
-0.0100580426754926));
#41683=CARTESIAN_POINT('Ctrl Pts',(-0.193020283179751,0.00750326846488784,
-0.0100705448117449));
#41684=CARTESIAN_POINT('Ctrl Pts',(-0.193003724950557,0.00750323391604461,
-0.0100696728225077));
#41685=CARTESIAN_POINT('Ctrl Pts',(-0.193001728824581,0.00750328363033614,
-0.010069640921573));
#41686=CARTESIAN_POINT('Ctrl Pts',(-0.193001286033377,0.00750326128071969,
-0.010069631677871));
#41687=CARTESIAN_POINT('Origin',(-0.193016821989473,0.00264931970905631,
-0.00862349334194056));
#41688=CARTESIAN_POINT('Ctrl Pts',(-0.193178913430778,0.00273545550310997,
-0.00867781944513263));
#41689=CARTESIAN_POINT('Ctrl Pts',(-0.193178786956274,0.00273148399745027,
-0.00868450526830737));
#41690=CARTESIAN_POINT('Ctrl Pts',(-0.193177865206733,0.00272678530631968,
-0.00869062192164722));
#41691=CARTESIAN_POINT('Ctrl Pts',(-0.193174378694683,0.00271560978211082,
-0.00870215245451658));
#41692=CARTESIAN_POINT('Ctrl Pts',(-0.193171686355034,0.00270913420128244,
-0.00870726645002183));
#41693=CARTESIAN_POINT('Ctrl Pts',(-0.193163020358285,0.00269149818684289,
-0.00871807095284634));
#41694=CARTESIAN_POINT('Ctrl Pts',(-0.193155886358353,0.00267948953902128,
-0.00872253867555305));
#41695=CARTESIAN_POINT('Ctrl Pts',(-0.193138925514157,0.00265465328672384,
-0.00872659620125043));
#41696=CARTESIAN_POINT('Ctrl Pts',(-0.193129671497449,0.002642574582794,
-0.00872620641933053));
#41697=CARTESIAN_POINT('Ctrl Pts',(-0.193106181219171,0.00261457933111291,
-0.00872055797890539));
#41698=CARTESIAN_POINT('Ctrl Pts',(-0.193094904929187,0.00260320861244047,
-0.00871383251213535));
#41699=CARTESIAN_POINT('Ctrl Pts',(-0.193091139850869,0.00259998782715419,
-0.00871194606472707));
#41700=CARTESIAN_POINT('Ctrl Pts',(-0.193090658832604,0.0025993312971884,
-0.00871155317921895));
#41701=CARTESIAN_POINT('Ctrl Pts',(-0.193090011126355,0.00259845151805998,
-0.00871102314495721));
#41702=CARTESIAN_POINT('Ctrl Pts',(-0.193089423336345,0.00259787423512406,
-0.00871066459632005));
#41703=CARTESIAN_POINT('Ctrl Pts',(-0.193258176380086,0.00222512554213558,
-0.008356333420045));
#41704=CARTESIAN_POINT('Ctrl Pts',(-0.193257406685722,0.00216515257785461,
-0.00844502540000934));
#41705=CARTESIAN_POINT('Ctrl Pts',(-0.193151455537886,0.00215890244938321,
-0.00843089879221508));
#41706=CARTESIAN_POINT('Ctrl Pts',(-0.193122002439102,0.00307212219069519,
-0.00892699819824813));
#41707=CARTESIAN_POINT('Ctrl Pts',(-0.19312097776627,0.00302162873844681,
-0.00902215789008911));
#41708=CARTESIAN_POINT('Ctrl Pts',(-0.193015373477763,0.00301107658670332,
-0.0090072570423295));
#41709=CARTESIAN_POINT('Ctrl Pts',(-0.192856798552873,0.004938435513375,
-0.00978238514439772));
#41710=CARTESIAN_POINT('Ctrl Pts',(-0.192855360966354,0.00490946584342564,
-0.00988735113571471));
#41711=CARTESIAN_POINT('Ctrl Pts',(-0.192747799146241,0.00491202380037548,
-0.00988180381919543));
#41712=CARTESIAN_POINT('Ctrl Pts',(-0.193063736243557,0.00699648123524497,
-0.0100130244108273));
#41713=CARTESIAN_POINT('Ctrl Pts',(-0.193062194778461,0.00699068968148678,
-0.0101205874911818));
#41714=CARTESIAN_POINT('Ctrl Pts',(-0.192956038359925,0.00700150933952738,
-0.0101121699854943));
#41715=CARTESIAN_POINT('Ctrl Pts',(-0.193146983756164,0.00802059256633889,
-0.00995750851088701));
#41716=CARTESIAN_POINT('Ctrl Pts',(-0.193145461334373,0.0080265884898962,
-0.0100644020028561));
#41717=CARTESIAN_POINT('Ctrl Pts',(-0.19303908563067,0.0080347289111402,
-0.0100550909375128));
#41718=CARTESIAN_POINT('Ctrl Pts',(-0.214216589193599,0.0124501517797991,
-0.00897739024746242));
#41719=CARTESIAN_POINT('Ctrl Pts',(-0.214214906549421,0.0125049445268657,
-0.00906167044569434));
#41720=CARTESIAN_POINT('Ctrl Pts',(-0.214314571072553,0.012494503099187,
-0.00906980642227252));
#41721=CARTESIAN_POINT('Ctrl Pts',(-0.214098604421142,0.0117052239517064,
-0.00946081335779316));
#41722=CARTESIAN_POINT('Ctrl Pts',(-0.214096725093907,0.0117518018313808,
-0.00955043625299295));
#41723=CARTESIAN_POINT('Ctrl Pts',(-0.214196353866795,0.0117403989593848,
-0.00955782479538539));
#41724=CARTESIAN_POINT('Ctrl Pts',(-0.213868936752257,0.0100586906401089,
-0.0102133997812258));
#41725=CARTESIAN_POINT('Ctrl Pts',(-0.213866781074678,0.010086875729085,
-0.0103113719504311));
#41726=CARTESIAN_POINT('Ctrl Pts',(-0.213967915697219,0.0100855217422406,
-0.0103112152848752));
#41727=CARTESIAN_POINT('Ctrl Pts',(-0.214026024666252,0.00825308653731274,
-0.0104575334667986));
#41728=CARTESIAN_POINT('Ctrl Pts',(-0.214023739513263,0.00826164733836335,
-0.0105581758061061));
#41729=CARTESIAN_POINT('Ctrl Pts',(-0.214123819636435,0.00827119179233783,
-0.010559097489943));
#41730=CARTESIAN_POINT('Ctrl Pts',(-0.214108345900493,0.00736178832954375,
-0.0104455690809484));
#41731=CARTESIAN_POINT('Ctrl Pts',(-0.21410606524853,0.00736033884333731,
-0.0105460685302323));
#41732=CARTESIAN_POINT('Ctrl Pts',(-0.214206164582688,0.00736950848589431,
-0.0105479371910573));
#41733=CARTESIAN_POINT('Ctrl Pts',(-0.214095598208164,0.00750036280421892,
-0.0104463507918903));
#41734=CARTESIAN_POINT('Ctrl Pts',(-0.214095450286403,0.00750036319807516,
-0.0104528962354918));
#41735=CARTESIAN_POINT('Ctrl Pts',(-0.214095948235342,0.00750036349347478,
-0.0104594399498248));
#41736=CARTESIAN_POINT('Ctrl Pts',(-0.214098293054094,0.00750036390124496,
-0.0104727451491399));
#41737=CARTESIAN_POINT('Ctrl Pts',(-0.214100217021513,0.00750036399949698,
-0.0104794566463362));
#41738=CARTESIAN_POINT('Ctrl Pts',(-0.214107648000867,0.00750036397740217,
-0.010497860091735));
#41739=CARTESIAN_POINT('Ctrl Pts',(-0.214114739600234,0.0075003635906343,
-0.0105087590474747));
#41740=CARTESIAN_POINT('Ctrl Pts',(-0.2141326670907,0.00750036233657987,
-0.0105272801749843));
#41741=CARTESIAN_POINT('Ctrl Pts',(-0.214143337315054,0.00750036136102943,
-0.0105347275236168));
#41742=CARTESIAN_POINT('Ctrl Pts',(-0.21416526406917,0.00750036056502232,
-0.0105444618788871));
#41743=CARTESIAN_POINT('Ctrl Pts',(-0.214176061651198,0.00750034115386931,
-0.0105472471779442));
#41744=CARTESIAN_POINT('Ctrl Pts',(-0.214189257514336,0.00750038006836895,
-0.0105484223801725));
#41745=CARTESIAN_POINT('Ctrl Pts',(-0.214191531845057,0.0075003523748629,
-0.0105485491122668));
#41746=CARTESIAN_POINT('Ctrl Pts',(-0.214193730602855,0.00750035199462301,
-0.0105485988658817));
#41747=CARTESIAN_POINT('Ctrl Pts',(-0.21418476171475,0.0122470248836337,
-0.00910661242247999));
#41748=CARTESIAN_POINT('Ctrl Pts',(-0.214184729492537,0.0122509958337976,
-0.0091128508218304));
#41749=CARTESIAN_POINT('Ctrl Pts',(-0.21418563061837,0.0122555871063697,
-0.00911855690753845));
#41750=CARTESIAN_POINT('Ctrl Pts',(-0.214189427897225,0.0122666878416324,
-0.00912974237444637));
#41751=CARTESIAN_POINT('Ctrl Pts',(-0.214192602948848,0.0122732155482737,
-0.00913480006953024));
#41752=CARTESIAN_POINT('Ctrl Pts',(-0.214202913814278,0.012290788265655,
-0.00914555709199986));
#41753=CARTESIAN_POINT('Ctrl Pts',(-0.214211662701835,0.0123027879767839,
-0.00915013351377761));
#41754=CARTESIAN_POINT('Ctrl Pts',(-0.214232489475916,0.0123272045160123,
-0.0091545341786767));
#41755=CARTESIAN_POINT('Ctrl Pts',(-0.214243724668783,0.012338802234618,
-0.00915444487536124));
#41756=CARTESIAN_POINT('Ctrl Pts',(-0.214271070311354,0.012364454941799,
-0.00915023794967844));
#41757=CARTESIAN_POINT('Ctrl Pts',(-0.214284343428429,0.0123749399149735,
-0.00914509100745944));
#41758=CARTESIAN_POINT('Ctrl Pts',(-0.214290958431559,0.0123799442675073,
-0.00914245939257118));
#41759=CARTESIAN_POINT('Ctrl Pts',(-0.214293751115597,0.0123821573006203,
-0.00914127256522943));
#41760=CARTESIAN_POINT('Ctrl Pts',(-0.214296544881388,0.0123843107719361,
-0.00913998276525925));
#41761=CARTESIAN_POINT('Ctrl Pts',(-0.214296932467762,0.0123846001898489,
-0.00913980814574909));
#41762=CARTESIAN_POINT('Origin',(-0.214347684294818,0.012331269897534,-0.00905622192851621));
#41763=CARTESIAN_POINT('Ctrl Pts',(-0.213184281197705,0.0122471129150008,
-0.00908524735490702));
#41764=CARTESIAN_POINT('Ctrl Pts',(-0.213184156012283,0.0122511428892307,
-0.0090917377174671));
#41765=CARTESIAN_POINT('Ctrl Pts',(-0.213183265788318,0.012255865025333,
-0.00909766666595631));
#41766=CARTESIAN_POINT('Ctrl Pts',(-0.213179903446603,0.0122670179573602,
-0.00910881858185788));
#41767=CARTESIAN_POINT('Ctrl Pts',(-0.21317731012386,0.0122734428477997,
-0.00911375708486854));
#41768=CARTESIAN_POINT('Ctrl Pts',(-0.213168885194293,0.0122910309742747,
-0.00912426161680266));
#41769=CARTESIAN_POINT('Ctrl Pts',(-0.213161889771395,0.012303025812301,
-0.00912858308631421));
#41770=CARTESIAN_POINT('Ctrl Pts',(-0.213145583015019,0.0123272295859375,
-0.00913230120812302));
#41771=CARTESIAN_POINT('Ctrl Pts',(-0.213136915228883,0.0123387079053039,
-0.00913193227948719));
#41772=CARTESIAN_POINT('Ctrl Pts',(-0.213117167511167,0.0123626169193058,
-0.0091273020756134));
#41773=CARTESIAN_POINT('Ctrl Pts',(-0.213107506698602,0.0123728239002587,
-0.0091226165296789));
#41774=CARTESIAN_POINT('Ctrl Pts',(-0.213100053077068,0.0123804799160748,
-0.00911833344043855));
#41775=CARTESIAN_POINT('Ctrl Pts',(-0.213097967534007,0.0123825341941126,
-0.00911715192851019));
#41776=CARTESIAN_POINT('Ctrl Pts',(-0.213095874558879,0.0123845334039177,
-0.00911589143619706));
#41777=CARTESIAN_POINT('Ctrl Pts',(-0.213095043824064,0.01238534178372,
-0.00911536679023199));
#41778=CARTESIAN_POINT('Ctrl Pts',(-0.214099251930435,0.00754007420866826,
-0.0104463437857496));
#41779=CARTESIAN_POINT('Ctrl Pts',(-0.214096973354194,0.00754042143926795,
-0.010546746497242));
#41780=CARTESIAN_POINT('Ctrl Pts',(-0.214196961785067,0.00753121108484114,
-0.0105486173304038));
#41781=CARTESIAN_POINT('Ctrl Pts',(-0.214020081132227,0.00668104711880522,
-0.01044839731125));
#41782=CARTESIAN_POINT('Ctrl Pts',(-0.214017802600064,0.00667177376162901,
-0.0105488323717457));
#41783=CARTESIAN_POINT('Ctrl Pts',(-0.214117810400573,0.00666260452057459,
-0.0105498212479641));
#41784=CARTESIAN_POINT('Ctrl Pts',(-0.21387699556738,0.00494790676441162,
-0.0102055683200936));
#41785=CARTESIAN_POINT('Ctrl Pts',(-0.213874843443667,0.00491981746697117,
-0.010303350730012));
#41786=CARTESIAN_POINT('Ctrl Pts',(-0.213975820466248,0.00492132683014941,
-0.010303508794821));
#41787=CARTESIAN_POINT('Ctrl Pts',(-0.214092364657753,0.00335460445828704,
-0.00948776443558196));
#41788=CARTESIAN_POINT('Ctrl Pts',(-0.214090476556027,0.00330875018108462,
-0.00957759356201309));
#41789=CARTESIAN_POINT('Ctrl Pts',(-0.214190056939973,0.00331969202055049,
-0.00958478139798083));
#41790=CARTESIAN_POINT('Ctrl Pts',(-0.214205206332109,0.00263311474131057,
-0.00903080833434456));
#41791=CARTESIAN_POINT('Ctrl Pts',(-0.21420350377054,0.0025792983289028,
-0.00911558882921577));
#41792=CARTESIAN_POINT('Ctrl Pts',(-0.214303063785917,0.00258973324630672,
-0.00912369765822408));
#41793=CARTESIAN_POINT('Ctrl Pts',(-0.214298632002388,0.00261569392237272,
-0.00914002695164348));
#41794=CARTESIAN_POINT('Ctrl Pts',(-0.214297526642216,0.00261652006806272,
-0.00914052536543213));
#41795=CARTESIAN_POINT('Ctrl Pts',(-0.214294851212556,0.00261849454413502,
-0.00914167725032275));
#41796=CARTESIAN_POINT('Ctrl Pts',(-0.214292183618819,0.00262052438289603,
-0.00914275417453498));
#41797=CARTESIAN_POINT('Ctrl Pts',(-0.214281346220273,0.00262906971274197,
-0.00914716403535739));
#41798=CARTESIAN_POINT('Ctrl Pts',(-0.214269186343652,0.00263913734339031,
-0.00915106719571335));
#41799=CARTESIAN_POINT('Ctrl Pts',(-0.214244917624073,0.00266202950687075,
-0.00915467550143725));
#41800=CARTESIAN_POINT('Ctrl Pts',(-0.214233875587385,0.00267347135966337,
-0.00915471589753221));
#41801=CARTESIAN_POINT('Ctrl Pts',(-0.214213246240943,0.00269770925175791,
-0.00915031153285751));
#41802=CARTESIAN_POINT('Ctrl Pts',(-0.214204528192406,0.00270969263822594,
-0.00914572400356269));
#41803=CARTESIAN_POINT('Ctrl Pts',(-0.21419426732704,0.00272722439751406,
-0.00913496538472965));
#41804=CARTESIAN_POINT('Ctrl Pts',(-0.214191112262838,0.00273372826159939,
-0.0091299171157316));
#41805=CARTESIAN_POINT('Ctrl Pts',(-0.214187339842144,0.00274478676577278,
-0.00911876281117197));
#41806=CARTESIAN_POINT('Ctrl Pts',(-0.214186444624373,0.00274936038677583,
-0.00911307602768412));
#41807=CARTESIAN_POINT('Ctrl Pts',(-0.214186475873142,0.00275331763246593,
-0.00910686068665908));
#41808=CARTESIAN_POINT('Ctrl Pts',(-0.213142440708018,0.00699294600996641,
-0.0104100731831301));
#41809=CARTESIAN_POINT('Ctrl Pts',(-0.213140554707719,0.00698694437899309,
-0.0105151055519326));
#41810=CARTESIAN_POINT('Ctrl Pts',(-0.213035974700116,0.00697822305542204,
-0.0105073143890869));
#41811=CARTESIAN_POINT('Ctrl Pts',(-0.213049377162493,0.00801213213024399,
-0.0104654545470825));
#41812=CARTESIAN_POINT('Ctrl Pts',(-0.213047475720085,0.00801810774455873,
-0.0105711737868596));
#41813=CARTESIAN_POINT('Ctrl Pts',(-0.212943124439694,0.00800638504375276,
-0.0105645204728977));
#41814=CARTESIAN_POINT('Ctrl Pts',(-0.212842352364478,0.0100623279960898,
-0.0102271605175154));
#41815=CARTESIAN_POINT('Ctrl Pts',(-0.212840544211089,0.01009180188059,
-0.0103301659891579));
#41816=CARTESIAN_POINT('Ctrl Pts',(-0.212734689214167,0.0100914727163342,
-0.0103258499497599));
#41817=CARTESIAN_POINT('Ctrl Pts',(-0.213129014550153,0.0119189081838315,
-0.00934123713579647));
#41818=CARTESIAN_POINT('Ctrl Pts',(-0.213127609118038,0.0119703221605139,
-0.00943382526992674));
#41819=CARTESIAN_POINT('Ctrl Pts',(-0.21302377890995,0.0119811156556074,
-0.00942016863823821));
#41820=CARTESIAN_POINT('Ctrl Pts',(-0.213264216023343,0.0127491362730295,
-0.00875480218796601));
#41821=CARTESIAN_POINT('Ctrl Pts',(-0.213263048470919,0.0128099587344319,
-0.00884064287774012));
#41822=CARTESIAN_POINT('Ctrl Pts',(-0.21315886773292,0.0128169295168079,
-0.00882760092589079));
#41823=CARTESIAN_POINT('Ctrl Pts',(-0.213095880539431,0.00750017780359572,
-0.0104239547305089));
#41824=CARTESIAN_POINT('Ctrl Pts',(-0.213095721214129,0.00750017803487418,
-0.0104304339542255));
#41825=CARTESIAN_POINT('Ctrl Pts',(-0.213094929764227,0.00750017836281809,
-0.0104368819660783));
#41826=CARTESIAN_POINT('Ctrl Pts',(-0.213092000414212,0.00750017925173218,
-0.0104500039596521));
#41827=CARTESIAN_POINT('Ctrl Pts',(-0.213089775050135,0.00750017982542014,
-0.0104566220242013));
#41828=CARTESIAN_POINT('Ctrl Pts',(-0.213081520029726,0.00750018179525219,
-0.0104746710065114));
#41829=CARTESIAN_POINT('Ctrl Pts',(-0.213073943407876,0.00750018343903434,
-0.0104852382500818));
#41830=CARTESIAN_POINT('Ctrl Pts',(-0.213055197914078,0.00750018768424061,
-0.0105029300505066));
#41831=CARTESIAN_POINT('Ctrl Pts',(-0.213044202463265,0.00750019002608837,
-0.0105098875003991));
#41832=CARTESIAN_POINT('Ctrl Pts',(-0.213021135749935,0.00750019768070943,
-0.010518903481104));
#41833=CARTESIAN_POINT('Ctrl Pts',(-0.213010247097905,0.00750017028527798,
-0.0105209450620031));
#41834=CARTESIAN_POINT('Ctrl Pts',(-0.212998853847316,0.00750023690197873,
-0.0105214428636747));
#41835=CARTESIAN_POINT('Ctrl Pts',(-0.212996578829288,0.00750021828623935,
-0.0105215072484914));
#41836=CARTESIAN_POINT('Ctrl Pts',(-0.212994302943105,0.00750019360234278,
-0.0105214911293679));
#41837=CARTESIAN_POINT('Ctrl Pts',(-0.212993240724087,0.00750019377101382,
-0.0105214671686418));
#41838=CARTESIAN_POINT('Origin',(-0.21302517694848,0.00266870828159353,
-0.00902982701552313));
#41839=CARTESIAN_POINT('Ctrl Pts',(-0.213185740409429,0.00275371303653609,
-0.00908578925174014));
#41840=CARTESIAN_POINT('Ctrl Pts',(-0.213185612971838,0.00274961466105284,
-0.00909239231469953));
#41841=CARTESIAN_POINT('Ctrl Pts',(-0.213184693731077,0.0027448011638584,
-0.00909841346185472));
#41842=CARTESIAN_POINT('Ctrl Pts',(-0.213181219083324,0.00273341254387324,
-0.00910971911879428));
#41843=CARTESIAN_POINT('Ctrl Pts',(-0.213178536862202,0.00272684414477028,
-0.00911470522324819));
#41844=CARTESIAN_POINT('Ctrl Pts',(-0.21316990049648,0.00270900982133904,
-0.00912516750127999));
#41845=CARTESIAN_POINT('Ctrl Pts',(-0.213162790186793,0.00269692100329651,
-0.00912940390992292));
#41846=CARTESIAN_POINT('Ctrl Pts',(-0.213146385039236,0.00267275589607126,
-0.0091328790996544));
#41847=CARTESIAN_POINT('Ctrl Pts',(-0.213137764208855,0.00266140345502128,
-0.00913242932358691));
#41848=CARTESIAN_POINT('Ctrl Pts',(-0.213117330046154,0.00263679519310755,
-0.00912750922551879));
#41849=CARTESIAN_POINT('Ctrl Pts',(-0.213107598825345,0.0026266537998736,
-0.00912243605506991));
#41850=CARTESIAN_POINT('Ctrl Pts',(-0.213101358052139,0.00262048871637618,
-0.00911897368291268));
#41851=CARTESIAN_POINT('Ctrl Pts',(-0.213099233398477,0.00261829223696965,
-0.00911770722992886));
#41852=CARTESIAN_POINT('Ctrl Pts',(-0.213097116059384,0.00261614680505331,
-0.0091163440307668));
#41853=CARTESIAN_POINT('Ctrl Pts',(-0.213096483107173,0.0026155313966941,
-0.00911594470885592));
#41854=CARTESIAN_POINT('Ctrl Pts',(-0.213265658282291,0.00225057084676559,
-0.00875447521358358));
#41855=CARTESIAN_POINT('Ctrl Pts',(-0.213264744741185,0.00218980535958929,
-0.008840281993757));
#41856=CARTESIAN_POINT('Ctrl Pts',(-0.213160606268671,0.00218265689036741,
-0.00882751612497404));
#41857=CARTESIAN_POINT('Ctrl Pts',(-0.213130481910092,0.00308438824308471,
-0.00934279710406928));
#41858=CARTESIAN_POINT('Ctrl Pts',(-0.213129329004748,0.00303307556144612,
-0.00943536985701307));
#41859=CARTESIAN_POINT('Ctrl Pts',(-0.213025538625966,0.00302219748557216,
-0.00942202949690465));
#41860=CARTESIAN_POINT('Ctrl Pts',(-0.212843199480043,0.00493694441905841,
-0.0102268568625341));
#41861=CARTESIAN_POINT('Ctrl Pts',(-0.212841649873723,0.00490748256281687,
-0.0103297954986793));
#41862=CARTESIAN_POINT('Ctrl Pts',(-0.212735839420919,0.00490746467376019,
-0.0103257302283149));
#41863=CARTESIAN_POINT('Ctrl Pts',(-0.213049443549872,0.00699508177473748,
-0.0104661729567559));
#41864=CARTESIAN_POINT('Ctrl Pts',(-0.213047796796832,0.00698916624074795,
-0.0105718413687105));
#41865=CARTESIAN_POINT('Ctrl Pts',(-0.212943495631933,0.00700098597986319,
-0.0105655225132302));
#41866=CARTESIAN_POINT('Ctrl Pts',(-0.213143561380097,0.00801624880458188,
-0.0104092466932483));
#41867=CARTESIAN_POINT('Ctrl Pts',(-0.213141931039774,0.00802233257455237,
-0.0105142129384645));
#41868=CARTESIAN_POINT('Ctrl Pts',(-0.213037395151643,0.00803106171242185,
-0.0105067282758358));
#41869=CARTESIAN_POINT('Ctrl Pts',(-0.224249358614769,0.00687656461498104,
-0.0107538129648876));
#41870=CARTESIAN_POINT('Ctrl Pts',(-0.224146963941182,0.00686817072021955,
-0.0107527866925382));
#41871=CARTESIAN_POINT('Ctrl Pts',(-0.22415008400599,0.00687543328094605,
-0.0106503629663698));
#41872=CARTESIAN_POINT('Ctrl Pts',(-0.224132405324884,0.00811458583753748,
-0.0108391610128464));
#41873=CARTESIAN_POINT('Ctrl Pts',(-0.224030296549097,0.00810362852284008,
-0.0108395232823109));
#41874=CARTESIAN_POINT('Ctrl Pts',(-0.224033448292523,0.00809656786194733,
-0.0107360879252381));
#41875=CARTESIAN_POINT('Ctrl Pts',(-0.223994326444125,0.009935896587635,
-0.0105862606529491));
#41876=CARTESIAN_POINT('Ctrl Pts',(-0.223890958264787,0.00993484545827698,
-0.0105884868534941));
#41877=CARTESIAN_POINT('Ctrl Pts',(-0.223894000185458,0.00990727874800546,
-0.0104878558471313));
#41878=CARTESIAN_POINT('Ctrl Pts',(-0.224201625418445,0.0122475977142339,
-0.00950202337095844));
#41879=CARTESIAN_POINT('Ctrl Pts',(-0.224100049629042,0.0122631652037639,
-0.00949385813830566));
#41880=CARTESIAN_POINT('Ctrl Pts',(-0.224102645082168,0.0122087968339061,
-0.00940581812444462));
#41881=CARTESIAN_POINT('Ctrl Pts',(-0.224501872325241,0.0132216434216143,
-0.00877052195614289));
#41882=CARTESIAN_POINT('Ctrl Pts',(-0.224401986451628,0.0132406747202252,
-0.00875564282850734));
#41883=CARTESIAN_POINT('Ctrl Pts',(-0.224404320778191,0.0131754555245871,
-0.00867586502401968));
#41884=CARTESIAN_POINT('Ctrl Pts',(-0.224648451537749,0.0137458892845509,
-0.00827431717742288));
#41885=CARTESIAN_POINT('Ctrl Pts',(-0.224547777311868,0.0137611889470385,
-0.00826038650712441));
#41886=CARTESIAN_POINT('Ctrl Pts',(-0.224549915217777,0.0136899440670359,
-0.00818634870946614));
#41887=CARTESIAN_POINT('Ctrl Pts',(-0.224092579354373,0.00750459639810974,
-0.0106722894261828));
#41888=CARTESIAN_POINT('Ctrl Pts',(-0.224092431483114,0.00750459981467394,
-0.0106788319827509));
#41889=CARTESIAN_POINT('Ctrl Pts',(-0.224092928593908,0.00750460341211288,
-0.0106853728753318));
#41890=CARTESIAN_POINT('Ctrl Pts',(-0.224095269901901,0.00750461110036911,
-0.0106986722511323));
#41891=CARTESIAN_POINT('Ctrl Pts',(-0.224097191048441,0.00750461518650435,
-0.0107053809658855));
#41892=CARTESIAN_POINT('Ctrl Pts',(-0.224104613212024,0.00750462699508637,
-0.0107237815254526));
#41893=CARTESIAN_POINT('Ctrl Pts',(-0.224111698620084,0.0075046347420132,
-0.0107346815510102));
#41894=CARTESIAN_POINT('Ctrl Pts',(-0.224129613368251,0.00750464951718822,
-0.0107532056091582));
#41895=CARTESIAN_POINT('Ctrl Pts',(-0.224140276779664,0.00750465641897557,
-0.010760655223077));
#41896=CARTESIAN_POINT('Ctrl Pts',(-0.224171583971623,0.00750467222431416,
-0.0107745674701099));
#41897=CARTESIAN_POINT('Ctrl Pts',(-0.224188125530322,0.00750471636626934,
-0.0107744642518765));
#41898=CARTESIAN_POINT('Ctrl Pts',(-0.224190207309728,0.00750464935161598,
-0.0107745253241387));
#41899=CARTESIAN_POINT('Ctrl Pts',(-0.224190650439283,0.00750467805224881,
-0.0107745361162036));
#41900=CARTESIAN_POINT('Ctrl Pts',(-0.224391683244397,0.0131382693052084,
-0.00867392737972874));
#41901=CARTESIAN_POINT('Ctrl Pts',(-0.224391710406589,0.0131432890534471,
-0.00867985880287643));
#41902=CARTESIAN_POINT('Ctrl Pts',(-0.22439285769896,0.013148886230224,
-0.00868509490634172));
#41903=CARTESIAN_POINT('Ctrl Pts',(-0.224397561810848,0.0131621998767523,
-0.0086951017775786));
#41904=CARTESIAN_POINT('Ctrl Pts',(-0.224401502093308,0.0131698613595927,
-0.00869933153551708));
#41905=CARTESIAN_POINT('Ctrl Pts',(-0.224413834049809,0.0131895382466903,
-0.00870743881998195));
#41906=CARTESIAN_POINT('Ctrl Pts',(-0.224424065927074,0.0132024287798354,
-0.00871006714770027));
#41907=CARTESIAN_POINT('Ctrl Pts',(-0.224447199176386,0.0132267953095936,
-0.00871030365850119));
#41908=CARTESIAN_POINT('Ctrl Pts',(-0.22445892069036,0.0132375333381397,
-0.00870850297455638));
#41909=CARTESIAN_POINT('Ctrl Pts',(-0.224487116206175,0.013260687524926,
-0.00870100701881826));
#41910=CARTESIAN_POINT('Ctrl Pts',(-0.224500648747928,0.0132697575697264,
-0.00869494905955054));
#41911=CARTESIAN_POINT('Ctrl Pts',(-0.224507713074331,0.0132742734863773,
-0.0086917394312852));
#41912=CARTESIAN_POINT('Ctrl Pts',(-0.224510690885442,0.0132762579354369,
-0.00869030259956035));
#41913=CARTESIAN_POINT('Ctrl Pts',(-0.224513666456228,0.013278172374563,
-0.0086887770895996));
#41914=CARTESIAN_POINT('Ctrl Pts',(-0.224514153384766,0.0132784758635244,
-0.00868853329176699));
#41915=CARTESIAN_POINT('Origin',(-0.224556048942401,0.0132144252691754,
-0.00861251969173161));
#41916=CARTESIAN_POINT('Ctrl Pts',(-0.223392308902647,0.0131383570271638,
-0.00865324427230983));
#41917=CARTESIAN_POINT('Ctrl Pts',(-0.223391478223472,0.0131771638355724,
-0.00870046215078917));
#41918=CARTESIAN_POINT('Ctrl Pts',(-0.223356797911615,0.0132504141439465,
-0.00869020496179645));
#41919=CARTESIAN_POINT('Ctrl Pts',(-0.223310623167959,0.0132796128233705,
-0.00866507631825959));
#41920=CARTESIAN_POINT('Ctrl Pts',(-0.224149821174384,0.00813275279168254,
-0.0106496691093151));
#41921=CARTESIAN_POINT('Ctrl Pts',(-0.224146591069773,0.00814013853683756,
-0.0107523669791903));
#41922=CARTESIAN_POINT('Ctrl Pts',(-0.224249274707641,0.0081317668384709,
-0.0107532183244048));
#41923=CARTESIAN_POINT('Ctrl Pts',(-0.224033317948185,0.00691366701361902,
-0.0107364086467913));
#41924=CARTESIAN_POINT('Ctrl Pts',(-0.224030056465752,0.00690672028603269,
-0.010840132722179));
#41925=CARTESIAN_POINT('Ctrl Pts',(-0.224132456425511,0.00689578562122801,
-0.0108395948104462));
#41926=CARTESIAN_POINT('Ctrl Pts',(-0.223897696321285,0.00510558493206286,
-0.0104908606147091));
#41927=CARTESIAN_POINT('Ctrl Pts',(-0.223894541433537,0.00507809492696955,
-0.0105918081483895));
#41928=CARTESIAN_POINT('Ctrl Pts',(-0.223998190955561,0.00507719189418989,
-0.0105894436356338));
#41929=CARTESIAN_POINT('Ctrl Pts',(-0.224105481204255,0.00280599846767248,
-0.00941458749263377));
#41930=CARTESIAN_POINT('Ctrl Pts',(-0.224102774907629,0.00275163113994665,
-0.00950296080652445));
#41931=CARTESIAN_POINT('Ctrl Pts',(-0.224204631329649,0.00276739369441223,
-0.0095109790856126));
#41932=CARTESIAN_POINT('Ctrl Pts',(-0.224411021980394,0.00183980157657985,
-0.00868815989720544));
#41933=CARTESIAN_POINT('Ctrl Pts',(-0.22440857672183,0.00177455565998491,
-0.00876828274438042));
#41934=CARTESIAN_POINT('Ctrl Pts',(-0.224508648171141,0.00179410941020286,
-0.0087832681782903));
#41935=CARTESIAN_POINT('Ctrl Pts',(-0.224558348333655,0.00132533951310742,
-0.00820104779287608));
#41936=CARTESIAN_POINT('Ctrl Pts',(-0.224556097212922,0.00125406268266188,
-0.00827544837477253));
#41937=CARTESIAN_POINT('Ctrl Pts',(-0.224657001291443,0.00126972303775823,
-0.00828942184362023));
#41938=CARTESIAN_POINT('Ctrl Pts',(-0.224519311691316,0.00173702433405029,
-0.00870149897983172));
#41939=CARTESIAN_POINT('Ctrl Pts',(-0.224519220600312,0.0017372814291356,
-0.00870171019746259));
#41940=CARTESIAN_POINT('Ctrl Pts',(-0.224519216540979,0.00173728966756444,
-0.00870171692049371));
#41941=CARTESIAN_POINT('Ctrl Pts',(-0.224519209013103,0.00173730456980275,
-0.00870172907411826));
#41942=CARTESIAN_POINT('Ctrl Pts',(-0.224519205575119,0.00173731124135664,
-0.00870173451241677));
#41943=CARTESIAN_POINT('Ctrl Pts',(-0.224519199433424,0.00173732293319819,
-0.00870174403826655));
#41944=CARTESIAN_POINT('Ctrl Pts',(-0.224519196754513,0.0017373279604,-0.00870174813260198));
#41945=CARTESIAN_POINT('Ctrl Pts',(-0.224519192095841,0.00173733658188121,
-0.00870175515163127));
#41946=CARTESIAN_POINT('Ctrl Pts',(-0.22451919013177,0.0017373401807803,
-0.00870175808082501));
#41947=CARTESIAN_POINT('Ctrl Pts',(-0.224519186779857,0.00173734626334747,
-0.00870176303019058));
#41948=CARTESIAN_POINT('Ctrl Pts',(-0.224519185400549,0.00173734874963384,
-0.00870176505289937));
#41949=CARTESIAN_POINT('Ctrl Pts',(-0.224519130731885,0.00173744664577636,
-0.00870184468127068));
#41950=CARTESIAN_POINT('Ctrl Pts',(-0.224519065751737,0.00173753884306144,
-0.0087019191232117));
#41951=CARTESIAN_POINT('Ctrl Pts',(-0.2245187439025,0.00173793770533865,
-0.00870223931247735));
#41952=CARTESIAN_POINT('Ctrl Pts',(-0.224518333336278,0.00173830175620587,
-0.00870252700870189));
#41953=CARTESIAN_POINT('Ctrl Pts',(-0.22451681766982,0.00173944371920888,
-0.00870340430495714));
#41954=CARTESIAN_POINT('Ctrl Pts',(-0.224515596397644,0.00174026901686821,
-0.00870401706726192));
#41955=CARTESIAN_POINT('Ctrl Pts',(-0.22451098119199,0.00174338793721464,
-0.00870627295981185));
#41956=CARTESIAN_POINT('Ctrl Pts',(-0.224503345553201,0.00174841869489124,
-0.0087097604492813));
#41957=CARTESIAN_POINT('Ctrl Pts',(-0.224475284124318,0.00176923113819895,
-0.00871980525483996));
#41958=CARTESIAN_POINT('Ctrl Pts',(-0.224458117016968,0.00178426683852684,
-0.00872315665637135));
#41959=CARTESIAN_POINT('Ctrl Pts',(-0.224430992756243,0.00181262222784833,
-0.00872295357100595));
#41960=CARTESIAN_POINT('Ctrl Pts',(-0.224420636237042,0.00182556167036,
-0.00872033878758797));
#41961=CARTESIAN_POINT('Ctrl Pts',(-0.224408119848623,0.001845342440675,
-0.00871221470017523));
#41962=CARTESIAN_POINT('Ctrl Pts',(-0.224404106074721,0.00185306562980442,
-0.00870795611609521));
#41963=CARTESIAN_POINT('Ctrl Pts',(-0.224399315895479,0.00186647544165982,
-0.00869786436819254));
#41964=CARTESIAN_POINT('Ctrl Pts',(-0.224398146464074,0.00187210650834024,
-0.00869258439038758));
#41965=CARTESIAN_POINT('Ctrl Pts',(-0.22439811687663,0.00187715215324153,
-0.0086865994148203));
#41966=CARTESIAN_POINT('Ctrl Pts',(-0.223149962924227,0.00688159725283423,
-0.0106277838502364));
#41967=CARTESIAN_POINT('Ctrl Pts',(-0.223149018566613,0.00687388623400185,
-0.0107379305151485));
#41968=CARTESIAN_POINT('Ctrl Pts',(-0.223039601465183,0.00686565537877052,
-0.0107253915764655));
#41969=CARTESIAN_POINT('Ctrl Pts',(-0.223032133013148,0.00810963982917846,
-0.010712135585432));
#41970=CARTESIAN_POINT('Ctrl Pts',(-0.223031162244556,0.00811737830930937,
-0.0108233620581352));
#41971=CARTESIAN_POINT('Ctrl Pts',(-0.222922021349851,0.00810490151169142,
-0.0108122114891207));
#41972=CARTESIAN_POINT('Ctrl Pts',(-0.222896079921506,0.00990391154468539,
-0.0104620565626817));
#41973=CARTESIAN_POINT('Ctrl Pts',(-0.222895202078949,0.00993344674867837,
-0.0105702383938425));
#41974=CARTESIAN_POINT('Ctrl Pts',(-0.222784776813472,0.00992939962176445,
-0.010561275979829));
#41975=CARTESIAN_POINT('Ctrl Pts',(-0.223098701300928,0.0121793888445334,
-0.00940057916956953));
#41976=CARTESIAN_POINT('Ctrl Pts',(-0.22309832541927,0.0122373659809578,
-0.00949551234578024));
#41977=CARTESIAN_POINT('Ctrl Pts',(-0.222989588048026,0.0122472772909027,
-0.00947737528566851));
#41978=CARTESIAN_POINT('Ctrl Pts',(-0.223394133274712,0.0131415067565888,
-0.00868370116431274));
#41979=CARTESIAN_POINT('Ctrl Pts',(-0.223394073245122,0.0132110639533715,
-0.00876992906736614));
#41980=CARTESIAN_POINT('Ctrl Pts',(-0.223287262630516,0.013224394796061,
-0.00874500740247201));
#41981=CARTESIAN_POINT('Ctrl Pts',(-0.223543103505894,0.0136646114584795,
-0.00819237472604023));
#41982=CARTESIAN_POINT('Ctrl Pts',(-0.223543240367587,0.0137407637285344,
-0.00827241646594224));
#41983=CARTESIAN_POINT('Ctrl Pts',(-0.22343553583012,0.0137491865171251,
-0.00824924824531338));
#41984=CARTESIAN_POINT('Ctrl Pts',(-0.223092860967492,0.00750411360131228,
-0.0106501154996819));
#41985=CARTESIAN_POINT('Ctrl Pts',(-0.223092689252814,0.00750411655891282,
-0.0106565195151663));
#41986=CARTESIAN_POINT('Ctrl Pts',(-0.223091900256382,0.007504119330255,
-0.0106628920790118));
#41987=CARTESIAN_POINT('Ctrl Pts',(-0.223088988672676,0.00750412464538914,
-0.0106759407068649));
#41988=CARTESIAN_POINT('Ctrl Pts',(-0.223086764633423,0.00750412713355253,
-0.0106825582346915));
#41989=CARTESIAN_POINT('Ctrl Pts',(-0.223078514335347,0.00750413331383906,
-0.0107006061115379));
#41990=CARTESIAN_POINT('Ctrl Pts',(-0.22307094167459,0.00750413617150116,
-0.0107111737687284));
#41991=CARTESIAN_POINT('Ctrl Pts',(-0.22305220504925,0.00750413928636017,
-0.0107288662343668));
#41992=CARTESIAN_POINT('Ctrl Pts',(-0.22304121484608,0.00750413950075735,
-0.0107358244608144));
#41993=CARTESIAN_POINT('Ctrl Pts',(-0.223016540981556,0.00750413733438505,
-0.01074547417355));
#41994=CARTESIAN_POINT('Ctrl Pts',(-0.223004164996846,0.00750411469378559,
-0.0107474049779053));
#41995=CARTESIAN_POINT('Ctrl Pts',(-0.222992339708995,0.00750413754074494,
-0.0107474330725274));
#41996=CARTESIAN_POINT('Ctrl Pts',(-0.222991913153699,0.00750413853913309,
-0.0107474311162282));
#41997=CARTESIAN_POINT('Ctrl Pts',(-0.222991332215326,0.00750414349283911,
-0.0107474252051021));
#41998=CARTESIAN_POINT('Ctrl Pts',(-0.222991075316954,0.00750414620344912,
-0.0107474218012963));
#41999=CARTESIAN_POINT('Ctrl Pts',(-0.222990721887929,0.0075041585497481,
-0.0107474159745127));
#42000=CARTESIAN_POINT('Ctrl Pts',(-0.222990363822996,0.00750425357435802,
-0.0107474086907247));
#42001=CARTESIAN_POINT('Origin',(-0.223237220057076,0.00179857992405682,
-0.00859864314724398));
#42002=CARTESIAN_POINT('Ctrl Pts',(-0.223398256964007,0.00187628033601208,
-0.00866522709035868));
#42003=CARTESIAN_POINT('Ctrl Pts',(-0.223398154124069,0.00187143799250317,
-0.00867114607163627));
#42004=CARTESIAN_POINT('Ctrl Pts',(-0.223397350846328,0.00186597106090046,
-0.00867642715907607));
#42005=CARTESIAN_POINT('Ctrl Pts',(-0.223394293473877,0.00185343700847406,
-0.00868604789434846));
#42006=CARTESIAN_POINT('Ctrl Pts',(-0.223391931127745,0.0018464009619336,
-0.00869012656777989));
#42007=CARTESIAN_POINT('Ctrl Pts',(-0.223383990852377,0.0018269365722086,
-0.00869852527535584));
#42008=CARTESIAN_POINT('Ctrl Pts',(-0.223377431966919,0.00181434780212607,
-0.00870103413584041));
#42009=CARTESIAN_POINT('Ctrl Pts',(-0.223362558207148,0.00178986818748107,
-0.00870155486970696));
#42010=CARTESIAN_POINT('Ctrl Pts',(-0.223354229968575,0.00177799425123853,
-0.00869951688709378));
#42011=CARTESIAN_POINT('Ctrl Pts',(-0.22333313535445,0.00175125673571012,
-0.00869015734281729));
#42012=CARTESIAN_POINT('Ctrl Pts',(-0.22332294719884,0.00174102013770642,
-0.00868214080278602));
#42013=CARTESIAN_POINT('Ctrl Pts',(-0.223319160138154,0.00173753989374147,
-0.00867940971146196));
#42014=CARTESIAN_POINT('Ctrl Pts',(-0.223318489660597,0.00173675249287678,
-0.00867877460776524));
#42015=CARTESIAN_POINT('Ctrl Pts',(-0.223317594518492,0.00173570789287372,
-0.0086779195615712));
#42016=CARTESIAN_POINT('Ctrl Pts',(-0.223316845454304,0.00173498134307272,
-0.00867730420572105));
#42017=CARTESIAN_POINT('Ctrl Pts',(-0.22303890850229,0.00814164430623871,
-0.0107248133017441));
#42018=CARTESIAN_POINT('Ctrl Pts',(-0.223148789072647,0.00813348754910934,
-0.0107379204692242));
#42019=CARTESIAN_POINT('Ctrl Pts',(-0.223149727731801,0.00812565130849946,
-0.0106272611136563));
#42020=CARTESIAN_POINT('Ctrl Pts',(-0.22292134689892,0.00690441691685615,
-0.010812507614285));
#42021=CARTESIAN_POINT('Ctrl Pts',(-0.223030955661194,0.00689190154903563,
-0.0108242264473683));
#42022=CARTESIAN_POINT('Ctrl Pts',(-0.223031920968427,0.00689956170670937,
-0.010712472343137));
#42023=CARTESIAN_POINT('Ctrl Pts',(-0.222788348228539,0.00508263051192417,
-0.0105641367381816));
#42024=CARTESIAN_POINT('Ctrl Pts',(-0.222899223939067,0.00507857159790477,
-0.0105737078620945));
#42025=CARTESIAN_POINT('Ctrl Pts',(-0.222900097730721,0.00510809073197549,
-0.0104649776228588));
#42026=CARTESIAN_POINT('Ctrl Pts',(-0.222991460019885,0.00276656231961293,
-0.0094855610854456));
#42027=CARTESIAN_POINT('Ctrl Pts',(-0.223100667398899,0.00277626708247984,
-0.0095041815587128));
#42028=CARTESIAN_POINT('Ctrl Pts',(-0.22310103778877,0.00283435031683848,
-0.00940870301260069));
#42029=CARTESIAN_POINT('Ctrl Pts',(-0.223292840953927,0.00179022353787926,
-0.00875673827642576));
#42030=CARTESIAN_POINT('Ctrl Pts',(-0.223400003218155,0.00180370409004607,
-0.00878241709270048));
#42031=CARTESIAN_POINT('Ctrl Pts',(-0.223400057319882,0.00187340518877495,
-0.00869563469557495));
#42032=CARTESIAN_POINT('Ctrl Pts',(-0.223442953334174,0.00126547903518434,
-0.00826334125889978));
#42033=CARTESIAN_POINT('Ctrl Pts',(-0.22355106295208,0.00127380217909774,
-0.00828714426754558));
#42034=CARTESIAN_POINT('Ctrl Pts',(-0.223550922316616,0.00135012429573583,
-0.00820654454718633));
#42035=CARTESIAN_POINT('Ctrl Pts',(-0.212223744032557,0.0125025714233182,
-0.00890371716457249));
#42036=CARTESIAN_POINT('Ctrl Pts',(-0.212222075153114,0.0125578143517975,
-0.00898781500481288));
#42037=CARTESIAN_POINT('Ctrl Pts',(-0.212321835550297,0.0125473597144221,
-0.00899591238820372));
#42038=CARTESIAN_POINT('Ctrl Pts',(-0.212102724242109,0.0117434852742709,
-0.00940161356959696));
#42039=CARTESIAN_POINT('Ctrl Pts',(-0.2121008512821,0.011790384772016,-0.00949119962975025));
#42040=CARTESIAN_POINT('Ctrl Pts',(-0.212200537118151,0.0117786534455685,
-0.00949867729488359));
#42041=CARTESIAN_POINT('Ctrl Pts',(-0.21186514967656,0.0100599062468189,
-0.0101749354638583));
#42042=CARTESIAN_POINT('Ctrl Pts',(-0.211862990722436,0.0100880414368075,
-0.010273079418359));
#42043=CARTESIAN_POINT('Ctrl Pts',(-0.211964249557042,0.0100869126121601,
-0.0102726729652089));
#42044=CARTESIAN_POINT('Ctrl Pts',(-0.212031119293791,0.00821222072325896,
-0.010417780967713));
#42045=CARTESIAN_POINT('Ctrl Pts',(-0.212028829701335,0.00822031116530004,
-0.0105185764981024));
#42046=CARTESIAN_POINT('Ctrl Pts',(-0.212128989819408,0.00822998234265434,
-0.010519447140182));
#42047=CARTESIAN_POINT('Ctrl Pts',(-0.212114323073989,0.00730098728432662,
-0.0103993599395582));
#42048=CARTESIAN_POINT('Ctrl Pts',(-0.212112040942403,0.00729885878555155,
-0.0104999410658259));
#42049=CARTESIAN_POINT('Ctrl Pts',(-0.212212246789137,0.00730790211731437,
-0.0105017797457116));
#42050=CARTESIAN_POINT('Ctrl Pts',(-0.212096204769044,0.0075000580009567,
-0.0104011630123803));
#42051=CARTESIAN_POINT('Ctrl Pts',(-0.212096056852805,0.00750005816148503,
-0.01040770818223));
#42052=CARTESIAN_POINT('Ctrl Pts',(-0.212096554695983,0.00750005821014383,
-0.0104142516334717));
#42053=CARTESIAN_POINT('Ctrl Pts',(-0.212098899076221,0.0075000580878504,
-0.0104275562750958));
#42054=CARTESIAN_POINT('Ctrl Pts',(-0.21210082269123,0.00750005790295219,
-0.0104342675106612));
#42055=CARTESIAN_POINT('Ctrl Pts',(-0.212108252487303,0.0075000570574498,
-0.0104526705817974));
#42056=CARTESIAN_POINT('Ctrl Pts',(-0.212115343160954,0.00750005612495993,
-0.0104635696258613));
#42057=CARTESIAN_POINT('Ctrl Pts',(-0.212133268656717,0.00750005380450097,
-0.0104820909648401));
#42058=CARTESIAN_POINT('Ctrl Pts',(-0.212143937749959,0.00750005232560142,
-0.010489538526628));
#42059=CARTESIAN_POINT('Ctrl Pts',(-0.212165860746876,0.00750005060557715,
-0.0104992724855804));
#42060=CARTESIAN_POINT('Ctrl Pts',(-0.212176657990042,0.00750003194978452,
-0.0105020589538083));
#42061=CARTESIAN_POINT('Ctrl Pts',(-0.212189859904008,0.00750006809023092,
-0.0105032346276707));
#42062=CARTESIAN_POINT('Ctrl Pts',(-0.212192126960573,0.00750004200194685,
-0.0105033609494816));
#42063=CARTESIAN_POINT('Ctrl Pts',(-0.212194328823658,0.00750004157488686,
-0.0105034107592895));
#42064=CARTESIAN_POINT('Ctrl Pts',(-0.21218385926235,0.0122487198827948,
-0.00906545454917522));
#42065=CARTESIAN_POINT('Ctrl Pts',(-0.212183827797059,0.0122526842341265,
-0.00907170643872819));
#42066=CARTESIAN_POINT('Ctrl Pts',(-0.212184731565329,0.0122572705102556,
-0.00907742635298329));
#42067=CARTESIAN_POINT('Ctrl Pts',(-0.212188538992215,0.0122683657498729,
-0.00908864426940098));
#42068=CARTESIAN_POINT('Ctrl Pts',(-0.212191722914003,0.0122748939085551,
-0.00909371908495357));
#42069=CARTESIAN_POINT('Ctrl Pts',(-0.212202056114265,0.0122924621358694,
-0.00910451018441334));
#42070=CARTESIAN_POINT('Ctrl Pts',(-0.212210818437941,0.0123044575381293,
-0.00910910546837787));
#42071=CARTESIAN_POINT('Ctrl Pts',(-0.212231927329752,0.0123291664640641,
-0.00911359453592));
#42072=CARTESIAN_POINT('Ctrl Pts',(-0.212243486433075,0.0123410475842637,
-0.00911346132650099));
#42073=CARTESIAN_POINT('Ctrl Pts',(-0.212272773255435,0.0123683538825616,
-0.00910877928464044));
#42074=CARTESIAN_POINT('Ctrl Pts',(-0.212287224212214,0.0123794352589682,
-0.00910270522660073));
#42075=CARTESIAN_POINT('Ctrl Pts',(-0.212292284315582,0.0123831279553651,
-0.00910069980871974));
#42076=CARTESIAN_POINT('Ctrl Pts',(-0.212293389463492,0.012384053549551,
-0.00910017313244616));
#42077=CARTESIAN_POINT('Ctrl Pts',(-0.212294871275834,0.0123852874724164,
-0.00909945683622047));
#42078=CARTESIAN_POINT('Ctrl Pts',(-0.212296027595393,0.0123861510372385,
-0.009098937945711));
#42079=CARTESIAN_POINT('Origin',(-0.21234693243841,0.0123329390950867,-0.00901527903468506));
#42080=CARTESIAN_POINT('Ctrl Pts',(-0.211183468881297,0.0122495385747751,
-0.00904367844858987));
#42081=CARTESIAN_POINT('Ctrl Pts',(-0.211183343796021,0.0122535585151899,
-0.00905017738989069));
#42082=CARTESIAN_POINT('Ctrl Pts',(-0.211182453405063,0.0122582724090962,
-0.0090561153782017));
#42083=CARTESIAN_POINT('Ctrl Pts',(-0.211179090245664,0.0122694120307349,
-0.00906728735112201));
#42084=CARTESIAN_POINT('Ctrl Pts',(-0.211176496173649,0.0122758323451357,
-0.00907223640641804));
#42085=CARTESIAN_POINT('Ctrl Pts',(-0.211168070280735,0.0122934113463099,
-0.00908276662220862));
#42086=CARTESIAN_POINT('Ctrl Pts',(-0.211161074881815,0.0123054047079806,
-0.00908710442762168));
#42087=CARTESIAN_POINT('Ctrl Pts',(-0.211144770725815,0.0123296125141419,
-0.00909085366891658));
#42088=CARTESIAN_POINT('Ctrl Pts',(-0.211136106097826,0.0123410951196305,
-0.00909049964893237));
#42089=CARTESIAN_POINT('Ctrl Pts',(-0.211116251718935,0.0123651604647786,
-0.00908587455126835));
#42090=CARTESIAN_POINT('Ctrl Pts',(-0.211106531274097,0.0123754212444389,
-0.00908112970234405));
#42091=CARTESIAN_POINT('Ctrl Pts',(-0.211099292974643,0.0123828819846203,
-0.00907697188113588));
#42092=CARTESIAN_POINT('Ctrl Pts',(-0.211097175768363,0.0123849684867918,
-0.00907577873419521));
#42093=CARTESIAN_POINT('Ctrl Pts',(-0.211095050524522,0.0123869971186745,
-0.00907450260566078));
#42094=CARTESIAN_POINT('Ctrl Pts',(-0.211094251609883,0.0123877761518248,
-0.00907399894463725));
#42095=CARTESIAN_POINT('Ctrl Pts',(-0.212122639608489,0.00778880978652429,
-0.0103971099742313));
#42096=CARTESIAN_POINT('Ctrl Pts',(-0.212120360088168,0.00779194299561869,
-0.0104975869020762));
#42097=CARTESIAN_POINT('Ctrl Pts',(-0.212220489784696,0.00778295730589407,
-0.0104996007168518));
#42098=CARTESIAN_POINT('Ctrl Pts',(-0.212036322893619,0.00684878518939332,
-0.0104254825969592));
#42099=CARTESIAN_POINT('Ctrl Pts',(-0.212034031410779,0.00684136848125649,
-0.0105262845556704));
#42100=CARTESIAN_POINT('Ctrl Pts',(-0.212134071486609,0.00683127857741346,
-0.0105272683569319));
#42101=CARTESIAN_POINT('Ctrl Pts',(-0.211859116564673,0.00494160052946475,
-0.0101852940024049));
#42102=CARTESIAN_POINT('Ctrl Pts',(-0.211856956852588,0.00491351503003851,
-0.0102834759349862));
#42103=CARTESIAN_POINT('Ctrl Pts',(-0.211958176675694,0.00491482182811779,
-0.0102830491123946));
#42104=CARTESIAN_POINT('Ctrl Pts',(-0.212112373295386,0.0032005167473659,
-0.00937556293289828));
#42105=CARTESIAN_POINT('Ctrl Pts',(-0.212110512545602,0.00315302214095645,
-0.00946478708467834));
#42106=CARTESIAN_POINT('Ctrl Pts',(-0.212210070325435,0.00316501813895363,
-0.00947257547566129));
#42107=CARTESIAN_POINT('Ctrl Pts',(-0.212236649846315,0.00242474532205975,
-0.00885552488235436));
#42108=CARTESIAN_POINT('Ctrl Pts',(-0.212235002070394,0.00236874779667176,
-0.00893902616285966));
#42109=CARTESIAN_POINT('Ctrl Pts',(-0.212334697644786,0.00237898510803345,
-0.00894721593752821));
#42110=CARTESIAN_POINT('Ctrl Pts',(-0.212297192971603,0.00261509486573022,
-0.0090997425089851));
#42111=CARTESIAN_POINT('Ctrl Pts',(-0.212296110945992,0.00261590407640106,
-0.00910022856999239));
#42112=CARTESIAN_POINT('Ctrl Pts',(-0.212293412623576,0.00261789339678241,
-0.0091013849447997));
#42113=CARTESIAN_POINT('Ctrl Pts',(-0.21229072211904,0.00261994008618735,
-0.00910246433139768));
#42114=CARTESIAN_POINT('Ctrl Pts',(-0.212279944466258,0.00262844975228672,
-0.00910683558573018));
#42115=CARTESIAN_POINT('Ctrl Pts',(-0.212267736210671,0.00263855465871684,
-0.00911073569201036));
#42116=CARTESIAN_POINT('Ctrl Pts',(-0.212243429959653,0.00266148531971882,
-0.00911429271001131));
#42117=CARTESIAN_POINT('Ctrl Pts',(-0.212232378426442,0.00267293677256201,
-0.00911430297192282));
#42118=CARTESIAN_POINT('Ctrl Pts',(-0.212211756375655,0.00269716377811193,
-0.00910982811301855));
#42119=CARTESIAN_POINT('Ctrl Pts',(-0.21220305063021,0.00270912604835164,
-0.00910521030688519));
#42120=CARTESIAN_POINT('Ctrl Pts',(-0.212192809462358,0.00272661431929928,
-0.00909441411988624));
#42121=CARTESIAN_POINT('Ctrl Pts',(-0.212189662427839,0.00273309690234965,
-0.00908935613340753));
#42122=CARTESIAN_POINT('Ctrl Pts',(-0.212185900147284,0.00274411373944175,
-0.00907819293916975));
#42123=CARTESIAN_POINT('Ctrl Pts',(-0.21218500728268,0.00274866811026422,
-0.00907250584239902));
#42124=CARTESIAN_POINT('Ctrl Pts',(-0.212185037759281,0.00275260737022776,
-0.00906629345677396));
#42125=CARTESIAN_POINT('Ctrl Pts',(-0.211142485728535,0.00699254756608383,
-0.0103648734390101));
#42126=CARTESIAN_POINT('Ctrl Pts',(-0.211140615484092,0.00698654179680735,
-0.0104703120129651));
#42127=CARTESIAN_POINT('Ctrl Pts',(-0.211035650260988,0.00697789315409504,
-0.0104621222159787));
#42128=CARTESIAN_POINT('Ctrl Pts',(-0.21105098460499,0.00801203950050848,
-0.0104201724986889));
#42129=CARTESIAN_POINT('Ctrl Pts',(-0.211049098611664,0.0080180188886255,
-0.0105262966533945));
#42130=CARTESIAN_POINT('Ctrl Pts',(-0.210944361367469,0.00800640351237446,
-0.010519208094519));
#42131=CARTESIAN_POINT('Ctrl Pts',(-0.21084304256263,0.0100629658036953,
-0.0101824905154317));
#42132=CARTESIAN_POINT('Ctrl Pts',(-0.210841251020845,0.0100924675827056,
-0.0102859051076613));
#42133=CARTESIAN_POINT('Ctrl Pts',(-0.210735015997111,0.0100917271809107,
-0.0102812652497566));
#42134=CARTESIAN_POINT('Ctrl Pts',(-0.211127758772214,0.0119207402552615,
-0.00929899445208153));
#42135=CARTESIAN_POINT('Ctrl Pts',(-0.211126372276215,0.0119721993876384,
-0.0093920197491322));
#42136=CARTESIAN_POINT('Ctrl Pts',(-0.211022169348734,0.0119829372674086,
-0.00937797181211293));
#42137=CARTESIAN_POINT('Ctrl Pts',(-0.211263625788997,0.0127522795019374,
-0.00871403619118547));
#42138=CARTESIAN_POINT('Ctrl Pts',(-0.211262479217963,0.0128131718323431,
-0.00880032500501877));
#42139=CARTESIAN_POINT('Ctrl Pts',(-0.211157922926716,0.0128199712353316,
-0.00878693220959459));
#42140=CARTESIAN_POINT('Ctrl Pts',(-0.211096536156126,0.00750001934821516,
-0.0103787795142135));
#42141=CARTESIAN_POINT('Ctrl Pts',(-0.211096376187743,0.00750001946084664,
-0.0103852544749745));
#42142=CARTESIAN_POINT('Ctrl Pts',(-0.211095584978032,0.00750001968840412,
-0.0103916982231778));
#42143=CARTESIAN_POINT('Ctrl Pts',(-0.211092657009911,0.00750002040873107,
-0.0104048157068072));
#42144=CARTESIAN_POINT('Ctrl Pts',(-0.211090432074856,0.00750002091781133,
-0.0104114334162529));
#42145=CARTESIAN_POINT('Ctrl Pts',(-0.211082178394124,0.00750002276793853,
-0.010429482029809));
#42146=CARTESIAN_POINT('Ctrl Pts',(-0.211074602730834,0.00750002441393692,
-0.0104400494546364));
#42147=CARTESIAN_POINT('Ctrl Pts',(-0.211055859246741,0.00750002879137767,
-0.010457741705717));
#42148=CARTESIAN_POINT('Ctrl Pts',(-0.211044864897043,0.00750003127898264,
-0.0104646995036328));
#42149=CARTESIAN_POINT('Ctrl Pts',(-0.211020920185128,0.00750003942093849,
-0.0104740601580318));
#42150=CARTESIAN_POINT('Ctrl Pts',(-0.211009741601578,0.00750002059763051,
-0.0104758093131767));
#42151=CARTESIAN_POINT('Ctrl Pts',(-0.210998442893526,0.00750008203547272,
-0.0104763032297964));
#42152=CARTESIAN_POINT('Ctrl Pts',(-0.210996045383314,0.0075000361891443,
-0.0104763287856277));
#42153=CARTESIAN_POINT('Ctrl Pts',(-0.210993906189512,0.00750003658947422,
-0.0104762805591888));
#42154=CARTESIAN_POINT('Origin',(-0.211023786144693,0.00266742943825413,
-0.00898917183642173));
#42155=CARTESIAN_POINT('Ctrl Pts',(-0.211184235669001,0.00275259873665137,
-0.00904500540329008));
#42156=CARTESIAN_POINT('Ctrl Pts',(-0.211184108309872,0.00274851237207321,
-0.00905161691332531));
#42157=CARTESIAN_POINT('Ctrl Pts',(-0.211183188947385,0.00274370938574701,
-0.00905764748316005));
#42158=CARTESIAN_POINT('Ctrl Pts',(-0.211179713684398,0.00273233943804887,
-0.00906897486538284));
#42159=CARTESIAN_POINT('Ctrl Pts',(-0.211177030906755,0.00272577864903201,
-0.00907397300667125));
#42160=CARTESIAN_POINT('Ctrl Pts',(-0.211168393401542,0.00270795989164768,
-0.00908446663829167));
#42161=CARTESIAN_POINT('Ctrl Pts',(-0.211161282430324,0.00269587613625519,
-0.00908872380984227));
#42162=CARTESIAN_POINT('Ctrl Pts',(-0.211144763685762,0.00267154571914486,
-0.00909226395652573));
#42163=CARTESIAN_POINT('Ctrl Pts',(-0.211136007252681,0.00266002880499524,
-0.00909179650619916));
#42164=CARTESIAN_POINT('Ctrl Pts',(-0.211114293659952,0.00263393192613597,
-0.00908649757919211));
#42165=CARTESIAN_POINT('Ctrl Pts',(-0.21110391131705,0.00262337571113696,
-0.00908068371600419));
#42166=CARTESIAN_POINT('Ctrl Pts',(-0.211098093898507,0.00261770147937051,
-0.00907744793165228));
#42167=CARTESIAN_POINT('Ctrl Pts',(-0.211096595484061,0.00261601608586272,
-0.00907641942581189));
#42168=CARTESIAN_POINT('Ctrl Pts',(-0.211094980169537,0.0026144429765102,
-0.00907540295747494));
#42169=CARTESIAN_POINT('Ctrl Pts',(-0.211264251736995,0.00224882937558932,
-0.00871473025010786));
#42170=CARTESIAN_POINT('Ctrl Pts',(-0.211263315213782,0.00218803254801025,
-0.00880095577930301));
#42171=CARTESIAN_POINT('Ctrl Pts',(-0.211158843112418,0.00218106932820431,
-0.00878785654339923));
#42172=CARTESIAN_POINT('Ctrl Pts',(-0.211128629078001,0.00308374196045554,
-0.00930120455681559));
#42173=CARTESIAN_POINT('Ctrl Pts',(-0.211127451514235,0.0030324147703501,
-0.00939417776413184));
#42174=CARTESIAN_POINT('Ctrl Pts',(-0.211023329710713,0.0030216079367658,
-0.00938046250689989));
#42175=CARTESIAN_POINT('Ctrl Pts',(-0.210843656731025,0.00493713697694662,
-0.0101823031690562));
#42176=CARTESIAN_POINT('Ctrl Pts',(-0.210842079736846,0.00490766886678799,
-0.0102856076466288));
#42177=CARTESIAN_POINT('Ctrl Pts',(-0.210735934247016,0.00490808327359709,
-0.0102812256263012));
#42178=CARTESIAN_POINT('Ctrl Pts',(-0.211051060565633,0.00699481541135514,
-0.0104208672824074));
#42179=CARTESIAN_POINT('Ctrl Pts',(-0.211049386046545,0.00698889960147933,
-0.0105268935653299));
#42180=CARTESIAN_POINT('Ctrl Pts',(-0.210944743332313,0.00700060848094322,
-0.0105201436677757));
#42181=CARTESIAN_POINT('Ctrl Pts',(-0.211143590272674,0.00801614047287985,
-0.010364127037553));
#42182=CARTESIAN_POINT('Ctrl Pts',(-0.211141932328472,0.00802222390702669,
-0.0104694534195357));
#42183=CARTESIAN_POINT('Ctrl Pts',(-0.211037055788434,0.00803088427681597,
-0.0104615756474694));
#42184=CARTESIAN_POINT('Ctrl Pts',(-0.202265290724368,0.0127832636642769,
-0.00852006183626685));
#42185=CARTESIAN_POINT('Ctrl Pts',(-0.202262909678109,0.012841850283284,
-0.00860438640498691));
#42186=CARTESIAN_POINT('Ctrl Pts',(-0.202364791393614,0.0128310798128724,
-0.0086115609851021));
#42187=CARTESIAN_POINT('Ctrl Pts',(-0.202126399278693,0.0119512167802099,
-0.00909768849379822));
#42188=CARTESIAN_POINT('Ctrl Pts',(-0.202123771768196,0.012000709183594,
-0.00918838710668978));
#42189=CARTESIAN_POINT('Ctrl Pts',(-0.202225304576364,0.0119862994107232,
-0.00919586084607411));
#42190=CARTESIAN_POINT('Ctrl Pts',(-0.201846781273398,0.0100683927693504,
-0.0099854198429024));
#42191=CARTESIAN_POINT('Ctrl Pts',(-0.201843792519172,0.0100967254867997,
-0.0100860378814493));
#42192=CARTESIAN_POINT('Ctrl Pts',(-0.201947320966196,0.0100968345400587,
-0.0100833761264778));
#42193=CARTESIAN_POINT('Ctrl Pts',(-0.202060563303902,0.00799480983044915,
-0.0102172781045443));
#42194=CARTESIAN_POINT('Ctrl Pts',(-0.202057447540456,0.00800043688524475,
-0.0103204296036954));
#42195=CARTESIAN_POINT('Ctrl Pts',(-0.202159609967776,0.00801057803168537,
-0.0103203078618906));
#42196=CARTESIAN_POINT('Ctrl Pts',(-0.202143369671317,0.00697652998217102,
-0.0101604268468326));
#42197=CARTESIAN_POINT('Ctrl Pts',(-0.202140278060583,0.00697067620638285,
-0.0102629252905548));
#42198=CARTESIAN_POINT('Ctrl Pts',(-0.20224266649913,0.00697898140682514,
-0.0102637635116727));
#42199=CARTESIAN_POINT('Ctrl Pts',(-0.202099470462991,0.00750048539628712,
-0.0101752292159335));
#42200=CARTESIAN_POINT('Ctrl Pts',(-0.202099322575853,0.00750048571666395,
-0.0101817727997466));
#42201=CARTESIAN_POINT('Ctrl Pts',(-0.20209981982129,0.0075004858146974,
-0.0101883147240483));
#42202=CARTESIAN_POINT('Ctrl Pts',(-0.20210216172605,0.00750048555557407,
-0.010201616141842));
#42203=CARTESIAN_POINT('Ctrl Pts',(-0.202104083353711,0.00750048516985556,
-0.0102083258634756));
#42204=CARTESIAN_POINT('Ctrl Pts',(-0.202111506517437,0.00750048337028386,
-0.0102267268383148));
#42205=CARTESIAN_POINT('Ctrl Pts',(-0.202118592045866,0.00750048137816934,
-0.0102376264068436));
#42206=CARTESIAN_POINT('Ctrl Pts',(-0.202136506508522,0.00750047596863676,
-0.0102561490420348));
#42207=CARTESIAN_POINT('Ctrl Pts',(-0.202147169384737,0.00750047260069426,
-0.0102635978567623));
#42208=CARTESIAN_POINT('Ctrl Pts',(-0.202174878281523,0.00750046356239206,
-0.010275909799322));
#42209=CARTESIAN_POINT('Ctrl Pts',(-0.202188847780365,0.00750044923868025,
-0.0102772242529343));
#42210=CARTESIAN_POINT('Ctrl Pts',(-0.202197059864926,0.00750045701803727,
-0.0102774632695266));
#42211=CARTESIAN_POINT('Ctrl Pts',(-0.202197548253278,0.00750045578297359,
-0.0102774753489076));
#42212=CARTESIAN_POINT('Ctrl Pts',(-0.202180802979017,0.0122592813346522,
-0.00885976042488077));
#42213=CARTESIAN_POINT('Ctrl Pts',(-0.202180775847905,0.0122631848049861,
-0.00886603768293643));
#42214=CARTESIAN_POINT('Ctrl Pts',(-0.202181681606649,0.0122677133629349,
-0.00887178950452203));
#42215=CARTESIAN_POINT('Ctrl Pts',(-0.202185493168263,0.0122787039443237,
-0.00888310262482018));
#42216=CARTESIAN_POINT('Ctrl Pts',(-0.202188683106617,0.0122851909308943,
-0.00888823749218621));
#42217=CARTESIAN_POINT('Ctrl Pts',(-0.202199031228896,0.012302669305196,
-0.00889918392779031));
#42218=CARTESIAN_POINT('Ctrl Pts',(-0.202207803768514,0.0123146277241332,
-0.00890388368097754));
#42219=CARTESIAN_POINT('Ctrl Pts',(-0.202229052741313,0.0123394414366878,
-0.00890861211537678));
#42220=CARTESIAN_POINT('Ctrl Pts',(-0.202240765246994,0.0123514568709592,
-0.00890855459003177));
#42221=CARTESIAN_POINT('Ctrl Pts',(-0.202270373507782,0.0123790254521622,
-0.00890396725067058));
#42222=CARTESIAN_POINT('Ctrl Pts',(-0.202284941527497,0.0123902440180487,
-0.00889785858207483));
#42223=CARTESIAN_POINT('Ctrl Pts',(-0.202290001326585,0.0123938505451035,
-0.00889591408271268));
#42224=CARTESIAN_POINT('Ctrl Pts',(-0.202290902964131,0.0123946426922635,
-0.00889546575730262));
#42225=CARTESIAN_POINT('Ctrl Pts',(-0.202292112602265,0.0123957005749798,
-0.00889485866884196));
#42226=CARTESIAN_POINT('Ctrl Pts',(-0.202293077439418,0.0123964246955439,
-0.00889443257618142));
#42227=CARTESIAN_POINT('Origin',(-0.202343912991874,0.0123440163406885,
-0.00881026170755109));
#42228=CARTESIAN_POINT('Ctrl Pts',(-0.201180514909525,0.0122597855112167,
-0.00883836470388977));
#42229=CARTESIAN_POINT('Ctrl Pts',(-0.201180390511959,0.0122637441796246,
-0.00884489930376825));
#42230=CARTESIAN_POINT('Ctrl Pts',(-0.201179501260221,0.0122684013630966,
-0.00885088006671312));
#42231=CARTESIAN_POINT('Ctrl Pts',(-0.201176141270069,0.0122794323622778,
-0.00886215414657635));
#42232=CARTESIAN_POINT('Ctrl Pts',(-0.201173549386715,0.0122858033738214,
-0.00886716297674856));
#42233=CARTESIAN_POINT('Ctrl Pts',(-0.201165128329775,0.0123032779251533,
-0.00887786039664943));
#42234=CARTESIAN_POINT('Ctrl Pts',(-0.201158135612939,0.0123152267687501,
-0.00888231322892227));
#42235=CARTESIAN_POINT('Ctrl Pts',(-0.201141838373897,0.0123393891695866,
-0.00888629578960458));
#42236=CARTESIAN_POINT('Ctrl Pts',(-0.201133177159222,0.0123508700904303,
-0.00888605332684157));
#42237=CARTESIAN_POINT('Ctrl Pts',(-0.201113045567628,0.0123753147450016,
-0.00888159927525391));
#42238=CARTESIAN_POINT('Ctrl Pts',(-0.201103352145789,0.0123855377193998,
-0.00887687172049721));
#42239=CARTESIAN_POINT('Ctrl Pts',(-0.201096412597187,0.0123927376362332,
-0.00887294806780029));
#42240=CARTESIAN_POINT('Ctrl Pts',(-0.20109426545364,0.0123948624411427,
-0.00887176173410875));
#42241=CARTESIAN_POINT('Ctrl Pts',(-0.201092109876422,0.0123969273961565,
-0.0088704880551081));
#42242=CARTESIAN_POINT('Ctrl Pts',(-0.201091342169912,0.0123976805086701,
-0.00887001123180993));
#42243=CARTESIAN_POINT('Ctrl Pts',(-0.202361917638471,0.00217353042035395,
-0.00861470493313823));
#42244=CARTESIAN_POINT('Ctrl Pts',(-0.202259856285326,0.00216286571190057,
-0.00860743380920193));
#42245=CARTESIAN_POINT('Ctrl Pts',(-0.202262561385939,0.00222152827281342,
-0.0085229612533595));
#42246=CARTESIAN_POINT('Ctrl Pts',(-0.202223288299755,0.00301801026424016,
-0.00919806500274725));
#42247=CARTESIAN_POINT('Ctrl Pts',(-0.202121575048064,0.00300371014208909,
-0.0091904858511563));
#42248=CARTESIAN_POINT('Ctrl Pts',(-0.202124525544528,0.0030532785590825,
-0.0090996406391749));
#42249=CARTESIAN_POINT('Ctrl Pts',(-0.201945891174042,0.00490640788157693,
-0.010083958182011));
#42250=CARTESIAN_POINT('Ctrl Pts',(-0.201842188963288,0.00490652939523789,
-0.0100864703603933));
#42251=CARTESIAN_POINT('Ctrl Pts',(-0.201845506877496,0.00493487034859226,
-0.00998567581196493));
#42252=CARTESIAN_POINT('Ctrl Pts',(-0.202159089889202,0.00699079557499788,
-0.0103202697089951));
#42253=CARTESIAN_POINT('Ctrl Pts',(-0.202056762552271,0.00700105132225664,
-0.0103202502333414));
#42254=CARTESIAN_POINT('Ctrl Pts',(-0.20206020309972,0.00700663927775264,
-0.0102169335833552));
#42255=CARTESIAN_POINT('Ctrl Pts',(-0.20224286412263,0.00802148069263829,
-0.0102637453647374));
#42256=CARTESIAN_POINT('Ctrl Pts',(-0.202140309173562,0.0080298578112884,
-0.0102627524167362));
#42257=CARTESIAN_POINT('Ctrl Pts',(-0.202143726326102,0.00802396304981702,
-0.0101600928451061));
#42258=CARTESIAN_POINT('Ctrl Pts',(-0.20229073304026,0.00260802933164804,
-0.00889712262070968));
#42259=CARTESIAN_POINT('Ctrl Pts',(-0.202289712354061,0.00260879620236029,
-0.00889757326702722));
#42260=CARTESIAN_POINT('Ctrl Pts',(-0.202286953018036,0.00261083227107042,
-0.00889873350857407));
#42261=CARTESIAN_POINT('Ctrl Pts',(-0.202284199630092,0.00261293162289047,
-0.0088998116244581));
#42262=CARTESIAN_POINT('Ctrl Pts',(-0.202274881790007,0.0026203321779655,
-0.00890352576831182));
#42263=CARTESIAN_POINT('Ctrl Pts',(-0.202262295585051,0.00263060385711503,
-0.00890774115835158));
#42264=CARTESIAN_POINT('Ctrl Pts',(-0.202236950697834,0.0026545294227545,
-0.00891122052825115));
#42265=CARTESIAN_POINT('Ctrl Pts',(-0.202225895790699,0.00266597494293841,
-0.00891112273377692));
#42266=CARTESIAN_POINT('Ctrl Pts',(-0.202205263183689,0.00269015250105854,
-0.00890642122194838));
#42267=CARTESIAN_POINT('Ctrl Pts',(-0.2021965521082,0.00270206949852077,
-0.00890169128285083));
#42268=CARTESIAN_POINT('Ctrl Pts',(-0.202186302463196,0.00271945585024983,
-0.00889073024673815));
#42269=CARTESIAN_POINT('Ctrl Pts',(-0.20218315201515,0.0027258921553306,
-0.00888560973687531));
#42270=CARTESIAN_POINT('Ctrl Pts',(-0.202179387654478,0.0027367989427911,
-0.00887434605633525));
#42271=CARTESIAN_POINT('Ctrl Pts',(-0.202178493553465,0.00274129479059584,
-0.00886862285140853));
#42272=CARTESIAN_POINT('Ctrl Pts',(-0.202178520809953,0.00274517218894165,
-0.00886238122749359));
#42273=CARTESIAN_POINT('Ctrl Pts',(-0.201155090292175,0.0128339461321558,
-0.00858641773309735));
#42274=CARTESIAN_POINT('Ctrl Pts',(-0.201260979997059,0.0128276733596081,
-0.008601020897081));
#42275=CARTESIAN_POINT('Ctrl Pts',(-0.201261993178973,0.0127668493824425,
-0.00851290802901172));
#42276=CARTESIAN_POINT('Ctrl Pts',(-0.201015035208462,0.011987649430818,
-0.00917044849004206));
#42277=CARTESIAN_POINT('Ctrl Pts',(-0.201120561593533,0.0119769211070483,
-0.00918585984469463));
#42278=CARTESIAN_POINT('Ctrl Pts',(-0.201121824479614,0.0119256299247488,
-0.00909110167463794));
#42279=CARTESIAN_POINT('Ctrl Pts',(-0.200741069345388,0.0100927310436652,
-0.0100583529007995));
#42280=CARTESIAN_POINT('Ctrl Pts',(-0.200848651520605,0.0100954146705308,
-0.0100640154274109));
#42281=CARTESIAN_POINT('Ctrl Pts',(-0.20085032774782,0.0100659660403532,
-0.00995911849787239));
#42282=CARTESIAN_POINT('Ctrl Pts',(-0.200951730607667,0.0080022228618309,
-0.0102933609042937));
#42283=CARTESIAN_POINT('Ctrl Pts',(-0.201057860798874,0.00801312022949754,
-0.0103020134424343));
#42284=CARTESIAN_POINT('Ctrl Pts',(-0.201059637391599,0.00800721062667035,
-0.0101944359329035));
#42285=CARTESIAN_POINT('Ctrl Pts',(-0.201035042743625,0.00696923703703989,
-0.0102357723537515));
#42286=CARTESIAN_POINT('Ctrl Pts',(-0.201141399474779,0.00697741160227575,
-0.0102453287437788));
#42287=CARTESIAN_POINT('Ctrl Pts',(-0.201143158232884,0.00698347932538022,
-0.0101384386393281));
#42288=CARTESIAN_POINT('Ctrl Pts',(-0.201099840401704,0.00750066861474714,
-0.0101529052072166));
#42289=CARTESIAN_POINT('Ctrl Pts',(-0.201099677169239,0.00750066912054103,
-0.0101593582616468));
#42290=CARTESIAN_POINT('Ctrl Pts',(-0.201098887242449,0.00750066989291298,
-0.0101657801072424));
#42291=CARTESIAN_POINT('Ctrl Pts',(-0.201095966520023,0.00750067202929758,
-0.0101788743168739));
#42292=CARTESIAN_POINT('Ctrl Pts',(-0.20109374392092,0.0075006734288361,
-0.0101854901135771));
#42293=CARTESIAN_POINT('Ctrl Pts',(-0.201085497549442,0.0075006781819555,
-0.010203536733078));
#42294=CARTESIAN_POINT('Ctrl Pts',(-0.201077927130068,0.00750068213977413,
-0.0102141051489183));
#42295=CARTESIAN_POINT('Ctrl Pts',(-0.201059194678892,0.00750069135896144,
-0.0102317998180977));
#42296=CARTESIAN_POINT('Ctrl Pts',(-0.201048206402947,0.00750069653436368,
-0.010238759491104));
#42297=CARTESIAN_POINT('Ctrl Pts',(-0.201021557960836,0.00750070864767776,
-0.0102491862051309));
#42298=CARTESIAN_POINT('Ctrl Pts',(-0.201008029147252,0.00750070956203601,
-0.0102505221971764));
#42299=CARTESIAN_POINT('Ctrl Pts',(-0.20099770582662,0.00750071937682855,
-0.0102503571197901));
#42300=CARTESIAN_POINT('Ctrl Pts',(-0.200997257667548,0.00750071911133179,
-0.0102503477931785));
#42301=CARTESIAN_POINT('Origin',(-0.201017212115499,0.00265911537344352,
-0.00878606880213356));
#42302=CARTESIAN_POINT('Ctrl Pts',(-0.201177754620579,0.0027448415119716,
-0.00884107761226325));
#42303=CARTESIAN_POINT('Ctrl Pts',(-0.201177628042387,0.00274082641373192,
-0.00884771612051796));
#42304=CARTESIAN_POINT('Ctrl Pts',(-0.201176712286097,0.00273609158279732,
-0.008853782822355));
#42305=CARTESIAN_POINT('Ctrl Pts',(-0.201173250003288,0.00272485674829661,
-0.00886520275453687));
#42306=CARTESIAN_POINT('Ctrl Pts',(-0.201170577213625,0.00271835999346171,
-0.00887025880407389));
#42307=CARTESIAN_POINT('Ctrl Pts',(-0.201161962995019,0.00270066932355189,
-0.00888092912017631));
#42308=CARTESIAN_POINT('Ctrl Pts',(-0.201154864234623,0.00268863669597218,
-0.00888531233553696));
#42309=CARTESIAN_POINT('Ctrl Pts',(-0.20113811014608,0.00266397446442915,
-0.00888917124572946));
#42310=CARTESIAN_POINT('Ctrl Pts',(-0.201129051225016,0.00265208658043163,
-0.0088887448390463));
#42311=CARTESIAN_POINT('Ctrl Pts',(-0.201106193044083,0.00262469960299615,
-0.0088831853591339));
#42312=CARTESIAN_POINT('Ctrl Pts',(-0.201095158723894,0.00261358759693136,
-0.00887674001446222));
#42313=CARTESIAN_POINT('Ctrl Pts',(-0.20109109045133,0.00260980814508552,
-0.00887454309705644));
#42314=CARTESIAN_POINT('Ctrl Pts',(-0.201090343739424,0.00260894149648861,
-0.00887402415850547));
#42315=CARTESIAN_POINT('Ctrl Pts',(-0.20108934207694,0.00260778484674993,
-0.00887332012892615));
#42316=CARTESIAN_POINT('Ctrl Pts',(-0.201088523107266,0.00260698192588514,
-0.0088728124292417));
#42317=CARTESIAN_POINT('Ctrl Pts',(-0.201258741752539,0.00223790006051546,
-0.00851599811712773));
#42318=CARTESIAN_POINT('Ctrl Pts',(-0.201257833511546,0.00217713357105664,
-0.00860416818402206));
#42319=CARTESIAN_POINT('Ctrl Pts',(-0.201151914418942,0.00217085125914763,
-0.00858968164457007));
#42320=CARTESIAN_POINT('Ctrl Pts',(-0.201119551825336,0.0030788662053447,
-0.0090932840728631));
#42321=CARTESIAN_POINT('Ctrl Pts',(-0.201118393839695,0.00302763434948745,
-0.00918808984717891));
#42322=CARTESIAN_POINT('Ctrl Pts',(-0.201012835888744,0.00301693193686283,
-0.00917280217687647));
#42323=CARTESIAN_POINT('Ctrl Pts',(-0.200848681291751,0.00493768758826015,
-0.00995971868738787));
#42324=CARTESIAN_POINT('Ctrl Pts',(-0.200847112869582,0.00490827835577488,
-0.0100646364930119));
#42325=CARTESIAN_POINT('Ctrl Pts',(-0.200739509642514,0.00491089619573715,
-0.010059053811372));
#42326=CARTESIAN_POINT('Ctrl Pts',(-0.20105915724458,0.0069945413110089,
-0.0101943176570579));
#42327=CARTESIAN_POINT('Ctrl Pts',(-0.201057487566078,0.006988641463598,
-0.0103019102012954));
#42328=CARTESIAN_POINT('Ctrl Pts',(-0.200951344751406,0.00699964817927347,
-0.0102933594943047));
#42329=CARTESIAN_POINT('Ctrl Pts',(-0.201143595912237,0.00801742258598695,
-0.0101382994581758));
#42330=CARTESIAN_POINT('Ctrl Pts',(-0.201141944150171,0.00802349301337347,
-0.0102452048937045));
#42331=CARTESIAN_POINT('Ctrl Pts',(-0.20103557348225,0.00803175898212767,
-0.0102357331328223));
#42332=CARTESIAN_POINT('Ctrl Pts',(-0.200264188629852,0.0127861801628926,
-0.00848016633972643));
#42333=CARTESIAN_POINT('Ctrl Pts',(-0.200261797905388,0.0128446548055681,
-0.00856471227770291));
#42334=CARTESIAN_POINT('Ctrl Pts',(-0.200363805385546,0.0128338532231718,
-0.00857173926582449));
#42335=CARTESIAN_POINT('Ctrl Pts',(-0.200125964276301,0.0119528335885076,
-0.00905604844208056));
#42336=CARTESIAN_POINT('Ctrl Pts',(-0.200123325889639,0.0120022189944504,
-0.00914693499322317));
#42337=CARTESIAN_POINT('Ctrl Pts',(-0.200224987570178,0.0119877937173126,
-0.00915425753864673));
#42338=CARTESIAN_POINT('Ctrl Pts',(-0.19984820163058,0.0100686222287371,
-0.00994082914119559));
#42339=CARTESIAN_POINT('Ctrl Pts',(-0.199845199470471,0.0100968901927037,
-0.0100415764810079));
#42340=CARTESIAN_POINT('Ctrl Pts',(-0.199948841017887,0.0100970427571912,
-0.0100388081310723));
#42341=CARTESIAN_POINT('Ctrl Pts',(-0.200061564759937,0.00799550694355067,
-0.0101718836147545));
#42342=CARTESIAN_POINT('Ctrl Pts',(-0.200058435840963,0.00800112432784995,
-0.0102751496995788));
#42343=CARTESIAN_POINT('Ctrl Pts',(-0.200160719650638,0.00801122946222692,
-0.0102749241092734));
#42344=CARTESIAN_POINT('Ctrl Pts',(-0.200144097286729,0.00697707856075904,
-0.0101153254435978));
#42345=CARTESIAN_POINT('Ctrl Pts',(-0.200140992571978,0.00697124582500046,
-0.0102179431873745));
#42346=CARTESIAN_POINT('Ctrl Pts',(-0.200243500976602,0.00697954697503826,
-0.0102186691874395));
#42347=CARTESIAN_POINT('Ctrl Pts',(-0.200100331002871,0.00750107109769107,
-0.0101300470129157));
#42348=CARTESIAN_POINT('Ctrl Pts',(-0.200100183117646,0.00750107182035176,
-0.0101365905644933));
#42349=CARTESIAN_POINT('Ctrl Pts',(-0.200100680353927,0.00750107222471504,
-0.0101431324573533));
#42350=CARTESIAN_POINT('Ctrl Pts',(-0.200103022217917,0.00750107239064495,
-0.010156433809306));
#42351=CARTESIAN_POINT('Ctrl Pts',(-0.200104943812047,0.00750107210931998,
-0.0101631434994043));
#42352=CARTESIAN_POINT('Ctrl Pts',(-0.200112366866152,0.00750107027570379,
-0.0101815444323523));
#42353=CARTESIAN_POINT('Ctrl Pts',(-0.200119452311889,0.00750106786353869,
-0.0101924440069437));
#42354=CARTESIAN_POINT('Ctrl Pts',(-0.200137366599506,0.00750106086311714,
-0.0102109666628549));
#42355=CARTESIAN_POINT('Ctrl Pts',(-0.200148029378955,0.00750105633974303,
-0.0102184154983561));
#42356=CARTESIAN_POINT('Ctrl Pts',(-0.200175341152975,0.007501044049354,
-0.0102305511306864));
#42357=CARTESIAN_POINT('Ctrl Pts',(-0.200189126148084,0.00750104583392516,
-0.010232025111573));
#42358=CARTESIAN_POINT('Ctrl Pts',(-0.200197937876526,0.0075010321737249,
-0.0102322815350947));
#42359=CARTESIAN_POINT('Ctrl Pts',(-0.200198408070096,0.00750103283571237,
-0.0102322930866153));
#42360=CARTESIAN_POINT('Ctrl Pts',(-0.200180145804599,0.0122615403574039,
-0.00881880956225188));
#42361=CARTESIAN_POINT('Ctrl Pts',(-0.200180119422939,0.0122654310898583,
-0.00882509212040225));
#42362=CARTESIAN_POINT('Ctrl Pts',(-0.200181024695127,0.012269947624273,
-0.00883085076702477));
#42363=CARTESIAN_POINT('Ctrl Pts',(-0.200184833727551,0.012280916013167,
-0.00884218362675862));
#42364=CARTESIAN_POINT('Ctrl Pts',(-0.200188022040074,0.0122873940992912,
-0.00884733112275432));
#42365=CARTESIAN_POINT('Ctrl Pts',(-0.200198364920575,0.0123048538863272,
-0.00885831053742095));
#42366=CARTESIAN_POINT('Ctrl Pts',(-0.200207132450346,0.0123168044121634,
-0.00886303220381333));
#42367=CARTESIAN_POINT('Ctrl Pts',(-0.200228410920646,0.0123416602759976,
-0.00886781500745342));
#42368=CARTESIAN_POINT('Ctrl Pts',(-0.200240168145585,0.0123537241143239,
-0.00886776943648934));
#42369=CARTESIAN_POINT('Ctrl Pts',(-0.200269920520539,0.0123814322404116,
-0.00886317053365818));
#42370=CARTESIAN_POINT('Ctrl Pts',(-0.20028454807678,0.0123927103831329,
-0.00885700343686482));
#42371=CARTESIAN_POINT('Ctrl Pts',(-0.200289515178599,0.0123962065901031,
-0.00885511747434229));
#42372=CARTESIAN_POINT('Ctrl Pts',(-0.200290340245052,0.0123969503360318,
-0.00885469577831727));
#42373=CARTESIAN_POINT('Ctrl Pts',(-0.200291447572802,0.0123979443029324,
-0.00885412567643322));
#42374=CARTESIAN_POINT('Ctrl Pts',(-0.200292341609995,0.0123986165584613,
-0.00885373182846497));
#42375=CARTESIAN_POINT('Origin',(-0.200343175462262,0.0123463747446592,
-0.0087694564592868));
#42376=CARTESIAN_POINT('Ctrl Pts',(-0.199179785887974,0.0122620277131703,
-0.00879745964969994));
#42377=CARTESIAN_POINT('Ctrl Pts',(-0.199179661572149,0.0122659741273922,
-0.0088040027320839));
#42378=CARTESIAN_POINT('Ctrl Pts',(-0.199178771661386,0.0122706202061008,
-0.00880999314679547));
#42379=CARTESIAN_POINT('Ctrl Pts',(-0.199175408875086,0.0122816306366328,
-0.00882128986615296));
#42380=CARTESIAN_POINT('Ctrl Pts',(-0.199172814695162,0.0122879926693539,
-0.00882631142860891));
#42381=CARTESIAN_POINT('Ctrl Pts',(-0.199164386859704,0.0123054469889948,
-0.0088370426202018));
#42382=CARTESIAN_POINT('Ctrl Pts',(-0.199157388756533,0.012317387084561,
-0.00884151841784895));
#42383=CARTESIAN_POINT('Ctrl Pts',(-0.199141079666825,0.0123415402785929,
-0.00884554723861314));
#42384=CARTESIAN_POINT('Ctrl Pts',(-0.19913241292987,0.0123530199318005,
-0.00884532702339733));
#42385=CARTESIAN_POINT('Ctrl Pts',(-0.199112251006035,0.0123774910375646,
-0.00884091757244983));
#42386=CARTESIAN_POINT('Ctrl Pts',(-0.199102544559066,0.0123877253055016,
-0.00883620109091419));
#42387=CARTESIAN_POINT('Ctrl Pts',(-0.19909563044449,0.0123949022594031,
-0.00883230825180998));
#42388=CARTESIAN_POINT('Ctrl Pts',(-0.199093476999217,0.0123970336359197,
-0.00883112407722527));
#42389=CARTESIAN_POINT('Ctrl Pts',(-0.199091315089946,0.0123991048910834,
-0.00882985186299045));
#42390=CARTESIAN_POINT('Ctrl Pts',(-0.199090551565165,0.0123998542387891,
-0.00882937949458529));
#42391=CARTESIAN_POINT('Ctrl Pts',(-0.200358957134347,0.00217086150225239,
-0.00857490676916749));
#42392=CARTESIAN_POINT('Ctrl Pts',(-0.200256928145031,0.00216031997502484,
-0.00856769265384055));
#42393=CARTESIAN_POINT('Ctrl Pts',(-0.200259634891842,0.00221877287151093,
-0.00848313450138094));
#42394=CARTESIAN_POINT('Ctrl Pts',(-0.200221663577824,0.0030168279086254,
-0.00915662824964644));
#42395=CARTESIAN_POINT('Ctrl Pts',(-0.200119977026507,0.00300268251391842,
-0.00914910188724964));
#42396=CARTESIAN_POINT('Ctrl Pts',(-0.200122930091165,0.0030520580293655,
-0.00905821337665723));
#42397=CARTESIAN_POINT('Ctrl Pts',(-0.199946837716981,0.00490697429828446,
-0.0100396594974494));
#42398=CARTESIAN_POINT('Ctrl Pts',(-0.199843194595014,0.0049071499232358,
-0.0100421011877827));
#42399=CARTESIAN_POINT('Ctrl Pts',(-0.199846517101214,0.00493537109414294,
-0.00994133786826413));
#42400=CARTESIAN_POINT('Ctrl Pts',(-0.200159811015846,0.00699125895088654,
-0.0102749556173087));
#42401=CARTESIAN_POINT('Ctrl Pts',(-0.200057531776169,0.00700151354044847,
-0.0102748800528092));
#42402=CARTESIAN_POINT('Ctrl Pts',(-0.200060976277344,0.00700707046734485,
-0.0101716158500798));
#42403=CARTESIAN_POINT('Ctrl Pts',(-0.2002437246959,0.0080221462246762,
-0.0102185853555578));
#42404=CARTESIAN_POINT('Ctrl Pts',(-0.200141219699188,0.00803052476732281,
-0.0102175393390583));
#42405=CARTESIAN_POINT('Ctrl Pts',(-0.200144640779559,0.00802464727946508,
-0.0101149279193058));
#42406=CARTESIAN_POINT('Ctrl Pts',(-0.200288491918007,0.00260606732410401,
-0.00885652097176724));
#42407=CARTESIAN_POINT('Ctrl Pts',(-0.200287495201655,0.00260681778558282,
-0.0088569600240947));
#42408=CARTESIAN_POINT('Ctrl Pts',(-0.200284717053799,0.00260886972400836,
-0.00885812502365241));
#42409=CARTESIAN_POINT('Ctrl Pts',(-0.200281945029545,0.00261098644985002,
-0.00885920566089888));
#42410=CARTESIAN_POINT('Ctrl Pts',(-0.200272773111516,0.0026182905132756,
-0.00886285415940844));
#42411=CARTESIAN_POINT('Ctrl Pts',(-0.200260149063117,0.00262859824983106,
-0.00886708771969354));
#42412=CARTESIAN_POINT('Ctrl Pts',(-0.200234736915584,0.00265262420116412,
-0.00887052425754006));
#42413=CARTESIAN_POINT('Ctrl Pts',(-0.200223688245904,0.00266407875563347,
-0.00887039745452822));
#42414=CARTESIAN_POINT('Ctrl Pts',(-0.200203089431465,0.0026882458772359,
-0.00886562944497509));
#42415=CARTESIAN_POINT('Ctrl Pts',(-0.200194400332019,0.00270014366015399,
-0.00886087059012383));
#42416=CARTESIAN_POINT('Ctrl Pts',(-0.200184181192038,0.0027174899119063,
-0.00884987271924794));
#42417=CARTESIAN_POINT('Ctrl Pts',(-0.200181042299458,0.00272390595868316,
-0.00884474249216518));
#42418=CARTESIAN_POINT('Ctrl Pts',(-0.200177292150585,0.0027347729314724,
-0.00883346936644047));
#42419=CARTESIAN_POINT('Ctrl Pts',(-0.200176401505629,0.00273925043048663,
-0.00882774489291586));
#42420=CARTESIAN_POINT('Ctrl Pts',(-0.200176428288968,0.00274311030530121,
-0.00882150516518164));
#42421=CARTESIAN_POINT('Ctrl Pts',(-0.199153925914828,0.0128366821545121,
-0.00854669799338706));
#42422=CARTESIAN_POINT('Ctrl Pts',(-0.199259867331971,0.012830442499507,
-0.00856126082459914));
#42423=CARTESIAN_POINT('Ctrl Pts',(-0.199260848897657,0.0127697866181808,
-0.00847297835399615));
#42424=CARTESIAN_POINT('Ctrl Pts',(-0.199014566784101,0.0119891616218098,
-0.00912886879878308));
#42425=CARTESIAN_POINT('Ctrl Pts',(-0.199120147481746,0.0119784757991412,
-0.00914424112649619));
#42426=CARTESIAN_POINT('Ctrl Pts',(-0.199121380077652,0.0119273408354419,
-0.00904935391227361));
#42427=CARTESIAN_POINT('Ctrl Pts',(-0.198742265564451,0.0100930977349455,
-0.0100137054011551));
#42428=CARTESIAN_POINT('Ctrl Pts',(-0.198849884594932,0.0100958392977007,
-0.0100193912995539));
#42429=CARTESIAN_POINT('Ctrl Pts',(-0.198851531194117,0.0100664774230896,
-0.00991443863121942));
#42430=CARTESIAN_POINT('Ctrl Pts',(-0.198952781415296,0.00800322977916761,
-0.0102479430315782));
#42431=CARTESIAN_POINT('Ctrl Pts',(-0.199058955570973,0.00801411281887282,
-0.0102566155570904));
#42432=CARTESIAN_POINT('Ctrl Pts',(-0.199060703267466,0.00800821003159929,
-0.0101489980208889));
#42433=CARTESIAN_POINT('Ctrl Pts',(-0.19903599944403,0.00697025739231732,
-0.010190711247955));
#42434=CARTESIAN_POINT('Ctrl Pts',(-0.199142399146872,0.00697843276992515,
-0.0102002818600052));
#42435=CARTESIAN_POINT('Ctrl Pts',(-0.199144128826406,0.00698446519833132,
-0.0100933452087197));
#42436=CARTESIAN_POINT('Ctrl Pts',(-0.19910085411519,0.00750164267895669,
-0.0101077379174169));
#42437=CARTESIAN_POINT('Ctrl Pts',(-0.199100690234321,0.00750164386369201,
-0.0101141870486527));
#42438=CARTESIAN_POINT('Ctrl Pts',(-0.199099900425191,0.00750164529645312,
-0.010120604956208));
#42439=CARTESIAN_POINT('Ctrl Pts',(-0.199096980593123,0.00750164874874024,
-0.0101336953338829));
#42440=CARTESIAN_POINT('Ctrl Pts',(-0.199094758035115,0.00750165079589565,
-0.0101403110956162));
#42441=CARTESIAN_POINT('Ctrl Pts',(-0.199086511791722,0.0075016572640334,
-0.010158357677076));
#42442=CARTESIAN_POINT('Ctrl Pts',(-0.19907894146395,0.00750166216143604,
-0.0101689261079603));
#42443=CARTESIAN_POINT('Ctrl Pts',(-0.199060209203537,0.00750167281253752,
-0.0101866208178074));
#42444=CARTESIAN_POINT('Ctrl Pts',(-0.199049221031088,0.0075016784662638,
-0.0101935805231524));
#42445=CARTESIAN_POINT('Ctrl Pts',(-0.199020116024875,0.00750169222744614,
-0.0102049685859948));
#42446=CARTESIAN_POINT('Ctrl Pts',(-0.199005661662064,0.00750168698491313,
-0.010205289239491));
#42447=CARTESIAN_POINT('Ctrl Pts',(-0.198998826136759,0.00750170224290608,
-0.0102051799706931));
#42448=CARTESIAN_POINT('Ctrl Pts',(-0.198998273076492,0.00750170106245327,
-0.0102051689708856));
#42449=CARTESIAN_POINT('Origin',(-0.199015196624372,0.00265663137285891,
-0.00874521521192296));
#42450=CARTESIAN_POINT('Ctrl Pts',(-0.199174969366088,0.0027425015311611,
-0.00880006183795226));
#42451=CARTESIAN_POINT('Ctrl Pts',(-0.199174842813697,0.00273849810823364,
-0.00880671010323751));
#42452=CARTESIAN_POINT('Ctrl Pts',(-0.199173925414073,0.0027337733786718,
-0.00881278723753809));
#42453=CARTESIAN_POINT('Ctrl Pts',(-0.199170456542776,0.00272255592635832,
-0.00882423111370532));
#42454=CARTESIAN_POINT('Ctrl Pts',(-0.199167778418797,0.00271606601452812,
-0.00882929991919414));
#42455=CARTESIAN_POINT('Ctrl Pts',(-0.199159149072896,0.00269839144076132,
-0.00884000172480209));
#42456=CARTESIAN_POINT('Ctrl Pts',(-0.199152038592254,0.0026863648561937,
-0.00884440574954461));
#42457=CARTESIAN_POINT('Ctrl Pts',(-0.199135085380916,0.00266145267956537,
-0.00884834654768667));
#42458=CARTESIAN_POINT('Ctrl Pts',(-0.199125804136305,0.00264931689278553,
-0.00884788255368404));
#42459=CARTESIAN_POINT('Ctrl Pts',(-0.19910220100882,0.00262117554154459,
-0.00884201033625836));
#42460=CARTESIAN_POINT('Ctrl Pts',(-0.199090880396505,0.00260977142339133,
-0.00883512294598114));
#42461=CARTESIAN_POINT('Ctrl Pts',(-0.199087183615344,0.00260668440517497,
-0.00883328156483494));
#42462=CARTESIAN_POINT('Ctrl Pts',(-0.199086747113234,0.00260606094030435,
-0.00883290238784639));
#42463=CARTESIAN_POINT('Ctrl Pts',(-0.199086158459772,0.00260522462644416,
-0.00883239115011147));
#42464=CARTESIAN_POINT('Ctrl Pts',(-0.199085607015723,0.00260468401114808,
-0.00883205078672203));
#42465=CARTESIAN_POINT('Ctrl Pts',(-0.199255095029157,0.00223457912828636,
-0.00847572645168213));
#42466=CARTESIAN_POINT('Ctrl Pts',(-0.199254232558087,0.00217396135577984,
-0.00856408799862321));
#42467=CARTESIAN_POINT('Ctrl Pts',(-0.199148223548041,0.00216779022884886,
-0.00854967377101157));
#42468=CARTESIAN_POINT('Ctrl Pts',(-0.19911735452896,0.00307715138405225,
-0.00905153587025602));
#42469=CARTESIAN_POINT('Ctrl Pts',(-0.199116240561307,0.00302606428734341,
-0.00914649828133776));
#42470=CARTESIAN_POINT('Ctrl Pts',(-0.199010586552336,0.00301548895708846,
-0.00913127651739455));
#42471=CARTESIAN_POINT('Ctrl Pts',(-0.198849911128423,0.00493808762162639,
-0.00991542469109674));
#42472=CARTESIAN_POINT('Ctrl Pts',(-0.198848386136249,0.00490876839268646,
-0.0100204318585757));
#42473=CARTESIAN_POINT('Ctrl Pts',(-0.198740725122237,0.00491151346327143,
-0.010014816198803));
#42474=CARTESIAN_POINT('Ctrl Pts',(-0.199060248816942,0.00699530919792622,
-0.0101490071671049));
#42475=CARTESIAN_POINT('Ctrl Pts',(-0.19905862191434,0.00698943349787215,
-0.0102566707772468));
#42476=CARTESIAN_POINT('Ctrl Pts',(-0.19895240571383,0.00700041025111481,
-0.0102480788233023));
#42477=CARTESIAN_POINT('Ctrl Pts',(-0.199144551422616,0.00801857716988301,
-0.0100930718875589));
#42478=CARTESIAN_POINT('Ctrl Pts',(-0.19914294272733,0.00802463741471564,
-0.0102000519321202));
#42479=CARTESIAN_POINT('Ctrl Pts',(-0.19903650115962,0.00803290185070517,
-0.0101905476764064));
#42480=CARTESIAN_POINT('Ctrl Pts',(-0.198263029449118,0.0127889692553363,
-0.00844048161250917));
#42481=CARTESIAN_POINT('Ctrl Pts',(-0.198260630058131,0.0128473039681307,
-0.00852521985761382));
#42482=CARTESIAN_POINT('Ctrl Pts',(-0.198362723942519,0.0128364944620873,
-0.00853213005721722));
#42483=CARTESIAN_POINT('Ctrl Pts',(-0.198125476177104,0.0119543980606105,
-0.00901449391313416));
#42484=CARTESIAN_POINT('Ctrl Pts',(-0.198122828059934,0.0120036536706846,
-0.00910553515936531));
#42485=CARTESIAN_POINT('Ctrl Pts',(-0.198224578879579,0.011989235059393,
-0.00911273974707262));
#42486=CARTESIAN_POINT('Ctrl Pts',(-0.197849387608806,0.01006903040502,
-0.00989615586142495));
#42487=CARTESIAN_POINT('Ctrl Pts',(-0.197846373450675,0.0100972224232102,
-0.00999699320190778));
#42488=CARTESIAN_POINT('Ctrl Pts',(-0.197950089640886,0.0100974185995862,
-0.00999415824051916));
#42489=CARTESIAN_POINT('Ctrl Pts',(-0.198062621662617,0.00799661069352205,
-0.010126450478369));
#42490=CARTESIAN_POINT('Ctrl Pts',(-0.198059480886231,0.00800222051560605,
-0.0102297912470711));
#42491=CARTESIAN_POINT('Ctrl Pts',(-0.198161844756368,0.00801231207768851,
-0.0102294986091472));
#42492=CARTESIAN_POINT('Ctrl Pts',(-0.198145073126219,0.00697819839513995,
-0.0100702620522896));
#42493=CARTESIAN_POINT('Ctrl Pts',(-0.198141956591681,0.00697239573675233,
-0.0101729602259579));
#42494=CARTESIAN_POINT('Ctrl Pts',(-0.198244544135673,0.00698070459421834,
-0.0101736135490439));
#42495=CARTESIAN_POINT('Ctrl Pts',(-0.198101345636185,0.00750214469193914,
-0.0100848681354076));
#42496=CARTESIAN_POINT('Ctrl Pts',(-0.198101197751573,0.00750214617774456,
-0.0100914116445182));
#42497=CARTESIAN_POINT('Ctrl Pts',(-0.19810169497294,0.00750214739593405,
-0.0100979534963226));
#42498=CARTESIAN_POINT('Ctrl Pts',(-0.198104036775493,0.00750214932141574,
-0.0101112547620612));
#42499=CARTESIAN_POINT('Ctrl Pts',(-0.198105958320376,0.00750214998598784,
-0.0101179644113016));
#42500=CARTESIAN_POINT('Ctrl Pts',(-0.198113381212346,0.00750215091575145,
-0.0101363652889876));
#42501=CARTESIAN_POINT('Ctrl Pts',(-0.198120466534415,0.00750215035194178,
-0.0101472648747458));
#42502=CARTESIAN_POINT('Ctrl Pts',(-0.198138380559241,0.00750214695175643,
-0.010165787562833));
#42503=CARTESIAN_POINT('Ctrl Pts',(-0.198149043192216,0.00750214414783725,
-0.0101732364295918));
#42504=CARTESIAN_POINT('Ctrl Pts',(-0.198172674415732,0.00750213659454397,
-0.010183736844365));
#42505=CARTESIAN_POINT('Ctrl Pts',(-0.198185801028644,0.00750218604830201,
-0.0101867199827473));
#42506=CARTESIAN_POINT('Ctrl Pts',(-0.198198986950856,0.00750212258616043,
-0.0101871036401355));
#42507=CARTESIAN_POINT('Ctrl Pts',(-0.198199421593232,0.00750212627687263,
-0.0101871141587648));
#42508=CARTESIAN_POINT('Ctrl Pts',(-0.198179421976457,0.0122637107296257,
-0.00877800506024049));
#42509=CARTESIAN_POINT('Ctrl Pts',(-0.198179396344291,0.0122675886867059,
-0.00878429351810534));
#42510=CARTESIAN_POINT('Ctrl Pts',(-0.198180301295335,0.0122720932380238,
-0.00879005955512643));
#42511=CARTESIAN_POINT('Ctrl Pts',(-0.198184108465672,0.0122830396599457,
-0.0088014133230424));
#42512=CARTESIAN_POINT('Ctrl Pts',(-0.198187295703864,0.01228950904073,
-0.00880657398770549));
#42513=CARTESIAN_POINT('Ctrl Pts',(-0.198197634790808,0.0123069503878714,
-0.0088175872800557));
#42514=CARTESIAN_POINT('Ctrl Pts',(-0.198206398292014,0.012318892994339,
-0.00882233127930981));
#42515=CARTESIAN_POINT('Ctrl Pts',(-0.19822773024133,0.012343816486207,
-0.00882717428033988));
#42516=CARTESIAN_POINT('Ctrl Pts',(-0.198239560095189,0.0123559532208523,
-0.00882713596148907));
#42517=CARTESIAN_POINT('Ctrl Pts',(-0.198269575746573,0.0123838978710278,
-0.00882248937213228));
#42518=CARTESIAN_POINT('Ctrl Pts',(-0.19828431706727,0.0123952751703846,
-0.00881620251558207));
#42519=CARTESIAN_POINT('Ctrl Pts',(-0.198289094376121,0.0123985489069097,
-0.00881443224052086));
#42520=CARTESIAN_POINT('Ctrl Pts',(-0.198289802981431,0.0123992211180763,
-0.00881404902421685));
#42521=CARTESIAN_POINT('Ctrl Pts',(-0.198290754893029,0.0124001206399054,
-0.00881353216580912));
#42522=CARTESIAN_POINT('Ctrl Pts',(-0.198291543142929,0.0124007144452265,
-0.00881318583917323));
#42523=CARTESIAN_POINT('Origin',(-0.198342362989776,0.0123486420924163,
-0.00872880441193628));
#42524=CARTESIAN_POINT('Ctrl Pts',(-0.197178980255201,0.0122642101438025,
-0.00875668392088435));
#42525=CARTESIAN_POINT('Ctrl Pts',(-0.197178856018515,0.0122681440730026,
-0.00876323575792611));
#42526=CARTESIAN_POINT('Ctrl Pts',(-0.197177965413713,0.0122727788823566,
-0.00876923608914849));
#42527=CARTESIAN_POINT('Ctrl Pts',(-0.19717459969814,0.0122837685448601,
-0.00878055600760033));
#42528=CARTESIAN_POINT('Ctrl Pts',(-0.197172003114716,0.0122901215768531,
-0.00878559056959148));
#42529=CARTESIAN_POINT('Ctrl Pts',(-0.197163568261289,0.0123075555926102,
-0.00879635605420354));
#42530=CARTESIAN_POINT('Ctrl Pts',(-0.197156564638062,0.0123194869785333,
-0.00880085511127768));
#42531=CARTESIAN_POINT('Ctrl Pts',(-0.197140243569857,0.0123436310953871,
-0.00880493069090822));
#42532=CARTESIAN_POINT('Ctrl Pts',(-0.197131571370146,0.0123551095223622,
-0.00880473298623716));
#42533=CARTESIAN_POINT('Ctrl Pts',(-0.197111374713174,0.0123796129489924,
-0.00880036789297042));
#42534=CARTESIAN_POINT('Ctrl Pts',(-0.197101653461885,0.0123898598822889,
-0.0087956602818417));
#42535=CARTESIAN_POINT('Ctrl Pts',(-0.197094772849081,0.0123970061969382,
-0.00879180261198509));
#42536=CARTESIAN_POINT('Ctrl Pts',(-0.197092611619732,0.0123991456177334,
-0.00879062001464486));
#42537=CARTESIAN_POINT('Ctrl Pts',(-0.197090441888492,0.0124012245213655,
-0.00878934849827443));
#42538=CARTESIAN_POINT('Ctrl Pts',(-0.197089683999265,0.0124019687088208,
-0.00878888148062584));
#42539=CARTESIAN_POINT('Ctrl Pts',(-0.198355740632463,0.00216798230497538,
-0.00853508005087582));
#42540=CARTESIAN_POINT('Ctrl Pts',(-0.198253891209442,0.00215756142816948,
-0.00852801123984347));
#42541=CARTESIAN_POINT('Ctrl Pts',(-0.198256371022465,0.00221569792273099,
-0.0084434712164535));
#42542=CARTESIAN_POINT('Ctrl Pts',(-0.198220012716574,0.00301557344026443,
-0.00911524185554709));
#42543=CARTESIAN_POINT('Ctrl Pts',(-0.198118497826422,0.00300159238337313,
-0.00910786031377932));
#42544=CARTESIAN_POINT('Ctrl Pts',(-0.198121225337493,0.00305067205412701,
-0.0090170397869099));
#42545=CARTESIAN_POINT('Ctrl Pts',(-0.197948601255717,0.00490772806496031,
-0.00999548097376579));
#42546=CARTESIAN_POINT('Ctrl Pts',(-0.19784517320138,0.00490797639378848,
-0.00999792585786736));
#42547=CARTESIAN_POINT('Ctrl Pts',(-0.197848267709436,0.00493603470329018,
-0.0098973401747785));
#42548=CARTESIAN_POINT('Ctrl Pts',(-0.198160921855801,0.00699217420993246,
-0.0102296850629028));
#42549=CARTESIAN_POINT('Ctrl Pts',(-0.198058837601862,0.0070023676241383,
-0.0102296245765728));
#42550=CARTESIAN_POINT('Ctrl Pts',(-0.198062056014678,0.00700790340885586,
-0.0101265584017485));
#42551=CARTESIAN_POINT('Ctrl Pts',(-0.198244664059479,0.00802338361730227,
-0.0101733946164067));
#42552=CARTESIAN_POINT('Ctrl Pts',(-0.198142357495407,0.00803173061364109,
-0.0101723737755292));
#42553=CARTESIAN_POINT('Ctrl Pts',(-0.198145551970183,0.0080258913884697,
-0.0100699536208949));
#42554=CARTESIAN_POINT('Ctrl Pts',(-0.198286052317126,0.00260395641848403,
-0.00881592224463899));
#42555=CARTESIAN_POINT('Ctrl Pts',(-0.198285052106862,0.002604711795387,
-0.00881636221563572));
#42556=CARTESIAN_POINT('Ctrl Pts',(-0.198282283015153,0.00260676363711584,
-0.00881752172403233));
#42557=CARTESIAN_POINT('Ctrl Pts',(-0.198279520069941,0.00260887968698758,
-0.0088185971915071));
#42558=CARTESIAN_POINT('Ctrl Pts',(-0.198270298464757,0.00261624321829764,
-0.00882225771182116));
#42559=CARTESIAN_POINT('Ctrl Pts',(-0.198257641167467,0.00262660986385978,
-0.00882648360551525));
#42560=CARTESIAN_POINT('Ctrl Pts',(-0.198232181686762,0.0026507514027741,
-0.00882985566173298));
#42561=CARTESIAN_POINT('Ctrl Pts',(-0.198221111224353,0.00266226369413246,
-0.00882968370958079));
#42562=CARTESIAN_POINT('Ctrl Pts',(-0.198200572555613,0.00268644702176355,
-0.00882479161107287));
#42563=CARTESIAN_POINT('Ctrl Pts',(-0.198191945617939,0.00269830091297626,
-0.00881998918431501));
#42564=CARTESIAN_POINT('Ctrl Pts',(-0.198181821514597,0.0027155505425809,
-0.00880895292975098));
#42565=CARTESIAN_POINT('Ctrl Pts',(-0.198178719887895,0.00272191486951209,
-0.00880382552404368));
#42566=CARTESIAN_POINT('Ctrl Pts',(-0.198175014888067,0.00273269000209349,
-0.0087925808302122));
#42567=CARTESIAN_POINT('Ctrl Pts',(-0.198174135307401,0.00273712881468879,
-0.00878687650525372));
#42568=CARTESIAN_POINT('Ctrl Pts',(-0.198174161532551,0.00274095524349409,
-0.00878066434858561));
#42569=CARTESIAN_POINT('Ctrl Pts',(-0.197152676116489,0.0128393614504822,
-0.00850713805088089));
#42570=CARTESIAN_POINT('Ctrl Pts',(-0.197258675429355,0.0128331580754525,
-0.00852166540087489));
#42571=CARTESIAN_POINT('Ctrl Pts',(-0.197259624390767,0.0127726713284735,
-0.00843320519526083));
#42572=CARTESIAN_POINT('Ctrl Pts',(-0.197014015809443,0.0119906110226541,
-0.0090873939546814));
#42573=CARTESIAN_POINT('Ctrl Pts',(-0.19711965698234,0.0119799690509704,
-0.00910273277093066));
#42574=CARTESIAN_POINT('Ctrl Pts',(-0.197120858311449,0.0119289913696173,
-0.00900770887161405));
#42575=CARTESIAN_POINT('Ctrl Pts',(-0.1967434320964,0.010093409573426,-0.0099690764507125));
#42576=CARTESIAN_POINT('Ctrl Pts',(-0.196851094172184,0.0100962166426703,
-0.00997479026530362));
#42577=CARTESIAN_POINT('Ctrl Pts',(-0.196852710184559,0.010066942105563,
-0.00986977505718237));
#42578=CARTESIAN_POINT('Ctrl Pts',(-0.196953826442827,0.00800423429314859,
-0.0102025203427104));
#42579=CARTESIAN_POINT('Ctrl Pts',(-0.197060050666728,0.00801510290894852,
-0.0102112192925465));
#42580=CARTESIAN_POINT('Ctrl Pts',(-0.197061768527618,0.00800920700147784,
-0.0101035551134565));
#42581=CARTESIAN_POINT('Ctrl Pts',(-0.197036943426159,0.00697129173689632,
-0.0101456507615118));
#42582=CARTESIAN_POINT('Ctrl Pts',(-0.19714339221939,0.00697946845198856,
-0.0101552416408534));
#42583=CARTESIAN_POINT('Ctrl Pts',(-0.197145091880529,0.00698546537262034,
-0.0100482517868171));
#42584=CARTESIAN_POINT('Ctrl Pts',(-0.197101862194412,0.00750262265417027,
-0.0100625703142549));
#42585=CARTESIAN_POINT('Ctrl Pts',(-0.197101697671371,0.00750262451484505,
-0.0100690155262311));
#42586=CARTESIAN_POINT('Ctrl Pts',(-0.197100907987531,0.00750262657291193,
-0.0100754295007868));
#42587=CARTESIAN_POINT('Ctrl Pts',(-0.197097989070983,0.00750263120389314,
-0.0100885160265501));
#42588=CARTESIAN_POINT('Ctrl Pts',(-0.197095766578603,0.00750263379167027,
-0.0100951317314081));
#42589=CARTESIAN_POINT('Ctrl Pts',(-0.197087520538495,0.00750264157329612,
-0.0101131782531217));
#42590=CARTESIAN_POINT('Ctrl Pts',(-0.197079950354737,0.00750264703705398,
-0.0101237467095286));
#42591=CARTESIAN_POINT('Ctrl Pts',(-0.197061218392508,0.00750265820233082,
-0.0101414414885696));
#42592=CARTESIAN_POINT('Ctrl Pts',(-0.197050230380519,0.00750266379358303,
-0.0101484012476249));
#42593=CARTESIAN_POINT('Ctrl Pts',(-0.197018045725239,0.00750267810501846,
-0.0101609946010674));
#42594=CARTESIAN_POINT('Ctrl Pts',(-0.197001295227288,0.00750267186841195,
-0.0101600242486746));
#42595=CARTESIAN_POINT('Ctrl Pts',(-0.196999724282808,0.00750269777634812,
-0.0101599991229918));
#42596=CARTESIAN_POINT('Ctrl Pts',(-0.196999282996544,0.00750268375780151,
-0.0101599899221715));
#42597=CARTESIAN_POINT('Origin',(-0.19701266044424,0.00265463512617686,
-0.0087047471371959));
#42598=CARTESIAN_POINT('Ctrl Pts',(-0.197176341115347,0.00274057713674786,
-0.00875946998943032));
#42599=CARTESIAN_POINT('Ctrl Pts',(-0.19717621449323,0.00273658033899075,
-0.00876613764532655));
#42600=CARTESIAN_POINT('Ctrl Pts',(-0.197175294731817,0.00273185885740524,
-0.00877223381232567));
#42601=CARTESIAN_POINT('Ctrl Pts',(-0.197171816455455,0.0027206414947534,
-0.0087837163247442));
#42602=CARTESIAN_POINT('Ctrl Pts',(-0.197169130834591,0.00271414787170457,
-0.0087888035389614));
#42603=CARTESIAN_POINT('Ctrl Pts',(-0.197160484426132,0.00269647084444689,
-0.0087995384357049));
#42604=CARTESIAN_POINT('Ctrl Pts',(-0.197153365839063,0.0026844444832896,
-0.00880395918817329));
#42605=CARTESIAN_POINT('Ctrl Pts',(-0.197136501486506,0.00265967921921435,
-0.00880790583160597));
#42606=CARTESIAN_POINT('Ctrl Pts',(-0.197127339136267,0.00264768562505251,
-0.0088074890418658));
#42607=CARTESIAN_POINT('Ctrl Pts',(-0.197104165460954,0.00261999057037431,
-0.00880186055873384));
#42608=CARTESIAN_POINT('Ctrl Pts',(-0.197093015487574,0.00260875339685481,
-0.00879526794355148));
#42609=CARTESIAN_POINT('Ctrl Pts',(-0.19708909427863,0.00260524930630241,
-0.00879321892863089));
#42610=CARTESIAN_POINT('Ctrl Pts',(-0.197088502629849,0.00260450913545116,
-0.00879277500053084));
#42611=CARTESIAN_POINT('Ctrl Pts',(-0.197087707786473,0.00260351927461845,
-0.00879217488636297));
#42612=CARTESIAN_POINT('Ctrl Pts',(-0.197087026280342,0.00260285013296824,
-0.00879175552978747));
#42613=CARTESIAN_POINT('Ctrl Pts',(-0.197256869972498,0.00223198241721985,
-0.00843619486098983));
#42614=CARTESIAN_POINT('Ctrl Pts',(-0.197256039653172,0.00217143518714522,
-0.00852488462310169));
#42615=CARTESIAN_POINT('Ctrl Pts',(-0.197149825227004,0.00216528939694016,
-0.00851026192212582));
#42616=CARTESIAN_POINT('Ctrl Pts',(-0.197118290041498,0.00307599018027203,
-0.00901018904184981));
#42617=CARTESIAN_POINT('Ctrl Pts',(-0.197117206671809,0.00302497917955987,
-0.00910545043129841));
#42618=CARTESIAN_POINT('Ctrl Pts',(-0.197011351483258,0.00301435832614128,
-0.00909000260578813));
#42619=CARTESIAN_POINT('Ctrl Pts',(-0.196850616071858,0.00493844615024685,
-0.00987108302336436));
#42620=CARTESIAN_POINT('Ctrl Pts',(-0.196849120143893,0.0049091727597524,
-0.00997633168506119));
#42621=CARTESIAN_POINT('Ctrl Pts',(-0.196741239182059,0.00491211626324586,
-0.00997054306786492));
#42622=CARTESIAN_POINT('Ctrl Pts',(-0.197061511162985,0.00699611927119618,
-0.0101037173049972));
#42623=CARTESIAN_POINT('Ctrl Pts',(-0.197059912250147,0.00699026221777102,
-0.0102116100519241));
#42624=CARTESIAN_POINT('Ctrl Pts',(-0.196953483034995,0.00700121689459126,
-0.010202788168383));
#42625=CARTESIAN_POINT('Ctrl Pts',(-0.19714541010813,0.00801971418708215,
-0.0100478527361994));
#42626=CARTESIAN_POINT('Ctrl Pts',(-0.197143829692753,0.00802577303021904,
-0.0101550639206471));
#42627=CARTESIAN_POINT('Ctrl Pts',(-0.19703717377299,0.00803402714762754,
-0.010145346940021));
#42628=CARTESIAN_POINT('Ctrl Pts',(-0.196261785015612,0.0127916962446281,
-0.00840096669647052));
#42629=CARTESIAN_POINT('Ctrl Pts',(-0.196259381274784,0.0128498400502766,
-0.00848583311340328));
#42630=CARTESIAN_POINT('Ctrl Pts',(-0.1963614813015,0.0128390750295401,
-0.00849268564311148));
#42631=CARTESIAN_POINT('Ctrl Pts',(-0.196124943532184,0.0119558621939739,
-0.00897306484675636));
#42632=CARTESIAN_POINT('Ctrl Pts',(-0.19612229019771,0.012004944437071,
-0.00906419088049844));
#42633=CARTESIAN_POINT('Ctrl Pts',(-0.196224049780035,0.0119905847978755,
-0.00907134057560896));
#42634=CARTESIAN_POINT('Ctrl Pts',(-0.195850337444749,0.0100694080936677,
-0.00985151727421576));
#42635=CARTESIAN_POINT('Ctrl Pts',(-0.195847316168474,0.0100974995137687,
-0.00995236546633424));
#42636=CARTESIAN_POINT('Ctrl Pts',(-0.195951025832399,0.0100977416688382,
-0.00994954663897551));
#42637=CARTESIAN_POINT('Ctrl Pts',(-0.196063688383263,0.00799749089638932,
-0.0100810227580311));
#42638=CARTESIAN_POINT('Ctrl Pts',(-0.196060540650448,0.00800308596337127,
-0.0101843566508062));
#42639=CARTESIAN_POINT('Ctrl Pts',(-0.196162901661524,0.0080131845991667,
-0.0101840741728357));
#42640=CARTESIAN_POINT('Ctrl Pts',(-0.196146246896505,0.00697929629222657,
-0.0100252005223376));
#42641=CARTESIAN_POINT('Ctrl Pts',(-0.19614312341995,0.00697352863131464,
-0.0101278980253559));
#42642=CARTESIAN_POINT('Ctrl Pts',(-0.196245707515403,0.00698184995272653,
-0.0101285582070294));
#42643=CARTESIAN_POINT('Ctrl Pts',(-0.196102466660209,0.00750312907896353,
-0.0100396915356686));
#42644=CARTESIAN_POINT('Ctrl Pts',(-0.196102318774524,0.00750313126710287,
-0.0100462350453267));
#42645=CARTESIAN_POINT('Ctrl Pts',(-0.196102815992879,0.00750313328765614,
-0.0100527768981209));
#42646=CARTESIAN_POINT('Ctrl Pts',(-0.196105157785642,0.00750313705085542,
-0.0100660781640112));
#42647=CARTESIAN_POINT('Ctrl Pts',(-0.196107079323156,0.00750313875719901,
-0.0100727878133388));
#42648=CARTESIAN_POINT('Ctrl Pts',(-0.196114502186249,0.00750314287748569,
-0.0100911886823653));
#42649=CARTESIAN_POINT('Ctrl Pts',(-0.196121587480966,0.00750314462020405,
-0.0101020882662016));
#42650=CARTESIAN_POINT('Ctrl Pts',(-0.196139501440965,0.00750314604761364,
-0.0101206109452192));
#42651=CARTESIAN_POINT('Ctrl Pts',(-0.196150164032413,0.00750314572377275,
-0.0101280598096453));
#42652=CARTESIAN_POINT('Ctrl Pts',(-0.196173794669146,0.00750314295768892,
-0.0101385599985622));
#42653=CARTESIAN_POINT('Ctrl Pts',(-0.196186921880472,0.00750331952577555,
-0.0101415431020705));
#42654=CARTESIAN_POINT('Ctrl Pts',(-0.196200104085276,0.00750312471114926,
-0.0101419269254443));
#42655=CARTESIAN_POINT('Ctrl Pts',(-0.196200541288955,0.00750313735745115,
-0.0101419375111811));
#42656=CARTESIAN_POINT('Ctrl Pts',(-0.196178618317942,0.0122657726141079,
-0.00873735943598018));
#42657=CARTESIAN_POINT('Ctrl Pts',(-0.196178593504016,0.0122696352114626,
-0.00874365008834643));
#42658=CARTESIAN_POINT('Ctrl Pts',(-0.196179497116263,0.0122741246939188,
-0.0087494203249196));
#42659=CARTESIAN_POINT('Ctrl Pts',(-0.196183298204856,0.0122850418366192,
-0.00876078948869322));
#42660=CARTESIAN_POINT('Ctrl Pts',(-0.196186480913547,0.0122914983868392,
-0.00876596141165356));
#42661=CARTESIAN_POINT('Ctrl Pts',(-0.196196807521002,0.0123089144864881,
-0.00877700827511887));
#42662=CARTESIAN_POINT('Ctrl Pts',(-0.196205561788726,0.0123208470597291,
-0.00878177623550929));
#42663=CARTESIAN_POINT('Ctrl Pts',(-0.196226774624743,0.0123456471402386,
-0.00878664780234662));
#42664=CARTESIAN_POINT('Ctrl Pts',(-0.196238473381177,0.0123576756480076,
-0.00878665704379384));
#42665=CARTESIAN_POINT('Ctrl Pts',(-0.196268052178449,0.0123853044299795,
-0.00878221469990786));
#42666=CARTESIAN_POINT('Ctrl Pts',(-0.196282603444165,0.0123965725498106,
-0.00877615578657818));
#42667=CARTESIAN_POINT('Ctrl Pts',(-0.196287641730374,0.0124001756233988,
-0.00877423853623206));
#42668=CARTESIAN_POINT('Ctrl Pts',(-0.196288528605167,0.0124009623318482,
-0.00877379890479523));
#42669=CARTESIAN_POINT('Ctrl Pts',(-0.196289718507424,0.0124020131242311,
-0.00877320367624877));
#42670=CARTESIAN_POINT('Ctrl Pts',(-0.196290669616441,0.0124027311765942,
-0.00877278680607922));
#42671=CARTESIAN_POINT('Origin',(-0.196341545593896,0.0123508451352711,
-0.00868829058453999));
#42672=CARTESIAN_POINT('Ctrl Pts',(-0.195178186257962,0.0122660193327441,
-0.00871622481824284));
#42673=CARTESIAN_POINT('Ctrl Pts',(-0.195178062117413,0.0122699395566604,
-0.00872278463078486));
#42674=CARTESIAN_POINT('Ctrl Pts',(-0.19517717113751,0.01227456152034,-0.00872879452985443));
#42675=CARTESIAN_POINT('Ctrl Pts',(-0.195173803716855,0.0122855263357825,
-0.00874013753178816));
#42676=CARTESIAN_POINT('Ctrl Pts',(-0.195171205718012,0.0122918678938226,
-0.00874518558968226));
#42677=CARTESIAN_POINT('Ctrl Pts',(-0.195162766091553,0.0123092764218653,
-0.00875598869146529));
#42678=CARTESIAN_POINT('Ctrl Pts',(-0.195155758242141,0.0123211961066292,
-0.00876051392612621));
#42679=CARTESIAN_POINT('Ctrl Pts',(-0.195139426702041,0.0123453268207502,
-0.00876464314654035));
#42680=CARTESIAN_POINT('Ctrl Pts',(-0.195130748768623,0.0123568030843096,
-0.00876447107949463));
#42681=CARTESIAN_POINT('Ctrl Pts',(-0.195110565284845,0.0123812771519621,
-0.00876016692235031));
#42682=CARTESIAN_POINT('Ctrl Pts',(-0.195100847936894,0.0123915253633481,
-0.0087554973074796));
#42683=CARTESIAN_POINT('Ctrl Pts',(-0.195093918061207,0.0123987217349169,
-0.00875163241365004));
#42684=CARTESIAN_POINT('Ctrl Pts',(-0.195091762741309,0.0124008562183796,
-0.00875045798311553));
#42685=CARTESIAN_POINT('Ctrl Pts',(-0.195089598961392,0.0124029310378485,
-0.00874919540157183));
#42686=CARTESIAN_POINT('Ctrl Pts',(-0.195088833371886,0.0124036830345601,
-0.00874872568289234));
#42687=CARTESIAN_POINT('Ctrl Pts',(-0.196360859055032,0.00216539872082755,
-0.0084957276445973));
#42688=CARTESIAN_POINT('Ctrl Pts',(-0.196258419764256,0.00215450188122847,
-0.00848894461062484));
#42689=CARTESIAN_POINT('Ctrl Pts',(-0.196261052500308,0.0022128124146575,
-0.00840377953460924));
#42690=CARTESIAN_POINT('Ctrl Pts',(-0.196223045774824,0.00301432493259675,
-0.00907396806990626));
#42691=CARTESIAN_POINT('Ctrl Pts',(-0.196120950035656,0.00299980977736295,
-0.00906689178531951));
#42692=CARTESIAN_POINT('Ctrl Pts',(-0.196123832235526,0.00304903240287206,
-0.00897545177118993));
#42693=CARTESIAN_POINT('Ctrl Pts',(-0.195949440420333,0.00490801871463543,
-0.00995116756051316));
#42694=CARTESIAN_POINT('Ctrl Pts',(-0.195845375145333,0.0049082851633093,
-0.00995414531367647));
#42695=CARTESIAN_POINT('Ctrl Pts',(-0.195848630152971,0.00493640698987308,
-0.00985293981030764));
#42696=CARTESIAN_POINT('Ctrl Pts',(-0.196162805580697,0.00699303769490664,
-0.0101844271380545));
#42697=CARTESIAN_POINT('Ctrl Pts',(-0.196060106214048,0.00700321707520669,
-0.0101848308040456));
#42698=CARTESIAN_POINT('Ctrl Pts',(-0.196063484599428,0.00700873741859737,
-0.0100811512250887));
#42699=CARTESIAN_POINT('Ctrl Pts',(-0.196246088270428,0.0080244759576494,
-0.010128210116568));
#42700=CARTESIAN_POINT('Ctrl Pts',(-0.196143162629668,0.0080328845270849,
-0.0101276651591394));
#42701=CARTESIAN_POINT('Ctrl Pts',(-0.19614651707733,0.00802701036852833,
-0.0100246338495604));
#42702=CARTESIAN_POINT('Ctrl Pts',(-0.196289742534361,0.00260194524226652,
-0.00877560306114225));
#42703=CARTESIAN_POINT('Ctrl Pts',(-0.196288786200047,0.00260266660909066,
-0.00877602123122052));
#42704=CARTESIAN_POINT('Ctrl Pts',(-0.196285968132903,0.00260474797982421,
-0.00877719370784045));
#42705=CARTESIAN_POINT('Ctrl Pts',(-0.196283156230408,0.00260689684470671,
-0.00877827782189942));
#42706=CARTESIAN_POINT('Ctrl Pts',(-0.196274251636572,0.0026140066765926,
-0.00878179470519303));
#42707=CARTESIAN_POINT('Ctrl Pts',(-0.196261536227681,0.00262436289230868,
-0.00878607841666256));
#42708=CARTESIAN_POINT('Ctrl Pts',(-0.196235746780876,0.00264877543324927,
-0.0087894236856269));
#42709=CARTESIAN_POINT('Ctrl Pts',(-0.196224650451408,0.00266029252809556,
-0.00878921975691903));
#42710=CARTESIAN_POINT('Ctrl Pts',(-0.196204084518718,0.00268445893936962,
-0.0087842549155602));
#42711=CARTESIAN_POINT('Ctrl Pts',(-0.196195454090691,0.0026962902459704,
-0.00877942124973539));
#42712=CARTESIAN_POINT('Ctrl Pts',(-0.196185330292752,0.00271349490247852,
-0.0087683461936074));
#42713=CARTESIAN_POINT('Ctrl Pts',(-0.196182229953234,0.00271983855251691,
-0.00876320809297492));
#42714=CARTESIAN_POINT('Ctrl Pts',(-0.196178527572347,0.00273057143602513,
-0.00875195367137863));
#42715=CARTESIAN_POINT('Ctrl Pts',(-0.196177648234497,0.00273498997121092,
-0.00874625028219231));
#42716=CARTESIAN_POINT('Ctrl Pts',(-0.196177672764501,0.00273879794676223,
-0.00874004230177787));
#42717=CARTESIAN_POINT('Ctrl Pts',(-0.195151512881996,0.0128416298218532,
-0.00846798718889344));
#42718=CARTESIAN_POINT('Ctrl Pts',(-0.195257533665328,0.0128354320026905,
-0.00848244732337054));
#42719=CARTESIAN_POINT('Ctrl Pts',(-0.195258449269627,0.0127751450299946,
-0.00839383594353875));
#42720=CARTESIAN_POINT('Ctrl Pts',(-0.195013512946357,0.0119916599223204,
-0.00904620160107736));
#42721=CARTESIAN_POINT('Ctrl Pts',(-0.195119177707696,0.0119810415291948,
-0.00906147061869671));
#42722=CARTESIAN_POINT('Ctrl Pts',(-0.195120346851283,0.0119302472688995,
-0.00896634073060416));
#42723=CARTESIAN_POINT('Ctrl Pts',(-0.19474419779016,0.0100934298404086,
-0.00992451520905792));
#42724=CARTESIAN_POINT('Ctrl Pts',(-0.194851869541245,0.0100962523749268,
-0.00993022299987102));
#42725=CARTESIAN_POINT('Ctrl Pts',(-0.194853453840199,0.0100670813731654,
-0.00982518221735306));
#42726=CARTESIAN_POINT('Ctrl Pts',(-0.194954744813264,0.00800503115987945,
-0.01015709544763));
#42727=CARTESIAN_POINT('Ctrl Pts',(-0.195060981356294,0.00801591560822246,
-0.0101657750852207));
#42728=CARTESIAN_POINT('Ctrl Pts',(-0.195062668194003,0.00801003144821768,
-0.0100581030663914));
#42729=CARTESIAN_POINT('Ctrl Pts',(-0.195038043104025,0.00697226031195997,
-0.0101005913568823));
#42730=CARTESIAN_POINT('Ctrl Pts',(-0.195144503954932,0.00698045989555377,
-0.0101101622792698));
#42731=CARTESIAN_POINT('Ctrl Pts',(-0.195146172454993,0.00698641929249386,
-0.0100031578282662));
#42732=CARTESIAN_POINT('Ctrl Pts',(-0.195102857644659,0.00750349585794822,
-0.0100174022791646));
#42733=CARTESIAN_POINT('Ctrl Pts',(-0.195102692485452,0.00750349828746446,
-0.0100238436041747));
#42734=CARTESIAN_POINT('Ctrl Pts',(-0.195101902927751,0.00750350069849524,
-0.0100302536786726));
#42735=CARTESIAN_POINT('Ctrl Pts',(-0.195098984922983,0.00750350560621888,
-0.0100433363955074));
#42736=CARTESIAN_POINT('Ctrl Pts',(-0.195096762496158,0.00750350808045609,
-0.01004995205496));
#42737=CARTESIAN_POINT('Ctrl Pts',(-0.19508851666777,0.00750351480991936,
-0.0100679985225843));
#42738=CARTESIAN_POINT('Ctrl Pts',(-0.195080946642692,0.0075035187252091,
-0.0100785670046555));
#42739=CARTESIAN_POINT('Ctrl Pts',(-0.195062215021252,0.00750352524311888,
-0.0100962618421349));
#42740=CARTESIAN_POINT('Ctrl Pts',(-0.195051227202046,0.00750352777528599,
-0.0101032216500095));
#42741=CARTESIAN_POINT('Ctrl Pts',(-0.195019265131039,0.00750353239339205,
-0.0101157282328778));
#42742=CARTESIAN_POINT('Ctrl Pts',(-0.195002697277718,0.00750350507918231,
-0.0101148512928373));
#42743=CARTESIAN_POINT('Ctrl Pts',(-0.19500072306832,0.00750355266323356,
-0.0101148197542948));
#42744=CARTESIAN_POINT('Ctrl Pts',(-0.195000280301755,0.00750353145507257,
-0.0101148105148487));
#42745=CARTESIAN_POINT('Origin',(-0.195016358203128,0.0026516719625554,
-0.00866391662495163));
#42746=CARTESIAN_POINT('Ctrl Pts',(-0.195178060704217,0.00273781719008554,
-0.00871849522740191));
#42747=CARTESIAN_POINT('Ctrl Pts',(-0.19517762418566,0.00272412448858684,
-0.00874143587971001));
#42748=CARTESIAN_POINT('Ctrl Pts',(-0.195163543470347,0.00269262426172652,
-0.00876037467869015));
#42749=CARTESIAN_POINT('Ctrl Pts',(-0.195146481811715,0.00266914690574364,
-0.00876512160782382));
#42750=CARTESIAN_POINT('Ctrl Pts',(-0.195130973719132,0.00264780730342053,
-0.00876943630067265));
#42751=CARTESIAN_POINT('Ctrl Pts',(-0.19511874958781,0.0026308641930614,
-0.0087672708333908));
#42752=CARTESIAN_POINT('Ctrl Pts',(-0.195095892349715,0.00260729719483703,
-0.0087551043908356));
#42753=CARTESIAN_POINT('Ctrl Pts',(-0.195093602562696,0.00260493630563481,
-0.00875388558381637));
#42754=CARTESIAN_POINT('Ctrl Pts',(-0.195091215951724,0.00260253308819682,
-0.00875252862861909));
#42755=CARTESIAN_POINT('Ctrl Pts',(-0.195088737224831,0.00260009358768204,
-0.00875100653258347));
#42756=CARTESIAN_POINT('Ctrl Pts',(-0.195258515249865,0.00222833195472316,
-0.00839606745134456));
#42757=CARTESIAN_POINT('Ctrl Pts',(-0.195257715261884,0.00216794822738603,
-0.00848493156407439));
#42758=CARTESIAN_POINT('Ctrl Pts',(-0.195151448734371,0.00216179672804389,
-0.00847031066803133));
#42759=CARTESIAN_POINT('Ctrl Pts',(-0.195120023433732,0.00307389698912644,
-0.00896847560096047));
#42760=CARTESIAN_POINT('Ctrl Pts',(-0.195118969009728,0.00302304055807606,
-0.00906387341398073));
#42761=CARTESIAN_POINT('Ctrl Pts',(-0.195013060612715,0.00301242429812119,
-0.00904843195044751));
#42762=CARTESIAN_POINT('Ctrl Pts',(-0.194853142386239,0.00493839989964462,
-0.00982675338910633));
#42763=CARTESIAN_POINT('Ctrl Pts',(-0.194851674310384,0.00490921859900544,
-0.00993206859484722));
#42764=CARTESIAN_POINT('Ctrl Pts',(-0.19474374897434,0.00491214826721647,
-0.00992622756956082));
#42765=CARTESIAN_POINT('Ctrl Pts',(-0.195062706736678,0.00699673232562924,
-0.0100584265394132));
#42766=CARTESIAN_POINT('Ctrl Pts',(-0.195061134895631,0.00699090164734755,
-0.0101663685336579));
#42767=CARTESIAN_POINT('Ctrl Pts',(-0.194954650496018,0.00700179905759746,
-0.0101575132200674));
#42768=CARTESIAN_POINT('Ctrl Pts',(-0.195146170526654,0.00802082773606981,
-0.0100026394254629));
#42769=CARTESIAN_POINT('Ctrl Pts',(-0.195144617516619,0.00802687470231159,
-0.0101099032731655));
#42770=CARTESIAN_POINT('Ctrl Pts',(-0.195037908039177,0.00803507912154476,
-0.0101001626767837));
#42771=CARTESIAN_POINT('Ctrl Pts',(-0.222249881326672,0.00687543454306065,
-0.010708608705939));
#42772=CARTESIAN_POINT('Ctrl Pts',(-0.222147507675063,0.00686704591829485,
-0.0107075587151972));
#42773=CARTESIAN_POINT('Ctrl Pts',(-0.22215063088296,0.00687429739500378,
-0.0106051559466831));
#42774=CARTESIAN_POINT('Ctrl Pts',(-0.22213303026492,0.00811344210707129,
-0.0107938596287791));
#42775=CARTESIAN_POINT('Ctrl Pts',(-0.222030943630378,0.00810248190675591,
-0.010794192368089));
#42776=CARTESIAN_POINT('Ctrl Pts',(-0.222034098562025,0.00809546126778267,
-0.0106907816028563));
#42777=CARTESIAN_POINT('Ctrl Pts',(-0.221994531826128,0.00993476248926103,
-0.0105419142089085));
#42778=CARTESIAN_POINT('Ctrl Pts',(-0.221891182125483,0.00993371370083797,
-0.0105441094985628));
#42779=CARTESIAN_POINT('Ctrl Pts',(-0.221894227111855,0.00990623992118876,
-0.0104434861240904));
#42780=CARTESIAN_POINT('Ctrl Pts',(-0.222202931566564,0.0122478622459772,
-0.00946095837100554));
#42781=CARTESIAN_POINT('Ctrl Pts',(-0.222101383624784,0.0122634552700619,
-0.00945277921907509));
#42782=CARTESIAN_POINT('Ctrl Pts',(-0.222103981254199,0.0122092535606527,
-0.00936466720929235));
#42783=CARTESIAN_POINT('Ctrl Pts',(-0.222503016192992,0.0132233862244586,
-0.00873138285702185));
#42784=CARTESIAN_POINT('Ctrl Pts',(-0.22240314604442,0.0132424080883783,
-0.00871654332699369));
#42785=CARTESIAN_POINT('Ctrl Pts',(-0.222405481336722,0.0131773681473555,
-0.00863664901956425));
#42786=CARTESIAN_POINT('Ctrl Pts',(-0.222649530248401,0.0137486960647823,
-0.00823639965487398));
#42787=CARTESIAN_POINT('Ctrl Pts',(-0.222548877010536,0.0137640118108876,
-0.00822249108542394));
#42788=CARTESIAN_POINT('Ctrl Pts',(-0.222551015132696,0.013692950370958,
-0.00814830722488945));
#42789=CARTESIAN_POINT('Ctrl Pts',(-0.222093148989078,0.00750347905706887,
-0.0106271011600294));
#42790=CARTESIAN_POINT('Ctrl Pts',(-0.222093001117879,0.00750348163845054,
-0.0106336437243019));
#42791=CARTESIAN_POINT('Ctrl Pts',(-0.222093498230638,0.00750348439599822,
-0.0106401846244798));
#42792=CARTESIAN_POINT('Ctrl Pts',(-0.222095839546678,0.00750349036668899,
-0.0106534840158653));
#42793=CARTESIAN_POINT('Ctrl Pts',(-0.222097760699624,0.0075034935809392,
-0.0106601927381583));
#42794=CARTESIAN_POINT('Ctrl Pts',(-0.222105182881688,0.00750350298274059,
-0.0106785933030817));
#42795=CARTESIAN_POINT('Ctrl Pts',(-0.222112268300804,0.00750350928445525,
-0.0106894933245119));
#42796=CARTESIAN_POINT('Ctrl Pts',(-0.222130183071353,0.00750352156683749,
-0.0107080173739093));
#42797=CARTESIAN_POINT('Ctrl Pts',(-0.222140846494675,0.00750352744091401,
-0.0107154669821436));
#42798=CARTESIAN_POINT('Ctrl Pts',(-0.222172223478591,0.00750354134005543,
-0.0107294102153455));
#42799=CARTESIAN_POINT('Ctrl Pts',(-0.222188823735049,0.00750357107008051,
-0.0107292797619568));
#42800=CARTESIAN_POINT('Ctrl Pts',(-0.22219077671284,0.00750352632614256,
-0.0107293370430334));
#42801=CARTESIAN_POINT('Ctrl Pts',(-0.222191219494722,0.00750354683273177,
-0.0107293478392253));
#42802=CARTESIAN_POINT('Ctrl Pts',(-0.222392848909985,0.013140240706079,
-0.0086347107226525));
#42803=CARTESIAN_POINT('Ctrl Pts',(-0.222392878685365,0.0131452498761335,
-0.00864065169899928));
#42804=CARTESIAN_POINT('Ctrl Pts',(-0.222394028589284,0.0131508377990427,
-0.00864589817563944));
#42805=CARTESIAN_POINT('Ctrl Pts',(-0.222398741299102,0.0131641425680373,
-0.00865593592085266));
#42806=CARTESIAN_POINT('Ctrl Pts',(-0.222402690636142,0.0131718061837692,
-0.00866018291654182));
#42807=CARTESIAN_POINT('Ctrl Pts',(-0.222415044365568,0.0131914856188858,
-0.00866832547181801));
#42808=CARTESIAN_POINT('Ctrl Pts',(-0.222425289775166,0.0132043797156318,
-0.00867097294064302));
#42809=CARTESIAN_POINT('Ctrl Pts',(-0.222448469021798,0.0132287804888377,
-0.00867124055874764));
#42810=CARTESIAN_POINT('Ctrl Pts',(-0.222460225938644,0.0132395460799034,
-0.00866944454699309));
#42811=CARTESIAN_POINT('Ctrl Pts',(-0.222488865700657,0.0132630567621544,
-0.00866184603742375));
#42812=CARTESIAN_POINT('Ctrl Pts',(-0.222502612807788,0.0132721998107884,
-0.00865561866607119));
#42813=CARTESIAN_POINT('Ctrl Pts',(-0.222508839896806,0.0132761722127939,
-0.00865279538552127));
#42814=CARTESIAN_POINT('Ctrl Pts',(-0.222511979440178,0.0132782693982421,
-0.00865128616260161));
#42815=CARTESIAN_POINT('Ctrl Pts',(-0.222515313566668,0.0132804052496997,
-0.00864958136878297));
#42816=CARTESIAN_POINT('Origin',(-0.222557069576793,0.0132165166889543,
-0.00857342793229397));
#42817=CARTESIAN_POINT('Ctrl Pts',(-0.221393342144309,0.013140302186429,
-0.00861407581869929));
#42818=CARTESIAN_POINT('Ctrl Pts',(-0.221392512653964,0.0131790082731684,
-0.00866137407639872));
#42819=CARTESIAN_POINT('Ctrl Pts',(-0.221357898020299,0.0132523373781119,
-0.00865122754666828));
#42820=CARTESIAN_POINT('Ctrl Pts',(-0.221311658118836,0.0132815271509267,
-0.00862621264935379));
#42821=CARTESIAN_POINT('Ctrl Pts',(-0.22215041348331,0.0081317000139514,
-0.010604324930572));
#42822=CARTESIAN_POINT('Ctrl Pts',(-0.222146866536432,0.00813909558534202,
-0.0107072984786383));
#42823=CARTESIAN_POINT('Ctrl Pts',(-0.222249835659344,0.00813070245192706,
-0.0107081718331986));
#42824=CARTESIAN_POINT('Ctrl Pts',(-0.222033898159491,0.00691248699556566,
-0.0106906639957997));
#42825=CARTESIAN_POINT('Ctrl Pts',(-0.222030320528098,0.00690556431974724,
-0.0107946638061863));
#42826=CARTESIAN_POINT('Ctrl Pts',(-0.222133004724419,0.00689459044374911,
-0.0107941464062241));
#42827=CARTESIAN_POINT('Ctrl Pts',(-0.2218981179966,0.00510426517379774,
-0.0104455594933188));
#42828=CARTESIAN_POINT('Ctrl Pts',(-0.221894644006361,0.00507676318916403,
-0.0105467911269829));
#42829=CARTESIAN_POINT('Ctrl Pts',(-0.221998582688886,0.00507586896512953,
-0.0105444525401242));
#42830=CARTESIAN_POINT('Ctrl Pts',(-0.222106568628605,0.00280338838995331,
-0.00937174878353225));
#42831=CARTESIAN_POINT('Ctrl Pts',(-0.222103550983437,0.00274895782721167,
-0.00946041018195773));
#42832=CARTESIAN_POINT('Ctrl Pts',(-0.222205687874948,0.00276476336427084,
-0.00946845290383881));
#42833=CARTESIAN_POINT('Ctrl Pts',(-0.222411478982832,0.00183582509294618,
-0.00864683768561999));
#42834=CARTESIAN_POINT('Ctrl Pts',(-0.222408729806004,0.001770486407663,
-0.00872724372961482));
#42835=CARTESIAN_POINT('Ctrl Pts',(-0.222509093970282,0.00179005747630213,
-0.00874221305404969));
#42836=CARTESIAN_POINT('Ctrl Pts',(-0.222558531085189,0.00132037684913637,
-0.00816064415141273));
#42837=CARTESIAN_POINT('Ctrl Pts',(-0.222555975148884,0.00124900577222267,
-0.00823534029207931));
#42838=CARTESIAN_POINT('Ctrl Pts',(-0.222657166444787,0.00126470219399182,
-0.00824931224599372));
#42839=CARTESIAN_POINT('Ctrl Pts',(-0.222519811891068,0.00173281601266729,
-0.00866059802620759));
#42840=CARTESIAN_POINT('Ctrl Pts',(-0.222519711787491,0.00173312127539872,
-0.00866084823972965));
#42841=CARTESIAN_POINT('Ctrl Pts',(-0.222519594558049,0.00173330438501034,
-0.00866099618213166));
#42842=CARTESIAN_POINT('Ctrl Pts',(-0.222519140601718,0.00173381349151495,
-0.00866140162405847));
#42843=CARTESIAN_POINT('Ctrl Pts',(-0.222518709616375,0.00173417891196423,
-0.00866168844501488));
#42844=CARTESIAN_POINT('Ctrl Pts',(-0.222517104151076,0.00173536521354638,
-0.00866259377003072));
#42845=CARTESIAN_POINT('Ctrl Pts',(-0.222515819635713,0.00173622911476649,
-0.00866323065497129));
#42846=CARTESIAN_POINT('Ctrl Pts',(-0.222511061100675,0.00173943859314526,
-0.00866552948731959));
#42847=CARTESIAN_POINT('Ctrl Pts',(-0.222503603668941,0.00174438148073145,
-0.00866891690307697));
#42848=CARTESIAN_POINT('Ctrl Pts',(-0.222475754872163,0.00176507779554153,
-0.00867887860705707));
#42849=CARTESIAN_POINT('Ctrl Pts',(-0.222458582137689,0.00178014243579629,
-0.00868222267468587));
#42850=CARTESIAN_POINT('Ctrl Pts',(-0.222431452624928,0.00180853115651544,
-0.00868199708331077));
#42851=CARTESIAN_POINT('Ctrl Pts',(-0.222421094900015,0.0018214782425271,
-0.00867936980954872));
#42852=CARTESIAN_POINT('Ctrl Pts',(-0.22240857660096,0.00184126011996096,
-0.00867122308273688));
#42853=CARTESIAN_POINT('Ctrl Pts',(-0.222404561479792,0.00184898184210888,
-0.00866695439586749));
#42854=CARTESIAN_POINT('Ctrl Pts',(-0.222399771942874,0.00186237598235397,
-0.00865684643894828));
#42855=CARTESIAN_POINT('Ctrl Pts',(-0.222398602189169,0.00186799481674966,
-0.00865156303303412));
#42856=CARTESIAN_POINT('Ctrl Pts',(-0.222398570120677,0.0018730271297317,
-0.008645575543849));
#42857=CARTESIAN_POINT('Ctrl Pts',(-0.221150464830925,0.00688034370022854,
-0.010582553178107));
#42858=CARTESIAN_POINT('Ctrl Pts',(-0.221149540493208,0.00687264310985869,
-0.0106927174515397));
#42859=CARTESIAN_POINT('Ctrl Pts',(-0.221040105820209,0.00686441410916952,
-0.0106801811534307));
#42860=CARTESIAN_POINT('Ctrl Pts',(-0.221032681327501,0.00810843535542784,
-0.0106668215581535));
#42861=CARTESIAN_POINT('Ctrl Pts',(-0.221031730409529,0.00811613590506075,
-0.0107780620582133));
#42862=CARTESIAN_POINT('Ctrl Pts',(-0.220922572418371,0.00810366232374963,
-0.0107669088928184));
#42863=CARTESIAN_POINT('Ctrl Pts',(-0.220896606320941,0.00990275697441929,
-0.0104177217566761));
#42864=CARTESIAN_POINT('Ctrl Pts',(-0.220895748847351,0.009932200154217,
-0.0105259351302228));
#42865=CARTESIAN_POINT('Ctrl Pts',(-0.220785304732471,0.00992817015338086,
-0.0105169648004527));
#42866=CARTESIAN_POINT('Ctrl Pts',(-0.221099708280645,0.0121797433482338,
-0.00935944466440972));
#42867=CARTESIAN_POINT('Ctrl Pts',(-0.221099353535905,0.0122375562745181,
-0.00945449197733792));
#42868=CARTESIAN_POINT('Ctrl Pts',(-0.220990602690162,0.0122475181246042,
-0.00943636041410781));
#42869=CARTESIAN_POINT('Ctrl Pts',(-0.221395176166451,0.0131433495521379,
-0.00864446468980765));
#42870=CARTESIAN_POINT('Ctrl Pts',(-0.221395137837132,0.0132127320462371,
-0.00873085305611693));
#42871=CARTESIAN_POINT('Ctrl Pts',(-0.221288309650929,0.0132261159542827,
-0.00870596282060123));
#42872=CARTESIAN_POINT('Ctrl Pts',(-0.221544135263697,0.0136675288337307,
-0.00815436056670324));
#42873=CARTESIAN_POINT('Ctrl Pts',(-0.221544294911465,0.0137435040814762,
-0.00823459311628976));
#42874=CARTESIAN_POINT('Ctrl Pts',(-0.221436574138446,0.0137519902155352,
-0.0082114432028954));
#42875=CARTESIAN_POINT('Ctrl Pts',(-0.221093381485671,0.00750288700333877,
-0.0106049435316979));
#42876=CARTESIAN_POINT('Ctrl Pts',(-0.22109320880867,0.00750288906317748,
-0.0106113416698315));
#42877=CARTESIAN_POINT('Ctrl Pts',(-0.221092419982598,0.00750289094644645,
-0.0106177083341688));
#42878=CARTESIAN_POINT('Ctrl Pts',(-0.221089509680449,0.0075028944558648,
-0.0106307512649));
#42879=CARTESIAN_POINT('Ctrl Pts',(-0.22108728565415,0.00750289603503224,
-0.0106373687796944));
#42880=CARTESIAN_POINT('Ctrl Pts',(-0.221079035395588,0.00750289975374608,
-0.0106554166409915));
#42881=CARTESIAN_POINT('Ctrl Pts',(-0.221071462762515,0.00750290119227914,
-0.0106659843001971));
#42882=CARTESIAN_POINT('Ctrl Pts',(-0.221052726190283,0.0075029019784618,
-0.0106836767790163));
#42883=CARTESIAN_POINT('Ctrl Pts',(-0.221041736012401,0.00750290130802815,
-0.0106906350161983));
#42884=CARTESIAN_POINT('Ctrl Pts',(-0.221016461332956,0.00750289787870694,
-0.0107005197427617));
#42885=CARTESIAN_POINT('Ctrl Pts',(-0.221003806041523,0.00750288073417112,
-0.0107022177264459));
#42886=CARTESIAN_POINT('Ctrl Pts',(-0.220992863211399,0.00750289680848803,
-0.0107022436617203));
#42887=CARTESIAN_POINT('Ctrl Pts',(-0.220992438489933,0.00750289754619727,
-0.0107022417574986));
#42888=CARTESIAN_POINT('Ctrl Pts',(-0.220991844919555,0.0075029014952033,
-0.0107022357170612));
#42889=CARTESIAN_POINT('Ctrl Pts',(-0.220991596752038,0.00750290355364233,
-0.0107022324043892));
#42890=CARTESIAN_POINT('Ctrl Pts',(-0.220991244605229,0.00750291318074831,
-0.0107022266022728));
#42891=CARTESIAN_POINT('Ctrl Pts',(-0.220990866858029,0.00750300510925417,
-0.0107022189130647));
#42892=CARTESIAN_POINT('Origin',(-0.221237471898473,0.00179552890401392,
-0.0085587796007864));
#42893=CARTESIAN_POINT('Ctrl Pts',(-0.221399010012836,0.00187318766792258,
-0.00862507770872998));
#42894=CARTESIAN_POINT('Ctrl Pts',(-0.221398907349878,0.00186835774631689,
-0.00863100475221132));
#42895=CARTESIAN_POINT('Ctrl Pts',(-0.22139810388374,0.00186290294648796,
-0.0086362961021297));
#42896=CARTESIAN_POINT('Ctrl Pts',(-0.221395045281478,0.00185039344029363,
-0.00864594208587137));
#42897=CARTESIAN_POINT('Ctrl Pts',(-0.221392681904453,0.0018433694093753,
-0.00865003605187046));
#42898=CARTESIAN_POINT('Ctrl Pts',(-0.221384736880726,0.00182393207571952,
-0.00865848009275339));
#42899=CARTESIAN_POINT('Ctrl Pts',(-0.221378173054657,0.0018113553860032,
-0.00866102038332009));
#42900=CARTESIAN_POINT('Ctrl Pts',(-0.221363548830083,0.00178732269172333,
-0.00866159342441401));
#42901=CARTESIAN_POINT('Ctrl Pts',(-0.2213555333964,0.00177585407827663,
-0.00865973428883798));
#42902=CARTESIAN_POINT('Ctrl Pts',(-0.221335870803864,0.00175074374557391,
-0.00865135187979251));
#42903=CARTESIAN_POINT('Ctrl Pts',(-0.22132649230484,0.00174100645599888,
-0.00864446213309051));
#42904=CARTESIAN_POINT('Ctrl Pts',(-0.22132190932138,0.00173649085409544,
-0.00864108723501383));
#42905=CARTESIAN_POINT('Ctrl Pts',(-0.221319832849445,0.0017343171811537,
-0.00863944412245893));
#42906=CARTESIAN_POINT('Ctrl Pts',(-0.221317763839132,0.00173223151638979,
-0.00863769727779015));
#42907=CARTESIAN_POINT('Ctrl Pts',(-0.221317525382339,0.00173199991205511,
-0.00863750196330413));
#42908=CARTESIAN_POINT('Ctrl Pts',(-0.221039493952704,0.00814028259742471,
-0.0106798048749903));
#42909=CARTESIAN_POINT('Ctrl Pts',(-0.221149177384937,0.00813212789921885,
-0.0106927176453606));
#42910=CARTESIAN_POINT('Ctrl Pts',(-0.221150165198724,0.00812434479483271,
-0.010582274352994));
#42911=CARTESIAN_POINT('Ctrl Pts',(-0.220922252472739,0.00690325684720192,
-0.0107670349642513));
#42912=CARTESIAN_POINT('Ctrl Pts',(-0.22103166212434,0.00689077782194489,
-0.0107785678254041));
#42913=CARTESIAN_POINT('Ctrl Pts',(-0.221032676501381,0.00689840577890317,
-0.0106670390937617));
#42914=CARTESIAN_POINT('Ctrl Pts',(-0.220788221206417,0.00508184180165128,
-0.0105191990487672));
#42915=CARTESIAN_POINT('Ctrl Pts',(-0.220898905314294,0.00507784583507543,
-0.0105285860406717));
#42916=CARTESIAN_POINT('Ctrl Pts',(-0.22089982808778,0.00510723661303933,
-0.0104200629949558));
#42917=CARTESIAN_POINT('Ctrl Pts',(-0.22099337460045,0.00276507260651043,
-0.00944375885445184));
#42918=CARTESIAN_POINT('Ctrl Pts',(-0.221102369107793,0.00277493695513631,
-0.00946223082472947));
#42919=CARTESIAN_POINT('Ctrl Pts',(-0.221102788022272,0.00283275709507392,
-0.00936685532907095));
#42920=CARTESIAN_POINT('Ctrl Pts',(-0.221293701763668,0.00178742795253052,
-0.00871679057028318));
#42921=CARTESIAN_POINT('Ctrl Pts',(-0.221400695380101,0.00180094083600155,
-0.00874219231644764));
#42922=CARTESIAN_POINT('Ctrl Pts',(-0.221400797118254,0.00187034626191687,
-0.00865545652030308));
#42923=CARTESIAN_POINT('Ctrl Pts',(-0.221443367427878,0.00126174482639335,
-0.00822459051870288));
#42924=CARTESIAN_POINT('Ctrl Pts',(-0.221551288994416,0.00127019986002699,
-0.00824817907764156));
#42925=CARTESIAN_POINT('Ctrl Pts',(-0.221551195199306,0.00134620621622744,
-0.00816758272347228));
#42926=CARTESIAN_POINT('Ctrl Pts',(-0.220250306618512,0.0068767635851955,
-0.0106635861607493));
#42927=CARTESIAN_POINT('Ctrl Pts',(-0.220147856493154,0.00686835894786593,
-0.0106626255349507));
#42928=CARTESIAN_POINT('Ctrl Pts',(-0.220150969995606,0.00687557763149086,
-0.0105601412393206));
#42929=CARTESIAN_POINT('Ctrl Pts',(-0.220133883086356,0.00811004854082277,
-0.0107480074268753));
#42930=CARTESIAN_POINT('Ctrl Pts',(-0.220031713557015,0.00809906691085948,
-0.0107484381821638));
#42931=CARTESIAN_POINT('Ctrl Pts',(-0.22003485851762,0.00809210119000192,
-0.0106449585226562));
#42932=CARTESIAN_POINT('Ctrl Pts',(-0.219995660265109,0.00992369026213599,
-0.0104991498138423));
#42933=CARTESIAN_POINT('Ctrl Pts',(-0.21989225493449,0.00992270949191421,
-0.0105013643797054));
#42934=CARTESIAN_POINT('Ctrl Pts',(-0.21989529130248,0.00989542327015895,
-0.0104006294419025));
#42935=CARTESIAN_POINT('Ctrl Pts',(-0.220201022339521,0.0122315251788832,
-0.00942943555407081));
#42936=CARTESIAN_POINT('Ctrl Pts',(-0.220099353543913,0.012246971481956,
-0.00942151978304597));
#42937=CARTESIAN_POINT('Ctrl Pts',(-0.220101943743354,0.012193078903321,
-0.00933313831981191));
#42938=CARTESIAN_POINT('Ctrl Pts',(-0.220498643283846,0.013206679346764,
-0.00870682343419975));
#42939=CARTESIAN_POINT('Ctrl Pts',(-0.220398717237275,0.0132259390201395,
-0.00869206884376114));
#42940=CARTESIAN_POINT('Ctrl Pts',(-0.220401045442068,0.0131612261295782,
-0.00861181318161109));
#42941=CARTESIAN_POINT('Ctrl Pts',(-0.220645208974285,0.0137320975088836,
-0.0082169211442826));
#42942=CARTESIAN_POINT('Ctrl Pts',(-0.220544466885696,0.0137474970413183,
-0.00820318515944086));
#42943=CARTESIAN_POINT('Ctrl Pts',(-0.22054659976056,0.0136767805992873,
-0.00812856487265608));
#42944=CARTESIAN_POINT('Ctrl Pts',(-0.220093677111814,0.00750238403012091,
-0.0105819118104658));
#42945=CARTESIAN_POINT('Ctrl Pts',(-0.220093529239301,0.00750238578936402,
-0.0105884544159041));
#42946=CARTESIAN_POINT('Ctrl Pts',(-0.220094026363594,0.00750238771684917,
-0.0105949953563592));
#42947=CARTESIAN_POINT('Ctrl Pts',(-0.220096367729295,0.00750239198187957,
-0.0106082948310363));
#42948=CARTESIAN_POINT('Ctrl Pts',(-0.220098288922505,0.00750239432577211,
-0.0106150035930982));
#42949=CARTESIAN_POINT('Ctrl Pts',(-0.220105711231248,0.00750240130929248,
-0.0106334041999022));
#42950=CARTESIAN_POINT('Ctrl Pts',(-0.220112796740053,0.00750240614050839,
-0.0106443042059039));
#42951=CARTESIAN_POINT('Ctrl Pts',(-0.220130711695223,0.00750241582164841,
-0.0106628282133226));
#42952=CARTESIAN_POINT('Ctrl Pts',(-0.220141375216936,0.00750242060037397,
-0.0106702777889441));
#42953=CARTESIAN_POINT('Ctrl Pts',(-0.220172641439852,0.00750243204482037,
-0.0106841716126293));
#42954=CARTESIAN_POINT('Ctrl Pts',(-0.220189148542913,0.00750250301964164,
-0.0106840844290246));
#42955=CARTESIAN_POINT('Ctrl Pts',(-0.220191305017738,0.00750239221586241,
-0.0106841477117758));
#42956=CARTESIAN_POINT('Ctrl Pts',(-0.220191748876597,0.00750243783530509,
-0.010684158519063));
#42957=CARTESIAN_POINT('Ctrl Pts',(-0.220393577735485,0.0131409926298503,
-0.00859656506818599));
#42958=CARTESIAN_POINT('Ctrl Pts',(-0.220393600784383,0.0131455013235971,
-0.00860197156800209));
#42959=CARTESIAN_POINT('Ctrl Pts',(-0.220394508723612,0.013150390707749,
-0.00860694383723535));
#42960=CARTESIAN_POINT('Ctrl Pts',(-0.220398273034233,0.0131617074700728,
-0.00861677217987557));
#42961=CARTESIAN_POINT('Ctrl Pts',(-0.22040141745688,0.0131680966885574,
-0.00862129135659766));
#42962=CARTESIAN_POINT('Ctrl Pts',(-0.220411875451266,0.0131850252832542,
-0.00863112133216668));
#42963=CARTESIAN_POINT('Ctrl Pts',(-0.220420838703223,0.0131960597967277,
-0.00863536618801003));
#42964=CARTESIAN_POINT('Ctrl Pts',(-0.220443547262691,0.0132187413918395,
-0.00863979428834782));
#42965=CARTESIAN_POINT('Ctrl Pts',(-0.220456699734264,0.0132295555728947,
-0.00863957428719857));
#42966=CARTESIAN_POINT('Ctrl Pts',(-0.220477028370402,0.0132439117277982,
-0.00863638017660647));
#42967=CARTESIAN_POINT('Ctrl Pts',(-0.220483964499296,0.0132484256939255,
-0.00863482543045935));
#42968=CARTESIAN_POINT('Ctrl Pts',(-0.2204943501556,0.0132546690049436,
-0.00863186022596393));
#42969=CARTESIAN_POINT('Ctrl Pts',(-0.220497771526208,0.0132566431653764,
-0.00863078258852987));
#42970=CARTESIAN_POINT('Ctrl Pts',(-0.220502900998905,0.013259490106136,
-0.00862901351443286));
#42971=CARTESIAN_POINT('Ctrl Pts',(-0.220504589263189,0.013260407142419,
-0.00862840655268303));
#42972=CARTESIAN_POINT('Ctrl Pts',(-0.220507103876826,0.0132617598017022,
-0.00862745672848966));
#42973=CARTESIAN_POINT('Ctrl Pts',(-0.220507997798412,0.01326223654587,
-0.00862711078108925));
#42974=CARTESIAN_POINT('Ctrl Pts',(-0.220509361404001,0.0132629886447625,
-0.00862654885235569));
#42975=CARTESIAN_POINT('Ctrl Pts',(-0.220509756647642,0.0132632201317573,
-0.00862637051561302));
#42976=CARTESIAN_POINT('Ctrl Pts',(-0.22051016964372,0.0132635045056427,
-0.00862614893167951));
#42977=CARTESIAN_POINT('Ctrl Pts',(-0.220510279030594,0.0132635929926122,
-0.00862607912610677));
#42978=CARTESIAN_POINT('Ctrl Pts',(-0.220510520647363,0.0132639284950142,
-0.0086258093258324));
#42979=CARTESIAN_POINT('Ctrl Pts',(-0.219280593258087,0.0129089030369612,
-0.0087540208922909));
#42980=CARTESIAN_POINT('Ctrl Pts',(-0.219279471351069,0.0129697183219162,
-0.00883447223599688));
#42981=CARTESIAN_POINT('Ctrl Pts',(-0.219232227122818,0.01303995698963,
-0.00877963895487713));
#42982=CARTESIAN_POINT('Ctrl Pts',(-0.219480859972423,0.0129956387985517,
-0.00869259253052726));
#42983=CARTESIAN_POINT('Ctrl Pts',(-0.219479765662262,0.0130574432834654,
-0.0087722973921775));
#42984=CARTESIAN_POINT('Ctrl Pts',(-0.219432533921543,0.0131270216872618,
-0.00871660628740151));
#42985=CARTESIAN_POINT('Ctrl Pts',(-0.219777491499906,0.0131256379037001,
-0.00859541257530931));
#42986=CARTESIAN_POINT('Ctrl Pts',(-0.21977673918151,0.0131889796566377,
-0.00867405729017068));
#42987=CARTESIAN_POINT('Ctrl Pts',(-0.219731924878373,0.01326225933775,
-0.0086132441302433));
#42988=CARTESIAN_POINT('Ctrl Pts',(-0.220181220363713,0.0131791518408284,
-0.00855905807384794));
#42989=CARTESIAN_POINT('Ctrl Pts',(-0.220179703043079,0.0132430749198211,
-0.0086374684420407));
#42990=CARTESIAN_POINT('Ctrl Pts',(-0.220187007242741,0.0133222515952173,
-0.00857148014111763));
#42991=CARTESIAN_POINT('Ctrl Pts',(-0.220388732889043,0.0131402149694449,
-0.00859463791750654));
#42992=CARTESIAN_POINT('Ctrl Pts',(-0.220387054388994,0.0132037278064557,
-0.00867326792055314));
#42993=CARTESIAN_POINT('Ctrl Pts',(-0.220408297394784,0.0132801431120848,
-0.00861058770866753));
#42994=CARTESIAN_POINT('Ctrl Pts',(-0.220499526505995,0.013122678869508,
-0.00861080275449944));
#42995=CARTESIAN_POINT('Ctrl Pts',(-0.220497842335634,0.0131860042786699,
-0.0086895830169195));
#42996=CARTESIAN_POINT('Ctrl Pts',(-0.220519081583513,0.0132625694282041,
-0.00862708545017783));
#42997=CARTESIAN_POINT('Ctrl Pts',(-0.219329717540431,0.0129304387340275,
-0.00873922893714474));
#42998=CARTESIAN_POINT('Ctrl Pts',(-0.219329619304978,0.0129346525482004,
-0.0087447320476796));
#42999=CARTESIAN_POINT('Ctrl Pts',(-0.219328881296596,0.0129392175326603,
-0.00874991025846167));
#43000=CARTESIAN_POINT('Ctrl Pts',(-0.219326066620048,0.0129492576252757,
-0.00875981945591603));
#43001=CARTESIAN_POINT('Ctrl Pts',(-0.219323909241627,0.0129547202760547,
-0.00876443358395337));
#43002=CARTESIAN_POINT('Ctrl Pts',(-0.219316118880593,0.0129704063023137,
-0.0087757011237742));
#43003=CARTESIAN_POINT('Ctrl Pts',(-0.219309194587094,0.0129807551150745,
-0.00878091792349644));
#43004=CARTESIAN_POINT('Ctrl Pts',(-0.219292289600658,0.013001250202485,
-0.00878728601601963));
#43005=CARTESIAN_POINT('Ctrl Pts',(-0.21928234369875,0.0130111975838273,
-0.00878821585785464));
#43006=CARTESIAN_POINT('Ctrl Pts',(-0.219260891119607,0.013029288793666,
-0.00878572430074405));
#43007=CARTESIAN_POINT('Ctrl Pts',(-0.219251496806023,0.0130355885641391,
-0.00878249392109267));
#43008=CARTESIAN_POINT('Ctrl Pts',(-0.219243411968739,0.0130407035975206,
-0.00877917947485082));
#43009=CARTESIAN_POINT('Ctrl Pts',(-0.21924126324647,0.0130419515911249,
-0.00877827875086926));
#43010=CARTESIAN_POINT('Ctrl Pts',(-0.219239363903856,0.0130430555261411,
-0.00877739438131471));
#43011=CARTESIAN_POINT('Ctrl Pts',(-0.220150919053116,0.00813012261928148,
-0.0105594969353601));
#43012=CARTESIAN_POINT('Ctrl Pts',(-0.220147560322325,0.00813744816509899,
-0.010662288922204));
#43013=CARTESIAN_POINT('Ctrl Pts',(-0.220250337214706,0.00812906192089311,
-0.0106631669086847));
#43014=CARTESIAN_POINT('Ctrl Pts',(-0.220034517280683,0.00691186126661964,
-0.0106452660313614));
#43015=CARTESIAN_POINT('Ctrl Pts',(-0.220031127462352,0.00690494866270766,
-0.0107490709111982));
#43016=CARTESIAN_POINT('Ctrl Pts',(-0.220133619056969,0.00689398622454344,
-0.0107485661923428));
#43017=CARTESIAN_POINT('Ctrl Pts',(-0.219898176228963,0.00510523286236233,
-0.0104011082367351));
#43018=CARTESIAN_POINT('Ctrl Pts',(-0.219894892210515,0.00507786839668421,
-0.0105021637906976));
#43019=CARTESIAN_POINT('Ctrl Pts',(-0.219998638957578,0.00507695382070288,
-0.0104998409426915));
#43020=CARTESIAN_POINT('Ctrl Pts',(-0.220106792893513,0.0028045235466563,
-0.00933167834600581));
#43021=CARTESIAN_POINT('Ctrl Pts',(-0.220103961877512,0.00275039714016751,
-0.00942029587214831));
#43022=CARTESIAN_POINT('Ctrl Pts',(-0.220205907292707,0.0027661935911115,
-0.00942830878118668));
#43023=CARTESIAN_POINT('Ctrl Pts',(-0.220411551979736,0.00183607302071643,
-0.00860959612604254));
#43024=CARTESIAN_POINT('Ctrl Pts',(-0.220408986658667,0.00177108263111936,
-0.00869003939775851));
#43025=CARTESIAN_POINT('Ctrl Pts',(-0.220509160419223,0.0017906577512894,
-0.00870494804850675));
#43026=CARTESIAN_POINT('Ctrl Pts',(-0.220558570384699,0.00131983115813253,
-0.00812527721236594));
#43027=CARTESIAN_POINT('Ctrl Pts',(-0.220556199753953,0.00124882039973508,
-0.00820005680446187));
#43028=CARTESIAN_POINT('Ctrl Pts',(-0.220657200684646,0.00126452842110998,
-0.00821397254802884));
#43029=CARTESIAN_POINT('Ctrl Pts',(-0.220398945127186,0.00187230965206566,
-0.00860743240415377));
#43030=CARTESIAN_POINT('Ctrl Pts',(-0.220398970043393,0.00186866745817968,
-0.00861178659251786));
#43031=CARTESIAN_POINT('Ctrl Pts',(-0.220399593273686,0.00186470597500052,
-0.00861579151699209));
#43032=CARTESIAN_POINT('Ctrl Pts',(-0.220402930635403,0.00185273261831202,
-0.0086261078828164));
#43033=CARTESIAN_POINT('Ctrl Pts',(-0.220406868913276,0.00184442241414017,
-0.00863127211875914));
#43034=CARTESIAN_POINT('Ctrl Pts',(-0.220418894088141,0.00182454980589882,
-0.00864039997366899));
#43035=CARTESIAN_POINT('Ctrl Pts',(-0.220428439657727,0.00181219952729001,
-0.00864351310290853));
#43036=CARTESIAN_POINT('Ctrl Pts',(-0.220452242219434,0.0017865171103747,
-0.00864509456873525));
#43037=CARTESIAN_POINT('Ctrl Pts',(-0.220465792372549,0.00177414120939264,
-0.00864328267353371));
#43038=CARTESIAN_POINT('Ctrl Pts',(-0.220486501745454,0.00175742793939046,
-0.00863784249252514));
#43039=CARTESIAN_POINT('Ctrl Pts',(-0.220493602587884,0.00175206904922223,
-0.00863552670233257));
#43040=CARTESIAN_POINT('Ctrl Pts',(-0.220504215447333,0.00174455715684026,
-0.00863145439251244));
#43041=CARTESIAN_POINT('Ctrl Pts',(-0.22050771555906,0.00174215999883712,
-0.00863001397738395));
#43042=CARTESIAN_POINT('Ctrl Pts',(-0.220512959035891,0.00173867870828759,
-0.00862770839708991));
#43043=CARTESIAN_POINT('Ctrl Pts',(-0.220514685798646,0.00173755168528413,
-0.00862692540284276));
#43044=CARTESIAN_POINT('Ctrl Pts',(-0.220517267823617,0.00173587973325043,
-0.00862571017892817));
#43045=CARTESIAN_POINT('Ctrl Pts',(-0.220518176036435,0.00173529568430238,
-0.00862527475663612));
#43046=CARTESIAN_POINT('Ctrl Pts',(-0.220519572749422,0.00173437365590044,
-0.00862457224594662));
#43047=CARTESIAN_POINT('Ctrl Pts',(-0.220519976590864,0.00173409409974473,
-0.00862435421538105));
#43048=CARTESIAN_POINT('Ctrl Pts',(-0.220520438475924,0.00173372995230389,
-0.00862406799262633));
#43049=CARTESIAN_POINT('Ctrl Pts',(-0.22052056788612,0.0017336078325201,
-0.0086239708361658));
#43050=CARTESIAN_POINT('Ctrl Pts',(-0.220520758525357,0.00173330231663648,
-0.00862372404872762));
#43051=CARTESIAN_POINT('Ctrl Pts',(-0.219148515071371,0.00691048297255687,
-0.0105396975990103));
#43052=CARTESIAN_POINT('Ctrl Pts',(-0.219147356380851,0.00690322974884955,
-0.0106487703174557));
#43053=CARTESIAN_POINT('Ctrl Pts',(-0.219038955168735,0.00689487685220507,
-0.010637242672756));
#43054=CARTESIAN_POINT('Ctrl Pts',(-0.219036137036226,0.00807747716428064,
-0.0106153242780037));
#43055=CARTESIAN_POINT('Ctrl Pts',(-0.219034955335834,0.00808468304500183,
-0.0107253460856709));
#43056=CARTESIAN_POINT('Ctrl Pts',(-0.218926799334561,0.00807242090324395,
-0.0107151659237768));
#43057=CARTESIAN_POINT('Ctrl Pts',(-0.218905132240887,0.00977915705389375,
-0.0103918892388122));
#43058=CARTESIAN_POINT('Ctrl Pts',(-0.218904029998625,0.00980665680374094,
-0.0104992708126475));
#43059=CARTESIAN_POINT('Ctrl Pts',(-0.218794734263875,0.0098026290016253,
-0.0104909783450489));
#43060=CARTESIAN_POINT('Ctrl Pts',(-0.219071089153358,0.0119671367922082,
-0.00943613238649878));
#43061=CARTESIAN_POINT('Ctrl Pts',(-0.219070437343078,0.0120216325715906,
-0.00953173065297142));
#43062=CARTESIAN_POINT('Ctrl Pts',(-0.218962442721151,0.0120305426252144,
-0.00951571104175434));
#43063=CARTESIAN_POINT('Ctrl Pts',(-0.21932523698136,0.0129089558008521,
-0.00878419964750562));
#43064=CARTESIAN_POINT('Ctrl Pts',(-0.21932487961028,0.0129746248050434,
-0.00887199152970325));
#43065=CARTESIAN_POINT('Ctrl Pts',(-0.219218564468832,0.0129875068392683,
-0.00884975676863126));
#43066=CARTESIAN_POINT('Ctrl Pts',(-0.219454102120046,0.0134244664873124,
-0.00833869489519783));
#43067=CARTESIAN_POINT('Ctrl Pts',(-0.21945392109255,0.0134964707033814,
-0.00842100564533139));
#43068=CARTESIAN_POINT('Ctrl Pts',(-0.219346826781403,0.0135047144980998,
-0.00840040661615055));
#43069=CARTESIAN_POINT('Ctrl Pts',(-0.219093941307367,0.00750191211356895,
-0.0105597759983895));
#43070=CARTESIAN_POINT('Ctrl Pts',(-0.219093767460342,0.00750191339671021,
-0.0105661672114314));
#43071=CARTESIAN_POINT('Ctrl Pts',(-0.219092978750846,0.00750191452875406,
-0.0105725269115254));
#43072=CARTESIAN_POINT('Ctrl Pts',(-0.219090069650718,0.0075019165336753,
-0.0105855632853716));
#43073=CARTESIAN_POINT('Ctrl Pts',(-0.219087845371762,0.00750191736905565,
-0.010592180920131));
#43074=CARTESIAN_POINT('Ctrl Pts',(-0.219079594227124,0.00750191908697261,
-0.0106102290130474));
#43075=CARTESIAN_POINT('Ctrl Pts',(-0.219072020861462,0.00750191940049146,
-0.0106207966092312));
#43076=CARTESIAN_POINT('Ctrl Pts',(-0.219053282710123,0.00750191812597504,
-0.010638488913879));
#43077=CARTESIAN_POINT('Ctrl Pts',(-0.219042291643416,0.0075019166823333,
-0.0106454469725408));
#43078=CARTESIAN_POINT('Ctrl Pts',(-0.21901994966729,0.00750191087528336,
-0.0106541838284163));
#43079=CARTESIAN_POINT('Ctrl Pts',(-0.21900904021347,0.00750192874869014,
-0.0106564768272035));
#43080=CARTESIAN_POINT('Ctrl Pts',(-0.218995822383935,0.00750187995871182,
-0.0106570539596742));
#43081=CARTESIAN_POINT('Ctrl Pts',(-0.218993530792735,0.00750190999230115,
-0.0106570779154422));
#43082=CARTESIAN_POINT('Ctrl Pts',(-0.218991340185995,0.00750190949851256,
-0.0106570284103405));
#43083=CARTESIAN_POINT('Ctrl Pts',(-0.220657718078581,0.0018751479361439,
-0.00861162539660087));
#43084=CARTESIAN_POINT('Ctrl Pts',(-0.220656233896277,0.00181097856082264,
-0.00869193835890256));
#43085=CARTESIAN_POINT('Ctrl Pts',(-0.220658316110286,0.00173232387629273,
-0.00862547314886965));
#43086=CARTESIAN_POINT('Ctrl Pts',(-0.22038644554275,0.00187704155792308,
-0.00860803515775927));
#43087=CARTESIAN_POINT('Ctrl Pts',(-0.220384869594419,0.00181290856447447,
-0.00868834779106167));
#43088=CARTESIAN_POINT('Ctrl Pts',(-0.220387269569338,0.00173488744681977,
-0.0086225160123027));
#43089=CARTESIAN_POINT('Ctrl Pts',(-0.220000575954751,0.00185543408637361,
-0.00858349740986387));
#43090=CARTESIAN_POINT('Ctrl Pts',(-0.219999192384961,0.001791130697238,
-0.00866379310111029));
#43091=CARTESIAN_POINT('Ctrl Pts',(-0.220002878180249,0.00171042904111559,
-0.00859532149219416));
#43092=CARTESIAN_POINT('Ctrl Pts',(-0.219511028165309,0.00195343846120863,
-0.00865283203789838));
#43093=CARTESIAN_POINT('Ctrl Pts',(-0.219510389522585,0.00189013343318333,
-0.00873358372156444));
#43094=CARTESIAN_POINT('Ctrl Pts',(-0.21946299979619,0.00181705681249047,
-0.00867264489778598));
#43095=CARTESIAN_POINT('Ctrl Pts',(-0.21933003719857,0.00208585294127225,
-0.00875179762193781));
#43096=CARTESIAN_POINT('Ctrl Pts',(-0.219329139091007,0.00202413227238718,
-0.0088332651959512));
#43097=CARTESIAN_POINT('Ctrl Pts',(-0.219257176298931,0.00196751447944682,
-0.00878690909359569));
#43098=CARTESIAN_POINT('Ctrl Pts',(-0.219194504687458,0.00217281033445456,
-0.00881277285849614));
#43099=CARTESIAN_POINT('Ctrl Pts',(-0.219193456552492,0.00211219507604886,
-0.00889529739755567));
#43100=CARTESIAN_POINT('Ctrl Pts',(-0.219134455871745,0.0020464823948761,
-0.00884311272090225));
#43101=CARTESIAN_POINT('Ctrl Pts',(-0.219334416590634,0.00208138222259607,
-0.00874824491983627));
#43102=CARTESIAN_POINT('Ctrl Pts',(-0.219334320063737,0.00207729391397082,
-0.00875360873145552));
#43103=CARTESIAN_POINT('Ctrl Pts',(-0.219333604008012,0.0020729254234734,
-0.00875871456669258));
#43104=CARTESIAN_POINT('Ctrl Pts',(-0.219330873127534,0.00206344571171821,
-0.00876859253859587));
#43105=CARTESIAN_POINT('Ctrl Pts',(-0.21932878304817,0.0020583446652351,
-0.00877327424185474));
#43106=CARTESIAN_POINT('Ctrl Pts',(-0.219321082227192,0.00204357506471506,
-0.00878514705354778));
#43107=CARTESIAN_POINT('Ctrl Pts',(-0.219314085814434,0.00203382895482756,
-0.00879102793417479));
#43108=CARTESIAN_POINT('Ctrl Pts',(-0.219296933162624,0.00201489256784713,
-0.00879883654619196));
#43109=CARTESIAN_POINT('Ctrl Pts',(-0.219286886376862,0.00200588731369565,
-0.00880062956795521));
#43110=CARTESIAN_POINT('Ctrl Pts',(-0.219267063004303,0.00199122629751845,
-0.00880003617161851));
#43111=CARTESIAN_POINT('Ctrl Pts',(-0.219257585685345,0.00198532728737071,
-0.00879831194460528));
#43112=CARTESIAN_POINT('Ctrl Pts',(-0.219246107062773,0.00197933492943865,
-0.0087945788756421));
#43113=CARTESIAN_POINT('Ctrl Pts',(-0.219244027871131,0.00197832881338241,
-0.00879386553455533));
#43114=CARTESIAN_POINT('Ctrl Pts',(-0.219242032666924,0.00197738200797957,
-0.00879310436763141));
#43115=CARTESIAN_POINT('Ctrl Pts',(-0.219456692804946,0.00160111516560854,
-0.00836091035860459));
#43116=CARTESIAN_POINT('Ctrl Pts',(-0.219456067988,0.00152938117372744,
-0.00844342455429431));
#43117=CARTESIAN_POINT('Ctrl Pts',(-0.21934905497045,0.00152127094901417,
-0.00842244164486835));
#43118=CARTESIAN_POINT('Ctrl Pts',(-0.219328501201104,0.00210658569623933,
-0.00879635302666999));
#43119=CARTESIAN_POINT('Ctrl Pts',(-0.219327710138628,0.0020410357238593,
-0.00888421377064837));
#43120=CARTESIAN_POINT('Ctrl Pts',(-0.219221528779172,0.00202801777676731,
-0.00886143697198539));
#43121=CARTESIAN_POINT('Ctrl Pts',(-0.219071052564132,0.00305712341290254,
-0.00945029735204128));
#43122=CARTESIAN_POINT('Ctrl Pts',(-0.219069957508154,0.00300287510524064,
-0.00954601666865521));
#43123=CARTESIAN_POINT('Ctrl Pts',(-0.218961981689591,0.00299433920943247,
-0.00952977548234196));
#43124=CARTESIAN_POINT('Ctrl Pts',(-0.21890924160936,0.00523430232329638,
-0.0103936309275109));
#43125=CARTESIAN_POINT('Ctrl Pts',(-0.218907695683505,0.00520698605406793,
-0.0105010210078774));
#43126=CARTESIAN_POINT('Ctrl Pts',(-0.218798486649354,0.00521092820910359,
-0.0104921956534221));
#43127=CARTESIAN_POINT('Ctrl Pts',(-0.219035732064863,0.00692495059794331,
-0.0106157551916045));
#43128=CARTESIAN_POINT('Ctrl Pts',(-0.219034112291182,0.0069178206797144,
-0.0107257579164001));
#43129=CARTESIAN_POINT('Ctrl Pts',(-0.218926003176411,0.00693008662460253,
-0.0107151679806557));
#43130=CARTESIAN_POINT('Ctrl Pts',(-0.21914839349402,0.00809331137238897,
-0.0105399211052043));
#43131=CARTESIAN_POINT('Ctrl Pts',(-0.219146795855022,0.00810064627671322,
-0.0106489679471506));
#43132=CARTESIAN_POINT('Ctrl Pts',(-0.219038451062826,0.00810890497429706,
-0.0106370139428235));
#43133=CARTESIAN_POINT('Ctrl Pts',(-0.218366734177772,0.0131720326746961,
-0.00853098609508188));
#43134=CARTESIAN_POINT('Ctrl Pts',(-0.218364368788007,0.0132365740471837,
-0.0086106656298705));
#43135=CARTESIAN_POINT('Ctrl Pts',(-0.218465622250289,0.0132237145107785,
-0.00862087933247721));
#43136=CARTESIAN_POINT('Ctrl Pts',(-0.218264676471441,0.0126816728273647,
-0.00892565173193766));
#43137=CARTESIAN_POINT('Ctrl Pts',(-0.218262150148847,0.0127406029499428,
-0.00900985123627725));
#43138=CARTESIAN_POINT('Ctrl Pts',(-0.218362864026326,0.0127246548055583,
-0.00902087117030197));
#43139=CARTESIAN_POINT('Ctrl Pts',(-0.218046218879305,0.011755491836367,
-0.00952662103886202));
#43140=CARTESIAN_POINT('Ctrl Pts',(-0.218043459768016,0.0118040969683048,
-0.00961757890671437));
#43141=CARTESIAN_POINT('Ctrl Pts',(-0.218145341696559,0.0117918242380693,
-0.00962344777185459));
#43142=CARTESIAN_POINT('Ctrl Pts',(-0.21791304015827,0.00964780445850701,
-0.0103903848894813));
#43143=CARTESIAN_POINT('Ctrl Pts',(-0.217909924561879,0.00967207053712899,
-0.0104913089502273));
#43144=CARTESIAN_POINT('Ctrl Pts',(-0.218012908881215,0.00967428276848505,
-0.0104896633779764));
#43145=CARTESIAN_POINT('Ctrl Pts',(-0.218040716494051,0.00803350871449782,
-0.0105873246231014));
#43146=CARTESIAN_POINT('Ctrl Pts',(-0.218037511620459,0.00803976883496589,
-0.0106904112618394));
#43147=CARTESIAN_POINT('Ctrl Pts',(-0.218139463091569,0.00805065232707797,
-0.0106903621342042));
#43148=CARTESIAN_POINT('Ctrl Pts',(-0.218146767290287,0.00693520855091888,
-0.0105189682128489));
#43149=CARTESIAN_POINT('Ctrl Pts',(-0.218143588420993,0.00692870570122577,
-0.0106212622622081));
#43150=CARTESIAN_POINT('Ctrl Pts',(-0.218245775367947,0.00693731273779504,
-0.010622470145281));
#43151=CARTESIAN_POINT('Ctrl Pts',(-0.218192328823198,0.00750145352954351,
-0.0106389704498565));
#43152=CARTESIAN_POINT('Ctrl Pts',(-0.2181543005054,0.00750020162177904,
-0.0106381076224975));
#43153=CARTESIAN_POINT('Ctrl Pts',(-0.218121876716844,0.00749892202213666,
-0.0106133962756449));
#43154=CARTESIAN_POINT('Ctrl Pts',(-0.218107640280115,0.00749903957930803,
-0.0105885851589611));
#43155=CARTESIAN_POINT('Ctrl Pts',(-0.218097198595685,0.00749912580136693,
-0.0105703874978662));
#43156=CARTESIAN_POINT('Ctrl Pts',(-0.218094029014762,0.00749974391570192,
-0.0105524213574574));
#43157=CARTESIAN_POINT('Ctrl Pts',(-0.218094302309927,0.00750066584756617,
-0.0105367248189618));
#43158=CARTESIAN_POINT('Ctrl Pts',(-0.218256492401995,0.012654359922174,
-0.00892058569152569));
#43159=CARTESIAN_POINT('Ctrl Pts',(-0.218256481075259,0.0126585238231222,
-0.00892637097765501));
#43160=CARTESIAN_POINT('Ctrl Pts',(-0.218257350196721,0.0126631391930071,
-0.00893172184708259));
#43161=CARTESIAN_POINT('Ctrl Pts',(-0.218261001203897,0.0126739431288319,
-0.00894229936358914));
#43162=CARTESIAN_POINT('Ctrl Pts',(-0.218264045113842,0.0126801169194239,
-0.00894718999230209));
#43163=CARTESIAN_POINT('Ctrl Pts',(-0.218274189130881,0.0126966972458564,
-0.00895796495222554));
#43164=CARTESIAN_POINT('Ctrl Pts',(-0.21828289381032,0.0127077179240462,
-0.00896277666495482));
#43165=CARTESIAN_POINT('Ctrl Pts',(-0.218303764735828,0.0127295276295352,
-0.00896800026065576));
#43166=CARTESIAN_POINT('Ctrl Pts',(-0.218315084933949,0.0127396308911177,
-0.00896847361115103));
#43167=CARTESIAN_POINT('Ctrl Pts',(-0.218338385874436,0.0127579969737962,
-0.00896614627596395));
#43168=CARTESIAN_POINT('Ctrl Pts',(-0.218350528380616,0.0127663971078985,
-0.0089633590109566));
#43169=CARTESIAN_POINT('Ctrl Pts',(-0.218365200384923,0.0127753616348796,
-0.00895831830330567));
#43170=CARTESIAN_POINT('Ctrl Pts',(-0.2183677753286,0.0127768749342853,
-0.00895738426770429));
#43171=CARTESIAN_POINT('Ctrl Pts',(-0.21837031549238,0.0127783363881555,
-0.00895639440167604));
#43172=CARTESIAN_POINT('Ctrl Pts',(-0.217040091656276,0.012403843259427,
-0.00906292069881238));
#43173=CARTESIAN_POINT('Ctrl Pts',(-0.217038761654309,0.0124598798457787,
-0.00914919008978224));
#43174=CARTESIAN_POINT('Ctrl Pts',(-0.216999104629513,0.012537682949266,
-0.00909454615819164));
#43175=CARTESIAN_POINT('Ctrl Pts',(-0.217281733864375,0.0124892414562469,
-0.00901276450047278));
#43176=CARTESIAN_POINT('Ctrl Pts',(-0.217280397845029,0.0125462736073253,
-0.00909836481671279));
#43177=CARTESIAN_POINT('Ctrl Pts',(-0.217239846774433,0.0126225707764438,
-0.00904344449318198));
#43178=CARTESIAN_POINT('Ctrl Pts',(-0.217615520035054,0.0126222176898706,
-0.0089287395813754));
#43179=CARTESIAN_POINT('Ctrl Pts',(-0.217614512072917,0.0126808196249854,
-0.00901335824389992));
#43180=CARTESIAN_POINT('Ctrl Pts',(-0.21757524696877,0.0127590442565254,
-0.00895505101893103));
#43181=CARTESIAN_POINT('Ctrl Pts',(-0.218095966824174,0.012688547985487,
-0.00889135063154049));
#43182=CARTESIAN_POINT('Ctrl Pts',(-0.218094341784189,0.0127478797061336,
-0.00897567723691454));
#43183=CARTESIAN_POINT('Ctrl Pts',(-0.218097022661123,0.0128322256816752,
-0.00891246103404046));
#43184=CARTESIAN_POINT('Ctrl Pts',(-0.218326482347675,0.0126415268496617,
-0.0089289208830992));
#43185=CARTESIAN_POINT('Ctrl Pts',(-0.218324514240548,0.0127003721197212,
-0.00901344065888466));
#43186=CARTESIAN_POINT('Ctrl Pts',(-0.218351703750586,0.0127806085914963,
-0.00895449084106678));
#43187=CARTESIAN_POINT('Ctrl Pts',(-0.218486740291147,0.0126204219818312,
-0.00894655101177062));
#43188=CARTESIAN_POINT('Ctrl Pts',(-0.21848498462662,0.0126790186976341,
-0.00903130724294094));
#43189=CARTESIAN_POINT('Ctrl Pts',(-0.218499591342393,0.0127613749089422,
-0.00897089160770076));
#43190=CARTESIAN_POINT('Ctrl Pts',(-0.217213461658688,0.0124664448294026,
-0.0090260632281852));
#43191=CARTESIAN_POINT('Ctrl Pts',(-0.21721334964017,0.0124703852687589,
-0.00903197163158273));
#43192=CARTESIAN_POINT('Ctrl Pts',(-0.217212551997362,0.0124747370879997,
-0.00903753852187564));
#43193=CARTESIAN_POINT('Ctrl Pts',(-0.217209524833361,0.0124844786784638,
-0.0090482314753298));
#43194=CARTESIAN_POINT('Ctrl Pts',(-0.217207205691832,0.0124898587949991,
-0.00905321498766304));
#43195=CARTESIAN_POINT('Ctrl Pts',(-0.217198995661428,0.0125052463498904,
-0.00906521834175148));
#43196=CARTESIAN_POINT('Ctrl Pts',(-0.217191850065853,0.0125154539764049,
-0.00907075651121354));
#43197=CARTESIAN_POINT('Ctrl Pts',(-0.217174446413349,0.0125361395163697,
-0.00907780358828333));
#43198=CARTESIAN_POINT('Ctrl Pts',(-0.217164146319917,0.01254643804596,
-0.00907897566944418));
#43199=CARTESIAN_POINT('Ctrl Pts',(-0.217144783322987,0.0125631339420775,
-0.0090770720803645));
#43200=CARTESIAN_POINT('Ctrl Pts',(-0.217135986280563,0.0125698791697788,
-0.00907488480431806));
#43201=CARTESIAN_POINT('Ctrl Pts',(-0.217125162398161,0.0125771752050296,
-0.00907073982030332));
#43202=CARTESIAN_POINT('Ctrl Pts',(-0.217123134210988,0.0125785287737803,
-0.00906988376298916));
#43203=CARTESIAN_POINT('Ctrl Pts',(-0.217121145625652,0.0125797949708599,
-0.00906899621093816));
#43204=CARTESIAN_POINT('Origin',(-0.221715499787086,0.00708341181933542,
-0.00318613591211986));
#43205=CARTESIAN_POINT('Ctrl Pts',(-0.218253133205786,0.00235141097830992,
-0.0089245544184659));
#43206=CARTESIAN_POINT('Ctrl Pts',(-0.218253410928626,0.00234810267626737,
-0.00892913201349592));
#43207=CARTESIAN_POINT('Ctrl Pts',(-0.218254239150138,0.00234445216715201,
-0.00893336289573748));
#43208=CARTESIAN_POINT('Ctrl Pts',(-0.218257213663284,0.00233570235473179,
-0.00894198142806612));
#43209=CARTESIAN_POINT('Ctrl Pts',(-0.218259582821079,0.00233056670380563,
-0.00894608123347948));
#43210=CARTESIAN_POINT('Ctrl Pts',(-0.218268103529493,0.00231517587711936,
-0.00895624950748682));
#43211=CARTESIAN_POINT('Ctrl Pts',(-0.218276029056875,0.0023039815039752,
-0.00896105351889245));
#43212=CARTESIAN_POINT('Ctrl Pts',(-0.218298885248443,0.00227709004331209,
-0.00896741642455435));
#43213=CARTESIAN_POINT('Ctrl Pts',(-0.218313668431264,0.00226278335865085,
-0.00896712995333946));
#43214=CARTESIAN_POINT('Ctrl Pts',(-0.218339073783571,0.00224206387255127,
-0.00896359231248858));
#43215=CARTESIAN_POINT('Ctrl Pts',(-0.218349354969513,0.00223499767086404,
-0.00896112793673578));
#43216=CARTESIAN_POINT('Ctrl Pts',(-0.218361577669561,0.00222939301302785,
-0.00895902039524703));
#43217=CARTESIAN_POINT('Ctrl Pts',(-0.218364773986022,0.00222841493280178,
-0.00895862510642795));
#43218=CARTESIAN_POINT('Ctrl Pts',(-0.218368303205535,0.00222784554213887,
-0.008958425171701));
#43219=CARTESIAN_POINT('Ctrl Pts',(-0.218368983786652,0.00222776219852354,
-0.00895839830988281));
#43220=CARTESIAN_POINT('Ctrl Pts',(-0.218370051622135,0.00222767735278557,
-0.00895837687448052));
#43221=CARTESIAN_POINT('Ctrl Pts',(-0.218370435101234,0.00222765604199265,
-0.0089583733051086));
#43222=CARTESIAN_POINT('Ctrl Pts',(-0.218370898995356,0.00222764180170897,
-0.00895837421103516));
#43223=CARTESIAN_POINT('Ctrl Pts',(-0.218370978719185,0.00222763976512466,
-0.00895837455258704));
#43224=CARTESIAN_POINT('Ctrl Pts',(-0.218371097454342,0.00222763734785523,
-0.00895837534004206));
#43225=CARTESIAN_POINT('Ctrl Pts',(-0.218371136455611,0.00222763665277974,
-0.00895837564347949));
#43226=CARTESIAN_POINT('Ctrl Pts',(-0.218371194729898,0.00222763576250506,
-0.00895837616398511));
#43227=CARTESIAN_POINT('Ctrl Pts',(-0.21837121400151,0.00222763549231493,
-0.00895837634708607));
#43228=CARTESIAN_POINT('Ctrl Pts',(-0.21837157020395,0.00222763094680333,
-0.00895837993439936));
#43229=CARTESIAN_POINT('Ctrl Pts',(-0.218371906861464,0.00222763406685814,
-0.00895838668294486));
#43230=CARTESIAN_POINT('Ctrl Pts',(-0.21837272401761,0.00222766001051709,
-0.00895841136466877));
#43231=CARTESIAN_POINT('Ctrl Pts',(-0.218373202789348,0.00222769062793541,
-0.00895843279476503));
#43232=CARTESIAN_POINT('Ctrl Pts',(-0.218374162278603,0.00222778845837024,
-0.00895849206198491));
#43233=CARTESIAN_POINT('Ctrl Pts',(-0.217137975046077,0.00696793545844773,
-0.010498682606056));
#43234=CARTESIAN_POINT('Ctrl Pts',(-0.217136098788072,0.00696139686822146,
-0.0106072154889929));
#43235=CARTESIAN_POINT('Ctrl Pts',(-0.217028226897065,0.00695342027943268,
-0.0105957515286141));
#43236=CARTESIAN_POINT('Ctrl Pts',(-0.217053838228916,0.00803642449059388,
-0.0105608338666006));
#43237=CARTESIAN_POINT('Ctrl Pts',(-0.217051942792171,0.00804295377515252,
-0.0106701621405877));
#43238=CARTESIAN_POINT('Ctrl Pts',(-0.216944315818264,0.00803207665662111,
-0.0106595760977952));
#43239=CARTESIAN_POINT('Ctrl Pts',(-0.216834062029484,0.0101942506675489,
-0.0102951033665484));
#43240=CARTESIAN_POINT('Ctrl Pts',(-0.216832278499687,0.0102265108470005,
-0.0104012659729614));
#43241=CARTESIAN_POINT('Ctrl Pts',(-0.216723046287982,0.0102229255069439,
-0.0103943346079308));
#43242=CARTESIAN_POINT('Ctrl Pts',(-0.217139620528726,0.0121082417373667,
-0.00931994380391762));
#43243=CARTESIAN_POINT('Ctrl Pts',(-0.217138290003539,0.0121639970902703,
-0.00941421194997972));
#43244=CARTESIAN_POINT('Ctrl Pts',(-0.217031554121602,0.0121751503709153,
-0.00939571084227512));
#43245=CARTESIAN_POINT('Ctrl Pts',(-0.217302514187605,0.0129451438661898,
-0.00868850801833797));
#43246=CARTESIAN_POINT('Ctrl Pts',(-0.21730144433856,0.0130107637348759,
-0.0087752130077434));
#43247=CARTESIAN_POINT('Ctrl Pts',(-0.217194260965553,0.0130166427226768,
-0.00875779847180095));
#43248=CARTESIAN_POINT('Ctrl Pts',(-0.217094602028452,0.00750113053183012,
-0.0105144286534109));
#43249=CARTESIAN_POINT('Ctrl Pts',(-0.217094437212978,0.00750113150038833,
-0.0105208711260764));
#43250=CARTESIAN_POINT('Ctrl Pts',(-0.217093647894512,0.0075011323107023,
-0.0105272823912877));
#43251=CARTESIAN_POINT('Ctrl Pts',(-0.217090730637772,0.00750113367523198,
-0.0105403653760066));
#43252=CARTESIAN_POINT('Ctrl Pts',(-0.217088509145498,0.00750113419953919,
-0.0105469802676839));
#43253=CARTESIAN_POINT('Ctrl Pts',(-0.217080266267631,0.00750113521677092,
-0.0105650259084567));
#43254=CARTESIAN_POINT('Ctrl Pts',(-0.217072698383241,0.00750113526272342,
-0.0105755947798971));
#43255=CARTESIAN_POINT('Ctrl Pts',(-0.217053971209092,0.00750113485315194,
-0.0105932906477769));
#43256=CARTESIAN_POINT('Ctrl Pts',(-0.217042985779792,0.0075011340222172,
-0.0106002512537286));
#43257=CARTESIAN_POINT('Ctrl Pts',(-0.217017963698496,0.00750113668349459,
-0.0106100456301875));
#43258=CARTESIAN_POINT('Ctrl Pts',(-0.217006490540518,0.00750110816344995,
-0.0106114329679777));
#43259=CARTESIAN_POINT('Ctrl Pts',(-0.216997738159605,0.00750119231094314,
-0.0106118147301237));
#43260=CARTESIAN_POINT('Ctrl Pts',(-0.216995365374494,0.00750115899475884,
-0.0106118866829067));
#43261=CARTESIAN_POINT('Ctrl Pts',(-0.216992999839987,0.00750111626434787,
-0.0106118648816169));
#43262=CARTESIAN_POINT('Ctrl Pts',(-0.216992039095986,0.00750111592075218,
-0.0106118432044358));
#43263=CARTESIAN_POINT('Ctrl Pts',(-0.218512610680756,0.00234799200238128,
-0.00892513212683489));
#43264=CARTESIAN_POINT('Ctrl Pts',(-0.218510961166635,0.00228569700038617,
-0.00901443661716485));
#43265=CARTESIAN_POINT('Ctrl Pts',(-0.218510479461922,0.00220162766540384,
-0.00894450423745255));
#43266=CARTESIAN_POINT('Ctrl Pts',(-0.218253521679468,0.00235591056916128,
-0.00892562091397768));
#43267=CARTESIAN_POINT('Ctrl Pts',(-0.218251625806045,0.00229376201742538,
-0.00901496892835533));
#43268=CARTESIAN_POINT('Ctrl Pts',(-0.218250013232297,0.0022113668624948,
-0.00894636662237075));
#43269=CARTESIAN_POINT('Ctrl Pts',(-0.217710461308748,0.00233840441957516,
-0.00890257715584968));
#43270=CARTESIAN_POINT('Ctrl Pts',(-0.217709301310539,0.00227593220586861,
-0.00899202305588306));
#43271=CARTESIAN_POINT('Ctrl Pts',(-0.217717598087536,0.00218340813805773,
-0.00891627557236298));
#43272=CARTESIAN_POINT('Ctrl Pts',(-0.217289578618135,0.00247969338690751,
-0.008992986854597));
#43273=CARTESIAN_POINT('Ctrl Pts',(-0.217288486176955,0.00241901651396548,
-0.00908277776569406));
#43274=CARTESIAN_POINT('Ctrl Pts',(-0.217215756044667,0.00235437055333393,
-0.00902768579769387));
#43275=CARTESIAN_POINT('Ctrl Pts',(-0.217070832594413,0.00262754346735014,
-0.00908405008417822));
#43276=CARTESIAN_POINT('Ctrl Pts',(-0.21706937681227,0.00256874785681079,
-0.00917523660469239));
#43277=CARTESIAN_POINT('Ctrl Pts',(-0.217012813213666,0.00249727254229426,
-0.00911768489661139));
#43278=CARTESIAN_POINT('Ctrl Pts',(-0.217217202596967,0.0025390925417853,
-0.00902979181142551));
#43279=CARTESIAN_POINT('Ctrl Pts',(-0.217217093433627,0.00253527919148381,
-0.00903552446223438));
#43280=CARTESIAN_POINT('Ctrl Pts',(-0.217216329286209,0.00253113398466886,
-0.00904098318928687));
#43281=CARTESIAN_POINT('Ctrl Pts',(-0.217213429525352,0.0025219928280744,
-0.00905156722422215));
#43282=CARTESIAN_POINT('Ctrl Pts',(-0.217211212022842,0.00251700491423114,
-0.009056582169978));
#43283=CARTESIAN_POINT('Ctrl Pts',(-0.217203165994395,0.00250257048297124,
-0.00906915389328079));
#43284=CARTESIAN_POINT('Ctrl Pts',(-0.217195977250999,0.00249296457500099,
-0.0090753340588464));
#43285=CARTESIAN_POINT('Ctrl Pts',(-0.21717841474632,0.00247391188454135,
-0.00908372182048253));
#43286=CARTESIAN_POINT('Ctrl Pts',(-0.217168087826125,0.00246464189341527,
-0.0090857168567731));
#43287=CARTESIAN_POINT('Ctrl Pts',(-0.217148131929838,0.00244954809164539,
-0.00908536881790682));
#43288=CARTESIAN_POINT('Ctrl Pts',(-0.217138815370543,0.0024434373481414,
-0.00908379239471274));
#43289=CARTESIAN_POINT('Ctrl Pts',(-0.217127386079639,0.00243704830970052,
-0.00908029240560058));
#43290=CARTESIAN_POINT('Ctrl Pts',(-0.21712532989568,0.00243592263217277,
-0.00907959027446985));
#43291=CARTESIAN_POINT('Ctrl Pts',(-0.217123295418768,0.00243486422508496,
-0.00907884373636323));
#43292=CARTESIAN_POINT('Ctrl Pts',(-0.217305590590327,0.00206475955975603,
-0.00869612615818939));
#43293=CARTESIAN_POINT('Ctrl Pts',(-0.217304725296217,0.00199931848412992,
-0.00878289128905937));
#43294=CARTESIAN_POINT('Ctrl Pts',(-0.217197584750829,0.00199323238160935,
-0.00876569203822327));
#43295=CARTESIAN_POINT('Ctrl Pts',(-0.217140314114961,0.00291363579254913,
-0.00933321669145991));
#43296=CARTESIAN_POINT('Ctrl Pts',(-0.217139184840844,0.002858204433682,
-0.00942760897514758));
#43297=CARTESIAN_POINT('Ctrl Pts',(-0.217032492189526,0.00284685187725704,
-0.00940936648213871));
#43298=CARTESIAN_POINT('Ctrl Pts',(-0.216837373073137,0.00481822843586069,
-0.010296613574004));
#43299=CARTESIAN_POINT('Ctrl Pts',(-0.216835800873413,0.00478613513583303,
-0.0104027295262049));
#43300=CARTESIAN_POINT('Ctrl Pts',(-0.216726609134844,0.00478956143554811,
-0.0103960267216009));
#43301=CARTESIAN_POINT('Ctrl Pts',(-0.217054377111761,0.00697128504474957,
-0.0105604810661386));
#43302=CARTESIAN_POINT('Ctrl Pts',(-0.217052690956768,0.00696483378685744,
-0.0106697439278292));
#43303=CARTESIAN_POINT('Ctrl Pts',(-0.216945096195469,0.00697563227639263,
-0.0106594296379724));
#43304=CARTESIAN_POINT('Ctrl Pts',(-0.217137406949296,0.00802996460581778,
-0.0104984600401621));
#43305=CARTESIAN_POINT('Ctrl Pts',(-0.217135740417579,0.00803645694558565,
-0.0106069320876849));
#43306=CARTESIAN_POINT('Ctrl Pts',(-0.21702790179751,0.00804439497834719,
-0.0105957520847982));
#43307=CARTESIAN_POINT('Ctrl Pts',(-0.216282845990138,0.0128929856408761,
-0.00870791588407719));
#43308=CARTESIAN_POINT('Ctrl Pts',(-0.21628054597117,0.0129542040883401,
-0.00879035739816422));
#43309=CARTESIAN_POINT('Ctrl Pts',(-0.216382357754694,0.0129431688471136,
-0.00879814483003904));
#43310=CARTESIAN_POINT('Ctrl Pts',(-0.216133718571471,0.012057373323281,
-0.00932799336983377));
#43311=CARTESIAN_POINT('Ctrl Pts',(-0.216131165247688,0.0121092546354352,
-0.00941743508173665));
#43312=CARTESIAN_POINT('Ctrl Pts',(-0.216232605411869,0.0120943919614193,
-0.00942553527241766));
#43313=CARTESIAN_POINT('Ctrl Pts',(-0.215835443717348,0.0101441471812373,
-0.0102857637590424));
#43314=CARTESIAN_POINT('Ctrl Pts',(-0.215832522774285,0.0101740039538028,
-0.0103861540384211));
#43315=CARTESIAN_POINT('Ctrl Pts',(-0.215936094441128,0.0101739288277866,
-0.0103832444006597));
#43316=CARTESIAN_POINT('Ctrl Pts',(-0.216055651587784,0.00800709561225113,
-0.0105372628493557));
#43317=CARTESIAN_POINT('Ctrl Pts',(-0.216052594542648,0.00801302128485416,
-0.0106404734829225));
#43318=CARTESIAN_POINT('Ctrl Pts',(-0.216154763548897,0.00802309106962762,
-0.0106402736064033));
#43319=CARTESIAN_POINT('Ctrl Pts',(-0.216139422648866,0.00696389597780172,
-0.0104755961789519));
#43320=CARTESIAN_POINT('Ctrl Pts',(-0.216136391047069,0.00695775334100502,
-0.0105780830921685));
#43321=CARTESIAN_POINT('Ctrl Pts',(-0.216238791290835,0.00696598534872043,
-0.0105788762726166));
#43322=CARTESIAN_POINT('Ctrl Pts',(-0.216094904650184,0.00750081531065442,
-0.0104915380007917));
#43323=CARTESIAN_POINT('Ctrl Pts',(-0.216094756795897,0.00750081620795364,
-0.0104980811404747));
#43324=CARTESIAN_POINT('Ctrl Pts',(-0.216095253916839,0.00750081722356874,
-0.0105046226317289));
#43325=CARTESIAN_POINT('Ctrl Pts',(-0.216097595249637,0.00750081955421988,
-0.0105179231430352));
#43326=CARTESIAN_POINT('Ctrl Pts',(-0.21609951640324,0.00750082087733701,
-0.0105246324342848));
#43327=CARTESIAN_POINT('Ctrl Pts',(-0.216106938011482,0.00750082498061469,
-0.0105430328719986));
#43328=CARTESIAN_POINT('Ctrl Pts',(-0.216114022367117,0.00750082798353315,
-0.0105539325807752));
#43329=CARTESIAN_POINT('Ctrl Pts',(-0.216131934369291,0.00750083480936225,
-0.0105724556140836));
#43330=CARTESIAN_POINT('Ctrl Pts',(-0.21614259590609,0.00750083832245985,
-0.0105799047757781));
#43331=CARTESIAN_POINT('Ctrl Pts',(-0.216167838768553,0.00750084939658654,
-0.0105911228479625));
#43332=CARTESIAN_POINT('Ctrl Pts',(-0.216179521428449,0.00750084106413271,
-0.0105928076172997));
#43333=CARTESIAN_POINT('Ctrl Pts',(-0.2161873624299,0.00750089292605126,
-0.0105935055836128));
#43334=CARTESIAN_POINT('Ctrl Pts',(-0.21618964357311,0.00750087208550254,
-0.0105936739646218));
#43335=CARTESIAN_POINT('Ctrl Pts',(-0.216191922147214,0.00750084456948937,
-0.0105937600086224));
#43336=CARTESIAN_POINT('Ctrl Pts',(-0.216192970650498,0.00750084471341908,
-0.0105937837104633));
#43337=CARTESIAN_POINT('Ctrl Pts',(-0.216191694510709,0.012362961460189,
-0.0090741750090641));
#43338=CARTESIAN_POINT('Ctrl Pts',(-0.216191822194119,0.0123768807643042,
-0.00909512604910344));
#43339=CARTESIAN_POINT('Ctrl Pts',(-0.216210230367078,0.012406465199571,
-0.00911336004700776));
#43340=CARTESIAN_POINT('Ctrl Pts',(-0.216228375424446,0.0124310958868995,
-0.0091172997600751));
#43341=CARTESIAN_POINT('Ctrl Pts',(-0.216230005813432,0.0124333090296043,
-0.00911765375536227));
#43342=CARTESIAN_POINT('Ctrl Pts',(-0.216231634734948,0.0124354692167458,
-0.00911792635430594));
#43343=CARTESIAN_POINT('Ctrl Pts',(-0.216233248932233,0.0124375588927111,
-0.00911812893263417));
#43344=CARTESIAN_POINT('Ctrl Pts',(-0.216251094709426,0.0124606613300867,
-0.00912036853974034));
#43345=CARTESIAN_POINT('Ctrl Pts',(-0.21626716337826,0.0124750802192241,
-0.00911813030457629));
#43346=CARTESIAN_POINT('Ctrl Pts',(-0.216295540195969,0.01249768233462,
-0.00910640980901082));
#43347=CARTESIAN_POINT('Ctrl Pts',(-0.216298702098623,0.0125002007878656,
-0.00910510384629096));
#43348=CARTESIAN_POINT('Ctrl Pts',(-0.216302017321607,0.0125028010528426,
-0.00910363126631569));
#43349=CARTESIAN_POINT('Ctrl Pts',(-0.216305506198624,0.0125054790081327,
-0.00910194677041158));
#43350=CARTESIAN_POINT('Origin',(-0.216343159043645,0.0124520636670066,
-0.00901812198471994));
#43351=CARTESIAN_POINT('Ctrl Pts',(-0.215095414441432,0.0124591460413101,
-0.00910819331956975));
#43352=CARTESIAN_POINT('Ctrl Pts',(-0.215120401030406,0.0124359848540545,
-0.00912362130480649));
#43353=CARTESIAN_POINT('Ctrl Pts',(-0.215133772132029,0.0124182892002308,
-0.00912603088362709));
#43354=CARTESIAN_POINT('Ctrl Pts',(-0.215148702658334,0.0123986783815203,
-0.00912385037729619));
#43355=CARTESIAN_POINT('Ctrl Pts',(-0.215150299639797,0.0123965807921044,
-0.0091236171485326));
#43356=CARTESIAN_POINT('Ctrl Pts',(-0.215151915486707,0.0123944349474128,
-0.00912329023287928));
#43357=CARTESIAN_POINT('Ctrl Pts',(-0.215153554980737,0.0123922157146173,
-0.00912285148268702));
#43358=CARTESIAN_POINT('Ctrl Pts',(-0.215170522460296,0.0123692483927538,
-0.00911831076172079));
#43359=CARTESIAN_POINT('Ctrl Pts',(-0.215184387550774,0.0123381808782917,
-0.00909998527609093));
#43360=CARTESIAN_POINT('Ctrl Pts',(-0.215184823658102,0.0123239090545933,
-0.00907757182940712));
#43361=CARTESIAN_POINT('Ctrl Pts',(-0.216139285036328,0.00803827977272542,
-0.0104749865165695));
#43362=CARTESIAN_POINT('Ctrl Pts',(-0.216135584338956,0.00804453914118892,
-0.0105781229455219));
#43363=CARTESIAN_POINT('Ctrl Pts',(-0.216238660816216,0.00803629527470715,
-0.0105788969339609));
#43364=CARTESIAN_POINT('Ctrl Pts',(-0.216055763094736,0.00699299166987041,
-0.0105363034745261));
#43365=CARTESIAN_POINT('Ctrl Pts',(-0.21605203840423,0.00698709339425489,
-0.0106401704688209));
#43366=CARTESIAN_POINT('Ctrl Pts',(-0.216154883042114,0.00697697631507577,
-0.0106399414472133));
#43367=CARTESIAN_POINT('Ctrl Pts',(-0.215836736738016,0.00486495828754412,
-0.0102881783975672));
#43368=CARTESIAN_POINT('Ctrl Pts',(-0.215833138858722,0.00483500982269961,
-0.010389261864091));
#43369=CARTESIAN_POINT('Ctrl Pts',(-0.215937390039039,0.00483525154752722,
-0.0103863545090138));
#43370=CARTESIAN_POINT('Ctrl Pts',(-0.216137707812793,0.00294240207909308,
-0.00932702833761163));
#43371=CARTESIAN_POINT('Ctrl Pts',(-0.216134494712672,0.00289008833417827,
-0.00941698370469411));
#43372=CARTESIAN_POINT('Ctrl Pts',(-0.216236595839286,0.00290507470426125,
-0.00942512670023606));
#43373=CARTESIAN_POINT('Ctrl Pts',(-0.216285909883727,0.00211376764744365,
-0.00871193737699649));
#43374=CARTESIAN_POINT('Ctrl Pts',(-0.216282947197694,0.00205216060863476,
-0.00879490657085487));
#43375=CARTESIAN_POINT('Ctrl Pts',(-0.216385423407197,0.00206332475774103,
-0.00880273997904361));
#43376=CARTESIAN_POINT('Ctrl Pts',(-0.216308829828652,0.00249826452155856,
-0.00910474619664736));
#43377=CARTESIAN_POINT('Ctrl Pts',(-0.216277540774277,0.00252224331941416,
-0.00911980910851503));
#43378=CARTESIAN_POINT('Ctrl Pts',(-0.216259966794798,0.00253762812048443,
-0.00912198916335422));
#43379=CARTESIAN_POINT('Ctrl Pts',(-0.216242133257728,0.00255926286473761,
-0.00912127524977043));
#43380=CARTESIAN_POINT('Ctrl Pts',(-0.216240281249037,0.00256150962791337,
-0.00912120111001024));
#43381=CARTESIAN_POINT('Ctrl Pts',(-0.216238426704362,0.00256383525815522,
-0.00912105340666394));
#43382=CARTESIAN_POINT('Ctrl Pts',(-0.216236553900389,0.00256625758763653,
-0.00912081190907445));
#43383=CARTESIAN_POINT('Ctrl Pts',(-0.216218499535794,0.00258960953490383,
-0.00911848380341484));
#43384=CARTESIAN_POINT('Ctrl Pts',(-0.216198685889085,0.00262068047583808,
-0.00910311875075495));
#43385=CARTESIAN_POINT('Ctrl Pts',(-0.216195457832998,0.00263678928674248,
-0.00908219213157078));
#43386=CARTESIAN_POINT('Ctrl Pts',(-0.216195172748967,0.00263821192768416,
-0.00908034400849087));
#43387=CARTESIAN_POINT('Ctrl Pts',(-0.216195017839807,0.00263953714974432,
-0.00907848253511195));
#43388=CARTESIAN_POINT('Ctrl Pts',(-0.216195006323166,0.00264076383020346,
-0.00907662663635085));
#43389=CARTESIAN_POINT('Ctrl Pts',(-0.215138268707419,0.00698344596248103,
-0.0104545905660588));
#43390=CARTESIAN_POINT('Ctrl Pts',(-0.215136339427148,0.00697718956481417,
-0.0105617541112084));
#43391=CARTESIAN_POINT('Ctrl Pts',(-0.21502973621825,0.0069690563131557,
-0.0105517156694489));
#43392=CARTESIAN_POINT('Ctrl Pts',(-0.215054198986798,0.00802081780291805,
-0.0105125259768653));
#43393=CARTESIAN_POINT('Ctrl Pts',(-0.215052252505421,0.00802704965957652,
-0.0106204194577288));
#43394=CARTESIAN_POINT('Ctrl Pts',(-0.214945873650048,0.00801615691193827,
-0.010611304630013));
#43395=CARTESIAN_POINT('Ctrl Pts',(-0.214841832736404,0.0101088263597614,
-0.0102648137814259));
#43396=CARTESIAN_POINT('Ctrl Pts',(-0.214839986037366,0.0101395482971445,
-0.0103698202132453));
#43397=CARTESIAN_POINT('Ctrl Pts',(-0.214732131678294,0.0101366736980693,
-0.0103638814523754));
#43398=CARTESIAN_POINT('Ctrl Pts',(-0.215123122693411,0.0119899129679057,
-0.00934455275222973));
#43399=CARTESIAN_POINT('Ctrl Pts',(-0.215121700939607,0.0120433858470247,
-0.00943849044895999));
#43400=CARTESIAN_POINT('Ctrl Pts',(-0.215015985777715,0.0120539646858002,
-0.00942223756738649));
#43401=CARTESIAN_POINT('Ctrl Pts',(-0.215268700133232,0.0128245611985155,
-0.00873920920956725));
#43402=CARTESIAN_POINT('Ctrl Pts',(-0.215267527785315,0.0128877157588611,
-0.00882601519127026));
#43403=CARTESIAN_POINT('Ctrl Pts',(-0.215161434357862,0.0128936434211584,
-0.00881066198364404));
#43404=CARTESIAN_POINT('Ctrl Pts',(-0.21509521040637,0.00750052117343929,
-0.0104691577567921));
#43405=CARTESIAN_POINT('Ctrl Pts',(-0.215095050257003,0.00750052168721324,
-0.0104756287762937));
#43406=CARTESIAN_POINT('Ctrl Pts',(-0.215094259973477,0.00750052209497991,
-0.0104820686809155));
#43407=CARTESIAN_POINT('Ctrl Pts',(-0.215091335823137,0.00750052273780868,
-0.0104951798602485));
#43408=CARTESIAN_POINT('Ctrl Pts',(-0.215089113650354,0.00750052295534443,
-0.0105017952878704));
#43409=CARTESIAN_POINT('Ctrl Pts',(-0.215080868589627,0.00750052329951441,
-0.0105198415751402));
#43410=CARTESIAN_POINT('Ctrl Pts',(-0.21507329908319,0.00750052316019882,
-0.0105304102155527));
#43411=CARTESIAN_POINT('Ctrl Pts',(-0.215054568613045,0.00750052282350388,
-0.0105481053155121));
#43412=CARTESIAN_POINT('Ctrl Pts',(-0.215043581478387,0.00750052228908468,
-0.0105550653082537));
#43413=CARTESIAN_POINT('Ctrl Pts',(-0.2150187109435,0.00750052547626067,
-0.0105647979495009));
#43414=CARTESIAN_POINT('Ctrl Pts',(-0.215007311554113,0.00750049889594075,
-0.0105662330298729));
#43415=CARTESIAN_POINT('Ctrl Pts',(-0.214998322630719,0.00750057650214591,
-0.010566627439243));
#43416=CARTESIAN_POINT('Ctrl Pts',(-0.214995979516134,0.00750054677270074,
-0.0105666968728011));
#43417=CARTESIAN_POINT('Ctrl Pts',(-0.214993635413369,0.00750050836006935,
-0.010566677172531));
#43418=CARTESIAN_POINT('Ctrl Pts',(-0.21499263918831,0.00750050820908203,
-0.0105666547606325));
#43419=CARTESIAN_POINT('Origin',(-0.215029774015556,0.00259990999948959,
-0.00902581867692437));
#43420=CARTESIAN_POINT('Ctrl Pts',(-0.215187397287789,0.00267846401374506,
-0.0090791176475646));
#43421=CARTESIAN_POINT('Ctrl Pts',(-0.21518696968744,0.00266415867860654,
-0.00910150656180909));
#43422=CARTESIAN_POINT('Ctrl Pts',(-0.215173125231804,0.00263299596606228,
-0.00911976224472072));
#43423=CARTESIAN_POINT('Ctrl Pts',(-0.215156200020307,0.00261007761913271,
-0.00912431726791484));
#43424=CARTESIAN_POINT('Ctrl Pts',(-0.215141017916609,0.00258951960603424,
-0.00912840317458063));
#43425=CARTESIAN_POINT('Ctrl Pts',(-0.215129066319246,0.00257341534231338,
-0.00912637292740067));
#43426=CARTESIAN_POINT('Ctrl Pts',(-0.215106261349755,0.00255100317834008,
-0.0091144188949001));
#43427=CARTESIAN_POINT('Ctrl Pts',(-0.215103643035173,0.00254842996306945,
-0.00911304641257252));
#43428=CARTESIAN_POINT('Ctrl Pts',(-0.21510089371507,0.0025458066359998,
-0.00911149443871825));
#43429=CARTESIAN_POINT('Ctrl Pts',(-0.21509802079524,0.00254314437078809,
-0.00910972203361875));
#43430=CARTESIAN_POINT('Ctrl Pts',(-0.215271626585773,0.00217581993097967,
-0.0087395861630685));
#43431=CARTESIAN_POINT('Ctrl Pts',(-0.215270612896943,0.00211272999214843,
-0.00882634758645658));
#43432=CARTESIAN_POINT('Ctrl Pts',(-0.215164580280835,0.00210664128134,
-0.00881118174408626));
#43433=CARTESIAN_POINT('Ctrl Pts',(-0.215125355803509,0.00301599520621347,
-0.00934778240909707));
#43434=CARTESIAN_POINT('Ctrl Pts',(-0.215124091178223,0.00296265152479492,
-0.00944170503104277));
#43435=CARTESIAN_POINT('Ctrl Pts',(-0.215018435808979,0.00295196260828074,
-0.00942567372829455));
#43436=CARTESIAN_POINT('Ctrl Pts',(-0.214843449546337,0.00488752405156655,
-0.0102630167362636));
#43437=CARTESIAN_POINT('Ctrl Pts',(-0.214841765608511,0.00485677866707993,
-0.0103679243946987));
#43438=CARTESIAN_POINT('Ctrl Pts',(-0.214733971784369,0.00485940615041609,
-0.0103621640961027));
#43439=CARTESIAN_POINT('Ctrl Pts',(-0.215054296090415,0.00698177131318153,
-0.0105127506298666));
#43440=CARTESIAN_POINT('Ctrl Pts',(-0.215052509277578,0.00697555952124977,
-0.0106205720293646));
#43441=CARTESIAN_POINT('Ctrl Pts',(-0.214946183406747,0.00698642042182544,
-0.0106117051843749));
#43442=CARTESIAN_POINT('Ctrl Pts',(-0.215138102089214,0.008016862224145,
-0.0104542932258017));
#43443=CARTESIAN_POINT('Ctrl Pts',(-0.215136333069552,0.00802310475840938,
-0.0105613805147221));
#43444=CARTESIAN_POINT('Ctrl Pts',(-0.21502978407555,0.00803120569858454,
-0.0105515845758995));
#43445=CARTESIAN_POINT('Ctrl Pts',(-0.1924290089395,0.0029155191620011,
-0.0087649001815275));
#43446=CARTESIAN_POINT('Ctrl Pts',(-0.192427813903335,0.00286412403846673,
-0.00885788426072911));
#43447=CARTESIAN_POINT('Ctrl Pts',(-0.192388140977693,0.00278108903612549,
-0.00880417838622631));
#43448=CARTESIAN_POINT('Ctrl Pts',(-0.192151357383384,0.00302045420861078,
-0.00881768715629337));
#43449=CARTESIAN_POINT('Ctrl Pts',(-0.192149891191152,0.00297037731033976,
-0.0089113558197304));
#43450=CARTESIAN_POINT('Ctrl Pts',(-0.192109318357643,0.0028883972306172,
-0.0088594852174804));
#43451=CARTESIAN_POINT('Ctrl Pts',(-0.191564370518527,0.00320957432995767,
-0.0089069598377226));
#43452=CARTESIAN_POINT('Ctrl Pts',(-0.19156378155172,0.00316120722641246,
-0.0090017598976799));
#43453=CARTESIAN_POINT('Ctrl Pts',(-0.191530402374114,0.00306724379457668,
-0.00894702953336356));
#43454=CARTESIAN_POINT('Ctrl Pts',(-0.191125263038703,0.0035084303185505,
-0.00904496669604534));
#43455=CARTESIAN_POINT('Ctrl Pts',(-0.191124237464691,0.00346354789673269,
-0.00914061051655912));
#43456=CARTESIAN_POINT('Ctrl Pts',(-0.191035800399296,0.00341041835692548,
-0.00910842868632399));
#43457=CARTESIAN_POINT('Ctrl Pts',(-0.190937017957496,0.0037465261723087,
-0.0091449485015039));
#43458=CARTESIAN_POINT('Ctrl Pts',(-0.190935691282421,0.00370453581711239,
-0.00924202969982603));
#43459=CARTESIAN_POINT('Ctrl Pts',(-0.190858333402855,0.00364208478676822,
-0.00920738829771903));
#43460=CARTESIAN_POINT('Ctrl Pts',(-0.190965502145366,0.00353026999546062,
-0.00915929064154693));
#43461=CARTESIAN_POINT('Ctrl Pts',(-0.190965605451063,0.00353079645007945,
-0.00915951112912086));
#43462=CARTESIAN_POINT('Ctrl Pts',(-0.190965733635172,0.00353130737617717,
-0.00915972129380536));
#43463=CARTESIAN_POINT('Ctrl Pts',(-0.190966490909549,0.00353376944855981,
-0.00916071300828134));
#43464=CARTESIAN_POINT('Ctrl Pts',(-0.190967482378507,0.00353551921344156,
-0.00916135128342715));
#43465=CARTESIAN_POINT('Ctrl Pts',(-0.190971146089304,0.0035400391972326,
-0.00916272934769088));
#43466=CARTESIAN_POINT('Ctrl Pts',(-0.190974269748778,0.00354238079049634,
-0.00916309172510267));
#43467=CARTESIAN_POINT('Ctrl Pts',(-0.19098337409412,0.00354882134562363,
-0.00916350304047491));
#43468=CARTESIAN_POINT('Ctrl Pts',(-0.190992994450311,0.00355431796352706,
-0.00916254541256994));
#43469=CARTESIAN_POINT('Ctrl Pts',(-0.191014214843227,0.00356811463625413,
-0.00915492575966953));
#43470=CARTESIAN_POINT('Ctrl Pts',(-0.191023999687439,0.00357530482732608,
-0.00914874127804869));
#43471=CARTESIAN_POINT('Ctrl Pts',(-0.191038764613866,0.00358848101622443,
-0.00913369118535732));
#43472=CARTESIAN_POINT('Ctrl Pts',(-0.191044168965102,0.00359437633404391,
-0.00912547730853556));
#43473=CARTESIAN_POINT('Ctrl Pts',(-0.191051371066627,0.00360489423478907,
-0.00910776989774631));
#43474=CARTESIAN_POINT('Ctrl Pts',(-0.191053379384272,0.00360949977795018,
-0.00909857985643356));
#43475=CARTESIAN_POINT('Ctrl Pts',(-0.191053878207127,0.00361347960381807,
-0.00908895687335754));
#43476=CARTESIAN_POINT('Ctrl Pts',(-0.192132462182123,0.00302309075119266,
-0.00882016247897886));
#43477=CARTESIAN_POINT('Ctrl Pts',(-0.192132442819634,0.00302125537502577,
-0.00882340434178846));
#43478=CARTESIAN_POINT('Ctrl Pts',(-0.192132668003466,0.0030191530391176,
-0.00882646181140498));
#43479=CARTESIAN_POINT('Ctrl Pts',(-0.192133661041556,0.0030140373109328,
-0.00883271844226365));
#43480=CARTESIAN_POINT('Ctrl Pts',(-0.192134510220713,0.00301097864583467,
-0.00883578008871502));
#43481=CARTESIAN_POINT('Ctrl Pts',(-0.192138197164547,0.0030000437412503,
-0.00884498967153028));
#43482=CARTESIAN_POINT('Ctrl Pts',(-0.192142128390703,0.00299134690026601,
-0.00884964983556151));
#43483=CARTESIAN_POINT('Ctrl Pts',(-0.192154479741903,0.00296719877950705,
-0.00885874451096875));
#43484=CARTESIAN_POINT('Ctrl Pts',(-0.1921653336808,0.00294909544095686,
-0.00886129523940827));
#43485=CARTESIAN_POINT('Ctrl Pts',(-0.192196429509983,0.00290264262977971,
-0.00885915219647058));
#43486=CARTESIAN_POINT('Ctrl Pts',(-0.192217925314133,0.00287403243266648,
-0.00885152302894445));
#43487=CARTESIAN_POINT('Ctrl Pts',(-0.1922431894099,0.00284378191811412,
-0.00883670835956577));
#43488=CARTESIAN_POINT('Ctrl Pts',(-0.192245761353967,0.00284072455684682,
-0.00883512844000508));
#43489=CARTESIAN_POINT('Ctrl Pts',(-0.192248330636423,0.00283771782980501,
-0.00883349208308415));
#43490=CARTESIAN_POINT('Ctrl Pts',(-0.192146295419618,0.007998500997684,
-0.00993609477708802));
#43491=CARTESIAN_POINT('Ctrl Pts',(-0.192143163680161,0.00800393442705837,
-0.0100379107780708));
#43492=CARTESIAN_POINT('Ctrl Pts',(-0.192244833050654,0.00799565242682731,
-0.0100394822591525));
#43493=CARTESIAN_POINT('Ctrl Pts',(-0.192066759891807,0.00703646350569687,
-0.00998607675950129));
#43494=CARTESIAN_POINT('Ctrl Pts',(-0.192063607017836,0.00703133130810636,
-0.0100884494227043));
#43495=CARTESIAN_POINT('Ctrl Pts',(-0.192165083030494,0.0070212017559552,
-0.0100890993436359));
#43496=CARTESIAN_POINT('Ctrl Pts',(-0.191868670782975,0.00507862867971864,
-0.00978403360874624));
#43497=CARTESIAN_POINT('Ctrl Pts',(-0.191865622779181,0.00505262673975468,
-0.00988428333480491));
#43498=CARTESIAN_POINT('Ctrl Pts',(-0.191968270900675,0.00505204884076484,
-0.00988281487389815));
#43499=CARTESIAN_POINT('Ctrl Pts',(-0.19209757540129,0.00327314217054443,
-0.00900318967073468));
#43500=CARTESIAN_POINT('Ctrl Pts',(-0.19209486680983,0.00322733400399338,
-0.00909490321918779));
#43501=CARTESIAN_POINT('Ctrl Pts',(-0.192196050463947,0.00323906751335872,
-0.00910136943874098));
#43502=CARTESIAN_POINT('Ctrl Pts',(-0.192205000280064,0.0024605199261876,
-0.00849014764764348));
#43503=CARTESIAN_POINT('Ctrl Pts',(-0.192202514426249,0.00240604705426371,
-0.00857635021631835));
#43504=CARTESIAN_POINT('Ctrl Pts',(-0.192303953731296,0.00241478292287016,
-0.00858251379116096));
#43505=CARTESIAN_POINT('Ctrl Pts',(-0.192104402373237,0.00750389176243192,
-0.00994933158139058));
#43506=CARTESIAN_POINT('Ctrl Pts',(-0.192103979165972,0.00750527449581046,
-0.00997324593122452));
#43507=CARTESIAN_POINT('Ctrl Pts',(-0.192111890405995,0.00750588809089745,
-0.0100049234964412));
#43508=CARTESIAN_POINT('Ctrl Pts',(-0.192141219896257,0.0075050875176516,
-0.0100289357476997));
#43509=CARTESIAN_POINT('Ctrl Pts',(-0.192157040747162,0.00750465567414363,
-0.0100418883849151));
#43510=CARTESIAN_POINT('Ctrl Pts',(-0.192179303563212,0.00750379772760193,
-0.0100510538033473));
#43511=CARTESIAN_POINT('Ctrl Pts',(-0.192202406927022,0.00750306323134365,
-0.0100515763887981));
#43512=CARTESIAN_POINT('Origin',(-0.194542786613652,0.00713436881430736,
-0.00197293957666947));
#43513=CARTESIAN_POINT('Ctrl Pts',(-0.191102282748796,0.00750206962804297,
-0.00992689565167905));
#43514=CARTESIAN_POINT('Ctrl Pts',(-0.19110084689697,0.00750224800180091,
-0.00995579396725443));
#43515=CARTESIAN_POINT('Ctrl Pts',(-0.191084835201888,0.00750291681681606,
-0.00999379021915688));
#43516=CARTESIAN_POINT('Ctrl Pts',(-0.191046197864609,0.00750287758542002,
-0.01001378202915));
#43517=CARTESIAN_POINT('Ctrl Pts',(-0.191033355225391,0.00750286454532199,
-0.0100204270937726));
#43518=CARTESIAN_POINT('Ctrl Pts',(-0.191018294913059,0.00750280309028856,
-0.0100247834669135));
#43519=CARTESIAN_POINT('Ctrl Pts',(-0.191002128651513,0.0075027969382303,
-0.0100254082193667));
#43520=CARTESIAN_POINT('Origin',(-0.195908379925447,0.00793866795006121,
-0.00229708592964099));
#43521=CARTESIAN_POINT('Ctrl Pts',(-0.192244563328644,0.012158535091762,
-0.00883493377276686));
#43522=CARTESIAN_POINT('Ctrl Pts',(-0.192244179096753,0.012158413276973,
-0.00883499662067414));
#43523=CARTESIAN_POINT('Ctrl Pts',(-0.192244009117953,0.0121583548679729,
-0.00883502642875641));
#43524=CARTESIAN_POINT('Ctrl Pts',(-0.192243835442115,0.0121582916006088,
-0.00883505847795769));
#43525=CARTESIAN_POINT('Ctrl Pts',(-0.192243830465275,0.0121582897845668,
-0.00883505939771415));
#43526=CARTESIAN_POINT('Ctrl Pts',(-0.192243820502454,0.0121582861430353,
-0.00883506124162917));
#43527=CARTESIAN_POINT('Ctrl Pts',(-0.192243815516433,0.0121582843175171,
-0.00883506216580142));
#43528=CARTESIAN_POINT('Ctrl Pts',(-0.192243719827578,0.0121582492244368,
-0.00883507992807604));
#43529=CARTESIAN_POINT('Ctrl Pts',(-0.192243629519956,0.0121582150908203,
-0.00883509714156986));
#43530=CARTESIAN_POINT('Ctrl Pts',(-0.192243318166538,0.0121580940099678,
-0.00883515799640806));
#43531=CARTESIAN_POINT('Ctrl Pts',(-0.192243099165596,0.0121580028658637,
-0.00883520345347272));
#43532=CARTESIAN_POINT('Ctrl Pts',(-0.192242404343482,0.0121576961340143,
-0.00883535544509771));
#43533=CARTESIAN_POINT('Ctrl Pts',(-0.192241937163062,0.0121574629129843,
-0.00883546958366822));
#43534=CARTESIAN_POINT('Ctrl Pts',(-0.192232139839439,0.0121521069651809,
-0.00883806590403842));
#43535=CARTESIAN_POINT('Ctrl Pts',(-0.192217601244657,0.0121348786044592,
-0.00884610483975265));
#43536=CARTESIAN_POINT('Ctrl Pts',(-0.192183260265204,0.0120914561509524,
-0.00885704352957424));
#43537=CARTESIAN_POINT('Ctrl Pts',(-0.192167589750093,0.0120694134393657,
-0.00885892799173005));
#43538=CARTESIAN_POINT('Ctrl Pts',(-0.192144836873875,0.0120336815526016,
-0.00885476525831273));
#43539=CARTESIAN_POINT('Ctrl Pts',(-0.192136970607259,0.0120197474923018,
-0.00885049237666547));
#43540=CARTESIAN_POINT('Ctrl Pts',(-0.192128650361237,0.0120021571809274,
-0.00884064170141953));
#43541=CARTESIAN_POINT('Ctrl Pts',(-0.192126285923881,0.0119964577393178,
-0.00883653504531708));
#43542=CARTESIAN_POINT('Ctrl Pts',(-0.192123366403244,0.0119873004964977,
-0.00882746897412633));
#43543=CARTESIAN_POINT('Ctrl Pts',(-0.1921225745397,0.0119837180093985,
-0.00882293875239021));
#43544=CARTESIAN_POINT('Ctrl Pts',(-0.192122375507901,0.0119807553525039,
-0.00881789966923123));
#43545=CARTESIAN_POINT('Origin',(-0.194558258525404,0.00786744520569803,
-0.00198084692036992));
#43546=CARTESIAN_POINT('Ctrl Pts',(-0.191053647336185,0.011398350991669,
-0.00908383078920412));
#43547=CARTESIAN_POINT('Ctrl Pts',(-0.191051239176385,0.0114090168040769,
-0.00912362545786433));
#43548=CARTESIAN_POINT('Ctrl Pts',(-0.191015561786232,0.0114450835541685,
-0.00917073228352145));
#43549=CARTESIAN_POINT('Ctrl Pts',(-0.190954180653395,0.0114759554932708,
-0.00915737097626284));
#43550=CARTESIAN_POINT('Ctrl Pts',(-0.1909336611347,0.0112622521590659,
-0.00914107486762373));
#43551=CARTESIAN_POINT('Ctrl Pts',(-0.190932330870403,0.0113043272600339,
-0.00923806989977741));
#43552=CARTESIAN_POINT('Ctrl Pts',(-0.19085519609301,0.0113669344340182,
-0.00920333160470119));
#43553=CARTESIAN_POINT('Ctrl Pts',(-0.191122119826402,0.0114988266428744,
-0.00904149146625021));
#43554=CARTESIAN_POINT('Ctrl Pts',(-0.191121088423278,0.0115437728913739,
-0.00913705611144188));
#43555=CARTESIAN_POINT('Ctrl Pts',(-0.191032928044611,0.0115971369215591,
-0.0091047534093575));
#43556=CARTESIAN_POINT('Ctrl Pts',(-0.191561405133145,0.0117972153315813,
-0.00890344882356972));
#43557=CARTESIAN_POINT('Ctrl Pts',(-0.191560810155806,0.0118456413151578,
-0.00899816312114753));
#43558=CARTESIAN_POINT('Ctrl Pts',(-0.191527443414654,0.011939457961494,
-0.00894345319026215));
#43559=CARTESIAN_POINT('Ctrl Pts',(-0.192148825589603,0.0119861110815885,
-0.00881409348298998));
#43560=CARTESIAN_POINT('Ctrl Pts',(-0.192147358846835,0.0120362465102458,
-0.00890767634883105));
#43561=CARTESIAN_POINT('Ctrl Pts',(-0.192106861687747,0.0121182030755903,
-0.00885578258088416));
#43562=CARTESIAN_POINT('Ctrl Pts',(-0.192426465779805,0.0120908510696967,
-0.00876130870259275));
#43563=CARTESIAN_POINT('Ctrl Pts',(-0.192425268473339,0.0121423011087959,
-0.00885420723634552));
#43564=CARTESIAN_POINT('Ctrl Pts',(-0.192385661689457,0.0122252927060059,
-0.00880048787717269));
#43565=CARTESIAN_POINT('Ctrl Pts',(-0.203143265159837,0.00801633370630912,
0.0101836825777989));
#43566=CARTESIAN_POINT('Ctrl Pts',(-0.203141479769113,0.00802239493892441,
0.0102900229538855));
#43567=CARTESIAN_POINT('Ctrl Pts',(-0.203035639253689,0.00803068137178952,
0.0102810066415951));
#43568=CARTESIAN_POINT('Ctrl Pts',(-0.203057840262184,0.00699344469555275,
0.0102395505548407));
#43569=CARTESIAN_POINT('Ctrl Pts',(-0.203056037604557,0.00698755444036989,
0.0103465767165832));
#43570=CARTESIAN_POINT('Ctrl Pts',(-0.202950424815462,0.00699862012239534,
0.0103385142775995));
#43571=CARTESIAN_POINT('Ctrl Pts',(-0.202848073423076,0.00493786641202183,
0.010005192713933));
#43572=CARTESIAN_POINT('Ctrl Pts',(-0.20284636887628,0.00490851213721418,
0.0101095556223153));
#43573=CARTESIAN_POINT('Ctrl Pts',(-0.202739295599067,0.00491062963068159,
0.0101043323211961));
#43574=CARTESIAN_POINT('Ctrl Pts',(-0.20312347492238,0.00307357464602607,
0.00913154713288676));
#43575=CARTESIAN_POINT('Ctrl Pts',(-0.203122182207117,0.00302234432021556,
0.00922571364394402));
#43576=CARTESIAN_POINT('Ctrl Pts',(-0.203017150689644,0.00301157267859386,
0.00921085094367838));
#43577=CARTESIAN_POINT('Ctrl Pts',(-0.203261837521653,0.00223709682645751,
0.00855350483889566));
#43578=CARTESIAN_POINT('Ctrl Pts',(-0.203260791220819,0.00217640800752592,
0.00864104067122755));
#43579=CARTESIAN_POINT('Ctrl Pts',(-0.203155400916974,0.00216992139680255,
0.00862693547917218));
#43580=CARTESIAN_POINT('Ctrl Pts',(-0.203091794492762,0.00260433584368978,
0.00891063288456858));
#43581=CARTESIAN_POINT('Ctrl Pts',(-0.203092578852937,0.0026051042160043,
0.00891112148092724));
#43582=CARTESIAN_POINT('Ctrl Pts',(-0.203094718463783,0.00260715346510506,
0.00891239001105441));
#43583=CARTESIAN_POINT('Ctrl Pts',(-0.203096849812164,0.00260926123651513,
0.00891357333550009));
#43584=CARTESIAN_POINT('Ctrl Pts',(-0.203103814059988,0.00261647262656566,
0.00891752136660277));
#43585=CARTESIAN_POINT('Ctrl Pts',(-0.203113335016935,0.00262651213720627,
0.00892216941256439));
#43586=CARTESIAN_POINT('Ctrl Pts',(-0.2031331443551,0.00265049040226918,
0.00892670658809943));
#43587=CARTESIAN_POINT('Ctrl Pts',(-0.203141708444645,0.00266179522616666,
0.0089270465013639));
#43588=CARTESIAN_POINT('Ctrl Pts',(-0.203158061311166,0.00268588448919631,
0.00892337370530938));
#43589=CARTESIAN_POINT('Ctrl Pts',(-0.203165168467178,0.00269794277366491,
0.00891903258144683));
#43590=CARTESIAN_POINT('Ctrl Pts',(-0.20317380042585,0.00271569204477004,
0.00890841480613177));
#43591=CARTESIAN_POINT('Ctrl Pts',(-0.203176481264999,0.00272221842788613,
0.00890337129535317));
#43592=CARTESIAN_POINT('Ctrl Pts',(-0.203179953610341,0.00273350931465458,
0.00889196533745507));
#43593=CARTESIAN_POINT('Ctrl Pts',(-0.203180871974325,0.00273826982050736,
0.00888590166379555));
#43594=CARTESIAN_POINT('Ctrl Pts',(-0.203180998697126,0.00274230934947549,
0.00887926197739174));
#43595=CARTESIAN_POINT('Ctrl Pts',(-0.203100639709157,0.00753037906826921,
0.0102107450661697));
#43596=CARTESIAN_POINT('Ctrl Pts',(-0.203099090135222,0.00752951923346159,
0.0102203116781152));
#43597=CARTESIAN_POINT('Ctrl Pts',(-0.203096168617054,0.00752883521908611,
0.0102296213721084));
#43598=CARTESIAN_POINT('Ctrl Pts',(-0.203086495197114,0.00752764953261652,
0.0102497511281073));
#43599=CARTESIAN_POINT('Ctrl Pts',(-0.203078942608029,0.00752723754370073,
0.0102600067102118));
#43600=CARTESIAN_POINT('Ctrl Pts',(-0.203060470790915,0.00752760843690622,
0.0102772538922881));
#43601=CARTESIAN_POINT('Ctrl Pts',(-0.203050718764228,0.00752840964011891,
0.0102830934125772));
#43602=CARTESIAN_POINT('Ctrl Pts',(-0.203036937214749,0.00753175678717982,
0.0102893280833497));
#43603=CARTESIAN_POINT('Ctrl Pts',(-0.203031505707383,0.00753367407208893,
0.0102911984979226));
#43604=CARTESIAN_POINT('Ctrl Pts',(-0.203026668027738,0.00753693501435748,
0.0102924850185916));
#43605=CARTESIAN_POINT('Origin',(-0.206700215990262,0.00793489080233831,
0.00270768538981742));
#43606=CARTESIAN_POINT('Ctrl Pts',(-0.203173149129105,0.0122530883762422,
0.00888129643155584));
#43607=CARTESIAN_POINT('Ctrl Pts',(-0.20317297440395,0.0122560948442299,
0.00888629945558956));
#43608=CARTESIAN_POINT('Ctrl Pts',(-0.203172378826803,0.0122595322427759,
0.00889101768852518));
#43609=CARTESIAN_POINT('Ctrl Pts',(-0.203169545170064,0.0122702686487425,
0.00890330463092521));
#43610=CARTESIAN_POINT('Ctrl Pts',(-0.203166444115766,0.0122781780964424,
0.00890980912223253));
#43611=CARTESIAN_POINT('Ctrl Pts',(-0.203157426591178,0.0122970194599052,
0.00892114765645108));
#43612=CARTESIAN_POINT('Ctrl Pts',(-0.203151137454044,0.012308013466242,
0.00892515690985519));
#43613=CARTESIAN_POINT('Ctrl Pts',(-0.203133565785846,0.0123357834919288,
0.00893042776982717));
#43614=CARTESIAN_POINT('Ctrl Pts',(-0.203122403731747,0.0123508441733906,
0.0089287818815233));
#43615=CARTESIAN_POINT('Ctrl Pts',(-0.203109264237317,0.0123696428494649,
0.00892395720889688));
#43616=CARTESIAN_POINT('Ctrl Pts',(-0.20310482039667,0.012376293311655,
0.00892138071276046));
#43617=CARTESIAN_POINT('Ctrl Pts',(-0.203101792285941,0.0123844394819698,
0.00891742855940335));
#43618=CARTESIAN_POINT('Ctrl Pts',(-0.203101356726026,0.0123866121346325,
0.00891626326363771));
#43619=CARTESIAN_POINT('Ctrl Pts',(-0.203101333135073,0.0123892896384871,
0.00891472662097877));
#43620=CARTESIAN_POINT('Ctrl Pts',(-0.203101370574358,0.0123899340365954,
0.00891434790493989));
#43621=CARTESIAN_POINT('Ctrl Pts',(-0.20310145223708,0.0123905738715769,
0.00891396305599815));
#43622=CARTESIAN_POINT('Origin',(-0.20434441778413,0.00265832731369415,
0.00885114693566833));
#43623=CARTESIAN_POINT('Ctrl Pts',(-0.204181316283697,0.00274294303023111,
0.00890078282268103));
#43624=CARTESIAN_POINT('Ctrl Pts',(-0.204181287056828,0.00273881907435617,
0.00890738725852497));
#43625=CARTESIAN_POINT('Ctrl Pts',(-0.204182292259389,0.00273400615712081,
0.00891340235304115));
#43626=CARTESIAN_POINT('Ctrl Pts',(-0.204186507159662,0.00272228467311434,
0.00892516085818481));
#43627=CARTESIAN_POINT('Ctrl Pts',(-0.204190032653031,0.00271535424362842,
0.00893042203587288));
#43628=CARTESIAN_POINT('Ctrl Pts',(-0.204201200298807,0.00269705888163771,
0.00894125171668725));
#43629=CARTESIAN_POINT('Ctrl Pts',(-0.204210471656198,0.00268472038578496,
0.00894569431453476));
#43630=CARTESIAN_POINT('Ctrl Pts',(-0.204231987787325,0.00266013135857193,
0.0089495490570302));
#43631=CARTESIAN_POINT('Ctrl Pts',(-0.204243288857956,0.00264868401162524,
0.00894923152111447));
#43632=CARTESIAN_POINT('Ctrl Pts',(-0.204271708133428,0.00262245426542647,
0.00894440471167718));
#43633=CARTESIAN_POINT('Ctrl Pts',(-0.2042855456873,0.00261180096071676,
0.00893858233952874));
#43634=CARTESIAN_POINT('Ctrl Pts',(-0.204290481497631,0.00260829237482262,
0.00893668044444359));
#43635=CARTESIAN_POINT('Ctrl Pts',(-0.204291369900567,0.00260750940639311,
0.00893623488881915));
#43636=CARTESIAN_POINT('Ctrl Pts',(-0.204292561846107,0.00260646367638606,
0.00893563174137504));
#43637=CARTESIAN_POINT('Ctrl Pts',(-0.20429351437778,0.00260574920645494,
0.00893520949065184));
#43638=CARTESIAN_POINT('Origin',(-0.203018603003138,0.0123389583705484,
0.00882666246850923));
#43639=CARTESIAN_POINT('Ctrl Pts',(-0.204179891859367,0.0122530438601656,
0.00890316754771291));
#43640=CARTESIAN_POINT('Ctrl Pts',(-0.204179863704633,0.0122570464468669,
0.00890958321584623));
#43641=CARTESIAN_POINT('Ctrl Pts',(-0.204180810870288,0.0122617012456198,
0.0089154459307373));
#43642=CARTESIAN_POINT('Ctrl Pts',(-0.204184790811729,0.0122730144205793,
0.00892694531711205));
#43643=CARTESIAN_POINT('Ctrl Pts',(-0.204188120976517,0.0122796964340686,
0.00893213201592682));
#43644=CARTESIAN_POINT('Ctrl Pts',(-0.204198812236045,0.012297539383815,
0.00894301985940397));
#43645=CARTESIAN_POINT('Ctrl Pts',(-0.204207792790586,0.0123096697165854,
0.00894760162878872));
#43646=CARTESIAN_POINT('Ctrl Pts',(-0.20422856390432,0.0123337324139222,
0.00895181197930262));
#43647=CARTESIAN_POINT('Ctrl Pts',(-0.204239392292698,0.0123448692438461,
0.00895175758388408));
#43648=CARTESIAN_POINT('Ctrl Pts',(-0.204264059719803,0.0123680501513342,
0.0089481455679986));
#43649=CARTESIAN_POINT('Ctrl Pts',(-0.204276250240103,0.0123780056183922,
0.00894405172270597));
#43650=CARTESIAN_POINT('Ctrl Pts',(-0.2042855365112,0.0123853730064948,
0.00894033700997319));
#43651=CARTESIAN_POINT('Ctrl Pts',(-0.204288263139933,0.0123874525706704,
0.00893926256526248));
#43652=CARTESIAN_POINT('Ctrl Pts',(-0.204290996832348,0.0123894716281726,
0.00893810788811969));
#43653=CARTESIAN_POINT('Ctrl Pts',(-0.204292042411585,0.0123902568575966,
0.00893764437443986));
#43654=CARTESIAN_POINT('Ctrl Pts',(-0.204265062019709,0.00221964372301113,
0.00856007836605492));
#43655=CARTESIAN_POINT('Ctrl Pts',(-0.204262719720836,0.0021612997731543,
0.00864368340093128));
#43656=CARTESIAN_POINT('Ctrl Pts',(-0.204363887539702,0.00217154023637526,
0.00865137136587931));
#43657=CARTESIAN_POINT('Ctrl Pts',(-0.20412805707869,0.00305073619898106,
0.00913959446919662));
#43658=CARTESIAN_POINT('Ctrl Pts',(-0.20412547082334,0.0030014403681275,
0.00922956938389137));
#43659=CARTESIAN_POINT('Ctrl Pts',(-0.204226293290499,0.00301522546561237,
0.00923757183785008));
#43660=CARTESIAN_POINT('Ctrl Pts',(-0.203844723877951,0.00493114335503218,
0.0100298425834166));
#43661=CARTESIAN_POINT('Ctrl Pts',(-0.203841781000808,0.00490291518671609,
0.0101297327317632));
#43662=CARTESIAN_POINT('Ctrl Pts',(-0.203944568193161,0.00490313323676524,
0.0101279022979083));
#43663=CARTESIAN_POINT('Ctrl Pts',(-0.20405840197198,0.00700620797942271,
0.0102626710355198));
#43664=CARTESIAN_POINT('Ctrl Pts',(-0.204055332333839,0.00700060634176611,
0.0103650944362403));
#43665=CARTESIAN_POINT('Ctrl Pts',(-0.204156747239523,0.00699020166858962,
0.0103656362115123));
#43666=CARTESIAN_POINT('Ctrl Pts',(-0.204143719711716,0.00802360799215748,
0.0102055713602495));
#43667=CARTESIAN_POINT('Ctrl Pts',(-0.204140674006327,0.00802944118873702,
0.0103073413719115));
#43668=CARTESIAN_POINT('Ctrl Pts',(-0.204242315972835,0.00802109309748085,
0.0103088959211302));
#43669=CARTESIAN_POINT('Ctrl Pts',(-0.204098734059757,0.00749980245225468,
0.0102204145824933));
#43670=CARTESIAN_POINT('Ctrl Pts',(-0.204098586165758,0.00749980223570916,
0.0102269586333304));
#43671=CARTESIAN_POINT('Ctrl Pts',(-0.204099083587065,0.00749980221762655,
0.0102335010073826));
#43672=CARTESIAN_POINT('Ctrl Pts',(-0.204101426216882,0.00749980258329951,
0.0102468033715967));
#43673=CARTESIAN_POINT('Ctrl Pts',(-0.204103348425244,0.00749980299171968,
0.0102535135368467));
#43674=CARTESIAN_POINT('Ctrl Pts',(-0.204110773522535,0.00749980474828837,
0.0102719151173418));
#43675=CARTESIAN_POINT('Ctrl Pts',(-0.204117860546261,0.00749980659017663,
0.010282814526926));
#43676=CARTESIAN_POINT('Ctrl Pts',(-0.204135778200342,0.00749981131633409,
0.0103013367558254));
#43677=CARTESIAN_POINT('Ctrl Pts',(-0.204146442862644,0.00749981423845238,
0.0103087851890371));
#43678=CARTESIAN_POINT('Ctrl Pts',(-0.204168352148334,0.0074998193372597,
0.0103185181067941));
#43679=CARTESIAN_POINT('Ctrl Pts',(-0.204179148198187,0.0074998348658371,
0.0103213088532629));
#43680=CARTESIAN_POINT('Ctrl Pts',(-0.204192371349525,0.00749981086548528,
0.0103224861895429));
#43681=CARTESIAN_POINT('Ctrl Pts',(-0.204194612627097,0.00749983027531024,
0.0103226110687671));
#43682=CARTESIAN_POINT('Ctrl Pts',(-0.204196825282634,0.00749983099238885,
0.0103226610749368));
#43683=CARTESIAN_POINT('Ctrl Pts',(-0.204143994057702,0.00697676071699483,
0.0102055666886271));
#43684=CARTESIAN_POINT('Ctrl Pts',(-0.2041408601556,0.00697091981646658,
0.0103074234560016));
#43685=CARTESIAN_POINT('Ctrl Pts',(-0.204242585767289,0.00697933425661569,
0.0103089798359738));
#43686=CARTESIAN_POINT('Ctrl Pts',(-0.204058114946837,0.0079928086477191,
0.0102622888245846));
#43687=CARTESIAN_POINT('Ctrl Pts',(-0.204054957478253,0.00799839543298179,
0.0103647962811805));
#43688=CARTESIAN_POINT('Ctrl Pts',(-0.204156454632279,0.00800888585074875,
0.0103653299370992));
#43689=CARTESIAN_POINT('Ctrl Pts',(-0.203843707641205,0.0100628925980128,
0.0100315736472558));
#43690=CARTESIAN_POINT('Ctrl Pts',(-0.203840675038655,0.0100910782349306,
0.0101315715362989));
#43691=CARTESIAN_POINT('Ctrl Pts',(-0.203943552101339,0.0100908447850691,
0.0101297390895283));
#43692=CARTESIAN_POINT('Ctrl Pts',(-0.204127325890448,0.0119475991503093,
0.00914023055516254));
#43693=CARTESIAN_POINT('Ctrl Pts',(-0.204124652395982,0.0119969311050922,
0.00923028348964983));
#43694=CARTESIAN_POINT('Ctrl Pts',(-0.204225570130192,0.0119831834122565,
0.00923826131726373));
#43695=CARTESIAN_POINT('Ctrl Pts',(-0.204263055354891,0.0127748578564395,
0.00856365183920312));
#43696=CARTESIAN_POINT('Ctrl Pts',(-0.204260624482029,0.0128332000492351,
0.00864736250104337));
#43697=CARTESIAN_POINT('Ctrl Pts',(-0.204361886645732,0.0128229809829309,
0.00865502158265919));
#43698=CARTESIAN_POINT('Ctrl Pts',(-0.205143217748733,0.00801648272260619,
0.0102288513503545));
#43699=CARTESIAN_POINT('Ctrl Pts',(-0.205141397070134,0.00802259035131162,
0.0103355159558339));
#43700=CARTESIAN_POINT('Ctrl Pts',(-0.205035270082177,0.00803097181891989,
0.0103261045172673));
#43701=CARTESIAN_POINT('Ctrl Pts',(-0.205056278613804,0.00699374265691425,
0.0102848962094768));
#43702=CARTESIAN_POINT('Ctrl Pts',(-0.205054440918194,0.0069878185985912,
0.0103922540218368));
#43703=CARTESIAN_POINT('Ctrl Pts',(-0.204948544649311,0.00699911071925452,
0.0103838328287035));
#43704=CARTESIAN_POINT('Ctrl Pts',(-0.204846431243139,0.00493848158252054,
0.0100498578329968));
#43705=CARTESIAN_POINT('Ctrl Pts',(-0.204844691090855,0.00490894474163874,
0.0101545286263539));
#43706=CARTESIAN_POINT('Ctrl Pts',(-0.204737314569065,0.0049109166968098,
0.0101488940353842));
#43707=CARTESIAN_POINT('Ctrl Pts',(-0.205124469597499,0.00307519585421071,
0.00917342141693886));
#43708=CARTESIAN_POINT('Ctrl Pts',(-0.205123141870177,0.00302363744285394,
0.00926778892652763));
#43709=CARTESIAN_POINT('Ctrl Pts',(-0.205017814730547,0.00301308425163072,
0.0092525626970204));
#43710=CARTESIAN_POINT('Ctrl Pts',(-0.205262224641199,0.00223986690673841,
0.00859354485513374));
#43711=CARTESIAN_POINT('Ctrl Pts',(-0.20526114296998,0.00217880555930881,
0.00868121881747347));
#43712=CARTESIAN_POINT('Ctrl Pts',(-0.205155455117607,0.00217252875054394,
0.00866676529248969));
#43713=CARTESIAN_POINT('Ctrl Pts',(-0.205092334702737,0.00260645295233614,
0.00895141938274717));
#43714=CARTESIAN_POINT('Ctrl Pts',(-0.205093133563206,0.0026072343879083,
0.00895191840030636));
#43715=CARTESIAN_POINT('Ctrl Pts',(-0.205095258409959,0.0026092688461218,
0.00895318228735311));
#43716=CARTESIAN_POINT('Ctrl Pts',(-0.205097375225393,0.00261136069190115,
0.00895436288913649));
#43717=CARTESIAN_POINT('Ctrl Pts',(-0.205104532774812,0.00261875781133091,
0.00895843071484043));
#43718=CARTESIAN_POINT('Ctrl Pts',(-0.205114102664032,0.00262887791286909,
0.00896304924228411));
#43719=CARTESIAN_POINT('Ctrl Pts',(-0.205133688318084,0.00265257222454595,
0.00896757768358735));
#43720=CARTESIAN_POINT('Ctrl Pts',(-0.205142252981025,0.00266387538604602,
0.00896793796110294));
#43721=CARTESIAN_POINT('Ctrl Pts',(-0.205158606120922,0.00268796880691882,
0.00896430844256256));
#43722=CARTESIAN_POINT('Ctrl Pts',(-0.20516571311459,0.00270003373063085,
0.00895998919280492));
#43723=CARTESIAN_POINT('Ctrl Pts',(-0.20517434484453,0.00271780094254793,
0.00894940393856633));
#43724=CARTESIAN_POINT('Ctrl Pts',(-0.205177025557873,0.00272433601707078,
0.0089443725583336));
#43725=CARTESIAN_POINT('Ctrl Pts',(-0.205180497843194,0.00273564720144894,
0.00893298795623472));
#43726=CARTESIAN_POINT('Ctrl Pts',(-0.205181416246512,0.00274041875726572,
0.00892693338808831));
#43727=CARTESIAN_POINT('Ctrl Pts',(-0.20518154308962,0.00274447060991368,
0.00892030161323929));
#43728=CARTESIAN_POINT('Ctrl Pts',(-0.205098436543116,0.00749984782009145,
0.010243256758359));
#43729=CARTESIAN_POINT('Ctrl Pts',(-0.205098274430575,0.00749984762351407,
0.0102497175728602));
#43730=CARTESIAN_POINT('Ctrl Pts',(-0.205097483994373,0.00749984725475431,
0.0102561471696715));
#43731=CARTESIAN_POINT('Ctrl Pts',(-0.2050945605171,0.00749984612943716,
0.0102692497779461));
#43732=CARTESIAN_POINT('Ctrl Pts',(-0.205092336917074,0.00749984534854801,
0.0102758663933169));
#43733=CARTESIAN_POINT('Ctrl Pts',(-0.205084087417224,0.00749984256928602,
0.0102939138606672));
#43734=CARTESIAN_POINT('Ctrl Pts',(-0.205076514757121,0.00749984013949185,
0.0103044818481159));
#43735=CARTESIAN_POINT('Ctrl Pts',(-0.20505777758101,0.00749983400823954,
0.0103221754888335));
#43736=CARTESIAN_POINT('Ctrl Pts',(-0.205046786694621,0.00749983051795828,
0.0103291343648038));
#43737=CARTESIAN_POINT('Ctrl Pts',(-0.20502348624436,0.00749982117772525,
0.0103382476987318));
#43738=CARTESIAN_POINT('Ctrl Pts',(-0.205012451916365,0.00749983699066525,
0.0103402134687604));
#43739=CARTESIAN_POINT('Ctrl Pts',(-0.205000337272074,0.00749978528464776,
0.0103407438028927));
#43740=CARTESIAN_POINT('Ctrl Pts',(-0.20499801233247,0.00749981993605052,
0.0103407686501798));
#43741=CARTESIAN_POINT('Ctrl Pts',(-0.204995837238769,0.0074998193282587,
0.0103407196921656));
#43742=CARTESIAN_POINT('Ctrl Pts',(-0.205260925816527,0.0127573393964206,
0.0085954370355821));
#43743=CARTESIAN_POINT('Ctrl Pts',(-0.205259981441613,0.012818177596082,
0.00868288953285713));
#43744=CARTESIAN_POINT('Ctrl Pts',(-0.205154563041824,0.0128246666377038,
0.00866886932633953));
#43745=CARTESIAN_POINT('Ctrl Pts',(-0.20512350504628,0.011918896615286,
0.00917641659755658));
#43746=CARTESIAN_POINT('Ctrl Pts',(-0.205122314353347,0.0119702189154387,
0.00927055622826414));
#43747=CARTESIAN_POINT('Ctrl Pts',(-0.205017252916804,0.0119808957925622,
0.00925580328110713));
#43748=CARTESIAN_POINT('Ctrl Pts',(-0.204846130960769,0.010062506110505,
0.0100487182598789));
#43749=CARTESIAN_POINT('Ctrl Pts',(-0.20484453360047,0.0100919672421221,
0.0101530708413611));
#43750=CARTESIAN_POINT('Ctrl Pts',(-0.204737436020278,0.0100902502137758,
0.010147851443999));
#43751=CARTESIAN_POINT('Ctrl Pts',(-0.205055807234136,0.00800548029823725,
0.0102849382972628));
#43752=CARTESIAN_POINT('Ctrl Pts',(-0.205054110390278,0.00801139161403613,
0.010391986660739));
#43753=CARTESIAN_POINT('Ctrl Pts',(-0.204948492565434,0.00800006338884696,
0.0103840497641343));
#43754=CARTESIAN_POINT('Ctrl Pts',(-0.205143559896196,0.00698344979987348,
0.0102286690008394));
#43755=CARTESIAN_POINT('Ctrl Pts',(-0.205141880339568,0.00697737023664258,
0.0103350246469026));
#43756=CARTESIAN_POINT('Ctrl Pts',(-0.205036031913016,0.00696893486623635,
0.0103260790360151));
#43757=CARTESIAN_POINT('Ctrl Pts',(-0.205180445672117,0.0122517034922546,
0.00892259327448536));
#43758=CARTESIAN_POINT('Ctrl Pts',(-0.205180323054652,0.0122556110563871,
0.00892899712366704));
#43759=CARTESIAN_POINT('Ctrl Pts',(-0.20517946244098,0.0122601909823991,
0.00893486620714245));
#43760=CARTESIAN_POINT('Ctrl Pts',(-0.205176214037774,0.0122710085088525,
0.00894594287415477));
#43761=CARTESIAN_POINT('Ctrl Pts',(-0.205173710804417,0.0122772429515444,
0.00895088031987881));
#43762=CARTESIAN_POINT('Ctrl Pts',(-0.205165499740559,0.0122944821254439,
0.00896156581316046));
#43763=CARTESIAN_POINT('Ctrl Pts',(-0.205158619362418,0.0123063363280765,
0.00896607202978781));
#43764=CARTESIAN_POINT('Ctrl Pts',(-0.205142087193769,0.0123309994366319,
0.00897032808637686));
#43765=CARTESIAN_POINT('Ctrl Pts',(-0.205132977416631,0.0123430619084986,
0.00897004433852129));
#43766=CARTESIAN_POINT('Ctrl Pts',(-0.205109337949273,0.012371579399479,
0.00896456266879536));
#43767=CARTESIAN_POINT('Ctrl Pts',(-0.20509769511444,0.0123831368420804,
0.00895767977417679));
#43768=CARTESIAN_POINT('Ctrl Pts',(-0.205093745802734,0.0123869198976546,
0.00895550568412799));
#43769=CARTESIAN_POINT('Ctrl Pts',(-0.205092545621893,0.0123883647568986,
0.00895462655013412));
#43770=CARTESIAN_POINT('Ctrl Pts',(-0.205091196983166,0.0123896832404942,
0.00895378545522166));
#43771=CARTESIAN_POINT('Origin',(-0.206344955241137,0.00266032655011837,
0.00889192021703303));
#43772=CARTESIAN_POINT('Ctrl Pts',(-0.206181807720331,0.00274488366429473,
0.00894172134960159));
#43773=CARTESIAN_POINT('Ctrl Pts',(-0.206181777333857,0.00274074553468597,
0.00894832213101722));
#43774=CARTESIAN_POINT('Ctrl Pts',(-0.206182782627333,0.00273591857292603,
0.00895433149772863));
#43775=CARTESIAN_POINT('Ctrl Pts',(-0.2061869987975,0.00272417054420443,
0.00896607038342512));
#43776=CARTESIAN_POINT('Ctrl Pts',(-0.206190524634843,0.00271722901686468,
0.0089713181216008));
#43777=CARTESIAN_POINT('Ctrl Pts',(-0.206201693107854,0.00269891001608653,
0.00898211194303197));
#43778=CARTESIAN_POINT('Ctrl Pts',(-0.206210965191943,0.00268656061040968,
0.00898653002283859));
#43779=CARTESIAN_POINT('Ctrl Pts',(-0.206232328954445,0.00266213443912686,
0.00899030799369234));
#43780=CARTESIAN_POINT('Ctrl Pts',(-0.206243446851708,0.00265085165508385,
0.00899000345364994));
#43781=CARTESIAN_POINT('Ctrl Pts',(-0.206271503877879,0.00262488401632038,
0.00898530206088853));
#43782=CARTESIAN_POINT('Ctrl Pts',(-0.20628521595814,0.00261433437329706,
0.00897961320218937));
#43783=CARTESIAN_POINT('Ctrl Pts',(-0.206290127794076,0.0026107230526453,
0.00897768264932748));
#43784=CARTESIAN_POINT('Ctrl Pts',(-0.206291273089138,0.00260976640865154,
0.00897714670056697));
#43785=CARTESIAN_POINT('Ctrl Pts',(-0.206292808630783,0.0026084913937421,
0.00897641700608666));
#43786=CARTESIAN_POINT('Ctrl Pts',(-0.206294003176714,0.00260759611925214,
0.00897588559731814));
#43787=CARTESIAN_POINT('Origin',(-0.205019744048073,0.0123372008288139,
0.00886724630700698));
#43788=CARTESIAN_POINT('Ctrl Pts',(-0.206181037530589,0.0122515254343705,
0.00894387539800756));
#43789=CARTESIAN_POINT('Ctrl Pts',(-0.206181008360377,0.0122555416227814,
0.00895028645839285));
#43790=CARTESIAN_POINT('Ctrl Pts',(-0.206181955433058,0.0122602096263031,
0.00895614280721616));
#43791=CARTESIAN_POINT('Ctrl Pts',(-0.206185935826737,0.0122715473608068,
0.00896762203649176));
#43792=CARTESIAN_POINT('Ctrl Pts',(-0.206189265738046,0.0122782394074966,
0.00897279547154573));
#43793=CARTESIAN_POINT('Ctrl Pts',(-0.206199956453773,0.0122961040213282,
0.00898364839558845));
#43794=CARTESIAN_POINT('Ctrl Pts',(-0.206208936856501,0.0123082440318456,
0.0089882064826025));
#43795=CARTESIAN_POINT('Ctrl Pts',(-0.206229707690682,0.0123323170437131,
0.00899236976530477));
#43796=CARTESIAN_POINT('Ctrl Pts',(-0.20624053610774,0.0123434551022436,
0.00899229343561907));
#43797=CARTESIAN_POINT('Ctrl Pts',(-0.206265161532738,0.012366592468694,
0.00898864163563936));
#43798=CARTESIAN_POINT('Ctrl Pts',(-0.206277327979804,0.0123765295081089,
0.00898454730676776));
#43799=CARTESIAN_POINT('Ctrl Pts',(-0.206286691450758,0.0123839492220929,
0.0089807883441402));
#43800=CARTESIAN_POINT('Ctrl Pts',(-0.206289406067974,0.012386018586932,
0.00897971337216977));
#43801=CARTESIAN_POINT('Ctrl Pts',(-0.20629212794999,0.0123880284654335,
0.00897855924406012));
#43802=CARTESIAN_POINT('Ctrl Pts',(-0.206293185535286,0.0123888219494838,
0.00897808876183893));
#43803=CARTESIAN_POINT('Ctrl Pts',(-0.206265361080271,0.00222221827535806,
0.00859997798124637));
#43804=CARTESIAN_POINT('Ctrl Pts',(-0.206263035706064,0.00216379824786295,
0.00868332185176802));
#43805=CARTESIAN_POINT('Ctrl Pts',(-0.206364035202085,0.00217391790280425,
0.00869114406698921));
#43806=CARTESIAN_POINT('Ctrl Pts',(-0.206129039916538,0.00305219375783605,
0.00918130268389152));
#43807=CARTESIAN_POINT('Ctrl Pts',(-0.206126471811688,0.00300282276552956,
0.00927104603765872));
#43808=CARTESIAN_POINT('Ctrl Pts',(-0.206227126009343,0.00301644299843148,
0.00927918109642607));
#43809=CARTESIAN_POINT('Ctrl Pts',(-0.205843114295396,0.00493078093842745,
0.0100742895591365));
#43810=CARTESIAN_POINT('Ctrl Pts',(-0.20584019217099,0.00490250351805925,
0.0101739988347731));
#43811=CARTESIAN_POINT('Ctrl Pts',(-0.205942808907154,0.0049029244902082,
0.010172369914728));
#43812=CARTESIAN_POINT('Ctrl Pts',(-0.206056905126677,0.00700670674502859,
0.010308041670639));
#43813=CARTESIAN_POINT('Ctrl Pts',(-0.206053855846052,0.00700109571471318,
0.0104102978886477));
#43814=CARTESIAN_POINT('Ctrl Pts',(-0.206155087564965,0.00699052260417267,
0.0104109705696189));
#43815=CARTESIAN_POINT('Ctrl Pts',(-0.206143835444834,0.00802364330158489,
0.010250719836519));
#43816=CARTESIAN_POINT('Ctrl Pts',(-0.206140810023571,0.0080294871033969,
0.0103523190431676));
#43817=CARTESIAN_POINT('Ctrl Pts',(-0.206242270945703,0.00802106546893099,
0.0103540384991376));
#43818=CARTESIAN_POINT('Ctrl Pts',(-0.206098144959998,0.00749989479917323,
0.0102656028080008));
#43819=CARTESIAN_POINT('Ctrl Pts',(-0.206097997059586,0.00749989463897083,
0.0102721471703159));
#43820=CARTESIAN_POINT('Ctrl Pts',(-0.206098494595543,0.00749989465445635,
0.0102786898446544));
#43821=CARTESIAN_POINT('Ctrl Pts',(-0.206100837702042,0.00749989504069795,
0.0102919928424395));
#43822=CARTESIAN_POINT('Ctrl Pts',(-0.206102760293655,0.00749989543298072,
0.0102987033059631));
#43823=CARTESIAN_POINT('Ctrl Pts',(-0.206110186665226,0.00749989706680563,
0.0103171052918464));
#43824=CARTESIAN_POINT('Ctrl Pts',(-0.206117274672292,0.00749989873859384,
0.0103280045983479));
#43825=CARTESIAN_POINT('Ctrl Pts',(-0.206135194433958,0.0074999029495758,
0.010346526573871));
#43826=CARTESIAN_POINT('Ctrl Pts',(-0.206145860283699,0.00749990553928964,
0.0103539747648798));
#43827=CARTESIAN_POINT('Ctrl Pts',(-0.206167772870826,0.00749990981405412,
0.0103637077806601));
#43828=CARTESIAN_POINT('Ctrl Pts',(-0.206178569199203,0.00749992615583955,
0.0103664975019689));
#43829=CARTESIAN_POINT('Ctrl Pts',(-0.206191787570224,0.00749989903157803,
0.0103676744623668));
#43830=CARTESIAN_POINT('Ctrl Pts',(-0.206194034750604,0.00749992015594775,
0.0103677996707739));
#43831=CARTESIAN_POINT('Ctrl Pts',(-0.206196245004281,0.00749992079740314,
0.0103678496339236));
#43832=CARTESIAN_POINT('Ctrl Pts',(-0.206144104594209,0.00697680057252784,
0.0102506660646432));
#43833=CARTESIAN_POINT('Ctrl Pts',(-0.206140934104293,0.00697094762846495,
0.0103523029798102));
#43834=CARTESIAN_POINT('Ctrl Pts',(-0.206242430803,0.00697941470148986,
0.0103541300309738));
#43835=CARTESIAN_POINT('Ctrl Pts',(-0.206056577677555,0.00799264761430986,
0.0103075953740775));
#43836=CARTESIAN_POINT('Ctrl Pts',(-0.206053383823223,0.0079982387982383,
0.0104098867566766));
#43837=CARTESIAN_POINT('Ctrl Pts',(-0.206154650474734,0.008008907775399,
0.0104106527590022));
#43838=CARTESIAN_POINT('Ctrl Pts',(-0.205842604186409,0.0100635095616092,
0.0100759104351038));
#43839=CARTESIAN_POINT('Ctrl Pts',(-0.205839534753177,0.0100917343277227,
0.0101756804741991));
#43840=CARTESIAN_POINT('Ctrl Pts',(-0.205942191076445,0.0100912285879667,
0.0101741825465384));
#43841=CARTESIAN_POINT('Ctrl Pts',(-0.206128983923121,0.0119465421786305,
0.00918167990255796));
#43842=CARTESIAN_POINT('Ctrl Pts',(-0.206126272027682,0.0119959385645935,
0.0092714515540072));
#43843=CARTESIAN_POINT('Ctrl Pts',(-0.206226974205861,0.011982429450636,
0.00927964772645204));
#43844=CARTESIAN_POINT('Ctrl Pts',(-0.206264007846902,0.0127726530819234,
0.00860324800585114));
#43845=CARTESIAN_POINT('Ctrl Pts',(-0.206261537061061,0.0128310540613221,
0.00868665044708584));
#43846=CARTESIAN_POINT('Ctrl Pts',(-0.206362583389019,0.0128210156501638,
0.00869452929791549));
#43847=CARTESIAN_POINT('Ctrl Pts',(-0.207142444673933,0.00800781553972708,
0.010275022722237));
#43848=CARTESIAN_POINT('Ctrl Pts',(-0.207140064658573,0.0080138362133013,
0.0103806849379504));
#43849=CARTESIAN_POINT('Ctrl Pts',(-0.207034903442016,0.00802228009373349,
0.0103717639889522));
#43850=CARTESIAN_POINT('Ctrl Pts',(-0.207054099445209,0.00698801037561799,
0.0103300780697022));
#43851=CARTESIAN_POINT('Ctrl Pts',(-0.2070517042754,0.00698211378551127,
0.0104364239726335));
#43852=CARTESIAN_POINT('Ctrl Pts',(-0.206946767716351,0.00699343558996355,
0.0104285245883844));
#43853=CARTESIAN_POINT('Ctrl Pts',(-0.206845339015377,0.0049362023550447,
0.0100937709797338));
#43854=CARTESIAN_POINT('Ctrl Pts',(-0.206843032419443,0.00490681719228294,
0.0101974457807158));
#43855=CARTESIAN_POINT('Ctrl Pts',(-0.206736622083599,0.00490835191115651,
0.010192192130957));
#43856=CARTESIAN_POINT('Ctrl Pts',(-0.207125456189955,0.00307642210849726,
0.00921573551924576));
#43857=CARTESIAN_POINT('Ctrl Pts',(-0.207123567613966,0.0030251050994184,
0.0093090903467788));
#43858=CARTESIAN_POINT('Ctrl Pts',(-0.207019188297482,0.0030145359074727,
0.00929436328058973));
#43859=CARTESIAN_POINT('Ctrl Pts',(-0.207262560200634,0.00224233294950047,
0.00863411935968771));
#43860=CARTESIAN_POINT('Ctrl Pts',(-0.207260912515351,0.00218160679793509,
0.00872080422753244));
#43861=CARTESIAN_POINT('Ctrl Pts',(-0.207156176888109,0.00217517650829302,
0.00870680543946287));
#43862=CARTESIAN_POINT('Ctrl Pts',(-0.207092854540501,0.00260851289160005,
0.00899226593441351));
#43863=CARTESIAN_POINT('Ctrl Pts',(-0.207093661671656,0.00260930138402402,
0.00899277156336772));
#43864=CARTESIAN_POINT('Ctrl Pts',(-0.207095778208369,0.00261132664878968,
0.00899403454397879));
#43865=CARTESIAN_POINT('Ctrl Pts',(-0.207097886856061,0.00261340871206773,
0.00899521536690078));
#43866=CARTESIAN_POINT('Ctrl Pts',(-0.20710509653825,0.00262084830596442,
0.00899932471837138));
#43867=CARTESIAN_POINT('Ctrl Pts',(-0.207114650508154,0.00263094785655132,
0.00900394444985275));
#43868=CARTESIAN_POINT('Ctrl Pts',(-0.207134211351354,0.00265460158472104,
0.00900851090477576));
#43869=CARTESIAN_POINT('Ctrl Pts',(-0.207142776523973,0.00266590395548275,
0.00900889219077089));
#43870=CARTESIAN_POINT('Ctrl Pts',(-0.207159130351548,0.00269000365493396,
0.00900530727549867));
#43871=CARTESIAN_POINT('Ctrl Pts',(-0.20716623750744,0.00270207623203594,
0.00900101040587168));
#43872=CARTESIAN_POINT('Ctrl Pts',(-0.207174869590674,0.00271986271764353,
0.0089904581290781));
#43873=CARTESIAN_POINT('Ctrl Pts',(-0.20717755046045,0.00272640706578969,
0.00898543882878451));
#43874=CARTESIAN_POINT('Ctrl Pts',(-0.207181023031312,0.00273773927407138,
0.00897407515034856));
#43875=CARTESIAN_POINT('Ctrl Pts',(-0.207181941566556,0.00274252203293754,
0.00896802941304953));
#43876=CARTESIAN_POINT('Ctrl Pts',(-0.207182068536114,0.00274658618351931,
0.0089614051446851));
#43877=CARTESIAN_POINT('Ctrl Pts',(-0.207097776915989,0.00750000158973935,
0.010288431808782));
#43878=CARTESIAN_POINT('Ctrl Pts',(-0.207097615449255,0.00750000150078048,
0.010294896926047));
#43879=CARTESIAN_POINT('Ctrl Pts',(-0.207096824768248,0.00750000127095302,
0.0103013308258036));
#43880=CARTESIAN_POINT('Ctrl Pts',(-0.207093899892511,0.00750000049420602,
0.0103144379848226));
#43881=CARTESIAN_POINT('Ctrl Pts',(-0.207091675856147,0.00749999992679673,
0.010321054956798));
#43882=CARTESIAN_POINT('Ctrl Pts',(-0.207083424988614,0.00749999783641234,
0.0103391027987811));
#43883=CARTESIAN_POINT('Ctrl Pts',(-0.207075851344921,0.00749999594507674,
0.0103496706025116));
#43884=CARTESIAN_POINT('Ctrl Pts',(-0.207057112101686,0.00749999098558329,
0.010367363790383));
#43885=CARTESIAN_POINT('Ctrl Pts',(-0.207046120079705,0.00749998813306785,
0.0103743223145231));
#43886=CARTESIAN_POINT('Ctrl Pts',(-0.207022666561015,0.00749997979926175,
0.0103834940223032));
#43887=CARTESIAN_POINT('Ctrl Pts',(-0.207011609070574,0.00749999733979672,
0.010385407894664));
#43888=CARTESIAN_POINT('Ctrl Pts',(-0.206999678146928,0.00749994229578302,
0.0103859299553424));
#43889=CARTESIAN_POINT('Ctrl Pts',(-0.206997332525893,0.00749998053119276,
0.0103859550031861));
#43890=CARTESIAN_POINT('Ctrl Pts',(-0.206995167637369,0.00749998003531992,
0.0103859062510846));
#43891=CARTESIAN_POINT('Ctrl Pts',(-0.207261886265387,0.0127551146813286,
0.00863509390574996));
#43892=CARTESIAN_POINT('Ctrl Pts',(-0.207261035868668,0.0128159573149126,
0.00872217657099504));
#43893=CARTESIAN_POINT('Ctrl Pts',(-0.207155887419512,0.0128226349039402,
0.0087085012780755));
#43894=CARTESIAN_POINT('Ctrl Pts',(-0.207125087189744,0.0119178974994294,
0.00921790212244517));
#43895=CARTESIAN_POINT('Ctrl Pts',(-0.207123991865616,0.011969232742892,
0.00931169547144037));
#43896=CARTESIAN_POINT('Ctrl Pts',(-0.20701919820191,0.0119799828515178,
0.00929732829977912));
#43897=CARTESIAN_POINT('Ctrl Pts',(-0.206845110243081,0.0100626154563815,
0.0100931300888338));
#43898=CARTESIAN_POINT('Ctrl Pts',(-0.206843612318736,0.0100920921441639,
0.010197172067879));
#43899=CARTESIAN_POINT('Ctrl Pts',(-0.206736785445693,0.0100908119228757,
0.0101922846257381));
#43900=CARTESIAN_POINT('Ctrl Pts',(-0.207054259433642,0.00800547639790048,
0.0103301544768812));
#43901=CARTESIAN_POINT('Ctrl Pts',(-0.207052661366926,0.00801140287506987,
0.0104369044212851));
#43902=CARTESIAN_POINT('Ctrl Pts',(-0.206947322354661,0.00799994996548187,
0.010429412007676));
#43903=CARTESIAN_POINT('Ctrl Pts',(-0.207143516918877,0.00698371431586357,
0.0102737402097756));
#43904=CARTESIAN_POINT('Ctrl Pts',(-0.207141936092252,0.00697763980344933,
0.0103797958532295));
#43905=CARTESIAN_POINT('Ctrl Pts',(-0.207036365342542,0.00696912440198335,
0.0103712553903634));
#43906=CARTESIAN_POINT('Ctrl Pts',(-0.207181566227228,0.0122501673758382,
0.00896336754694151));
#43907=CARTESIAN_POINT('Ctrl Pts',(-0.207181443529624,0.0122540864740861,
0.00896976251367002));
#43908=CARTESIAN_POINT('Ctrl Pts',(-0.20718058317538,0.012258676661758,
0.00897562162657197));
#43909=CARTESIAN_POINT('Ctrl Pts',(-0.207177335976054,0.0122695128914114,
0.00898667546788692));
#43910=CARTESIAN_POINT('Ctrl Pts',(-0.207174833751635,0.0122757552730441,
0.00899160021002775));
#43911=CARTESIAN_POINT('Ctrl Pts',(-0.207166625261092,0.012293012287366,
0.0090022524895017));
#43912=CARTESIAN_POINT('Ctrl Pts',(-0.207159746438497,0.0123048741518531,
0.00900673653866809));
#43913=CARTESIAN_POINT('Ctrl Pts',(-0.207143242800486,0.0123295060202738,
0.00901094050830801));
#43914=CARTESIAN_POINT('Ctrl Pts',(-0.207134165724431,0.0123415303218528,
0.00901064297181319));
#43915=CARTESIAN_POINT('Ctrl Pts',(-0.207115612578345,0.0123639197185274,
0.00900632226716967));
#43916=CARTESIAN_POINT('Ctrl Pts',(-0.207106180654793,0.0123745726871226,
0.00900226869215929));
#43917=CARTESIAN_POINT('Ctrl Pts',(-0.207094994078381,0.0123853378653371,
0.00899608376006582));
#43918=CARTESIAN_POINT('Ctrl Pts',(-0.20709372520993,0.0123868362173346,
0.00899517010746788));
#43919=CARTESIAN_POINT('Ctrl Pts',(-0.207092315986968,0.012388212238266,
0.00899428849862686));
#43920=CARTESIAN_POINT('Origin',(-0.208345484142396,0.00266244643750944,
0.0089328629507606));
#43921=CARTESIAN_POINT('Ctrl Pts',(-0.208182309222901,0.00274692227615215,
0.00898281378318786));
#43922=CARTESIAN_POINT('Ctrl Pts',(-0.208182277952001,0.00274277083451149,
0.0089894098019654));
#43923=CARTESIAN_POINT('Ctrl Pts',(-0.208183283209678,0.00273793104540203,
0.00899541268676956));
#43924=CARTESIAN_POINT('Ctrl Pts',(-0.208187499969814,0.00272615894310283,
0.00900713179321195));
#43925=CARTESIAN_POINT('Ctrl Pts',(-0.208191025783579,0.00271920742887892,
0.00901236665814065));
#43926=CARTESIAN_POINT('Ctrl Pts',(-0.208202194255079,0.00270086747218974,
0.00902312656656882));
#43927=CARTESIAN_POINT('Ctrl Pts',(-0.20821146643949,0.00268850905365718,
0.00902752167695764));
#43928=CARTESIAN_POINT('Ctrl Pts',(-0.208232757864608,0.00266415672876088,
0.00903124128829879));
#43929=CARTESIAN_POINT('Ctrl Pts',(-0.208243789470648,0.00265295194952518,
0.00903093244186576));
#43930=CARTESIAN_POINT('Ctrl Pts',(-0.208266197965404,0.0026321884360446,
0.00902718224347479));
#43931=CARTESIAN_POINT('Ctrl Pts',(-0.208277625842864,0.00262232779038878,
0.00902366625820533));
#43932=CARTESIAN_POINT('Ctrl Pts',(-0.208291122506059,0.00261230317031573,
0.00901833264904263));
#43933=CARTESIAN_POINT('Ctrl Pts',(-0.208292752737439,0.00261086851622097,
0.00901750864256678));
#43934=CARTESIAN_POINT('Ctrl Pts',(-0.208294498840167,0.00260956111026396,
0.00901672932862339));
#43935=CARTESIAN_POINT('Origin',(-0.207020842672714,0.0123355638655574,
0.00890784819837363));
#43936=CARTESIAN_POINT('Ctrl Pts',(-0.208182119617078,0.0122499879746583,
0.00898468528329885));
#43937=CARTESIAN_POINT('Ctrl Pts',(-0.208182089694991,0.0122540172315659,
0.0089910909843969));
#43938=CARTESIAN_POINT('Ctrl Pts',(-0.208183036687498,0.0122586976544962,
0.00899694045039098));
#43939=CARTESIAN_POINT('Ctrl Pts',(-0.208187017406401,0.0122700585909288,
0.00900839967133868));
#43940=CARTESIAN_POINT('Ctrl Pts',(-0.208190347149437,0.0122767602329116,
0.0090135603977819));
#43941=CARTESIAN_POINT('Ctrl Pts',(-0.208201037604085,0.0122946451894827,
0.00902437981604124));
#43942=CARTESIAN_POINT('Ctrl Pts',(-0.208210017974045,0.0123067937546356,
0.00902891519986445));
#43943=CARTESIAN_POINT('Ctrl Pts',(-0.208230788381485,0.0123308742080499,
0.00903303342014732));
#43944=CARTESIAN_POINT('Ctrl Pts',(-0.208241616538774,0.0123420119266663,
0.00903293626524176));
#43945=CARTESIAN_POINT('Ctrl Pts',(-0.208265385785225,0.0123643383350005,
0.00902936943810583));
#43946=CARTESIAN_POINT('Ctrl Pts',(-0.208277296931519,0.0123741925119681,
0.00902557501439544));
#43947=CARTESIAN_POINT('Ctrl Pts',(-0.208287775341226,0.0123824863977806,
0.00902135349364886));
#43948=CARTESIAN_POINT('Ctrl Pts',(-0.208290484416003,0.0123845498665015,
0.00902027628333439));
#43949=CARTESIAN_POINT('Ctrl Pts',(-0.208293200976528,0.0123865543346131,
0.00901912040146179));
#43950=CARTESIAN_POINT('Ctrl Pts',(-0.208294263946347,0.0123873509824498,
0.0090186459804785));
#43951=CARTESIAN_POINT('Ctrl Pts',(-0.208254768538843,0.00229164450644493,
0.00868658687555039));
#43952=CARTESIAN_POINT('Ctrl Pts',(-0.20825245751503,0.00223391860146863,
0.00877013646409537));
#43953=CARTESIAN_POINT('Ctrl Pts',(-0.208353202742803,0.00224414377019507,
0.00877813922762492));
#43954=CARTESIAN_POINT('Ctrl Pts',(-0.208122384277123,0.00310399998892067,
0.00924699455230831));
#43955=CARTESIAN_POINT('Ctrl Pts',(-0.208119840484776,0.00305516247643459,
0.00933672629287622));
#43956=CARTESIAN_POINT('Ctrl Pts',(-0.208220318667977,0.00306823181203351,
0.00934476558783898));
#43957=CARTESIAN_POINT('Ctrl Pts',(-0.207848303618453,0.00493309708019399,
0.0101100452809943));
#43958=CARTESIAN_POINT('Ctrl Pts',(-0.207845421398244,0.0049048112167105,
0.0102094175693445));
#43959=CARTESIAN_POINT('Ctrl Pts',(-0.207947761301341,0.00490547979792474,
0.010208203470148));
#43960=CARTESIAN_POINT('Ctrl Pts',(-0.208049730569645,0.006951724782394,
0.0103470289032258));
#43961=CARTESIAN_POINT('Ctrl Pts',(-0.208046721415412,0.00694549324445781,
0.0104489865111578));
#43962=CARTESIAN_POINT('Ctrl Pts',(-0.208147746503408,0.00693506629254703,
0.0104497771185207));
#43963=CARTESIAN_POINT('Ctrl Pts',(-0.20813673385937,0.00794205725535903,
0.0103001245699642));
#43964=CARTESIAN_POINT('Ctrl Pts',(-0.208133744121088,0.00794698726026996,
0.0104015414775745));
#43965=CARTESIAN_POINT('Ctrl Pts',(-0.208234946083908,0.00793834125015301,
0.0104033834628677));
#43966=CARTESIAN_POINT('Ctrl Pts',(-0.208097498904532,0.00750000157090282,
0.0103107897516593));
#43967=CARTESIAN_POINT('Ctrl Pts',(-0.208097350998533,0.00750000147467617,
0.0103173344020294));
#43968=CARTESIAN_POINT('Ctrl Pts',(-0.208097848642823,0.00750000152421671,
0.0103238773537081));
#43969=CARTESIAN_POINT('Ctrl Pts',(-0.208100192198594,0.00750000191733527,
0.0103371809375536));
#43970=CARTESIAN_POINT('Ctrl Pts',(-0.208102115151153,0.00750000227840782,
0.0103438916765363));
#43971=CARTESIAN_POINT('Ctrl Pts',(-0.208109542727457,0.00750000372441253,
0.0103622940444594));
#43972=CARTESIAN_POINT('Ctrl Pts',(-0.208116631669298,0.00750000515796395,
0.0103731932565404));
#43973=CARTESIAN_POINT('Ctrl Pts',(-0.208134553438137,0.00750000867236801,
0.0103917150014214));
#43974=CARTESIAN_POINT('Ctrl Pts',(-0.20814522042124,0.00750001081833758,
0.0103991629677472));
#43975=CARTESIAN_POINT('Ctrl Pts',(-0.208167136522622,0.00750001403039175,
0.0104088962499627));
#43976=CARTESIAN_POINT('Ctrl Pts',(-0.208177933155013,0.00750003110817561,
0.0104116848717577));
#43977=CARTESIAN_POINT('Ctrl Pts',(-0.208191146075881,0.00750000062131712,
0.0104128614042931));
#43978=CARTESIAN_POINT('Ctrl Pts',(-0.208193399877725,0.00750002349787222,
0.0104129869823138));
#43979=CARTESIAN_POINT('Ctrl Pts',(-0.208195607365359,0.00750002403881075,
0.0104130368945439));
#43980=CARTESIAN_POINT('Ctrl Pts',(-0.208129717403001,0.00713943526630543,
0.0103043208883982));
#43981=CARTESIAN_POINT('Ctrl Pts',(-0.208127433729327,0.00713551312926382,
0.0104050179882739));
#43982=CARTESIAN_POINT('Ctrl Pts',(-0.208227838903267,0.00714426099060607,
0.0104068541862071));
#43983=CARTESIAN_POINT('Ctrl Pts',(-0.208043973659639,0.00810286960191034,
0.0103409197394026));
#43984=CARTESIAN_POINT('Ctrl Pts',(-0.208041674140705,0.00810972080058238,
0.0104420318495822));
#43985=CARTESIAN_POINT('Ctrl Pts',(-0.208141951845999,0.0081198345803917,
0.0104428483686937));
#43986=CARTESIAN_POINT('Ctrl Pts',(-0.207854652784077,0.0100593757296637,
0.010103906718878));
#43987=CARTESIAN_POINT('Ctrl Pts',(-0.207852485956685,0.01008736209812,
0.010202440838558));
#43988=CARTESIAN_POINT('Ctrl Pts',(-0.207953993445674,0.0100865744749508,
0.0102015120896318));
#43989=CARTESIAN_POINT('Ctrl Pts',(-0.208115460371667,0.0118454327588012,
0.00927136703343939));
#43990=CARTESIAN_POINT('Ctrl Pts',(-0.208113606081108,0.0118932388858219,
0.0093607345340023));
#43991=CARTESIAN_POINT('Ctrl Pts',(-0.20821336750236,0.011880714719645,
0.00936851289219113));
#43992=CARTESIAN_POINT('Ctrl Pts',(-0.208243338997617,0.0126380043079271,
0.00873539247773069));
#43993=CARTESIAN_POINT('Ctrl Pts',(-0.208241707494196,0.0126944515532892,
0.00881888793575907));
#43994=CARTESIAN_POINT('Ctrl Pts',(-0.20834166317492,0.0126841741346925,
0.00882686968717256));
#43995=CARTESIAN_POINT('Ctrl Pts',(-0.20914253069387,0.00800768546079551,
0.0103201868919279));
#43996=CARTESIAN_POINT('Ctrl Pts',(-0.209140158727521,0.00801370758595218,
0.0104254987444665));
#43997=CARTESIAN_POINT('Ctrl Pts',(-0.209035328314277,0.00802224413564764,
0.0104169409854339));
#43998=CARTESIAN_POINT('Ctrl Pts',(-0.209052502335453,0.00698800171825145,
0.0103753680037525));
#43999=CARTESIAN_POINT('Ctrl Pts',(-0.209050115505252,0.00698210423024609,
0.0104813658057015));
#44000=CARTESIAN_POINT('Ctrl Pts',(-0.20894551118575,0.00699356179921356,
0.0104738686489309));
#44001=CARTESIAN_POINT('Ctrl Pts',(-0.20884391279819,0.00493657161352178,
0.010138368073117));
#44002=CARTESIAN_POINT('Ctrl Pts',(-0.208841613705275,0.00490719070191681,
0.0102416870201151));
#44003=CARTESIAN_POINT('Ctrl Pts',(-0.208735525137882,0.0049083303013487,
0.0102367321435203));
#44004=CARTESIAN_POINT('Ctrl Pts',(-0.209126397964456,0.00307771249090385,
0.00925753373586065));
#44005=CARTESIAN_POINT('Ctrl Pts',(-0.209124514363621,0.00302640308937374,
0.00935049596620794));
#44006=CARTESIAN_POINT('Ctrl Pts',(-0.209020453031246,0.00301578732888502,
0.0093361236084367));
#44007=CARTESIAN_POINT('Ctrl Pts',(-0.209262833615147,0.00224487032025302,
0.00867419277172518));
#44008=CARTESIAN_POINT('Ctrl Pts',(-0.209261189107054,0.00218416846403701,
0.00876046668203946));
#44009=CARTESIAN_POINT('Ctrl Pts',(-0.209156773635649,0.00217758333808884,
0.00874678629964514));
#44010=CARTESIAN_POINT('Ctrl Pts',(-0.209093315567622,0.00261035486184449,
0.0090330700905398));
#44011=CARTESIAN_POINT('Ctrl Pts',(-0.209094120821064,0.00261114070661801,
0.00903357611206334));
#44012=CARTESIAN_POINT('Ctrl Pts',(-0.209096239518301,0.00261316568678703,
0.00903484434778787));
#44013=CARTESIAN_POINT('Ctrl Pts',(-0.209098350289981,0.00261524780172148,
0.00903603028854842));
#44014=CARTESIAN_POINT('Ctrl Pts',(-0.209105547676708,0.00262266893378366,
0.00904014786330693));
#44015=CARTESIAN_POINT('Ctrl Pts',(-0.209115105486559,0.00263276396907685,
0.00904479212974383));
#44016=CARTESIAN_POINT('Ctrl Pts',(-0.209134673402525,0.00265642100159974,
0.00904940747341608));
#44017=CARTESIAN_POINT('Ctrl Pts',(-0.209143238710959,0.00266772421138318,
0.00904981136009591));
#44018=CARTESIAN_POINT('Ctrl Pts',(-0.209159593323108,0.0026918341576449,
0.00904627431702745));
#44019=CARTESIAN_POINT('Ctrl Pts',(-0.209166700895917,0.00270391634463159,
0.0090420012009457));
#44020=CARTESIAN_POINT('Ctrl Pts',(-0.209175333936052,0.00272172484600436,
0.00903148343667792));
#44021=CARTESIAN_POINT('Ctrl Pts',(-0.209178015309464,0.00272827965420737,
0.00902647642775316));
#44022=CARTESIAN_POINT('Ctrl Pts',(-0.209181488583474,0.00273963457004301,
0.00901513347071432));
#44023=CARTESIAN_POINT('Ctrl Pts',(-0.209182407362429,0.00274442903389408,
0.00900909632180704));
#44024=CARTESIAN_POINT('Ctrl Pts',(-0.209182534463097,0.0027485057034167,
0.00900247906972172));
#44025=CARTESIAN_POINT('Ctrl Pts',(-0.209097174476702,0.00750003461914674,
0.0103336083237276));
#44026=CARTESIAN_POINT('Ctrl Pts',(-0.209097013644898,0.00750003454899016,
0.0103400777327138));
#44027=CARTESIAN_POINT('Ctrl Pts',(-0.209096222702432,0.00750003434545369,
0.010346515921967));
#44028=CARTESIAN_POINT('Ctrl Pts',(-0.20909329636813,0.00750003363702495,
0.0103596276713648));
#44029=CARTESIAN_POINT('Ctrl Pts',(-0.209091071837928,0.00750003311269133,
0.0103662450459666));
#44030=CARTESIAN_POINT('Ctrl Pts',(-0.209082819421827,0.00750003116198735,
0.0103842933115514));
#44031=CARTESIAN_POINT('Ctrl Pts',(-0.209075244663783,0.00750002938167454,
0.0103948609074878));
#44032=CARTESIAN_POINT('Ctrl Pts',(-0.209056503078323,0.00750002464315622,
0.0104125535831743));
#44033=CARTESIAN_POINT('Ctrl Pts',(-0.209045509769346,0.00750002191516809,
0.0104195117091797));
#44034=CARTESIAN_POINT('Ctrl Pts',(-0.209021617401814,0.00750001345630346,
0.0104288533084413));
#44035=CARTESIAN_POINT('Ctrl Pts',(-0.209010431787089,0.00750003042004547,
0.0104306206808396));
#44036=CARTESIAN_POINT('Ctrl Pts',(-0.208999076913879,0.00749997330983711,
0.0104311172901319));
#44037=CARTESIAN_POINT('Ctrl Pts',(-0.208996706739788,0.00750001530311512,
0.0104311425771752));
#44038=CARTESIAN_POINT('Ctrl Pts',(-0.208994553969907,0.00750001483683845,
0.0104310940718314));
#44039=CARTESIAN_POINT('Ctrl Pts',(-0.209262779834381,0.0127530221952519,
0.00867490352571389));
#44040=CARTESIAN_POINT('Ctrl Pts',(-0.209261907724246,0.0128139114200784,
0.00876165882827295));
#44041=CARTESIAN_POINT('Ctrl Pts',(-0.209156981788614,0.012820678596178,
0.00874817825753072));
#44042=CARTESIAN_POINT('Ctrl Pts',(-0.209126646748533,0.0119169803293661,
0.00925954195823561));
#44043=CARTESIAN_POINT('Ctrl Pts',(-0.209125531306061,0.0119683694124045,
0.00935303445838102));
#44044=CARTESIAN_POINT('Ctrl Pts',(-0.209020958517736,0.0119791049845719,
0.0093388928112537));
#44045=CARTESIAN_POINT('Ctrl Pts',(-0.208844099307297,0.0100626751446717,
0.0101376946082389));
#44046=CARTESIAN_POINT('Ctrl Pts',(-0.208842582846295,0.0100921812902052,
0.0102414874601498));
#44047=CARTESIAN_POINT('Ctrl Pts',(-0.208735979740018,0.0100913135780991,
0.0102367496736839));
#44048=CARTESIAN_POINT('Ctrl Pts',(-0.209052615735226,0.00800535755099375,
0.0103754827269987));
#44049=CARTESIAN_POINT('Ctrl Pts',(-0.20905100004752,0.00801128846267801,
0.0104819939673908));
#44050=CARTESIAN_POINT('Ctrl Pts',(-0.208945895941917,0.00799967234605693,
0.0104747668175588));
#44051=CARTESIAN_POINT('Ctrl Pts',(-0.209143634222637,0.00698384875614079,
0.0103189178445225));
#44052=CARTESIAN_POINT('Ctrl Pts',(-0.20914203548401,0.00697776519261641,
0.0104247315141036));
#44053=CARTESIAN_POINT('Ctrl Pts',(-0.209036698006323,0.00696916149533664,
0.0104164133964875));
#44054=CARTESIAN_POINT('Ctrl Pts',(-0.209182644409035,0.0122486795278824,
0.00900419949295514));
#44055=CARTESIAN_POINT('Ctrl Pts',(-0.209182521643671,0.0122526095831882,
0.00901058504921382));
#44056=CARTESIAN_POINT('Ctrl Pts',(-0.209181661669861,0.0122572093094837,
0.0090164338194715));
#44057=CARTESIAN_POINT('Ctrl Pts',(-0.209178416135399,0.0122680624431654,
0.00902746434418135));
#44058=CARTESIAN_POINT('Ctrl Pts',(-0.209175915285084,0.012274311695359,
0.00903237634726934));
#44059=CARTESIAN_POINT('Ctrl Pts',(-0.209167710129561,0.0122915844470447,
0.00904299633559153));
#44060=CARTESIAN_POINT('Ctrl Pts',(-0.209160833161763,0.0123034529544618,
0.00904745920985657));
#44061=CARTESIAN_POINT('Ctrl Pts',(-0.209144368242992,0.0123280371679506,
0.00905161116321708));
#44062=CARTESIAN_POINT('Ctrl Pts',(-0.209135335915253,0.0123400083561572,
0.00905130441416833));
#44063=CARTESIAN_POINT('Ctrl Pts',(-0.209112342658012,0.0123677708343673,
0.00904594077689228));
#44064=CARTESIAN_POINT('Ctrl Pts',(-0.209101177031499,0.0123789797724797,
0.00903949015665347));
#44065=CARTESIAN_POINT('Ctrl Pts',(-0.209096245091944,0.0123837538311807,
0.0090367533421206));
#44066=CARTESIAN_POINT('Ctrl Pts',(-0.209094881900175,0.0123853276342592,
0.00903579255933166));
#44067=CARTESIAN_POINT('Ctrl Pts',(-0.209093388609595,0.0123867838297658,
0.00903485559890448));
#44068=CARTESIAN_POINT('Origin',(-0.210345958636625,0.00266466447152654,
0.00897396025668633));
#44069=CARTESIAN_POINT('Ctrl Pts',(-0.210183018258064,0.00274902051429104,
0.00902403655092187));
#44070=CARTESIAN_POINT('Ctrl Pts',(-0.210182986078409,0.00274485631500351,
0.00903062764218945));
#44071=CARTESIAN_POINT('Ctrl Pts',(-0.210183991131823,0.00274000451982491,
0.00903662419786442));
#44072=CARTESIAN_POINT('Ctrl Pts',(-0.210188207874478,0.00272821082078781,
0.00904832417145669));
#44073=CARTESIAN_POINT('Ctrl Pts',(-0.210191733117001,0.00272125100204574,
0.00905354691312546));
#44074=CARTESIAN_POINT('Ctrl Pts',(-0.210202900403688,0.00270289424632346,
0.0090642756442902));
#44075=CARTESIAN_POINT('Ctrl Pts',(-0.210212171803793,0.00269052988924587,
0.0090686500280575));
#44076=CARTESIAN_POINT('Ctrl Pts',(-0.210233488109546,0.00266614464063956,
0.00907233386721743));
#44077=CARTESIAN_POINT('Ctrl Pts',(-0.210244550889318,0.00265491334574057,
0.00907200029364349));
#44078=CARTESIAN_POINT('Ctrl Pts',(-0.210273032995874,0.00262854735965918,
0.00906716900269468));
#44079=CARTESIAN_POINT('Ctrl Pts',(-0.210287082514763,0.00261786366084564,
0.00906121416973908));
#44080=CARTESIAN_POINT('Ctrl Pts',(-0.210291941494424,0.00261427253208097,
0.00905928867009177));
#44081=CARTESIAN_POINT('Ctrl Pts',(-0.210293509512885,0.00261287915022715,
0.00905848296687824));
#44082=CARTESIAN_POINT('Ctrl Pts',(-0.210295198244815,0.0026116162614646,
0.00905772710662984));
#44083=CARTESIAN_POINT('Origin',(-0.209022184336501,0.0123339684657499,
0.00894852096435255));
#44084=CARTESIAN_POINT('Ctrl Pts',(-0.210183435338165,0.0122485460076652,
0.00902552908127326));
#44085=CARTESIAN_POINT('Ctrl Pts',(-0.210183404672864,0.0122525882063418,
0.00903192950713903));
#44086=CARTESIAN_POINT('Ctrl Pts',(-0.210184351646517,0.0122572809704391,
0.00903777213926606));
#44087=CARTESIAN_POINT('Ctrl Pts',(-0.21018833291572,0.0122686650660501,
0.00904921147354004));
#44088=CARTESIAN_POINT('Ctrl Pts',(-0.21019166268256,0.0122753763527015,
0.00905435951685488));
#44089=CARTESIAN_POINT('Ctrl Pts',(-0.210202353382174,0.0122932818182202,
0.00906514542427994));
#44090=CARTESIAN_POINT('Ctrl Pts',(-0.210211334152892,0.0123054392161153,
0.00906965808582159));
#44091=CARTESIAN_POINT('Ctrl Pts',(-0.210232105195764,0.0123295279541306,
0.00907373115597808));
#44092=CARTESIAN_POINT('Ctrl Pts',(-0.210242933631105,0.0123406657908483,
0.0090736130899169));
#44093=CARTESIAN_POINT('Ctrl Pts',(-0.210266698853524,0.0123629818522671,
0.00907000489842172));
#44094=CARTESIAN_POINT('Ctrl Pts',(-0.21027859935186,0.0123728221870957,
0.00906619671479487));
#44095=CARTESIAN_POINT('Ctrl Pts',(-0.21028910046586,0.0123811241479557,
0.00906195160088883));
#44096=CARTESIAN_POINT('Ctrl Pts',(-0.210291801841148,0.0123831802714617,
0.00906087284311615));
#44097=CARTESIAN_POINT('Ctrl Pts',(-0.210294510886685,0.0123851780658678,
0.0090597161082102));
#44098=CARTESIAN_POINT('Ctrl Pts',(-0.210295581644675,0.0123859796838815,
0.00905923666941981));
#44099=CARTESIAN_POINT('Ctrl Pts',(-0.210235728831914,0.00241507780074195,
0.00880998116420352));
#44100=CARTESIAN_POINT('Ctrl Pts',(-0.210234071406577,0.00235904669073682,
0.00889370041917784));
#44101=CARTESIAN_POINT('Ctrl Pts',(-0.210333962911911,0.00236943696297074,
0.00890175177268792));
#44102=CARTESIAN_POINT('Ctrl Pts',(-0.210110088197621,0.00319578551215262,
0.00933201998592346));
#44103=CARTESIAN_POINT('Ctrl Pts',(-0.210108215185178,0.00314830174918374,
0.00942147779615604));
#44104=CARTESIAN_POINT('Ctrl Pts',(-0.210207963690016,0.00316052625529352,
0.00942914090505225));
#44105=CARTESIAN_POINT('Ctrl Pts',(-0.209858705116303,0.00493729344559936,
0.0101400029770193));
#44106=CARTESIAN_POINT('Ctrl Pts',(-0.209856530969995,0.00490918845389919,
0.010238384157586));
#44107=CARTESIAN_POINT('Ctrl Pts',(-0.209957959507333,0.0049101000603546,
0.0102376501196028));
#44108=CARTESIAN_POINT('Ctrl Pts',(-0.210038519626352,0.00685239975317306,
0.0103808740076419));
#44109=CARTESIAN_POINT('Ctrl Pts',(-0.21003621314574,0.00684503735312283,
0.0104818812876138));
#44110=CARTESIAN_POINT('Ctrl Pts',(-0.210136464709093,0.00683510449030559,
0.0104827068374165));
#44111=CARTESIAN_POINT('Ctrl Pts',(-0.210123396348251,0.00779507013823767,
0.0103517138661237));
#44112=CARTESIAN_POINT('Ctrl Pts',(-0.210121102243751,0.00779827092525759,
0.0104523876710869));
#44113=CARTESIAN_POINT('Ctrl Pts',(-0.210221446144753,0.00778939338474545,
0.0104542160251016));
#44114=CARTESIAN_POINT('Ctrl Pts',(-0.210096835005399,0.00750005701517807,
0.0103559762949856));
#44115=CARTESIAN_POINT('Ctrl Pts',(-0.210096687094351,0.00750005694619478,
0.0103625212097521));
#44116=CARTESIAN_POINT('Ctrl Pts',(-0.2100971848396,0.00750005699373978,
0.0103690644157446));
#44117=CARTESIAN_POINT('Ctrl Pts',(-0.21009952881361,0.00750005732184499,
0.0103823685377432));
#44118=CARTESIAN_POINT('Ctrl Pts',(-0.210101452102109,0.00750005761622642,
0.0103890795293896));
#44119=CARTESIAN_POINT('Ctrl Pts',(-0.210108880803097,0.00750005877942611,
0.0104074822535115));
#44120=CARTESIAN_POINT('Ctrl Pts',(-0.210115970621333,0.00750005992136825,
0.0104183813798077));
#44121=CARTESIAN_POINT('Ctrl Pts',(-0.210133894274973,0.00750006265497224,
0.0104369029164948));
#44122=CARTESIAN_POINT('Ctrl Pts',(-0.210144562324342,0.00750006432698296,
0.0104443506765333));
#44123=CARTESIAN_POINT('Ctrl Pts',(-0.210166482013843,0.0075000664469057,
0.0104540843436323));
#44124=CARTESIAN_POINT('Ctrl Pts',(-0.210177278956079,0.00750008423230304,
0.0104568718346631));
#44125=CARTESIAN_POINT('Ctrl Pts',(-0.210190486034838,0.00750005044434054,
0.0104580479112367));
#44126=CARTESIAN_POINT('Ctrl Pts',(-0.210192746853844,0.0075000750390866,
0.0104581738820239));
#44127=CARTESIAN_POINT('Ctrl Pts',(-0.210194951359283,0.00750007548126885,
0.0104582237389144));
#44128=CARTESIAN_POINT('Ctrl Pts',(-0.210122793732566,0.0072130985215446,
0.0103519917672711));
#44129=CARTESIAN_POINT('Ctrl Pts',(-0.210120511886917,0.00720999322852045,
0.0104525810605786));
#44130=CARTESIAN_POINT('Ctrl Pts',(-0.210220762860161,0.00721890481119139,
0.0104544782767662));
#44131=CARTESIAN_POINT('Ctrl Pts',(-0.210037720781374,0.00815258917703958,
0.0103800527152135));
#44132=CARTESIAN_POINT('Ctrl Pts',(-0.210035427035482,0.00816000131863083,
0.0104809628804394));
#44133=CARTESIAN_POINT('Ctrl Pts',(-0.210135589792883,0.00816995626869976,
0.0104818539938396));
#44134=CARTESIAN_POINT('Ctrl Pts',(-0.209859677707026,0.0100577432524158,
0.0101407613056068));
#44135=CARTESIAN_POINT('Ctrl Pts',(-0.209857515480827,0.0100857673151341,
0.0102390654985703));
#44136=CARTESIAN_POINT('Ctrl Pts',(-0.209958847930015,0.01008472544421,
0.0102384646295444));
#44137=CARTESIAN_POINT('Ctrl Pts',(-0.210110429917104,0.0117990274139096,
0.00933430221347137));
#44138=CARTESIAN_POINT('Ctrl Pts',(-0.210108568093871,0.0118464108462543,
0.00942370750730259));
#44139=CARTESIAN_POINT('Ctrl Pts',(-0.210208238820813,0.0118343155306104,
0.00943138597517952));
#44140=CARTESIAN_POINT('Ctrl Pts',(-0.210234836619464,0.0125753775929816,
0.00881634681983917));
#44141=CARTESIAN_POINT('Ctrl Pts',(-0.210233188506976,0.012631254401039,
0.00890006330818432));
#44142=CARTESIAN_POINT('Ctrl Pts',(-0.210332995760394,0.0126209274539493,
0.00890814505908907));
#44143=CARTESIAN_POINT('Ctrl Pts',(-0.193150248578096,0.002155718567371,
0.00842869397060042));
#44144=CARTESIAN_POINT('Ctrl Pts',(-0.193256283550229,0.00216190824138389,
0.00844307130174834));
#44145=CARTESIAN_POINT('Ctrl Pts',(-0.193257164103685,0.00222199064266424,
0.00835431756888208));
#44146=CARTESIAN_POINT('Ctrl Pts',(-0.193012984040365,0.00300714201445438,
0.00900503485649586));
#44147=CARTESIAN_POINT('Ctrl Pts',(-0.193118665659607,0.00301772975659131,
0.0090202174587487));
#44148=CARTESIAN_POINT('Ctrl Pts',(-0.193119801031167,0.0030683347568226,
0.00892498937300423));
#44149=CARTESIAN_POINT('Ctrl Pts',(-0.192745011683614,0.00490686685772646,
0.0098801636284191));
#44150=CARTESIAN_POINT('Ctrl Pts',(-0.192852683475637,0.00490403518209803,
0.00988585649881339));
#44151=CARTESIAN_POINT('Ctrl Pts',(-0.192854234568138,0.00493309436623873,
0.00978079682132178));
#44152=CARTESIAN_POINT('Ctrl Pts',(-0.192955683255973,0.00699520299814787,
0.010111749605735));
#44153=CARTESIAN_POINT('Ctrl Pts',(-0.193061924225102,0.00698430847540474,
0.0101203996272913));
#44154=CARTESIAN_POINT('Ctrl Pts',(-0.193063578454204,0.00699016812253032,
0.0100127282934439));
#44155=CARTESIAN_POINT('Ctrl Pts',(-0.193039146112862,0.00802792285482773,
0.0100554658624458));
#44156=CARTESIAN_POINT('Ctrl Pts',(-0.193145610777312,0.00801970468892787,
0.0100650060203432));
#44157=CARTESIAN_POINT('Ctrl Pts',(-0.193147246517876,0.00801377089926689,
0.00995799710993926));
#44158=CARTESIAN_POINT('Ctrl Pts',(-0.193087906597634,0.00259433621160271,
0.00870850400383643));
#44159=CARTESIAN_POINT('Ctrl Pts',(-0.193088660379233,0.00259507710819496,
0.00870896461926417));
#44160=CARTESIAN_POINT('Ctrl Pts',(-0.193090838197641,0.00259716508697917,
0.00871022994405992));
#44161=CARTESIAN_POINT('Ctrl Pts',(-0.193093007507657,0.00259931370221831,
0.00871140548417046));
#44162=CARTESIAN_POINT('Ctrl Pts',(-0.193099786390759,0.00260636033187971,
0.00871517111274946));
#44163=CARTESIAN_POINT('Ctrl Pts',(-0.193109374534362,0.00261646326772918,
0.00871977795304027));
#44164=CARTESIAN_POINT('Ctrl Pts',(-0.193129347090727,0.00264061390658031,
0.0087240933815241));
#44165=CARTESIAN_POINT('Ctrl Pts',(-0.193137930238211,0.00265191377293256,
0.00872431831244535));
#44166=CARTESIAN_POINT('Ctrl Pts',(-0.193154323635676,0.00267595556989629,
0.00872040298226909));
#44167=CARTESIAN_POINT('Ctrl Pts',(-0.19316144921592,0.00268796736359503,
0.00871594058854767));
#44168=CARTESIAN_POINT('Ctrl Pts',(-0.193170103619306,0.00270560796812055,
0.00870514470897271));
#44169=CARTESIAN_POINT('Ctrl Pts',(-0.193172791808667,0.00271208445690734,
0.00870003504614985));
#44170=CARTESIAN_POINT('Ctrl Pts',(-0.193176272919966,0.00272326292681188,
0.00868851352183221));
#44171=CARTESIAN_POINT('Ctrl Pts',(-0.193177193207206,0.00272796362356798,
0.0086824011184089));
#44172=CARTESIAN_POINT('Ctrl Pts',(-0.193177319394213,0.00273193776376147,
0.00867571960454275));
#44173=CARTESIAN_POINT('Ctrl Pts',(-0.193103854794884,0.00749669679535383,
0.00997223701970883));
#44174=CARTESIAN_POINT('Ctrl Pts',(-0.193103688879779,0.00749669454298784,
0.00997867376305629));
#44175=CARTESIAN_POINT('Ctrl Pts',(-0.193102899462808,0.00749669250460742,
0.00998507923961693));
#44176=CARTESIAN_POINT('Ctrl Pts',(-0.193099982508425,0.00749668876680328,
0.00999815748298232));
#44177=CARTESIAN_POINT('Ctrl Pts',(-0.193097760138914,0.00749668711867432,
0.0100047731041968));
#44178=CARTESIAN_POINT('Ctrl Pts',(-0.193089514503717,0.00749668333127773,
0.0100228195151261));
#44179=CARTESIAN_POINT('Ctrl Pts',(-0.193081944631272,0.00749668200346064,
0.01003338801341));
#44180=CARTESIAN_POINT('Ctrl Pts',(-0.193063213341713,0.00749668173385395,
0.0100510828898264));
#44181=CARTESIAN_POINT('Ctrl Pts',(-0.193052225711713,0.00749668280519559,
0.0100580427360768));
#44182=CARTESIAN_POINT('Ctrl Pts',(-0.19302027734347,0.00749668852449542,
0.010070544244531));
#44183=CARTESIAN_POINT('Ctrl Pts',(-0.193003720397325,0.00749672313589827,
0.0100696729208636));
#44184=CARTESIAN_POINT('Ctrl Pts',(-0.193001721429014,0.00749667300664829,
0.0100696409746475));
#44185=CARTESIAN_POINT('Ctrl Pts',(-0.193001278631462,0.00749669549250376,
0.0100696317309843));
#44186=CARTESIAN_POINT('Ctrl Pts',(-0.193258116673284,0.0127748021146355,
0.00835637632548243));
#44187=CARTESIAN_POINT('Ctrl Pts',(-0.19325734733193,0.0128347753589733,
0.0084450700687607));
#44188=CARTESIAN_POINT('Ctrl Pts',(-0.1931513946487,0.0128410248114817,
0.00843094236671849));
#44189=CARTESIAN_POINT('Ctrl Pts',(-0.193121943698077,0.0119278082044051,
0.00892703216180217));
#44190=CARTESIAN_POINT('Ctrl Pts',(-0.193120919356265,0.011978301925409,
0.00902219357317199));
#44191=CARTESIAN_POINT('Ctrl Pts',(-0.193015313553372,0.0119888536363698,
0.00900729145699337));
#44192=CARTESIAN_POINT('Ctrl Pts',(-0.192856751458538,0.0100615008924823,
0.00978240230173624));
#44193=CARTESIAN_POINT('Ctrl Pts',(-0.192855314176916,0.0100904700801754,
0.00988737015200106));
#44194=CARTESIAN_POINT('Ctrl Pts',(-0.192747750734788,0.0100879112589918,
0.0098818218088034));
#44195=CARTESIAN_POINT('Ctrl Pts',(-0.193063722049803,0.00800347256964883,
0.010013024834604));
#44196=CARTESIAN_POINT('Ctrl Pts',(-0.193062180924944,0.00800926363390783,
0.0101205895545703));
#44197=CARTESIAN_POINT('Ctrl Pts',(-0.192956023165166,0.00799844202683973,
0.0101121707024309));
#44198=CARTESIAN_POINT('Ctrl Pts',(-0.193146983637435,0.00697937055318562,
0.00995750654052233));
#44199=CARTESIAN_POINT('Ctrl Pts',(-0.193145461549892,0.00697337420362424,
0.0100644016451243));
#44200=CARTESIAN_POINT('Ctrl Pts',(-0.193039084458002,0.00696523223500842,
0.0100550890613376));
#44201=CARTESIAN_POINT('Ctrl Pts',(-0.193178854938834,0.0122644745065787,
0.00867785711110863));
#44202=CARTESIAN_POINT('Ctrl Pts',(-0.193178732684009,0.0122683134690069,
0.00868431988905915));
#44203=CARTESIAN_POINT('Ctrl Pts',(-0.193177867248174,0.0122728334582095,
0.00869025340848932));
#44204=CARTESIAN_POINT('Ctrl Pts',(-0.193174598785043,0.0122835448345936,
0.0087014760988186));
#44205=CARTESIAN_POINT('Ctrl Pts',(-0.193172079221637,0.0122897359511657,
0.00870649292851449));
#44206=CARTESIAN_POINT('Ctrl Pts',(-0.193163823813424,0.0123068720960452,
0.00871737792668749));
#44207=CARTESIAN_POINT('Ctrl Pts',(-0.193156912387403,0.0123186810332227,
0.0087220158449302));
#44208=CARTESIAN_POINT('Ctrl Pts',(-0.193140066915631,0.0123436664345626,
0.00872660846703081));
#44209=CARTESIAN_POINT('Ctrl Pts',(-0.193130622805463,0.0123560881528755,
0.00872637846084337));
#44210=CARTESIAN_POINT('Ctrl Pts',(-0.193106574731809,0.0123848966283851,
0.00872085579898184));
#44211=CARTESIAN_POINT('Ctrl Pts',(-0.193094959201527,0.0123966062123334,
0.00871393611643193));
#44212=CARTESIAN_POINT('Ctrl Pts',(-0.193091121761129,0.0123999085096778,
0.00871200439517824));
#44213=CARTESIAN_POINT('Ctrl Pts',(-0.193090627838197,0.0124005744669603,
0.00871160617095989));
#44214=CARTESIAN_POINT('Ctrl Pts',(-0.19308996299534,0.0124014666379723,
0.00871106882775808));
#44215=CARTESIAN_POINT('Ctrl Pts',(-0.193089364511003,0.0124020544162197,
0.00871070376520487));
#44216=CARTESIAN_POINT('Origin',(-0.194340687084312,0.00264715365052573,
0.00864799567634145));
#44217=CARTESIAN_POINT('Ctrl Pts',(-0.194177759801894,0.00273230901719225,
0.00869689124250935));
#44218=CARTESIAN_POINT('Ctrl Pts',(-0.194177734563329,0.00272825679049417,
0.0087035201702409));
#44219=CARTESIAN_POINT('Ctrl Pts',(-0.194178737007743,0.00272351230975779,
0.0087095688792266));
#44220=CARTESIAN_POINT('Ctrl Pts',(-0.194182937678093,0.00271191998453251,
0.00872142829908946));
#44221=CARTESIAN_POINT('Ctrl Pts',(-0.194186453742996,0.00270504337667792,
0.00872675563944484));
#44222=CARTESIAN_POINT('Ctrl Pts',(-0.194197594088965,0.00268685648376357,
0.00873776163623637));
#44223=CARTESIAN_POINT('Ctrl Pts',(-0.194206842940504,0.00267456231482886,
0.00874232351067159));
#44224=CARTESIAN_POINT('Ctrl Pts',(-0.19422845325808,0.00264984454257071,
0.00874644507296066));
#44225=CARTESIAN_POINT('Ctrl Pts',(-0.194239902406931,0.00263823421510073,
0.00874620622855402));
#44226=CARTESIAN_POINT('Ctrl Pts',(-0.194268856357757,0.00261146863134927,
0.00874142573297465));
#44227=CARTESIAN_POINT('Ctrl Pts',(-0.194282924857919,0.00260056732491295,
0.00873542278756813));
#44228=CARTESIAN_POINT('Ctrl Pts',(-0.194287483390899,0.0025974904442716,
0.00873376963576102));
#44229=CARTESIAN_POINT('Ctrl Pts',(-0.194288131908502,0.00259685179335783,
0.00873340705306226));
#44230=CARTESIAN_POINT('Ctrl Pts',(-0.194289003765303,0.00259599649080464,
0.00873291853305801));
#44231=CARTESIAN_POINT('Ctrl Pts',(-0.194289738575767,0.00259544077467718,
0.00873259744100971));
#44232=CARTESIAN_POINT('Origin',(-0.193016773520565,0.0123506084835679,
0.00862353297935073));
#44233=CARTESIAN_POINT('Ctrl Pts',(-0.194178213525151,0.0122641753917418,
0.00869897007119024));
#44234=CARTESIAN_POINT('Ctrl Pts',(-0.19417818900797,0.0122681099513547,
0.00870541070607376));
#44235=CARTESIAN_POINT('Ctrl Pts',(-0.194179133897106,0.0122726998135444,
0.00871130683949189));
#44236=CARTESIAN_POINT('Ctrl Pts',(-0.194183101697783,0.0122838897135974,
0.00872290434119992));
#44237=CARTESIAN_POINT('Ctrl Pts',(-0.194186423814274,0.0122905196648154,
0.00872815483354177));
#44238=CARTESIAN_POINT('Ctrl Pts',(-0.194197091348588,0.0123082547642953,
0.00873921387701456));
#44239=CARTESIAN_POINT('Ctrl Pts',(-0.194206051681268,0.012320338923391,
0.00874391202827635));
#44240=CARTESIAN_POINT('Ctrl Pts',(-0.194226779022762,0.0123443606653273,
0.00874835472895947));
#44241=CARTESIAN_POINT('Ctrl Pts',(-0.194237586866862,0.0123555001763983,
0.00874840789326625));
#44242=CARTESIAN_POINT('Ctrl Pts',(-0.194262383165019,0.012378886469752,
0.00874499443907016));
#44243=CARTESIAN_POINT('Ctrl Pts',(-0.19427464652378,0.012388931904822,
0.00874091634599449));
#44244=CARTESIAN_POINT('Ctrl Pts',(-0.19428359687381,0.012396093564287,
0.00873739094093589));
#44245=CARTESIAN_POINT('Ctrl Pts',(-0.194286369122631,0.0123982203159595,
0.00873632096909965));
#44246=CARTESIAN_POINT('Ctrl Pts',(-0.194289147403157,0.0124002824398107,
0.0087351659660157));
#44247=CARTESIAN_POINT('Ctrl Pts',(-0.194290139287956,0.0124010331447966,
0.00873473267146801));
#44248=CARTESIAN_POINT('Ctrl Pts',(-0.194260506267582,0.00220572340070951,
0.00836167384219302));
#44249=CARTESIAN_POINT('Ctrl Pts',(-0.194258100970628,0.00214777522781843,
0.00844667263238102));
#44250=CARTESIAN_POINT('Ctrl Pts',(-0.194360207871775,0.00215850129660316,
0.00845346577350011));
#44251=CARTESIAN_POINT('Ctrl Pts',(-0.194124326267857,0.00304288389765983,
0.00893183123041262));
#44252=CARTESIAN_POINT('Ctrl Pts',(-0.19412167047553,0.00299397998963251,
0.00902304578615173));
#44253=CARTESIAN_POINT('Ctrl Pts',(-0.194223439496858,0.0030082858629339,
0.00903013800120372));
#44254=CARTESIAN_POINT('Ctrl Pts',(-0.193851172469893,0.00493055345358367,
0.00980700548405018));
#44255=CARTESIAN_POINT('Ctrl Pts',(-0.193848146793342,0.00490256758354324,
0.00990786728226616));
#44256=CARTESIAN_POINT('Ctrl Pts',(-0.193951850968722,0.00490228471229653,
0.00990506238773098));
#44257=CARTESIAN_POINT('Ctrl Pts',(-0.19406447559344,0.007002084092692,
0.0100356201917367));
#44258=CARTESIAN_POINT('Ctrl Pts',(-0.194061323729412,0.00699650921242796,
0.0101389487716742));
#44259=CARTESIAN_POINT('Ctrl Pts',(-0.194163683898811,0.00698641223011458,
0.0101386734868917));
#44260=CARTESIAN_POINT('Ctrl Pts',(-0.194147067815913,0.00802012051698481,
0.00998010568044098));
#44261=CARTESIAN_POINT('Ctrl Pts',(-0.194143940209193,0.00802585838081097,
0.0100828035425696));
#44262=CARTESIAN_POINT('Ctrl Pts',(-0.194246522734699,0.00801753202529335,
0.0100834664650456));
#44263=CARTESIAN_POINT('Ctrl Pts',(-0.194103277573009,0.00749642324651037,
0.00999450835808371));
#44264=CARTESIAN_POINT('Ctrl Pts',(-0.194103129691022,0.00749642071073177,
0.0100010516868068));
#44265=CARTESIAN_POINT('Ctrl Pts',(-0.19410362684754,0.00749641796588605,
0.0100075933642326));
#44266=CARTESIAN_POINT('Ctrl Pts',(-0.194105968382486,0.00749641195276905,
0.0100208942631091));
#44267=CARTESIAN_POINT('Ctrl Pts',(-0.194107889712825,0.00749640867914678,
0.0100276037389201));
#44268=CARTESIAN_POINT('Ctrl Pts',(-0.194115311897938,0.00749639900304797,
0.0100460043878287));
#44269=CARTESIAN_POINT('Ctrl Pts',(-0.194122396681178,0.00749639239915879,
0.0100569040309536));
#44270=CARTESIAN_POINT('Ctrl Pts',(-0.194140309556159,0.00749637928051436,
0.0100754268638114));
#44271=CARTESIAN_POINT('Ctrl Pts',(-0.19415097154416,0.00749637288296616,
0.0100828758665553));
#44272=CARTESIAN_POINT('Ctrl Pts',(-0.1941746012313,0.0074963611503292,
0.0100933764134099));
#44273=CARTESIAN_POINT('Ctrl Pts',(-0.194187727972084,0.00749618054610755,
0.0100963596764324));
#44274=CARTESIAN_POINT('Ctrl Pts',(-0.194200910015988,0.00749636354091595,
0.0100967435529685));
#44275=CARTESIAN_POINT('Ctrl Pts',(-0.194201347570367,0.00749635091189165,
0.0100967541477686));
#44276=CARTESIAN_POINT('Ctrl Pts',(-0.194360528299949,0.0128383615463125,
0.00845560308938517));
#44277=CARTESIAN_POINT('Ctrl Pts',(-0.194258272737925,0.0128491304722729,
0.00844891950105934));
#44278=CARTESIAN_POINT('Ctrl Pts',(-0.194260717158237,0.0127911313733274,
0.00836378093723286));
#44279=CARTESIAN_POINT('Ctrl Pts',(-0.194224114589826,0.0119877834030537,
0.00903232837929657));
#44280=CARTESIAN_POINT('Ctrl Pts',(-0.194122194143984,0.012002116243167,
0.00902535590699909));
#44281=CARTESIAN_POINT('Ctrl Pts',(-0.194124889316599,0.01195318233319,
0.00893399239655918));
#44282=CARTESIAN_POINT('Ctrl Pts',(-0.193953516481441,0.0100921752283048,
0.00990683661153991));
#44283=CARTESIAN_POINT('Ctrl Pts',(-0.193849673625334,0.0100919068339616,
0.0099097432667668));
#44284=CARTESIAN_POINT('Ctrl Pts',(-0.19385274022071,0.0100639398252907,
0.00980872003459304));
#44285=CARTESIAN_POINT('Ctrl Pts',(-0.194164107388867,0.0080066176885033,
0.0101391372864121));
#44286=CARTESIAN_POINT('Ctrl Pts',(-0.194061595152703,0.00799659454517679,
0.0101395100125378));
#44287=CARTESIAN_POINT('Ctrl Pts',(-0.19406478636751,0.00799109269338365,
0.0100360321855207));
#44288=CARTESIAN_POINT('Ctrl Pts',(-0.194246313132581,0.00697484113490648,
0.0100830349322283));
#44289=CARTESIAN_POINT('Ctrl Pts',(-0.194143580799908,0.00696655979783964,
0.0100824785919351));
#44290=CARTESIAN_POINT('Ctrl Pts',(-0.194146747597959,0.00697239106197278,
0.00997964182851975));
#44291=CARTESIAN_POINT('Ctrl Pts',(-0.21314244217965,0.00800704485816821,
0.0104100735882361));
#44292=CARTESIAN_POINT('Ctrl Pts',(-0.213140557332318,0.00801304626172808,
0.010515107812128));
#44293=CARTESIAN_POINT('Ctrl Pts',(-0.213035975570542,0.00802176781725835,
0.0105073159363579));
#44294=CARTESIAN_POINT('Ctrl Pts',(-0.213049378421211,0.00698785896905304,
0.0104654522252342));
#44295=CARTESIAN_POINT('Ctrl Pts',(-0.213047478135136,0.00698188315917987,
0.0105711732503626));
#44296=CARTESIAN_POINT('Ctrl Pts',(-0.212943125098063,0.00699360586976436,
0.0105645191388941));
#44297=CARTESIAN_POINT('Ctrl Pts',(-0.21284235286589,0.00493765989046783,
0.0102271645351171));
#44298=CARTESIAN_POINT('Ctrl Pts',(-0.212840545854496,0.00490818586219254,
0.0103301719884767));
#44299=CARTESIAN_POINT('Ctrl Pts',(-0.212734689125797,0.00490851668823669,
0.0103258556199139));
#44300=CARTESIAN_POINT('Ctrl Pts',(-0.213128996239289,0.00308108542687099,
0.00934123157192873));
#44301=CARTESIAN_POINT('Ctrl Pts',(-0.213127591971784,0.00302966984888558,
0.00943382096925474));
#44302=CARTESIAN_POINT('Ctrl Pts',(-0.213023759867318,0.0030188772658784,
0.00942016390252589));
#44303=CARTESIAN_POINT('Ctrl Pts',(-0.213264189117079,0.00225085884863554,
0.00875478600723178));
#44304=CARTESIAN_POINT('Ctrl Pts',(-0.213263022759027,0.00219003479095467,
0.00884062777732394));
#44305=CARTESIAN_POINT('Ctrl Pts',(-0.21315884015455,0.00218306511806226,
0.00882758561253449));
#44306=CARTESIAN_POINT('Ctrl Pts',(-0.21309502125729,0.00261465160980138,
0.00911535617230443));
#44307=CARTESIAN_POINT('Ctrl Pts',(-0.213095852147055,0.00261546012528567,
0.00911588091549215));
#44308=CARTESIAN_POINT('Ctrl Pts',(-0.213097944988729,0.00261745919854445,
0.00911714133440077));
#44309=CARTESIAN_POINT('Ctrl Pts',(-0.213100030401507,0.00261951332673603,
0.00911832279138069));
#44310=CARTESIAN_POINT('Ctrl Pts',(-0.213107399960229,0.00262708280290663,
0.00912255754016195));
#44311=CARTESIAN_POINT('Ctrl Pts',(-0.213116909534435,0.00263712569580249,
0.00912717772590095));
#44312=CARTESIAN_POINT('Ctrl Pts',(-0.213136390591303,0.00266064930220927,
0.00913185073406218));
#44313=CARTESIAN_POINT('Ctrl Pts',(-0.213144957944981,0.00267194878783946,
0.00913229266932233));
#44314=CARTESIAN_POINT('Ctrl Pts',(-0.213161315291064,0.00269606564430115,
0.00912883668359065));
#44315=CARTESIAN_POINT('Ctrl Pts',(-0.213168423636603,0.00270815996238018,
0.00912460454553612));
#44316=CARTESIAN_POINT('Ctrl Pts',(-0.213177057657863,0.00272600171322136,
0.00911414773088799));
#44317=CARTESIAN_POINT('Ctrl Pts',(-0.213179739287994,0.00273257276596848,
0.0091091633924076));
#44318=CARTESIAN_POINT('Ctrl Pts',(-0.213183213079011,0.00274396560695684,
0.0090978602830844));
#44319=CARTESIAN_POINT('Ctrl Pts',(-0.213184132100665,0.00274878070299104,
0.00909184013117857));
#44320=CARTESIAN_POINT('Ctrl Pts',(-0.213184259448588,0.00275288038367511,
0.00908523762214338));
#44321=CARTESIAN_POINT('Ctrl Pts',(-0.213095881749409,0.00749981308898754,
0.0104239596527637));
#44322=CARTESIAN_POINT('Ctrl Pts',(-0.213095722179992,0.00749981285121825,
0.010430437431427));
#44323=CARTESIAN_POINT('Ctrl Pts',(-0.213094930767734,0.00749981251703481,
0.0104368839919119));
#44324=CARTESIAN_POINT('Ctrl Pts',(-0.213092001729469,0.00749981161579216,
0.0104500045880059));
#44325=CARTESIAN_POINT('Ctrl Pts',(-0.213089776365308,0.00749981103605203,
0.0104566226524584));
#44326=CARTESIAN_POINT('Ctrl Pts',(-0.213081521344629,0.00749980905034941,
0.010474671634648));
#44327=CARTESIAN_POINT('Ctrl Pts',(-0.213073944722568,0.00749980739807012,
0.0104852388781492));
#44328=CARTESIAN_POINT('Ctrl Pts',(-0.213055199228367,0.00749980314047178,
0.0105029306783858));
#44329=CARTESIAN_POINT('Ctrl Pts',(-0.213044203777357,0.00749980079481611,
0.0105098881281539));
#44330=CARTESIAN_POINT('Ctrl Pts',(-0.213021129873168,0.00749979313590021,
0.0105189069191168));
#44331=CARTESIAN_POINT('Ctrl Pts',(-0.213010238547216,0.00749982047260193,
0.0105209461160442));
#44332=CARTESIAN_POINT('Ctrl Pts',(-0.212998855188053,0.0074997539260879,
0.0105214434901032));
#44333=CARTESIAN_POINT('Ctrl Pts',(-0.21299658018429,0.00749977253963051,
0.0105215078747055));
#44334=CARTESIAN_POINT('Ctrl Pts',(-0.212994304312368,0.00749979722059817,
0.0105214917573229));
#44335=CARTESIAN_POINT('Ctrl Pts',(-0.212993242078276,0.00749979705225721,
0.0105214677966727));
#44336=CARTESIAN_POINT('Ctrl Pts',(-0.213265643152316,0.0127494169330871,
0.0087544692044563));
#44337=CARTESIAN_POINT('Ctrl Pts',(-0.21326473253461,0.0128101841803463,
0.00884027806311097));
#44338=CARTESIAN_POINT('Ctrl Pts',(-0.213160591305935,0.0128173325297111,
0.00882751233582958));
#44339=CARTESIAN_POINT('Ctrl Pts',(-0.213130471882447,0.0119156035997271,
0.00934279777846922));
#44340=CARTESIAN_POINT('Ctrl Pts',(-0.213129321865349,0.0119669179384452,
0.0094353728123257));
#44341=CARTESIAN_POINT('Ctrl Pts',(-0.213025528705725,0.0119777956790885,
0.00942203256996151));
#44342=CARTESIAN_POINT('Ctrl Pts',(-0.212843201419264,0.010063046280529,
0.010226865697998));
#44343=CARTESIAN_POINT('Ctrl Pts',(-0.212841654709403,0.0100925082785676,
0.0103298072401898));
#44344=CARTESIAN_POINT('Ctrl Pts',(-0.212735841572136,0.0100925267904534,
0.0103257419102505));
#44345=CARTESIAN_POINT('Ctrl Pts',(-0.21304944510932,0.00800490895468439,
0.0104661698013438));
#44346=CARTESIAN_POINT('Ctrl Pts',(-0.213047801242471,0.00801082470959272,
0.0105718409234886));
#44347=CARTESIAN_POINT('Ctrl Pts',(-0.212943497366402,0.0079990046369987,
0.0105655221405287));
#44348=CARTESIAN_POINT('Ctrl Pts',(-0.213143562589862,0.00698374221754044,
0.0104092444559369));
#44349=CARTESIAN_POINT('Ctrl Pts',(-0.213141935136846,0.006977658566979,
0.0105142134722975));
#44350=CARTESIAN_POINT('Ctrl Pts',(-0.213037396541874,0.00696892923864034,
0.0105067288521001));
#44351=CARTESIAN_POINT('Ctrl Pts',(-0.213185728279609,0.0122462777113575,
0.0090857895003052));
#44352=CARTESIAN_POINT('Ctrl Pts',(-0.213185605522206,0.0122502256407507,
0.00909215008990704));
#44353=CARTESIAN_POINT('Ctrl Pts',(-0.213184747944004,0.0122548388876003,
0.00909797344983545));
#44354=CARTESIAN_POINT('Ctrl Pts',(-0.213181512007441,0.0122657110834179,
0.00910894984843468));
#44355=CARTESIAN_POINT('Ctrl Pts',(-0.213179018878935,0.0122719649390347,
0.00911383454991018));
#44356=CARTESIAN_POINT('Ctrl Pts',(-0.213170832096408,0.0122892521858956,
0.00912439517024284));
#44357=CARTESIAN_POINT('Ctrl Pts',(-0.213163965267044,0.0123011258937518,
0.00912882261041887));
#44358=CARTESIAN_POINT('Ctrl Pts',(-0.213147672649622,0.0123254768658068,
0.00913286791781534));
#44359=CARTESIAN_POINT('Ctrl Pts',(-0.213138835653607,0.0123372160682492,
0.00913257902200331));
#44360=CARTESIAN_POINT('Ctrl Pts',(-0.213117808936497,0.01236268389567,
0.00912776054568632));
#44361=CARTESIAN_POINT('Ctrl Pts',(-0.213107738955393,0.0123731866485371,
0.00912252033124069));
#44362=CARTESIAN_POINT('Ctrl Pts',(-0.213101344146465,0.0123795035575569,
0.00911897238156799));
#44363=CARTESIAN_POINT('Ctrl Pts',(-0.213099219437922,0.0123817001155079,
0.00911770584894932));
#44364=CARTESIAN_POINT('Ctrl Pts',(-0.213097102033634,0.0123838455880542,
0.00911634252929533));
#44365=CARTESIAN_POINT('Ctrl Pts',(-0.21309647053259,0.012384459580252,
0.0091159441211624));
#44366=CARTESIAN_POINT('Origin',(-0.214347662483129,0.00266871923262899,
0.00905620843311971));
#44367=CARTESIAN_POINT('Ctrl Pts',(-0.214184739127859,0.00275296418162114,
0.00910660044517797));
#44368=CARTESIAN_POINT('Ctrl Pts',(-0.214184705167232,0.00274877407735516,
0.00911318294739935));
#44369=CARTESIAN_POINT('Ctrl Pts',(-0.214185710281598,0.0027438969349025,
0.00911916725721471));
#44370=CARTESIAN_POINT('Ctrl Pts',(-0.214189928699547,0.00273205492134834,
0.00913082903422289));
#44371=CARTESIAN_POINT('Ctrl Pts',(-0.214193454323423,0.00272507453530064,
0.0091360264580834));
#44372=CARTESIAN_POINT('Ctrl Pts',(-0.214204622414102,0.00270667397370094,
0.00914668775089928));
#44373=CARTESIAN_POINT('Ctrl Pts',(-0.214213894585907,0.00269428945700686,
0.00915101610138924));
#44374=CARTESIAN_POINT('Ctrl Pts',(-0.214234997941506,0.00267012597954294,
0.0091545717540337));
#44375=CARTESIAN_POINT('Ctrl Pts',(-0.214245806144954,0.00265912295208112,
0.00915424567834094));
#44376=CARTESIAN_POINT('Ctrl Pts',(-0.214271986514769,0.00263479199100398,
0.00914986381913527));
#44377=CARTESIAN_POINT('Ctrl Pts',(-0.214284570577821,0.00262485942138193,
0.00914497748979659));
#44378=CARTESIAN_POINT('Ctrl Pts',(-0.214290934974484,0.00262004427343166,
0.00914244557852087));
#44379=CARTESIAN_POINT('Ctrl Pts',(-0.214293725152539,0.00261783324017151,
0.00914125976115354));
#44380=CARTESIAN_POINT('Ctrl Pts',(-0.214296516354532,0.00261568157392703,
0.00913997117675835));
#44381=CARTESIAN_POINT('Ctrl Pts',(-0.214296908994206,0.00261538838033364,
0.00913979427543505));
#44382=CARTESIAN_POINT('Origin',(-0.213025165970707,0.0123312822178751,
0.0090298267726731));
#44383=CARTESIAN_POINT('Ctrl Pts',(-0.214186464570385,0.0122466727702326,
0.00910686109075036));
#44384=CARTESIAN_POINT('Ctrl Pts',(-0.214186432446519,0.0122507411748032,
0.00911325092952807));
#44385=CARTESIAN_POINT('Ctrl Pts',(-0.214187379505248,0.012255459315398,
0.00911907945239577));
#44386=CARTESIAN_POINT('Ctrl Pts',(-0.214191362266413,0.0122668921338603,
0.00913047768807081));
#44387=CARTESIAN_POINT('Ctrl Pts',(-0.214194692444062,0.0122736244775929,
0.00913559918392179));
#44388=CARTESIAN_POINT('Ctrl Pts',(-0.214205384205187,0.0122915757188726,
0.00914631422887851));
#44389=CARTESIAN_POINT('Ctrl Pts',(-0.214214366271417,0.0123037547460295,
0.00915077847840976));
#44390=CARTESIAN_POINT('Ctrl Pts',(-0.21423513972337,0.0123278689671253,
0.00915475462039644));
#44391=CARTESIAN_POINT('Ctrl Pts',(-0.214245969070987,0.0123390113447535,
0.00915459131747644));
#44392=CARTESIAN_POINT('Ctrl Pts',(-0.214269715947045,0.012361305516168,
0.00915089521639169));
#44393=CARTESIAN_POINT('Ctrl Pts',(-0.214281568601509,0.0123711055205838,
0.00914706836117744));
#44394=CARTESIAN_POINT('Ctrl Pts',(-0.214292171730787,0.0123794661551032,
0.0091427537421371));
#44395=CARTESIAN_POINT('Ctrl Pts',(-0.214294839359734,0.0123814960193334,
0.00914167679027904));
#44396=CARTESIAN_POINT('Ctrl Pts',(-0.21429751482476,0.0123834705158705,
0.00914052487394618));
#44397=CARTESIAN_POINT('Ctrl Pts',(-0.214298620129385,0.012384296620628,
0.00914002647745522));
#44398=CARTESIAN_POINT('Ctrl Pts',(-0.214216754079608,0.00254864162832996,
0.00897659909113701));
#44399=CARTESIAN_POINT('Ctrl Pts',(-0.214215071756275,0.00249383408308367,
0.00906087149037426));
#44400=CARTESIAN_POINT('Ctrl Pts',(-0.214314737987371,0.00250427417561616,
0.00906900710735247));
#44401=CARTESIAN_POINT('Ctrl Pts',(-0.214098711059485,0.00329387750221925,
0.00946040117636586));
#44402=CARTESIAN_POINT('Ctrl Pts',(-0.214096831881102,0.00324728810829633,
0.00955002047493883));
#44403=CARTESIAN_POINT('Ctrl Pts',(-0.214196461482836,0.00325869649582198,
0.00955741154943173));
#44404=CARTESIAN_POINT('Ctrl Pts',(-0.213868831622076,0.00494124278014463,
0.0102135400153998));
#44405=CARTESIAN_POINT('Ctrl Pts',(-0.213866675848953,0.0049130570953545,
0.0103115153730948));
#44406=CARTESIAN_POINT('Ctrl Pts',(-0.213967812670003,0.00491441191731313,
0.0103113549971935));
#44407=CARTESIAN_POINT('Ctrl Pts',(-0.214026111204022,0.00674788150248729,
0.0104576635446883));
#44408=CARTESIAN_POINT('Ctrl Pts',(-0.214023825957855,0.0067393313698133,
0.0105583088393878));
#44409=CARTESIAN_POINT('Ctrl Pts',(-0.214123907054786,0.00672978090006651,
0.0105592295780455));
#44410=CARTESIAN_POINT('Ctrl Pts',(-0.214108479671163,0.00763963123678071,
0.0104455505972963));
#44411=CARTESIAN_POINT('Ctrl Pts',(-0.214106198989655,0.00764109666123514,
0.0105460513513631));
#44412=CARTESIAN_POINT('Ctrl Pts',(-0.214206299904641,0.00763192741742352,
0.0105479200166305));
#44413=CARTESIAN_POINT('Ctrl Pts',(-0.214095599716215,0.00749962544805674,
0.0104463514425309));
#44414=CARTESIAN_POINT('Ctrl Pts',(-0.214095451794398,0.00749962504495062,
0.0104528968860796));
#44415=CARTESIAN_POINT('Ctrl Pts',(-0.214095949743277,0.0074996247400838,
0.0104594406003646));
#44416=CARTESIAN_POINT('Ctrl Pts',(-0.214098294561895,0.00749962431257035,
0.0104727457995799));
#44417=CARTESIAN_POINT('Ctrl Pts',(-0.214100218529235,0.00749962420408635,
0.0104794572967246));
#44418=CARTESIAN_POINT('Ctrl Pts',(-0.214107649508439,0.00749962419724419,
0.0104978607422557));
#44419=CARTESIAN_POINT('Ctrl Pts',(-0.214114741107808,0.00749962456581655,
0.0105087596981603));
#44420=CARTESIAN_POINT('Ctrl Pts',(-0.214132668598254,0.00749962578572488,
0.0105272808258854));
#44421=CARTESIAN_POINT('Ctrl Pts',(-0.214143338822552,0.00749962674612676,
0.0105347281746056));
#44422=CARTESIAN_POINT('Ctrl Pts',(-0.214165265741731,0.00749962751269912,
0.0105444626034586));
#44423=CARTESIAN_POINT('Ctrl Pts',(-0.214176063329797,0.00749964698774914,
0.0105472478399211));
#44424=CARTESIAN_POINT('Ctrl Pts',(-0.214189258751872,0.00749960790352974,
0.01054842300869));
#44425=CARTESIAN_POINT('Ctrl Pts',(-0.214191533580253,0.00749963570601337,
0.0105485497685965));
#44426=CARTESIAN_POINT('Ctrl Pts',(-0.214193732110184,0.00749963608528694,
0.0105485995171194));
#44427=CARTESIAN_POINT('Ctrl Pts',(-0.214099253446307,0.00745991385637808,
0.0104463443855313));
#44428=CARTESIAN_POINT('Ctrl Pts',(-0.214096974871178,0.0074595664991226,
0.0105467469842101));
#44429=CARTESIAN_POINT('Ctrl Pts',(-0.214196963190226,0.00746877681718598,
0.0105486179406832));
#44430=CARTESIAN_POINT('Ctrl Pts',(-0.214020082389909,0.00831894594433586,
0.0104483989904472));
#44431=CARTESIAN_POINT('Ctrl Pts',(-0.21401780385469,0.00832821903762263,
0.0105488339524259));
#44432=CARTESIAN_POINT('Ctrl Pts',(-0.214117811546728,0.00833738824368495,
0.0105498229681975));
#44433=CARTESIAN_POINT('Ctrl Pts',(-0.213876996985919,0.0100520920635664,
0.010205574644505));
#44434=CARTESIAN_POINT('Ctrl Pts',(-0.213874844832131,0.0100801808822668,
0.0103033571540271));
#44435=CARTESIAN_POINT('Ctrl Pts',(-0.213975821734514,0.010078672567526,
0.0103035150590047));
#44436=CARTESIAN_POINT('Ctrl Pts',(-0.2140923557601,0.0116453800387162,
0.00948777426694368));
#44437=CARTESIAN_POINT('Ctrl Pts',(-0.214090467670465,0.0116912347252608,
0.00957760306600306));
#44438=CARTESIAN_POINT('Ctrl Pts',(-0.214190047996671,0.0116802934198075,
0.00958479083026525));
#44439=CARTESIAN_POINT('Ctrl Pts',(-0.214205194686077,0.0123668777182512,
0.00903080634119371));
#44440=CARTESIAN_POINT('Ctrl Pts',(-0.214203492147884,0.0124206946345659,
0.00911558638282872));
#44441=CARTESIAN_POINT('Ctrl Pts',(-0.214303052117812,0.0124102602652885,
0.00912369507589516));
#44442=CARTESIAN_POINT('Ctrl Pts',(-0.223149958381768,0.00811836849261824,
0.0106277848801897));
#44443=CARTESIAN_POINT('Ctrl Pts',(-0.223149017147776,0.00812607888323874,
0.0107379352117485));
#44444=CARTESIAN_POINT('Ctrl Pts',(-0.223039596559705,0.00813431010703398,
0.0107253955357731));
#44445=CARTESIAN_POINT('Ctrl Pts',(-0.223032128491294,0.00689032892248409,
0.0107121280996051));
#44446=CARTESIAN_POINT('Ctrl Pts',(-0.223031160847443,0.006882589693257,
0.0108233580442053));
#44447=CARTESIAN_POINT('Ctrl Pts',(-0.222922016432433,0.00689506675999886,
0.010812206747988));
#44448=CARTESIAN_POINT('Ctrl Pts',(-0.222896076226969,0.00509605881161538,
0.0104620567002983));
#44449=CARTESIAN_POINT('Ctrl Pts',(-0.222895201503254,0.00506652282554446,
0.010570242247404));
#44450=CARTESIAN_POINT('Ctrl Pts',(-0.222784772879459,0.00507057089023076,
0.0105612791384786));
#44451=CARTESIAN_POINT('Ctrl Pts',(-0.223098674012225,0.00282059013172128,
0.00940055961423081));
#44452=CARTESIAN_POINT('Ctrl Pts',(-0.223098301276066,0.00276261015251879,
0.00949549531498266));
#44453=CARTESIAN_POINT('Ctrl Pts',(-0.222989560059633,0.00275270061654399,
0.00947735836584344));
#44454=CARTESIAN_POINT('Ctrl Pts',(-0.223394109819826,0.00185848636376366,
0.00868366986817202));
#44455=CARTESIAN_POINT('Ctrl Pts',(-0.223394052938567,0.00178892652705542,
0.00876990019161811));
#44456=CARTESIAN_POINT('Ctrl Pts',(-0.223287239065902,0.00177559498381319,
0.00874497678071077));
#44457=CARTESIAN_POINT('Ctrl Pts',(-0.223543079689471,0.0013353842698584,
0.00819234018549985));
#44458=CARTESIAN_POINT('Ctrl Pts',(-0.223543219690721,0.00125922959931456,
0.00827238454094328));
#44459=CARTESIAN_POINT('Ctrl Pts',(-0.223435511657072,0.00125080723173669,
0.00824921551534157));
#44460=CARTESIAN_POINT('Ctrl Pts',(-0.223310598482097,0.00172037988617517,
0.00866504379818179));
#44461=CARTESIAN_POINT('Ctrl Pts',(-0.223334018892059,0.00174295523481006,
0.0086842432411052));
#44462=CARTESIAN_POINT('Ctrl Pts',(-0.223347735408989,0.00175981983936743,
0.00868820455961472));
#44463=CARTESIAN_POINT('Ctrl Pts',(-0.223360552734813,0.00178149963234084,
0.00868907076646229));
#44464=CARTESIAN_POINT('Ctrl Pts',(-0.223361712493225,0.00178346129912069,
0.00868914914401873));
#44465=CARTESIAN_POINT('Ctrl Pts',(-0.223362865477419,0.00178547527971709,
0.00868917146628374));
#44466=CARTESIAN_POINT('Ctrl Pts',(-0.223364018586399,0.00178755268391809,
0.00868912731689215));
#44467=CARTESIAN_POINT('Ctrl Pts',(-0.223377915519196,0.00181258895287393,
0.00868859524131362));
#44468=CARTESIAN_POINT('Ctrl Pts',(-0.223391925265875,0.0018448159954703,
0.00867367215760806));
#44469=CARTESIAN_POINT('Ctrl Pts',(-0.223392285502192,0.00186163021866878,
0.00865321401664211));
#44470=CARTESIAN_POINT('Ctrl Pts',(-0.223092856247512,0.00749585351918229,
0.0106501223902346));
#44471=CARTESIAN_POINT('Ctrl Pts',(-0.223092684188288,0.00749585053885153,
0.0106565243090426));
#44472=CARTESIAN_POINT('Ctrl Pts',(-0.223091895251065,0.00749584774490668,
0.0106628947681154));
#44473=CARTESIAN_POINT('Ctrl Pts',(-0.223088984119591,0.00749584238255244,
0.0106759413684013));
#44474=CARTESIAN_POINT('Ctrl Pts',(-0.223086760080309,0.00749583987015413,
0.0106825588960641));
#44475=CARTESIAN_POINT('Ctrl Pts',(-0.223078509782108,0.00749583362413322,
0.0107006067727498));
#44476=CARTESIAN_POINT('Ctrl Pts',(-0.223070937121219,0.00749583072844963,
0.0107111744299137));
#44477=CARTESIAN_POINT('Ctrl Pts',(-0.223052200495654,0.00749582755061298,
0.0107288668954373));
#44478=CARTESIAN_POINT('Ctrl Pts',(-0.223041210292398,0.00749582731204073,
0.0107358251218091));
#44479=CARTESIAN_POINT('Ctrl Pts',(-0.223016508793546,0.00749582944608222,
0.010745485641849));
#44480=CARTESIAN_POINT('Ctrl Pts',(-0.223004129993207,0.00749585232722507,
0.0107474057105056));
#44481=CARTESIAN_POINT('Ctrl Pts',(-0.222992335031057,0.00749582914091336,
0.0107474337334615));
#44482=CARTESIAN_POINT('Ctrl Pts',(-0.222991908351812,0.00749582812340553,
0.0107474317741862));
#44483=CARTESIAN_POINT('Ctrl Pts',(-0.222991328193623,0.00749582309807586,
0.0107474258711083));
#44484=CARTESIAN_POINT('Ctrl Pts',(-0.222991070791995,0.00749582034034479,
0.0107474224622069));
#44485=CARTESIAN_POINT('Ctrl Pts',(-0.222990717313771,0.00749580780121696,
0.0107474166346042));
#44486=CARTESIAN_POINT('Ctrl Pts',(-0.222990358652687,0.00749571058866991,
0.0107474093363226));
#44487=CARTESIAN_POINT('Ctrl Pts',(-0.223038904064572,0.00685832243219836,
0.010724812432214));
#44488=CARTESIAN_POINT('Ctrl Pts',(-0.223148784830004,0.00686647913663685,
0.010737919478636));
#44489=CARTESIAN_POINT('Ctrl Pts',(-0.223149723157941,0.00687431556120157,
0.0106272599439884));
#44490=CARTESIAN_POINT('Ctrl Pts',(-0.222921342326663,0.00809554936511713,
0.0108125078527399));
#44491=CARTESIAN_POINT('Ctrl Pts',(-0.223030951289103,0.00810806473741712,
0.0108242266003475));
#44492=CARTESIAN_POINT('Ctrl Pts',(-0.223031916258244,0.00810040520679048,
0.0107124723755508));
#44493=CARTESIAN_POINT('Ctrl Pts',(-0.222788345558373,0.00991734046137115,
0.010564156394036));
#44494=CARTESIAN_POINT('Ctrl Pts',(-0.222899221435757,0.00992139891278033,
0.0105737275036333));
#44495=CARTESIAN_POINT('Ctrl Pts',(-0.222900094931727,0.00989188064193713,
0.0104649966425086));
#44496=CARTESIAN_POINT('Ctrl Pts',(-0.222991444217135,0.0122334116145978,
0.0094855742606813));
#44497=CARTESIAN_POINT('Ctrl Pts',(-0.223100651811751,0.0122237070864208,
0.00950419456187707));
#44498=CARTESIAN_POINT('Ctrl Pts',(-0.223101021860234,0.0121656229844738,
0.00940871624898466));
#44499=CARTESIAN_POINT('Ctrl Pts',(-0.223292823363305,0.0132097454493491,
0.0087567416927032));
#44500=CARTESIAN_POINT('Ctrl Pts',(-0.223399985861735,0.0131962649911677,
0.008782420408174));
#44501=CARTESIAN_POINT('Ctrl Pts',(-0.223400039587377,0.0131265633700794,
0.00869563825883883));
#44502=CARTESIAN_POINT('Ctrl Pts',(-0.22344293546994,0.0137344903751146,
0.00826334397677012));
#44503=CARTESIAN_POINT('Ctrl Pts',(-0.223551045285294,0.0137261671689852,
0.00828714676645308));
#44504=CARTESIAN_POINT('Ctrl Pts',(-0.223550904301479,0.0136498450124133,
0.00820654686920794));
#44505=CARTESIAN_POINT('Ctrl Pts',(-0.223398239295461,0.0131236886374436,
0.00866523263057392));
#44506=CARTESIAN_POINT('Ctrl Pts',(-0.223398136457366,0.0131285310204962,
0.0086711516106654));
#44507=CARTESIAN_POINT('Ctrl Pts',(-0.223397333177559,0.0131339979980512,
0.00867643268304301));
#44508=CARTESIAN_POINT('Ctrl Pts',(-0.223394275796221,0.0131465321569875,
0.0086860533648667));
#44509=CARTESIAN_POINT('Ctrl Pts',(-0.223391913440977,0.0131535682654236,
0.00869013199620513));
#44510=CARTESIAN_POINT('Ctrl Pts',(-0.223383973147319,0.013173032799877,
0.00869853055476966));
#44511=CARTESIAN_POINT('Ctrl Pts',(-0.223377414256092,0.0131856216462082,
0.00870103929587356));
#44512=CARTESIAN_POINT('Ctrl Pts',(-0.223362537151336,0.0132101069037078,
0.00870155990773004));
#44513=CARTESIAN_POINT('Ctrl Pts',(-0.223354204813562,0.0132219860216964,
0.00869951986497978));
#44514=CARTESIAN_POINT('Ctrl Pts',(-0.223333099159678,0.0132487347662511,
0.0086901514900253));
#44515=CARTESIAN_POINT('Ctrl Pts',(-0.223322907202441,0.0132589745048153,
0.00868212703059623));
#44516=CARTESIAN_POINT('Ctrl Pts',(-0.223319122967919,0.0132624468986076,
0.00867940053158316));
#44517=CARTESIAN_POINT('Ctrl Pts',(-0.223318458580742,0.0132632291985661,
0.00867876926620867));
#44518=CARTESIAN_POINT('Ctrl Pts',(-0.223317571560149,0.0132642671045371,
0.00867791950814091));
#44519=CARTESIAN_POINT('Ctrl Pts',(-0.223316827901763,0.0132649884239581,
0.00867730857776536));
#44520=CARTESIAN_POINT('Origin',(-0.224556024162841,0.00178554708722032,
0.00861247505820972));
#44521=CARTESIAN_POINT('Ctrl Pts',(-0.224391663448231,0.00186170363230323,
0.00867388685638973));
#44522=CARTESIAN_POINT('Ctrl Pts',(-0.224391690962794,0.00185664352167643,
0.00867986565017952));
#44523=CARTESIAN_POINT('Ctrl Pts',(-0.224392856591787,0.00185099742226291,
0.00868513708397277));
#44524=CARTESIAN_POINT('Ctrl Pts',(-0.224397633435892,0.00183756116645332,
0.00869519920844558));
#44525=CARTESIAN_POINT('Ctrl Pts',(-0.224401634564269,0.00182982774161729,
0.00869943878686519));
#44526=CARTESIAN_POINT('Ctrl Pts',(-0.224414113949786,0.00181002423968987,
0.00870751274989629));
#44527=CARTESIAN_POINT('Ctrl Pts',(-0.22442443867922,0.00179707585700994,
0.00871009377290731));
#44528=CARTESIAN_POINT('Ctrl Pts',(-0.224447611009241,0.00177277200820337,
0.00871020581134868));
#44529=CARTESIAN_POINT('Ctrl Pts',(-0.224459249259747,0.00176213704190661,
0.00870838563173362));
#44530=CARTESIAN_POINT('Ctrl Pts',(-0.224487175198716,0.00173924228049195,
0.00870091542899512));
#44531=CARTESIAN_POINT('Ctrl Pts',(-0.224500555793624,0.00173026352267406,
0.0086949372519814));
#44532=CARTESIAN_POINT('Ctrl Pts',(-0.224507687952234,0.00172570160913579,
0.00869169706224443));
#44533=CARTESIAN_POINT('Ctrl Pts',(-0.224510650816698,0.00172372736060054,
0.00869026741305131));
#44534=CARTESIAN_POINT('Ctrl Pts',(-0.224513611096056,0.00172182181281534,
0.00868875013016184));
#44535=CARTESIAN_POINT('Ctrl Pts',(-0.2245141337222,0.00172149608377577,
0.00868848845801025));
#44536=CARTESIAN_POINT('Origin',(-0.223237201119695,0.0132013902797598,
0.00859864717831064));
#44537=CARTESIAN_POINT('Ctrl Pts',(-0.224519290304243,0.0132629343303462,
0.00870151198403918));
#44538=CARTESIAN_POINT('Ctrl Pts',(-0.224519200559076,0.0132626799782016,
0.00870172096410461));
#44539=CARTESIAN_POINT('Ctrl Pts',(-0.224519196449931,0.0132626715913979,
0.00870172780918351));
#44540=CARTESIAN_POINT('Ctrl Pts',(-0.224519188792359,0.0132626563556557,
0.00870174023641345));
#44541=CARTESIAN_POINT('Ctrl Pts',(-0.224519185274485,0.0132626494990939,
0.00870174582616742));
#44542=CARTESIAN_POINT('Ctrl Pts',(-0.224519178967634,0.0132626374476326,
0.0087017556460159));
#44543=CARTESIAN_POINT('Ctrl Pts',(-0.224519176204388,0.0132626322455634,
0.00870175988314548));
#44544=CARTESIAN_POINT('Ctrl Pts',(-0.224519171386791,0.0132626233061751,
0.00870176716154422));
#44545=CARTESIAN_POINT('Ctrl Pts',(-0.224519169349119,0.01326261956404,
0.0087017702075175));
#44546=CARTESIAN_POINT('Ctrl Pts',(-0.224519165865502,0.0132626132308922,
0.00870177536105968));
#44547=CARTESIAN_POINT('Ctrl Pts',(-0.224519164428724,0.0132626106370534,
0.00870177747136503));
#44548=CARTESIAN_POINT('Ctrl Pts',(-0.224519109814946,0.0132625127185912,
0.00870185712094413));
#44549=CARTESIAN_POINT('Ctrl Pts',(-0.224519044966251,0.0132624206026821,
0.00870193150053024));
#44550=CARTESIAN_POINT('Ctrl Pts',(-0.224518723363153,0.0132620216461391,
0.00870225178079486));
#44551=CARTESIAN_POINT('Ctrl Pts',(-0.22451831276061,0.0132616574362571,
0.00870253961290821));
#44552=CARTESIAN_POINT('Ctrl Pts',(-0.224516797031972,0.0132605153113935,
0.0087034170474696));
#44553=CARTESIAN_POINT('Ctrl Pts',(-0.224515575979251,0.0132596901374382,
0.00870402972759247));
#44554=CARTESIAN_POINT('Ctrl Pts',(-0.224510961241942,0.0132565714802701,
0.00870628548407886));
#44555=CARTESIAN_POINT('Ctrl Pts',(-0.224503324979594,0.0132515404150939,
0.0087097732800045));
#44556=CARTESIAN_POINT('Ctrl Pts',(-0.224475263000761,0.0132307277045983,
0.00871981812048934));
#44557=CARTESIAN_POINT('Ctrl Pts',(-0.224458096051566,0.0132156922405316,
0.00872316939171254));
#44558=CARTESIAN_POINT('Ctrl Pts',(-0.224430971986936,0.0131873371827302,
0.00872296615606519));
#44559=CARTESIAN_POINT('Ctrl Pts',(-0.224420615526776,0.0131743978476805,
0.00872035132447665));
#44560=CARTESIAN_POINT('Ctrl Pts',(-0.224408099207843,0.0131546171954294,
0.00871222719279687));
#44561=CARTESIAN_POINT('Ctrl Pts',(-0.224404085463319,0.0131468940503105,
0.00870796860159257));
#44562=CARTESIAN_POINT('Ctrl Pts',(-0.22439929544596,0.0131334846526406,
0.00869787714577718));
#44563=CARTESIAN_POINT('Ctrl Pts',(-0.224398126033773,0.0131278539099209,
0.0086925975449782));
#44564=CARTESIAN_POINT('Ctrl Pts',(-0.224398096309527,0.0131228084948154,
0.00868661304198621));
#44565=CARTESIAN_POINT('Ctrl Pts',(-0.224249357172095,0.00812340187734315,
0.0107538157471281));
#44566=CARTESIAN_POINT('Ctrl Pts',(-0.224146973897669,0.00813179493343109,
0.0107527927564782));
#44567=CARTESIAN_POINT('Ctrl Pts',(-0.224150079053515,0.00812453493531191,
0.0106503798565657));
#44568=CARTESIAN_POINT('Ctrl Pts',(-0.22413240338219,0.00688538717073963,
0.0108391603821318));
#44569=CARTESIAN_POINT('Ctrl Pts',(-0.224030305893638,0.00689634351625541,
0.0108395260737771));
#44570=CARTESIAN_POINT('Ctrl Pts',(-0.224033442754283,0.00690340499464296,
0.0107361019261074));
#44571=CARTESIAN_POINT('Ctrl Pts',(-0.223994325524645,0.00506403357770048,
0.0105862477504909));
#44572=CARTESIAN_POINT('Ctrl Pts',(-0.22389096912139,0.00506508187178619,
0.0105884758775558));
#44573=CARTESIAN_POINT('Ctrl Pts',(-0.223893996001451,0.00509264619037901,
0.010487856035286));
#44574=CARTESIAN_POINT('Ctrl Pts',(-0.224201604501605,0.00275240868515444,
0.00950201908119746));
#44575=CARTESIAN_POINT('Ctrl Pts',(-0.224100039602147,0.00273684373946514,
0.0094938587310791));
#44576=CARTESIAN_POINT('Ctrl Pts',(-0.224102620321083,0.0027912050241893,
0.00940582756518366));
#44577=CARTESIAN_POINT('Ctrl Pts',(-0.224501847843731,0.00177835042191264,
0.00877050099325137));
#44578=CARTESIAN_POINT('Ctrl Pts',(-0.224401973174767,0.00175931878963782,
0.00875562557648048));
#44579=CARTESIAN_POINT('Ctrl Pts',(-0.224404292962857,0.00182452912855932,
0.00867585493377426));
#44580=CARTESIAN_POINT('Ctrl Pts',(-0.224648447652107,0.00125404116273978,
0.00827422479137384));
#44581=CARTESIAN_POINT('Ctrl Pts',(-0.224547784514112,0.00123874181242394,
0.00826029823960483));
#44582=CARTESIAN_POINT('Ctrl Pts',(-0.22454990776902,0.00130997806636779,
0.00818626753716696));
#44583=CARTESIAN_POINT('Ctrl Pts',(-0.224092574620247,0.00749537127813137,
0.0106722901056483));
#44584=CARTESIAN_POINT('Ctrl Pts',(-0.224092426749193,0.00749536783406251,
0.0106788326616221));
#44585=CARTESIAN_POINT('Ctrl Pts',(-0.224092923860089,0.00749536420926534,
0.0106853735535888));
#44586=CARTESIAN_POINT('Ctrl Pts',(-0.224095265168082,0.00749535646538972,
0.0106986729281663));
#44587=CARTESIAN_POINT('Ctrl Pts',(-0.224097186314513,0.00749535235120555,
0.0107053816423148));
#44588=CARTESIAN_POINT('Ctrl Pts',(-0.224104608477795,0.00749534046510422,
0.0107237822010604));
#44589=CARTESIAN_POINT('Ctrl Pts',(-0.224111693885709,0.00749533267179103,
0.0107346822263825));
#44590=CARTESIAN_POINT('Ctrl Pts',(-0.224129608634221,0.00749531781049727,
0.0107532062850313));
#44591=CARTESIAN_POINT('Ctrl Pts',(-0.22414027204642,0.00749531087304268,
0.0107606558993738));
#44592=CARTESIAN_POINT('Ctrl Pts',(-0.224171640221325,0.00749529490524347,
0.0107745952453094));
#44593=CARTESIAN_POINT('Ctrl Pts',(-0.224188233088826,0.0074952638518399,
0.0107744682362007));
#44594=CARTESIAN_POINT('Ctrl Pts',(-0.224190202947882,0.00749531042008945,
0.0107745260061853));
#44595=CARTESIAN_POINT('Ctrl Pts',(-0.224190645755837,0.00749528925575554,
0.0107745367966582));
#44596=CARTESIAN_POINT('Ctrl Pts',(-0.224149812609561,0.00686720535741763,
0.010649790663496));
#44597=CARTESIAN_POINT('Ctrl Pts',(-0.224146711244469,0.00685983841997734,
0.0107523672886193));
#44598=CARTESIAN_POINT('Ctrl Pts',(-0.224249268941159,0.00686819969821718,
0.0107532186162631));
#44599=CARTESIAN_POINT('Ctrl Pts',(-0.224033310137068,0.00808631398537909,
0.0107365279258389));
#44600=CARTESIAN_POINT('Ctrl Pts',(-0.22403017708648,0.00809326520017373,
0.0108401277556867));
#44601=CARTESIAN_POINT('Ctrl Pts',(-0.22413245162769,0.00810418695798438,
0.0108395912055622));
#44602=CARTESIAN_POINT('Ctrl Pts',(-0.2238976842394,0.00989438682845739,
0.0104910133496839));
#44603=CARTESIAN_POINT('Ctrl Pts',(-0.223894659126775,0.00992184394931338,
0.0105918383770759));
#44604=CARTESIAN_POINT('Ctrl Pts',(-0.223998181022725,0.0099227443382153,
0.010589479005002));
#44605=CARTESIAN_POINT('Ctrl Pts',(-0.224105465849081,0.0121940707688781,
0.00941469086371163));
#44606=CARTESIAN_POINT('Ctrl Pts',(-0.224102886673673,0.0122483552961644,
0.00950296817005453));
#44607=CARTESIAN_POINT('Ctrl Pts',(-0.224204619171975,0.0122326177690983,
0.0095109744704432));
#44608=CARTESIAN_POINT('Ctrl Pts',(-0.224411006674875,0.0131602565471824,
0.00868824099025048));
#44609=CARTESIAN_POINT('Ctrl Pts',(-0.224408686153195,0.0132254016455477,
0.00876828599846793));
#44610=CARTESIAN_POINT('Ctrl Pts',(-0.224508634511665,0.013205870656239,
0.00878325506714548));
#44611=CARTESIAN_POINT('Ctrl Pts',(-0.224558309212759,0.0136746544994099,
0.0082011925670837));
#44612=CARTESIAN_POINT('Ctrl Pts',(-0.224556183524894,0.0137458268082903,
0.00827552216554079));
#44613=CARTESIAN_POINT('Ctrl Pts',(-0.224656964137442,0.0137301873698191,
0.00828947824167215));
#44614=CARTESIAN_POINT('Ctrl Pts',(-0.211142486563875,0.0080074480565038,
0.0103648761595404));
#44615=CARTESIAN_POINT('Ctrl Pts',(-0.211140614754186,0.00801345371234465,
0.0104703133205799));
#44616=CARTESIAN_POINT('Ctrl Pts',(-0.211035650930516,0.00802210230267836,
0.01046212346533));
#44617=CARTESIAN_POINT('Ctrl Pts',(-0.211050986105208,0.00698795766404281,
0.010420173009799));
#44618=CARTESIAN_POINT('Ctrl Pts',(-0.211049098556023,0.00698197862819438,
0.0105262957002229));
#44619=CARTESIAN_POINT('Ctrl Pts',(-0.210944362702546,0.00699359357385201,
0.0105192069513736));
#44620=CARTESIAN_POINT('Ctrl Pts',(-0.210843042872648,0.00493702977004334,
0.0101824991063636));
#44621=CARTESIAN_POINT('Ctrl Pts',(-0.2108412497187,0.00490752878610045,
0.0102859125807657));
#44622=CARTESIAN_POINT('Ctrl Pts',(-0.210735016148891,0.00490827075542475,
0.0102812729590393));
#44623=CARTESIAN_POINT('Ctrl Pts',(-0.211127743567256,0.0030792588706987,
0.00929899472494895));
#44624=CARTESIAN_POINT('Ctrl Pts',(-0.211126355522171,0.00302779946025978,
0.00939201828722784));
#44625=CARTESIAN_POINT('Ctrl Pts',(-0.211022153864861,0.00301706240296407,
0.00937797060777647));
#44626=CARTESIAN_POINT('Ctrl Pts',(-0.21126360341789,0.00224772336844146,
0.00871402935073148));
#44627=CARTESIAN_POINT('Ctrl Pts',(-0.211262455310447,0.00218683116784316,
0.00880031650240356));
#44628=CARTESIAN_POINT('Ctrl Pts',(-0.211157900322863,0.00218003268842091,
0.00878692414041944));
#44629=CARTESIAN_POINT('Ctrl Pts',(-0.21109423290342,0.00261222544444838,
0.00907399385816615));
#44630=CARTESIAN_POINT('Ctrl Pts',(-0.211095031960242,0.00261300460420345,
0.00907449760819488));
#44631=CARTESIAN_POINT('Ctrl Pts',(-0.211097157079409,0.00261503310819839,
0.00907577366587372));
#44632=CARTESIAN_POINT('Ctrl Pts',(-0.211099274163331,0.00261711947062296,
0.00907696675928809));
#44633=CARTESIAN_POINT('Ctrl Pts',(-0.211106432645342,0.00262449778379525,
0.00908107870213868));
#44634=CARTESIAN_POINT('Ctrl Pts',(-0.21111600284729,0.00263459647919183,
0.00908575699516419));
#44635=CARTESIAN_POINT('Ctrl Pts',(-0.211135588383209,0.00265827370691382,
0.00909042483809797));
#44636=CARTESIAN_POINT('Ctrl Pts',(-0.211144153168982,0.00266957861391556,
0.00909085164184115));
#44637=CARTESIAN_POINT('Ctrl Pts',(-0.211160507568082,0.00269370053702988,
0.00908736306728261));
#44638=CARTESIAN_POINT('Ctrl Pts',(-0.21116761520281,0.00270579305709638,
0.00908311389605883));
#44639=CARTESIAN_POINT('Ctrl Pts',(-0.211176248866459,0.00272362436611357,
0.00907263073110103));
#44640=CARTESIAN_POINT('Ctrl Pts',(-0.211178930690465,0.00273018991641854,
0.00906763592813339));
#44641=CARTESIAN_POINT('Ctrl Pts',(-0.211182404594494,0.00274156776870138,
0.00905631334382395));
#44642=CARTESIAN_POINT('Ctrl Pts',(-0.211183323601348,0.00274637390157652,
0.0090502845748891));
#44643=CARTESIAN_POINT('Ctrl Pts',(-0.211183450833508,0.00275046291514153,
0.0090436740602087));
#44644=CARTESIAN_POINT('Ctrl Pts',(-0.21109653717437,0.00749997694345283,
0.0103787828226083));
#44645=CARTESIAN_POINT('Ctrl Pts',(-0.211096377051465,0.0074999768281518,
0.0103852568676532));
#44646=CARTESIAN_POINT('Ctrl Pts',(-0.211095585865638,0.00749997659773733,
0.0103916996961516));
#44647=CARTESIAN_POINT('Ctrl Pts',(-0.211092658094877,0.00749997587113233,
0.0104048162942189));
#44648=CARTESIAN_POINT('Ctrl Pts',(-0.211090433159657,0.00749997535858776,
0.0104114340036142));
#44649=CARTESIAN_POINT('Ctrl Pts',(-0.211082179478388,0.00749997349822519,
0.0104294826171081));
#44650=CARTESIAN_POINT('Ctrl Pts',(-0.211074603814682,0.00749997184524541,
0.0104400500418335));
#44651=CARTESIAN_POINT('Ctrl Pts',(-0.211055860329739,0.00749996745397796,
0.0104577422926592));
#44652=CARTESIAN_POINT('Ctrl Pts',(-0.211044865979588,0.0074999649596482,
0.010464700090393));
#44653=CARTESIAN_POINT('Ctrl Pts',(-0.211020921400677,0.00749995680559278,
0.0104740606920776));
#44654=CARTESIAN_POINT('Ctrl Pts',(-0.211009742857274,0.00749997562380762,
0.0104758098878422));
#44655=CARTESIAN_POINT('Ctrl Pts',(-0.210998444007994,0.00749991418408376,
0.010476303815204));
#44656=CARTESIAN_POINT('Ctrl Pts',(-0.210996046515157,0.00749996002718701,
0.0104763293718199));
#44657=CARTESIAN_POINT('Ctrl Pts',(-0.210993907311933,0.00749995962611463,
0.0104762811460141));
#44658=CARTESIAN_POINT('Ctrl Pts',(-0.211264233927682,0.0127511389206587,
0.00871469219517674));
#44659=CARTESIAN_POINT('Ctrl Pts',(-0.211263339626816,0.0128119565920338,
0.00880095561734849));
#44660=CARTESIAN_POINT('Ctrl Pts',(-0.211158825258817,0.0128189223440845,
0.00878785171549552));
#44661=CARTESIAN_POINT('Ctrl Pts',(-0.211128617377145,0.0119162340263877,
0.00930117032032682));
#44662=CARTESIAN_POINT('Ctrl Pts',(-0.211127481783243,0.0119675771074036,
0.00939418426185652));
#44663=CARTESIAN_POINT('Ctrl Pts',(-0.211023317817383,0.0119783876644333,
0.00938046409104126));
#44664=CARTESIAN_POINT('Ctrl Pts',(-0.210843657835916,0.0100628466537089,
0.0101822731973737));
#44665=CARTESIAN_POINT('Ctrl Pts',(-0.210842123435839,0.0100923256739967,
0.0102856191594558));
#44666=CARTESIAN_POINT('Ctrl Pts',(-0.210735935133894,0.0100919118355424,
0.0102812355219947));
#44667=CARTESIAN_POINT('Ctrl Pts',(-0.211051061885002,0.00800517834552088,
0.0104208257432116));
#44668=CARTESIAN_POINT('Ctrl Pts',(-0.211049429352862,0.00801110099720398,
0.0105268952080997));
#44669=CARTESIAN_POINT('Ctrl Pts',(-0.21094474436933,0.00799938724367094,
0.010520142978524));
#44670=CARTESIAN_POINT('Ctrl Pts',(-0.21114359232468,0.00698385841965477,
0.0103640872892378));
#44671=CARTESIAN_POINT('Ctrl Pts',(-0.211141976460829,0.00697777627165395,
0.0104694570977041));
#44672=CARTESIAN_POINT('Ctrl Pts',(-0.211037057567724,0.00696911234332138,
0.0104615765116688));
#44673=CARTESIAN_POINT('Ctrl Pts',(-0.211184221002222,0.0122473944266094,
0.00904500436478942));
#44674=CARTESIAN_POINT('Ctrl Pts',(-0.211184098199553,0.0122513346632141,
0.00905137936580629));
#44675=CARTESIAN_POINT('Ctrl Pts',(-0.211183238943289,0.0122559428744482,
0.00905721691973273));
#44676=CARTESIAN_POINT('Ctrl Pts',(-0.211179996364333,0.0122668101284925,
0.0090682227412344));
#44677=CARTESIAN_POINT('Ctrl Pts',(-0.211177497911413,0.0122730645346206,
0.00907312167743916));
#44678=CARTESIAN_POINT('Ctrl Pts',(-0.211169298567438,0.0122903498693054,
0.00908371038952613));
#44679=CARTESIAN_POINT('Ctrl Pts',(-0.211162424900141,0.0123022235298793,
0.0090881533960612));
#44680=CARTESIAN_POINT('Ctrl Pts',(-0.211146016988589,0.0123267344228518,
0.00909225293758861));
#44681=CARTESIAN_POINT('Ctrl Pts',(-0.211137049460936,0.0123386291345285,
0.00909194384282742));
#44682=CARTESIAN_POINT('Ctrl Pts',(-0.211114733857186,0.0123655993569228,
0.00908674967640739));
#44683=CARTESIAN_POINT('Ctrl Pts',(-0.211104000080846,0.0123765165947633,
0.00908073975421946));
#44684=CARTESIAN_POINT('Ctrl Pts',(-0.211098076742061,0.0123822937242966,
0.00907744499712002));
#44685=CARTESIAN_POINT('Ctrl Pts',(-0.211096579367605,0.0123839782188275,
0.00907641698839438));
#44686=CARTESIAN_POINT('Ctrl Pts',(-0.211094964997266,0.012385550393988,
0.00907540111084567));
#44687=CARTESIAN_POINT('Origin',(-0.21234691445843,0.00266705858836579,
0.00901527131884535));
#44688=CARTESIAN_POINT('Ctrl Pts',(-0.212183839051124,0.00275127645488708,
0.00906545020201979));
#44689=CARTESIAN_POINT('Ctrl Pts',(-0.212183806161036,0.00274710028676507,
0.00907203561543755));
#44690=CARTESIAN_POINT('Ctrl Pts',(-0.212184810900476,0.0027422375390462,
0.00907802538757539));
#44691=CARTESIAN_POINT('Ctrl Pts',(-0.212189027067766,0.00273042441974619,
0.00908970636821214));
#44692=CARTESIAN_POINT('Ctrl Pts',(-0.212192551418784,0.00272345730579584,
0.00909491757756041));
#44693=CARTESIAN_POINT('Ctrl Pts',(-0.212203716791087,0.00270508615455126,
0.00910561706884515));
#44694=CARTESIAN_POINT('Ctrl Pts',(-0.212212986854008,0.00269271750821749,
0.00910997223485915));
#44695=CARTESIAN_POINT('Ctrl Pts',(-0.212234368520539,0.00266825497643102,
0.00911363069173713));
#44696=CARTESIAN_POINT('Ctrl Pts',(-0.212245511720789,0.00265695351087488,
0.0091132640080577));
#44697=CARTESIAN_POINT('Ctrl Pts',(-0.212273582499721,0.00263101628233386,
0.00910841099827345));
#44698=CARTESIAN_POINT('Ctrl Pts',(-0.212287289141522,0.002620499708973,
0.00910266326508716));
#44699=CARTESIAN_POINT('Ctrl Pts',(-0.21229225893459,0.00261687235876597,
0.00910069349159562));
#44700=CARTESIAN_POINT('Ctrl Pts',(-0.212293365405452,0.00261594584361789,
0.00910016633472597));
#44701=CARTESIAN_POINT('Ctrl Pts',(-0.212294848987994,0.00261471070565374,
0.00909944936359943));
#44702=CARTESIAN_POINT('Ctrl Pts',(-0.212296006564873,0.00261384619513498,
0.00909892989563823));
#44703=CARTESIAN_POINT('Origin',(-0.21102377360653,0.0123325634480328,0.00898917035815447));
#44704=CARTESIAN_POINT('Ctrl Pts',(-0.212185024851611,0.0122473868968752,
0.00906629440501006));
#44705=CARTESIAN_POINT('Ctrl Pts',(-0.21218499368264,0.0122514417819006,
0.00907268872464956));
#44706=CARTESIAN_POINT('Ctrl Pts',(-0.212185940713764,0.0122561465343213,
0.00907852372725697));
#44707=CARTESIAN_POINT('Ctrl Pts',(-0.212189922634149,0.0122675536441838,
0.00908994240071966));
#44708=CARTESIAN_POINT('Ctrl Pts',(-0.212193252686342,0.012274274904222,
0.00909507756545489));
#44709=CARTESIAN_POINT('Ctrl Pts',(-0.212203944292361,0.0122922017002173,
0.00910582928455576));
#44710=CARTESIAN_POINT('Ctrl Pts',(-0.212212926014891,0.0123043686350945,
0.00911031870680742));
#44711=CARTESIAN_POINT('Ctrl Pts',(-0.212233698933047,0.0123284672250172,
0.00911434545853006));
#44712=CARTESIAN_POINT('Ctrl Pts',(-0.212244528204772,0.0123396058993226,
0.00911420588103199));
#44713=CARTESIAN_POINT('Ctrl Pts',(-0.212268288631956,0.0123619113149257,
0.00911055546564033));
#44714=CARTESIAN_POINT('Ctrl Pts',(-0.212280174342974,0.01237173556129,
0.00910673512663782));
#44715=CARTESIAN_POINT('Ctrl Pts',(-0.212290708620157,0.0123800530976797,
0.00910246249537526));
#44716=CARTESIAN_POINT('Ctrl Pts',(-0.212293399168351,0.0123820998196263,
0.00910138307795224));
#44717=CARTESIAN_POINT('Ctrl Pts',(-0.212296097533959,0.0123840891664848,
0.00910022666793963));
#44718=CARTESIAN_POINT('Ctrl Pts',(-0.212297179495208,0.0123848983299051,
0.00909974062817284));
#44719=CARTESIAN_POINT('Ctrl Pts',(-0.212223983669684,0.00249578230024466,
0.0089026290048257));
#44720=CARTESIAN_POINT('Ctrl Pts',(-0.212222315239459,0.00244051993255814,
0.00898671564148847));
#44721=CARTESIAN_POINT('Ctrl Pts',(-0.212322077234447,0.00245097194074628,
0.00899481297505414));
#44722=CARTESIAN_POINT('Ctrl Pts',(-0.212102881444989,0.00325528982487909,
0.00940104945131877));
#44723=CARTESIAN_POINT('Ctrl Pts',(-0.212101008701363,0.00320837525514172,
0.00949063004707617));
#44724=CARTESIAN_POINT('Ctrl Pts',(-0.212200694817127,0.00322011434363844,
0.00949811209657471));
#44725=CARTESIAN_POINT('Ctrl Pts',(-0.211865003483227,0.00494001687375164,
0.0101751329037738));
#44726=CARTESIAN_POINT('Ctrl Pts',(-0.211862844425244,0.00491188107110286,
0.0102732804691239));
#44727=CARTESIAN_POINT('Ctrl Pts',(-0.21196410551886,0.00491301061554956,
0.0102728695412691));
#44728=CARTESIAN_POINT('Ctrl Pts',(-0.212031241817383,0.00678912318233929,
0.0104179560391845));
#44729=CARTESIAN_POINT('Ctrl Pts',(-0.212028952115924,0.00678104752068375,
0.0105187548105473));
#44730=CARTESIAN_POINT('Ctrl Pts',(-0.212129112768025,0.00677136833426455,
0.0105196250578453));
#44731=CARTESIAN_POINT('Ctrl Pts',(-0.212114504545825,0.00770097981231512,
0.0103993205832573));
#44732=CARTESIAN_POINT('Ctrl Pts',(-0.212112222397844,0.00770313035708446,
0.0104999025723028));
#44733=CARTESIAN_POINT('Ctrl Pts',(-0.212212429687323,0.00769408823802094,
0.0105017420392689));
#44734=CARTESIAN_POINT('Ctrl Pts',(-0.212096206023604,0.00749993571117328,
0.0104011636214085));
#44735=CARTESIAN_POINT('Ctrl Pts',(-0.212096058107311,0.00749993554536779,
0.0104077087912101));
#44736=CARTESIAN_POINT('Ctrl Pts',(-0.212096555950432,0.00749993549141056,
0.0104142522424083));
#44737=CARTESIAN_POINT('Ctrl Pts',(-0.212098900330544,0.0074999356028455,
0.0104275568839437));
#44738=CARTESIAN_POINT('Ctrl Pts',(-0.212100823945479,0.00749993578221901,
0.0104342681194624));
#44739=CARTESIAN_POINT('Ctrl Pts',(-0.21210825374142,0.00749993661233937,
0.0104526711907501));
#44740=CARTESIAN_POINT('Ctrl Pts',(-0.212115344415089,0.00749993753547336,
0.0104635702349915));
#44741=CARTESIAN_POINT('Ctrl Pts',(-0.212133269910862,0.00749993983848996,
0.0104820915741914));
#44742=CARTESIAN_POINT('Ctrl Pts',(-0.212143939004055,0.00749994130999428,
0.0104895391360646));
#44743=CARTESIAN_POINT('Ctrl Pts',(-0.212165862168942,0.00749994301250812,
0.010499273169891));
#44744=CARTESIAN_POINT('Ctrl Pts',(-0.21217665941563,0.00749996174420459,
0.0105020595732478));
#44745=CARTESIAN_POINT('Ctrl Pts',(-0.212189860872875,0.00749992542283543,
0.0105032352134824));
#44746=CARTESIAN_POINT('Ctrl Pts',(-0.21219212844858,0.00749995163156639,
0.0105033615643368));
#44747=CARTESIAN_POINT('Ctrl Pts',(-0.212194330077505,0.0074999520583401,
0.0105034113689146));
#44748=CARTESIAN_POINT('Ctrl Pts',(-0.212122643014497,0.00721116078184923,
0.0103971097759903));
#44749=CARTESIAN_POINT('Ctrl Pts',(-0.212120363487194,0.00720802729624083,
0.010497586965253));
#44750=CARTESIAN_POINT('Ctrl Pts',(-0.212220493457096,0.00721701301401138,
0.0104996005393699));
#44751=CARTESIAN_POINT('Ctrl Pts',(-0.212036325010947,0.00815119828716712,
0.0104254852752672));
#44752=CARTESIAN_POINT('Ctrl Pts',(-0.212034033518481,0.00815861469739573,
0.0105262875146844));
#44753=CARTESIAN_POINT('Ctrl Pts',(-0.212134073861582,0.00816870458555384,
0.0105272711067881));
#44754=CARTESIAN_POINT('Ctrl Pts',(-0.211859115886666,0.0100584037447509,
0.0101853003279626));
#44755=CARTESIAN_POINT('Ctrl Pts',(-0.21185695613268,0.0100864888835407,
0.0102834827569533));
#44756=CARTESIAN_POINT('Ctrl Pts',(-0.211958176233036,0.0100851831560035,
0.0102830553358484));
#44757=CARTESIAN_POINT('Ctrl Pts',(-0.212112363322094,0.0117994791176497,
0.00937556698882922));
#44758=CARTESIAN_POINT('Ctrl Pts',(-0.21211050258229,0.0118469745004918,
0.00946479106560511));
#44759=CARTESIAN_POINT('Ctrl Pts',(-0.212210060685816,0.0118349787021983,
0.00947257912918343));
#44760=CARTESIAN_POINT('Ctrl Pts',(-0.212236638315871,0.0125752680371152,
0.00885550734677693));
#44761=CARTESIAN_POINT('Ctrl Pts',(-0.212234990566732,0.0126312664694345,
0.00893900834297023));
#44762=CARTESIAN_POINT('Ctrl Pts',(-0.212334686483614,0.0126210294980898,
0.00894719768338886));
#44763=CARTESIAN_POINT('Ctrl Pts',(-0.201155083193269,0.00216605663322667,
0.00858641232141098));
#44764=CARTESIAN_POINT('Ctrl Pts',(-0.20126096852948,0.00217232885330737,
0.00860101494802211));
#44765=CARTESIAN_POINT('Ctrl Pts',(-0.201261986180025,0.00223315111724539,
0.00851290633848732));
#44766=CARTESIAN_POINT('Ctrl Pts',(-0.201015029040136,0.00301234855195945,
0.00917044619233868));
#44767=CARTESIAN_POINT('Ctrl Pts',(-0.201120551074898,0.00302307644571231,
0.00918585713566367));
#44768=CARTESIAN_POINT('Ctrl Pts',(-0.201121818425293,0.00307436667035424,
0.00909110352796063));
#44769=CARTESIAN_POINT('Ctrl Pts',(-0.200741067091076,0.00490726025933776,
0.0100583553626889));
#44770=CARTESIAN_POINT('Ctrl Pts',(-0.200848644805918,0.00490457525049167,
0.0100640174517916));
#44771=CARTESIAN_POINT('Ctrl Pts',(-0.200850325606794,0.00493402244947655,
0.00995912466295495));
#44772=CARTESIAN_POINT('Ctrl Pts',(-0.200951724696489,0.00699776383342617,
0.0102933591526183));
#44773=CARTESIAN_POINT('Ctrl Pts',(-0.201057850521067,0.00698686745950293,
0.0103020115942979));
#44774=CARTESIAN_POINT('Ctrl Pts',(-0.201059631591013,0.00699277642326086,
0.0101944386176339));
#44775=CARTESIAN_POINT('Ctrl Pts',(-0.201035033694427,0.00803074714201528,
0.0102357737307844));
#44776=CARTESIAN_POINT('Ctrl Pts',(-0.201141386046049,0.00802257307788267,
0.0102453298409531));
#44777=CARTESIAN_POINT('Ctrl Pts',(-0.201143149297188,0.00801650549987341,
0.0101384442232337));
#44778=CARTESIAN_POINT('Ctrl Pts',(-0.201091335837404,0.0026023195479385,
0.00887000708307585));
#44779=CARTESIAN_POINT('Ctrl Pts',(-0.201092103354299,0.00260307247533696,
0.00887048379371787));
#44780=CARTESIAN_POINT('Ctrl Pts',(-0.201094259127555,0.00260513759398771,
0.00887175759780278));
#44781=CARTESIAN_POINT('Ctrl Pts',(-0.201096406464209,0.00260726257920991,
0.00887294403254245));
#44782=CARTESIAN_POINT('Ctrl Pts',(-0.201103264331842,0.00261437781908026,
0.0088768215853111));
#44783=CARTESIAN_POINT('Ctrl Pts',(-0.201112806708188,0.00262443779776055,
0.00888148334083447));
#44784=CARTESIAN_POINT('Ctrl Pts',(-0.20113267431363,0.00264850045287698,
0.00888598603513365));
#44785=CARTESIAN_POINT('Ctrl Pts',(-0.201141236183842,0.00265980541514074,
0.00888630262824218));
#44786=CARTESIAN_POINT('Ctrl Pts',(-0.201157583248774,0.00268388487459801,
0.0088825801587399));
#44787=CARTESIAN_POINT('Ctrl Pts',(-0.201164687512606,0.00269593311189708,
0.0088782145592798));
#44788=CARTESIAN_POINT('Ctrl Pts',(-0.201173315148115,0.00271365901443599,
0.00886756153217392));
#44789=CARTESIAN_POINT('Ctrl Pts',(-0.201175994276017,0.00272017405179653,
0.00886250578309987));
#44790=CARTESIAN_POINT('Ctrl Pts',(-0.201179464367247,0.00273144061067142,
0.00885107958730227));
#44791=CARTESIAN_POINT('Ctrl Pts',(-0.201180382062519,0.00273618870506716,
0.00884500762653599));
#44792=CARTESIAN_POINT('Ctrl Pts',(-0.201180508584589,0.00274021505325842,
0.00883836137431511));
#44793=CARTESIAN_POINT('Ctrl Pts',(-0.201099833981514,0.00749931673585989,
0.0101528932886838));
#44794=CARTESIAN_POINT('Ctrl Pts',(-0.201098485659853,0.00749931248699838,
0.0102056974765971));
#44795=CARTESIAN_POINT('Ctrl Pts',(-0.201049336965903,0.00749928794470734,
0.010251525133989));
#44796=CARTESIAN_POINT('Ctrl Pts',(-0.200997245792689,0.0074992653969341,
0.0102503478276375));
#44797=CARTESIAN_POINT('Ctrl Pts',(-0.201256650812755,0.0127742337711833,
0.00853880624905052));
#44798=CARTESIAN_POINT('Ctrl Pts',(-0.201250184418728,0.0127904275512369,
0.00856079060756085));
#44799=CARTESIAN_POINT('Ctrl Pts',(-0.201237195582423,0.0128229554728312,
0.00860494987658638));
#44800=CARTESIAN_POINT('Ctrl Pts',(-0.201182619048712,0.0128358773798212,
0.00861051744946986));
#44801=CARTESIAN_POINT('Ctrl Pts',(-0.201155303926009,0.0128424090648251,
0.00861339759601743));
#44802=CARTESIAN_POINT('Ctrl Pts',(-0.201208595417358,0.0124465598212127,
0.00871977498087392));
#44803=CARTESIAN_POINT('Ctrl Pts',(-0.201202102965136,0.0124617746892246,
0.00874233334840889));
#44804=CARTESIAN_POINT('Ctrl Pts',(-0.201189061786604,0.0124923363019008,
0.00878764561077419));
#44805=CARTESIAN_POINT('Ctrl Pts',(-0.201134434005491,0.0125046664137396,
0.00879380973072894));
#44806=CARTESIAN_POINT('Ctrl Pts',(-0.201107093146125,0.0125108979201374,
0.00879699065408895));
#44807=CARTESIAN_POINT('Ctrl Pts',(-0.201127094918058,0.0119476316067464,
0.00903388131834477));
#44808=CARTESIAN_POINT('Ctrl Pts',(-0.201120570437375,0.0119614484304572,
0.00905738721554734));
#44809=CARTESIAN_POINT('Ctrl Pts',(-0.201107464924307,0.0119892018368183,
0.00910460275007228));
#44810=CARTESIAN_POINT('Ctrl Pts',(-0.201052858340458,0.012001410986791,
0.00911138733244231));
#44811=CARTESIAN_POINT('Ctrl Pts',(-0.201025527938516,0.0120075758779105,
0.00911488262945839));
#44812=CARTESIAN_POINT('Ctrl Pts',(-0.201008085070164,0.0110295302488516,
0.00946855886042181));
#44813=CARTESIAN_POINT('Ctrl Pts',(-0.201001473220532,0.0110404306864664,
0.0094935350509485));
#44814=CARTESIAN_POINT('Ctrl Pts',(-0.200988192212286,0.0110623260425169,
0.00954370391606149));
#44815=CARTESIAN_POINT('Ctrl Pts',(-0.200933255780015,0.0110714126965106,
0.00955270028796668));
#44816=CARTESIAN_POINT('Ctrl Pts',(-0.200905760079558,0.0110760036237351,
0.00955730787255131));
#44817=CARTESIAN_POINT('Ctrl Pts',(-0.2009503980621,0.0100226663357829,
0.00982992257831994));
#44818=CARTESIAN_POINT('Ctrl Pts',(-0.200943711780911,0.010030070211669,
0.00985618971045741));
#44819=CARTESIAN_POINT('Ctrl Pts',(-0.200930281264408,0.0100449421374034,
0.00990895164817973));
#44820=CARTESIAN_POINT('Ctrl Pts',(-0.200875054282338,0.0100483822204513,
0.00992028137773493));
#44821=CARTESIAN_POINT('Ctrl Pts',(-0.200847412988371,0.0100501346700953,
0.00992606124313427));
#44822=CARTESIAN_POINT('Ctrl Pts',(-0.200985752557974,0.00896573313553926,
0.010048170465822));
#44823=CARTESIAN_POINT('Ctrl Pts',(-0.200979059787987,0.00896968565447399,
0.0100751056398674));
#44824=CARTESIAN_POINT('Ctrl Pts',(-0.200965616237646,0.00897762495126472,
0.0101292094517371));
#44825=CARTESIAN_POINT('Ctrl Pts',(-0.200910533124437,0.00897646676150334,
0.010141131282486));
#44826=CARTESIAN_POINT('Ctrl Pts',(-0.20088296373237,0.00897590505164646,
0.0101472101147103));
#44827=CARTESIAN_POINT('Ctrl Pts',(-0.20105982521262,0.00795581183071892,
0.0101560920619458));
#44828=CARTESIAN_POINT('Ctrl Pts',(-0.201053134234794,0.0079566211870063,
0.0101833039398003));
#44829=CARTESIAN_POINT('Ctrl Pts',(-0.201039694284309,0.00795824691477156,
0.0102379635576509));
#44830=CARTESIAN_POINT('Ctrl Pts',(-0.200984724529276,0.00795415818384021,
0.0102497134489866));
#44831=CARTESIAN_POINT('Ctrl Pts',(-0.200957211820981,0.00795211748649824,
0.0102557075311292));
#44832=CARTESIAN_POINT('Ctrl Pts',(-0.201111796847579,0.00736530035222225,
0.0101482803792522));
#44833=CARTESIAN_POINT('Ctrl Pts',(-0.201105107498193,0.00736435844767988,
0.0101754262075262));
#44834=CARTESIAN_POINT('Ctrl Pts',(-0.2010916708187,0.00736246647452709,
0.0102299531537233));
#44835=CARTESIAN_POINT('Ctrl Pts',(-0.201036707330346,0.00735763278097222,
0.0102413477195797));
#44836=CARTESIAN_POINT('Ctrl Pts',(-0.201009197762365,0.00735521193479846,
0.0102471638589911));
#44837=CARTESIAN_POINT('Ctrl Pts',(-0.201142066721907,0.00699237110554977,
0.0101642439779473));
#44838=CARTESIAN_POINT('Ctrl Pts',(-0.201135378229863,0.00699029770385,
0.0101914152333036));
#44839=CARTESIAN_POINT('Ctrl Pts',(-0.201121943272494,0.00698613292899819,
0.0102459932540579));
#44840=CARTESIAN_POINT('Ctrl Pts',(-0.20106700142688,0.00698054335286895,
0.0102572385002951));
#44841=CARTESIAN_POINT('Ctrl Pts',(-0.201039502683419,0.00697773961910315,
0.0102629800957228));
#44842=CARTESIAN_POINT('Ctrl Pts',(-0.201177053601335,0.0122550060276839,
0.00884070721774072));
#44843=CARTESIAN_POINT('Ctrl Pts',(-0.20117084753263,0.0122690513730654,
0.0088625295460327));
#44844=CARTESIAN_POINT('Ctrl Pts',(-0.201164660143918,0.0122901709254442,
0.00888140040275825));
#44845=CARTESIAN_POINT('Ctrl Pts',(-0.201150491997757,0.012310871344524,
0.00888736415769192));
#44846=CARTESIAN_POINT('Ctrl Pts',(-0.201132286732426,0.0123374702105669,
0.00889502724499377));
#44847=CARTESIAN_POINT('Ctrl Pts',(-0.201103744801886,0.0123645072421567,
0.00888409859256188));
#44848=CARTESIAN_POINT('Ctrl Pts',(-0.20108848344321,0.0123927133101065,
0.00887232988670267));
#44849=CARTESIAN_POINT('Origin',(-0.202343907248651,0.0026559890716155,
0.00881026065166738));
#44850=CARTESIAN_POINT('Ctrl Pts',(-0.202180796597781,0.00274072101466718,
0.00885976287803625));
#44851=CARTESIAN_POINT('Ctrl Pts',(-0.20218076839761,0.00273661010376764,
0.0088663730597778));
#44852=CARTESIAN_POINT('Ctrl Pts',(-0.202181774626836,0.00273180944123569,
0.00887239520899083));
#44853=CARTESIAN_POINT('Ctrl Pts',(-0.202185992690961,0.00272010970759771,
0.00888417484072343));
#44854=CARTESIAN_POINT('Ctrl Pts',(-0.202189521425533,0.00271318748468188,
0.00888944907905161));
#44855=CARTESIAN_POINT('Ctrl Pts',(-0.202200697689997,0.0026949096883953,
0.00890031160453069));
#44856=CARTESIAN_POINT('Ctrl Pts',(-0.202209975776181,0.00268257757595377,
0.00890477601358085));
#44857=CARTESIAN_POINT('Ctrl Pts',(-0.202231502282787,0.00265799781199361,
0.00890867262799436));
#44858=CARTESIAN_POINT('Ctrl Pts',(-0.202242804632951,0.00264655434339955,
0.00890837604318305));
#44859=CARTESIAN_POINT('Ctrl Pts',(-0.202271224259584,0.00262032723305801,
0.00890360222775761));
#44860=CARTESIAN_POINT('Ctrl Pts',(-0.202285063897618,0.00260966649176247,
0.00889780688643869));
#44861=CARTESIAN_POINT('Ctrl Pts',(-0.202290010562206,0.00260614356034156,
0.00889590681455424));
#44862=CARTESIAN_POINT('Ctrl Pts',(-0.202290907367527,0.00260535459335703,
0.00889546010904801));
#44863=CARTESIAN_POINT('Ctrl Pts',(-0.202292110547019,0.00260430091210787,
0.00889485527913338));
#44864=CARTESIAN_POINT('Ctrl Pts',(-0.202293070892211,0.00260358016718893,
0.00889443116859542));
#44865=CARTESIAN_POINT('Origin',(-0.201017179898206,0.0123408640444401,
0.0087860767507338));
#44866=CARTESIAN_POINT('Ctrl Pts',(-0.202178488577975,0.0122548116993251,
0.00886238997990231));
#44867=CARTESIAN_POINT('Ctrl Pts',(-0.202178460670578,0.0122588178162135,
0.00886883835749566));
#44868=CARTESIAN_POINT('Ctrl Pts',(-0.202179416149129,0.0122634820086249,
0.00887473017188245));
#44869=CARTESIAN_POINT('Ctrl Pts',(-0.202183428804187,0.0122748259653014,
0.00888628518227572));
#44870=CARTESIAN_POINT('Ctrl Pts',(-0.202186785687581,0.0122815298877756,
0.00889149430525874));
#44871=CARTESIAN_POINT('Ctrl Pts',(-0.202197543161461,0.0122994101048659,
0.00890240889430388));
#44872=CARTESIAN_POINT('Ctrl Pts',(-0.202206565485128,0.0123115589479267,
0.0089069960771264));
#44873=CARTESIAN_POINT('Ctrl Pts',(-0.202227367447855,0.0123355961269311,
0.00891119198501783));
#44874=CARTESIAN_POINT('Ctrl Pts',(-0.202238171446361,0.0123466906680839,
0.00891114135503747));
#44875=CARTESIAN_POINT('Ctrl Pts',(-0.202262860105077,0.0123698697743196,
0.00890754832784731));
#44876=CARTESIAN_POINT('Ctrl Pts',(-0.202275059499577,0.0123798177466737,
0.00890344762387098));
#44877=CARTESIAN_POINT('Ctrl Pts',(-0.20228416687705,0.012387051170581,
0.00889981733451039));
#44878=CARTESIAN_POINT('Ctrl Pts',(-0.202286920089651,0.0123891504139199,
0.0088987392573964));
#44879=CARTESIAN_POINT('Ctrl Pts',(-0.202289679251312,0.01239118638763,
0.00889757906871427));
#44880=CARTESIAN_POINT('Ctrl Pts',(-0.202290700091811,0.0123919533806702,
0.00889712834741086));
#44881=CARTESIAN_POINT('Ctrl Pts',(-0.202265283386786,0.00221674355360878,
0.0085200608006989));
#44882=CARTESIAN_POINT('Ctrl Pts',(-0.202262903766929,0.00215815693190638,
0.00860438499719491));
#44883=CARTESIAN_POINT('Ctrl Pts',(-0.202364785162833,0.00216892793183714,
0.00861155864805056));
#44884=CARTESIAN_POINT('Ctrl Pts',(-0.202126393174205,0.00304878504751519,
0.0090976895221217));
#44885=CARTESIAN_POINT('Ctrl Pts',(-0.202123767066444,0.00299929247320867,
0.00918838770691312));
#44886=CARTESIAN_POINT('Ctrl Pts',(-0.202225299563324,0.00301370238024901,
0.00919586042731392));
#44887=CARTESIAN_POINT('Ctrl Pts',(-0.201846780434746,0.00493160127209062,
0.00998542514888836));
#44888=CARTESIAN_POINT('Ctrl Pts',(-0.20184379305394,0.00490326887046296,
0.0100860430326691));
#44889=CARTESIAN_POINT('Ctrl Pts',(-0.20194732115168,0.00490316112478149,
0.0100833805366352));
#44890=CARTESIAN_POINT('Ctrl Pts',(-0.202060558052025,0.00700518294088309,
0.0102172780069111));
#44891=CARTESIAN_POINT('Ctrl Pts',(-0.202057443704119,0.00699955579133595,
0.0103204291575386));
#44892=CARTESIAN_POINT('Ctrl Pts',(-0.202159605819829,0.00698941479977137,
0.0103203063255642));
#44893=CARTESIAN_POINT('Ctrl Pts',(-0.202143361846868,0.00802345793181346,
0.0101604293836056));
#44894=CARTESIAN_POINT('Ctrl Pts',(-0.202140271632653,0.00802931137431162,
0.0102629275659062));
#44895=CARTESIAN_POINT('Ctrl Pts',(-0.202242659763401,0.00802100637154811,
0.0102637647012907));
#44896=CARTESIAN_POINT('Ctrl Pts',(-0.202099463949638,0.00749950457486307,
0.0101752294684686));
#44897=CARTESIAN_POINT('Ctrl Pts',(-0.20209931606238,0.00749950424735862,
0.0101817730524425));
#44898=CARTESIAN_POINT('Ctrl Pts',(-0.202099813307759,0.0074995041438527,
0.010188314976911));
#44899=CARTESIAN_POINT('Ctrl Pts',(-0.202102155212527,0.00749950439525637,
0.0102016163950763));
#44900=CARTESIAN_POINT('Ctrl Pts',(-0.202104076840267,0.00749950477897649,
0.0102083261168978));
#44901=CARTESIAN_POINT('Ctrl Pts',(-0.202111500004307,0.00749950657857423,
0.0102267270920281));
#44902=CARTESIAN_POINT('Ctrl Pts',(-0.202118585533017,0.00749950857758533,
0.0102376266605826));
#44903=CARTESIAN_POINT('Ctrl Pts',(-0.202136499996345,0.00749951401374605,
0.0102561492958782));
#44904=CARTESIAN_POINT('Ctrl Pts',(-0.202147162872982,0.00749951740124023,
0.0102635981106341));
#44905=CARTESIAN_POINT('Ctrl Pts',(-0.202175158064661,0.0074995265905247,
0.0102760372628172));
#44906=CARTESIAN_POINT('Ctrl Pts',(-0.202189268457591,0.00749954163844324,
0.0102772369414757));
#44907=CARTESIAN_POINT('Ctrl Pts',(-0.202197037592779,0.00749953297569803,
0.0102774630649767));
#44908=CARTESIAN_POINT('Ctrl Pts',(-0.202197541742858,0.00749953433505264,
0.0102774756030113));
#44909=CARTESIAN_POINT('Ctrl Pts',(-0.202361880888437,0.0128264515031921,
0.0086147092298632));
#44910=CARTESIAN_POINT('Ctrl Pts',(-0.202260113951347,0.0128370847197872,
0.0086074593432484));
#44911=CARTESIAN_POINT('Ctrl Pts',(-0.202262517511821,0.0127786173864275,
0.00852320316472772));
#44912=CARTESIAN_POINT('Ctrl Pts',(-0.202223258922033,0.0119819745234462,
0.00919807175636186));
#44913=CARTESIAN_POINT('Ctrl Pts',(-0.20212183907179,0.0119962328416967,
0.00919051456852261));
#44914=CARTESIAN_POINT('Ctrl Pts',(-0.202124488350021,0.0119468443820253,
0.00909990279227285));
#44915=CARTESIAN_POINT('Ctrl Pts',(-0.201945876329119,0.0100935785167927,
0.010083967214963));
#44916=CARTESIAN_POINT('Ctrl Pts',(-0.201842473337064,0.0100934554540095,
0.0100864724546506));
#44917=CARTESIAN_POINT('Ctrl Pts',(-0.201845483364813,0.0100651943495382,
0.00998596792976334));
#44918=CARTESIAN_POINT('Ctrl Pts',(-0.202159081801773,0.00800919428865958,
0.0103202693714982));
#44919=CARTESIAN_POINT('Ctrl Pts',(-0.202057049752887,0.0079989680904996,
0.0103202497035326));
#44920=CARTESIAN_POINT('Ctrl Pts',(-0.202060185966541,0.00799336645668808,
0.0102172231029901));
#44921=CARTESIAN_POINT('Ctrl Pts',(-0.202242858976565,0.00697850976193525,
0.0102637454365422));
#44922=CARTESIAN_POINT('Ctrl Pts',(-0.202140599979829,0.0069701564498707,
0.0102627551815556));
#44923=CARTESIAN_POINT('Ctrl Pts',(-0.20214371220484,0.0069760105515131,
0.0101603809964741));
#44924=CARTESIAN_POINT('Ctrl Pts',(-0.199153917445656,0.00216330382806559,
0.0085466816420894));
#44925=CARTESIAN_POINT('Ctrl Pts',(-0.199259854338567,0.00216954278467004,
0.00856124395669496));
#44926=CARTESIAN_POINT('Ctrl Pts',(-0.199260840617245,0.00223019704828265,
0.00847296600068187));
#44927=CARTESIAN_POINT('Ctrl Pts',(-0.199014559592398,0.00301082025703676,
0.00912885805490715));
#44928=CARTESIAN_POINT('Ctrl Pts',(-0.199120135788544,0.0030215055052538,
0.0091442300040962));
#44929=CARTESIAN_POINT('Ctrl Pts',(-0.19912137309385,0.00307263960711639,
0.00904934758541328));
#44930=CARTESIAN_POINT('Ctrl Pts',(-0.198742264019069,0.00490687946315208,
0.0100137040478795));
#44931=CARTESIAN_POINT('Ctrl Pts',(-0.198849878408609,0.0049041364027777,
0.0100193895857334));
#44932=CARTESIAN_POINT('Ctrl Pts',(-0.19885152983239,0.00493349699554989,
0.00991444126272149));
#44933=CARTESIAN_POINT('Ctrl Pts',(-0.198952774929459,0.00699674633684083,
0.0102479409536527));
#44934=CARTESIAN_POINT('Ctrl Pts',(-0.199058944563945,0.0069858644231249,
0.0102566134579587));
#44935=CARTESIAN_POINT('Ctrl Pts',(-0.199060696986617,0.00699176666959928,
0.0101490006187123));
#44936=CARTESIAN_POINT('Ctrl Pts',(-0.199035988933059,0.00802971819184572,
0.0101907130089996));
#44937=CARTESIAN_POINT('Ctrl Pts',(-0.199142384098032,0.00802154341492879,
0.0102002834057196));
#44938=CARTESIAN_POINT('Ctrl Pts',(-0.19914411851978,0.00801551120631029,
0.0100933513992024));
#44939=CARTESIAN_POINT('Ctrl Pts',(-0.199090544161673,0.00260012940780254,
0.0088293656616242));
#44940=CARTESIAN_POINT('Ctrl Pts',(-0.19909130728753,0.00260087836723755,
0.00882983779134686));
#44941=CARTESIAN_POINT('Ctrl Pts',(-0.199093469606293,0.00260294996891118,
0.00883111025990233));
#44942=CARTESIAN_POINT('Ctrl Pts',(-0.199095623457249,0.00260508172848499,
0.00883229463920616));
#44943=CARTESIAN_POINT('Ctrl Pts',(-0.199102455445532,0.00261217358753728,
0.00883614138729688));
#44944=CARTESIAN_POINT('Ctrl Pts',(-0.199112010710586,0.00262224476993763,
0.00884079237775844));
#44945=CARTESIAN_POINT('Ctrl Pts',(-0.199131908567056,0.00264633414288908,
0.0088452514389217));
#44946=CARTESIAN_POINT('Ctrl Pts',(-0.199140475861325,0.00265763798807928,
0.0088455461646959));
#44947=CARTESIAN_POINT('Ctrl Pts',(-0.199156834842009,0.00268170883000255,
0.00884177770164222));
#44948=CARTESIAN_POINT('Ctrl Pts',(-0.199163944618197,0.00269374857837251,
0.00883738897005369));
#44949=CARTESIAN_POINT('Ctrl Pts',(-0.199172579209817,0.00271145441669992,
0.0088267017145877));
#44950=CARTESIAN_POINT('Ctrl Pts',(-0.19917526070757,0.002717960405818,
0.00882163297988479));
#44951=CARTESIAN_POINT('Ctrl Pts',(-0.199178733682342,0.00272920614009963,
0.00881018371261812));
#44952=CARTESIAN_POINT('Ctrl Pts',(-0.19917965205846,0.00273394296772727,
0.00880410193455148));
#44953=CARTESIAN_POINT('Ctrl Pts',(-0.19917977849694,0.0027379568580951,
0.00879744706911775));
#44954=CARTESIAN_POINT('Ctrl Pts',(-0.199100846801734,0.00749833347458839,
0.0101077255427978));
#44955=CARTESIAN_POINT('Ctrl Pts',(-0.19909949185117,0.00749832362100577,
0.0101605248182571));
#44956=CARTESIAN_POINT('Ctrl Pts',(-0.199050347020319,0.00749829538362156,
0.0102063461419179));
#44957=CARTESIAN_POINT('Ctrl Pts',(-0.198998259704992,0.00749827421839395,
0.0102051689206332));
#44958=CARTESIAN_POINT('Ctrl Pts',(-0.199252995072792,0.0127774882842919,
0.00849852558719801));
#44959=CARTESIAN_POINT('Ctrl Pts',(-0.199246529899215,0.0127936285615535,
0.00852055158884003));
#44960=CARTESIAN_POINT('Ctrl Pts',(-0.199233543673028,0.0128260486178342,
0.00856479396468572));
#44961=CARTESIAN_POINT('Ctrl Pts',(-0.199178953436479,0.0128388912776996,
0.00857043901569242));
#44962=CARTESIAN_POINT('Ctrl Pts',(-0.199151631540807,0.0128453829053665,
0.00857335780561756));
#44963=CARTESIAN_POINT('Ctrl Pts',(-0.199205485012669,0.0124493328032341,
0.00867900065461348));
#44964=CARTESIAN_POINT('Ctrl Pts',(-0.199198993780824,0.0124644960051388,
0.00870159673323534));
#44965=CARTESIAN_POINT('Ctrl Pts',(-0.199185955212879,0.0124949534657617,
0.00874698419026339));
#44966=CARTESIAN_POINT('Ctrl Pts',(-0.199131314364772,0.0125072036339993,
0.0087532195982415));
#44967=CARTESIAN_POINT('Ctrl Pts',(-0.19910396705067,0.0125133947551101,
0.00875643604575879));
#44968=CARTESIAN_POINT('Ctrl Pts',(-0.199124866985969,0.0119495412903626,
0.00899228522622666));
#44969=CARTESIAN_POINT('Ctrl Pts',(-0.199118343519783,0.0119633083281558,
0.00901582261420499));
#44970=CARTESIAN_POINT('Ctrl Pts',(-0.199105240204551,0.0119909613933932,
0.00906310082576092));
#44971=CARTESIAN_POINT('Ctrl Pts',(-0.199050620029599,0.0120030870736398,
0.00906994918457371));
#44972=CARTESIAN_POINT('Ctrl Pts',(-0.199023282910386,0.0120092098423158,
0.00907347621110877));
#44973=CARTESIAN_POINT('Ctrl Pts',(-0.199007287267715,0.0110303351348565,
0.00942571112218718));
#44974=CARTESIAN_POINT('Ctrl Pts',(-0.199000676818597,0.0110411926535879,
0.00945070822400934));
#44975=CARTESIAN_POINT('Ctrl Pts',(-0.198987398785699,0.0110630015334869,
0.00950091847968093));
#44976=CARTESIAN_POINT('Ctrl Pts',(-0.198932453345222,0.0110720073961954,
0.00950995769117948));
#44977=CARTESIAN_POINT('Ctrl Pts',(-0.198904953221552,0.0110765576063949,
0.00951458647297514));
#44978=CARTESIAN_POINT('Ctrl Pts',(-0.198950876441888,0.0100226308845471,
0.00978597479287774));
#44979=CARTESIAN_POINT('Ctrl Pts',(-0.198944192313863,0.0100300028344982,
0.00981225272852039));
#44980=CARTESIAN_POINT('Ctrl Pts',(-0.198930766286339,0.0100448104507761,
0.00986503572218605));
#44981=CARTESIAN_POINT('Ctrl Pts',(-0.198875537616916,0.0100481896171548,
0.0098763822509411));
#44982=CARTESIAN_POINT('Ctrl Pts',(-0.198847895564142,0.0100499113777636,
0.00988217023395557));
#44983=CARTESIAN_POINT('Ctrl Pts',(-0.198986795866928,0.00896522208316481,
0.0100034584399927));
#44984=CARTESIAN_POINT('Ctrl Pts',(-0.198980105148717,0.0089691562897449,
0.0100303985815119));
#44985=CARTESIAN_POINT('Ctrl Pts',(-0.198966665883862,0.00897705870657931,
0.0100845117104313));
#44986=CARTESIAN_POINT('Ctrl Pts',(-0.198911580935987,0.00897588131856843,
0.0100964358107904));
#44987=CARTESIAN_POINT('Ctrl Pts',(-0.198884010711124,0.00897530988002672,
0.0101025154623784));
#44988=CARTESIAN_POINT('Ctrl Pts',(-0.199060893012184,0.00795492981715577,
0.0101109376831195));
#44989=CARTESIAN_POINT('Ctrl Pts',(-0.19905420386632,0.00795573250050825,
0.0101381519892747));
#44990=CARTESIAN_POINT('Ctrl Pts',(-0.199040767759749,0.00795734480487209,
0.0101928158170936));
#44991=CARTESIAN_POINT('Ctrl Pts',(-0.198985794732566,0.00795325937128545,
0.0102045659851305));
#44992=CARTESIAN_POINT('Ctrl Pts',(-0.198958280471805,0.00795122028247677,
0.0102105598756125));
#44993=CARTESIAN_POINT('Ctrl Pts',(-0.199112792949338,0.00736427983216101,
0.0101030859175174));
#44994=CARTESIAN_POINT('Ctrl Pts',(-0.199106105446657,0.00736333742444203,
0.0101302344227966));
#44995=CARTESIAN_POINT('Ctrl Pts',(-0.199092672640656,0.00736144446369592,
0.0101847660801409));
#44996=CARTESIAN_POINT('Ctrl Pts',(-0.199037705857924,0.00735661611559613,
0.0101961630417089));
#44997=CARTESIAN_POINT('Ctrl Pts',(-0.199010194726408,0.00735419795088647,
0.0102019800507694));
#44998=CARTESIAN_POINT('Ctrl Pts',(-0.199143042960716,0.00699123828422424,
0.0101189604526251));
#44999=CARTESIAN_POINT('Ctrl Pts',(-0.199136356282475,0.0069891684572404,
0.0101461340332429));
#45000=CARTESIAN_POINT('Ctrl Pts',(-0.199122925132461,0.00698501091358601,
0.0102007160579938));
#45001=CARTESIAN_POINT('Ctrl Pts',(-0.199067979737894,0.00697943123747824,
0.0102119640717528));
#45002=CARTESIAN_POINT('Ctrl Pts',(-0.199040479303471,0.00697663249430555,
0.0102177067208405));
#45003=CARTESIAN_POINT('Ctrl Pts',(-0.199174846040548,0.0122573379664025,
0.00879984889793131));
#45004=CARTESIAN_POINT('Ctrl Pts',(-0.199174163106151,0.0122823816012495,
0.00884168590479541));
#45005=CARTESIAN_POINT('Ctrl Pts',(-0.199137777220614,0.0123252893097993,
0.00885359374849819));
#45006=CARTESIAN_POINT('Ctrl Pts',(-0.19910812755215,0.0123635456293657,
0.00884505562956225));
#45007=CARTESIAN_POINT('Ctrl Pts',(-0.199099738487824,0.0123743698558192,
0.00884263985789638));
#45008=CARTESIAN_POINT('Ctrl Pts',(-0.199091892717798,0.0123851046964944,
0.00883840677396556));
#45009=CARTESIAN_POINT('Ctrl Pts',(-0.19908556181331,0.0123952967315942,
0.00883206936057618));
#45010=CARTESIAN_POINT('Origin',(-0.20034316899928,0.00265361948026404,
0.00876944888039472));
#45011=CARTESIAN_POINT('Ctrl Pts',(-0.200180138467595,0.00273845005850156,
0.00881880524816497));
#45012=CARTESIAN_POINT('Ctrl Pts',(-0.200180111069365,0.0027343534632471,
0.0088254195296896));
#45013=CARTESIAN_POINT('Ctrl Pts',(-0.20018111626804,0.00272956660640373,
0.00883144775892295));
#45014=CARTESIAN_POINT('Ctrl Pts',(-0.200185329611713,0.00271789323850519,
0.00884324632224045));
#45015=CARTESIAN_POINT('Ctrl Pts',(-0.200188854916373,0.00271098217482735,
0.00884853338008211));
#45016=CARTESIAN_POINT('Ctrl Pts',(-0.200200021494589,0.00269272660018771,
0.00885943065655154));
#45017=CARTESIAN_POINT('Ctrl Pts',(-0.200209291703764,0.00268040388413873,
0.00886391870869385));
#45018=CARTESIAN_POINT('Ctrl Pts',(-0.200230849539644,0.00265577661479843,
0.00886787204504395));
#45019=CARTESIAN_POINT('Ctrl Pts',(-0.200242201866841,0.00264427919255049,
0.00886758640057448));
#45020=CARTESIAN_POINT('Ctrl Pts',(-0.200270784471942,0.00261789598308321,
0.00886279510022952));
#45021=CARTESIAN_POINT('Ctrl Pts',(-0.20028469313402,0.00260716979711846,
0.00885693527935284));
#45022=CARTESIAN_POINT('Ctrl Pts',(-0.200289538153472,0.00260376631764392,
0.00885509819941641));
#45023=CARTESIAN_POINT('Ctrl Pts',(-0.200290353810089,0.00260302859526534,
0.00885467958226884));
#45024=CARTESIAN_POINT('Ctrl Pts',(-0.200291448570889,0.0026020425860909,
0.00885411375756756));
#45025=CARTESIAN_POINT('Ctrl Pts',(-0.200292333969178,0.00260137683365692,
0.00885372371479089));
#45026=CARTESIAN_POINT('Origin',(-0.199015160118143,0.0123433413565343,
0.00874522744837511));
#45027=CARTESIAN_POINT('Ctrl Pts',(-0.200176391911418,0.0122568678944164,
0.00882151754982349));
#45028=CARTESIAN_POINT('Ctrl Pts',(-0.20017636446585,0.0122608604306115,
0.00882797128920379));
#45029=CARTESIAN_POINT('Ctrl Pts',(-0.200177318434311,0.0122655116038751,
0.00883387049142189));
#45030=CARTESIAN_POINT('Ctrl Pts',(-0.200181324848676,0.0122768299522418,
0.00884544598348673));
#45031=CARTESIAN_POINT('Ctrl Pts',(-0.200184676853031,0.0122835225431615,
0.00885066860115435));
#45032=CARTESIAN_POINT('Ctrl Pts',(-0.200195420287465,0.012301379346308,
0.00886161958207752));
#45033=CARTESIAN_POINT('Ctrl Pts',(-0.200204430514006,0.0123135167776523,
0.00886623133374718));
#45034=CARTESIAN_POINT('Ctrl Pts',(-0.200225204203302,0.0123375397346441,
0.00887047629071223));
#45035=CARTESIAN_POINT('Ctrl Pts',(-0.200235993979062,0.0123486318822383,
0.00887044874845416));
#45036=CARTESIAN_POINT('Ctrl Pts',(-0.200260725447184,0.0123718830794046,
0.00886689271441571));
#45037=CARTESIAN_POINT('Ctrl Pts',(-0.200272949041827,0.0123818561551207,
0.00886277886901737));
#45038=CARTESIAN_POINT('Ctrl Pts',(-0.200281908067139,0.012388990717191,
0.00885921502571013));
#45039=CARTESIAN_POINT('Ctrl Pts',(-0.200284679859229,0.0123911072988095,
0.00885813444516822));
#45040=CARTESIAN_POINT('Ctrl Pts',(-0.200287457775747,0.0123931591103749,
0.00885696952162079));
#45041=CARTESIAN_POINT('Ctrl Pts',(-0.200288454700047,0.0123939097369423,
0.00885653037079223));
#45042=CARTESIAN_POINT('Ctrl Pts',(-0.200264179876147,0.00221381594909614,
0.00848015784889415));
#45043=CARTESIAN_POINT('Ctrl Pts',(-0.20026179025018,0.00215534095857477,
0.00856470365446266));
#45044=CARTESIAN_POINT('Ctrl Pts',(-0.200363797814067,0.00216614310006481,
0.00857172965097436));
#45045=CARTESIAN_POINT('Ctrl Pts',(-0.200125957436327,0.00304715701388984,
0.00905604306368936));
#45046=CARTESIAN_POINT('Ctrl Pts',(-0.200123320123447,0.00299777112378732,
0.00914692946592738));
#45047=CARTESIAN_POINT('Ctrl Pts',(-0.200224981899174,0.00301219654003019,
0.0091542509252648));
#45048=CARTESIAN_POINT('Ctrl Pts',(-0.199848200870376,0.00493136048449093,
0.00994083078053965));
#45049=CARTESIAN_POINT('Ctrl Pts',(-0.199845199746795,0.00490309257337129,
0.0100415783091978));
#45050=CARTESIAN_POINT('Ctrl Pts',(-0.199948841338395,0.00490294139784739,
0.0100388091649515));
#45051=CARTESIAN_POINT('Ctrl Pts',(-0.200061558378191,0.00700447670195284,
0.0101718827938119));
#45052=CARTESIAN_POINT('Ctrl Pts',(-0.200058430539336,0.00699885912125533,
0.0102751489227272));
#45053=CARTESIAN_POINT('Ctrl Pts',(-0.200160714440828,0.00698875414792091,
0.0102749221532313));
#45054=CARTESIAN_POINT('Ctrl Pts',(-0.200144088013061,0.00802290026385727,
0.0101153280660965));
#45055=CARTESIAN_POINT('Ctrl Pts',(-0.200140984359156,0.0080287326218905,
0.0102179459412791));
#45056=CARTESIAN_POINT('Ctrl Pts',(-0.200243492857047,0.00802043167606583,
0.0102186707749455));
#45057=CARTESIAN_POINT('Ctrl Pts',(-0.200100323214919,0.00749890966891628,
0.0101300471986839));
#45058=CARTESIAN_POINT('Ctrl Pts',(-0.200100175329577,0.0074989089326428,
0.0101365907504349));
#45059=CARTESIAN_POINT('Ctrl Pts',(-0.20010067256581,0.00749890851664256,
0.0101431326434737));
#45060=CARTESIAN_POINT('Ctrl Pts',(-0.200103014429842,0.00749890833111619,
0.0101564339958254));
#45061=CARTESIAN_POINT('Ctrl Pts',(-0.200104936024074,0.00749890860481728,
0.010163143686125));
#45062=CARTESIAN_POINT('Ctrl Pts',(-0.200112359078578,0.00749891042409756,
0.0101815446193971));
#45063=CARTESIAN_POINT('Ctrl Pts',(-0.200119444524665,0.0074989128359811,
0.0101924441940189));
#45064=CARTESIAN_POINT('Ctrl Pts',(-0.200137358813104,0.00749891985374453,
0.0102109668500448));
#45065=CARTESIAN_POINT('Ctrl Pts',(-0.200148021593063,0.00749892439464753,
0.0102184156855726));
#45066=CARTESIAN_POINT('Ctrl Pts',(-0.200175045045713,0.00749893661254169,
0.0102304232056775));
#45067=CARTESIAN_POINT('Ctrl Pts',(-0.200188714108781,0.00749893573954711,
0.0102320135358485));
#45068=CARTESIAN_POINT('Ctrl Pts',(-0.200197940246902,0.00749894856295794,
0.0102322820181257));
#45069=CARTESIAN_POINT('Ctrl Pts',(-0.200198400285571,0.00749894802607654,
0.0102322932741428));
#45070=CARTESIAN_POINT('Ctrl Pts',(-0.20035891519497,0.012829115342383,
0.00857491507414323));
#45071=CARTESIAN_POINT('Ctrl Pts',(-0.20025717573531,0.0128396259952154,
0.00856772156231838));
#45072=CARTESIAN_POINT('Ctrl Pts',(-0.200259586169385,0.0127813643735082,
0.00848337674133248));
#45073=CARTESIAN_POINT('Ctrl Pts',(-0.200221630466784,0.0119831507262477,
0.00915663829108513));
#45074=CARTESIAN_POINT('Ctrl Pts',(-0.200120232456941,0.0119972551590367,
0.00914913325111272));
#45075=CARTESIAN_POINT('Ctrl Pts',(-0.200122889507142,0.0119480558515039,
0.00905847473897322));
#45076=CARTESIAN_POINT('Ctrl Pts',(-0.199946820616977,0.0100930042470462,
0.0100396703535222));
#45077=CARTESIAN_POINT('Ctrl Pts',(-0.199843471700871,0.0100928272432444,
0.0100421051316997));
#45078=CARTESIAN_POINT('Ctrl Pts',(-0.199846491720836,0.0100646842389006,
0.00994162695940243));
#45079=CARTESIAN_POINT('Ctrl Pts',(-0.200159800951594,0.00800872160038045,
0.0102749558378368));
#45080=CARTESIAN_POINT('Ctrl Pts',(-0.200057812077642,0.00799849597590558,
0.0102748799873785));
#45081=CARTESIAN_POINT('Ctrl Pts',(-0.20006095755435,0.00799292564384356,
0.0101719009533559));
#45082=CARTESIAN_POINT('Ctrl Pts',(-0.200243718387518,0.00697783487179026,
0.0102185848089423));
#45083=CARTESIAN_POINT('Ctrl Pts',(-0.200141504405587,0.00696947970956505,
0.0102175413210191));
#45084=CARTESIAN_POINT('Ctrl Pts',(-0.200144625882982,0.00697531736293823,
0.0101152105196031));
#45085=CARTESIAN_POINT('Ctrl Pts',(-0.197152652670088,0.0021605811934014,
0.00850709261495718));
#45086=CARTESIAN_POINT('Ctrl Pts',(-0.197258645563439,0.00216678404947317,
0.00852161638163525));
#45087=CARTESIAN_POINT('Ctrl Pts',(-0.197259599012086,0.00222726834004635,
0.00843316287831881));
#45088=CARTESIAN_POINT('Ctrl Pts',(-0.197014009033787,0.00300933269914294,
0.00908736405676043));
#45089=CARTESIAN_POINT('Ctrl Pts',(-0.197119643888281,0.00301997324048751,
0.00910269918253681));
#45090=CARTESIAN_POINT('Ctrl Pts',(-0.197120849704256,0.00307094934136566,
0.00900768228901369));
#45091=CARTESIAN_POINT('Ctrl Pts',(-0.196743444704333,0.00490654029458651,
0.009969069964755));
#45092=CARTESIAN_POINT('Ctrl Pts',(-0.196851099911388,0.00490373400048392,
0.00997478148765791));
#45093=CARTESIAN_POINT('Ctrl Pts',(-0.196852720516954,0.00493300694734234,
0.00986977292339073));
#45094=CARTESIAN_POINT('Ctrl Pts',(-0.196953821593501,0.00699572957181629,
0.0102025186563745));
#45095=CARTESIAN_POINT('Ctrl Pts',(-0.197060039270723,0.0069848622369541,
0.0102112148095307));
#45096=CARTESIAN_POINT('Ctrl Pts',(-0.197061761627991,0.00699075765333439,
0.0101035576162893));
#45097=CARTESIAN_POINT('Ctrl Pts',(-0.197036936888857,0.00802867877765998,
0.0101456529653734));
#45098=CARTESIAN_POINT('Ctrl Pts',(-0.197143379084148,0.00802050281413876,
0.0101552409857996));
#45099=CARTESIAN_POINT('Ctrl Pts',(-0.197145083256844,0.00801450629794631,
0.0100482580482319));
#45100=CARTESIAN_POINT('Ctrl Pts',(-0.19708966640812,0.00259797400119342,
0.00878884298022014));
#45101=CARTESIAN_POINT('Ctrl Pts',(-0.197090422962005,0.00259871688481011,
0.00878930919013162));
#45102=CARTESIAN_POINT('Ctrl Pts',(-0.197092594086397,0.00260079696505936,
0.00879058153882454));
#45103=CARTESIAN_POINT('Ctrl Pts',(-0.197094756701536,0.00260293768788332,
0.00879176480312747));
#45104=CARTESIAN_POINT('Ctrl Pts',(-0.197101550058633,0.00260999384516736,
0.00879557393678802));
#45105=CARTESIAN_POINT('Ctrl Pts',(-0.197111121274289,0.00262007842499146,
0.00880021806540418));
#45106=CARTESIAN_POINT('Ctrl Pts',(-0.197131056914606,0.00264420422969141,
0.0088046346515727));
#45107=CARTESIAN_POINT('Ctrl Pts',(-0.197139629688112,0.00265550717491842,
0.00880490734767921));
#45108=CARTESIAN_POINT('Ctrl Pts',(-0.197156000870632,0.00267956982940497,
0.00880109254121348));
#45109=CARTESIAN_POINT('Ctrl Pts',(-0.197163116330695,0.00269160121674832,
0.00879668045913739));
#45110=CARTESIAN_POINT('Ctrl Pts',(-0.197171758146352,0.00270928700228767,
0.00878595857646887));
#45111=CARTESIAN_POINT('Ctrl Pts',(-0.197174442130602,0.00271578394302307,
0.00878087664097018));
#45112=CARTESIAN_POINT('Ctrl Pts',(-0.197177918132516,0.00272700868139428,
0.00876940382769687));
#45113=CARTESIAN_POINT('Ctrl Pts',(-0.197178837227364,0.00273173408342081,
0.00876331200781784));
#45114=CARTESIAN_POINT('Ctrl Pts',(-0.197178963584415,0.00273573528602628,
0.00875664828842276));
#45115=CARTESIAN_POINT('Ctrl Pts',(-0.197101855005559,0.00749734545555895,
0.0100625711568172));
#45116=CARTESIAN_POINT('Ctrl Pts',(-0.197101690442853,0.00749734357232736,
0.0100690161322291));
#45117=CARTESIAN_POINT('Ctrl Pts',(-0.197100900765169,0.00749734148888539,
0.0100754298692072));
#45118=CARTESIAN_POINT('Ctrl Pts',(-0.197097981899033,0.00749733679991958,
0.0100885161664239));
#45119=CARTESIAN_POINT('Ctrl Pts',(-0.197095759406202,0.00749733417927401,
0.0100951318714899));
#45120=CARTESIAN_POINT('Ctrl Pts',(-0.197087513364756,0.00749732629771051,
0.0101131783932643));
#45121=CARTESIAN_POINT('Ctrl Pts',(-0.197079943180104,0.00749732076252694,
0.0101237468493541));
#45122=CARTESIAN_POINT('Ctrl Pts',(-0.197061211216097,0.00749730944906349,
0.0101414416276148));
#45123=CARTESIAN_POINT('Ctrl Pts',(-0.197050223203192,0.00749730378248083,
0.0101484013861565));
#45124=CARTESIAN_POINT('Ctrl Pts',(-0.197018046539333,0.0074972892795021,
0.0101609916103687));
#45125=CARTESIAN_POINT('Ctrl Pts',(-0.197001302675901,0.00749729577011255,
0.0101600246187684));
#45126=CARTESIAN_POINT('Ctrl Pts',(-0.19699971712443,0.00749726941310258,
0.0101599992595542));
#45127=CARTESIAN_POINT('Ctrl Pts',(-0.196999275842678,0.00749728354040296,
0.0101599900590452));
#45128=CARTESIAN_POINT('Ctrl Pts',(-0.197256820089405,0.0127679866759842,
0.00843621590655516));
#45129=CARTESIAN_POINT('Ctrl Pts',(-0.197255983919717,0.0128285304405105,
0.00852489944995749));
#45130=CARTESIAN_POINT('Ctrl Pts',(-0.197149776203591,0.0128346755026245,
0.00851027926216887));
#45131=CARTESIAN_POINT('Ctrl Pts',(-0.197118253662537,0.0119239787910673,
0.00901021072020725));
#45132=CARTESIAN_POINT('Ctrl Pts',(-0.197117164455696,0.0119749872889838,
0.0091054653969711));
#45133=CARTESIAN_POINT('Ctrl Pts',(-0.197011315898106,0.0119856063978868,
0.00909002022551536));
#45134=CARTESIAN_POINT('Ctrl Pts',(-0.196850600591309,0.0100615170300595,
0.00987110312810501));
#45135=CARTESIAN_POINT('Ctrl Pts',(-0.196849098706584,0.0100907877610896,
0.00997634525975825));
#45136=CARTESIAN_POINT('Ctrl Pts',(-0.196741224795717,0.0100878459637636,
0.00997055758727937));
#45137=CARTESIAN_POINT('Ctrl Pts',(-0.197061500370654,0.00800384808569401,
0.0101037236165437));
#45138=CARTESIAN_POINT('Ctrl Pts',(-0.19705989562741,0.00800970369698869,
0.0102116092393013));
#45139=CARTESIAN_POINT('Ctrl Pts',(-0.196953473326002,0.00799874894913888,
0.0102027890447947));
#45140=CARTESIAN_POINT('Ctrl Pts',(-0.197145405828628,0.00698025475593223,
0.0100478570432307));
#45141=CARTESIAN_POINT('Ctrl Pts',(-0.197143819563754,0.00697419554098605,
0.0101550610895007));
#45142=CARTESIAN_POINT('Ctrl Pts',(-0.197037170579532,0.00696594143372946,
0.0101453456903674));
#45143=CARTESIAN_POINT('Ctrl Pts',(-0.197176298810346,0.0122593881381477,
0.00875948681888613));
#45144=CARTESIAN_POINT('Ctrl Pts',(-0.197176176439832,0.0122632507361322,
0.0087659306057829));
#45145=CARTESIAN_POINT('Ctrl Pts',(-0.197175313201552,0.0122677917440443,
0.00877184319222938));
#45146=CARTESIAN_POINT('Ctrl Pts',(-0.197172053774191,0.0122785410350562,
0.00878301774032121));
#45147=CARTESIAN_POINT('Ctrl Pts',(-0.197169541543235,0.0122847481433668,
0.0087880082107202));
#45148=CARTESIAN_POINT('Ctrl Pts',(-0.197161307159831,0.0123019228673441,
0.00879882601323132));
#45149=CARTESIAN_POINT('Ctrl Pts',(-0.197154411747571,0.0123137493536575,
0.00880341874342543));
#45150=CARTESIAN_POINT('Ctrl Pts',(-0.197137656856923,0.0123386748828606,
0.00880790236212758));
#45151=CARTESIAN_POINT('Ctrl Pts',(-0.197128297243567,0.0123510214261447,
0.00880764252441401));
#45152=CARTESIAN_POINT('Ctrl Pts',(-0.197104538659764,0.0123795609881269,
0.00880212446974175));
#45153=CARTESIAN_POINT('Ctrl Pts',(-0.197093039129748,0.0123911488545319,
0.00879532119320332));
#45154=CARTESIAN_POINT('Ctrl Pts',(-0.197089059974131,0.0123947079343662,
0.00879324060162505));
#45155=CARTESIAN_POINT('Ctrl Pts',(-0.19708846547414,0.012395450350782,
0.00879279541010521));
#45156=CARTESIAN_POINT('Ctrl Pts',(-0.197087666832481,0.0123964431722424,
0.00879219355122506));
#45157=CARTESIAN_POINT('Ctrl Pts',(-0.19708698285431,0.0123971147297022,
0.00879177268117346));
#45158=CARTESIAN_POINT('Origin',(-0.198342348487265,0.00265133456699769,
0.00872878636643693));
#45159=CARTESIAN_POINT('Ctrl Pts',(-0.198179411628685,0.00273625916616763,
0.00877798858090942));
#45160=CARTESIAN_POINT('Ctrl Pts',(-0.19817938500885,0.00273217717639081,
0.0087846072054196));
#45161=CARTESIAN_POINT('Ctrl Pts',(-0.198180389211287,0.00272740441884125,
0.00879064180724154));
#45162=CARTESIAN_POINT('Ctrl Pts',(-0.198184597990081,0.00271575815394672,
0.00880245994552571));
#45163=CARTESIAN_POINT('Ctrl Pts',(-0.19818811996947,0.00270885869545007,
0.00880776021054462));
#45164=CARTESIAN_POINT('Ctrl Pts',(-0.198199277211723,0.00269062642511689,
0.00881869335267521));
#45165=CARTESIAN_POINT('Ctrl Pts',(-0.198208539838762,0.00267831376926954,
0.00882320585945375));
#45166=CARTESIAN_POINT('Ctrl Pts',(-0.198230164370323,0.00265360052534109,
0.00882722432949729));
#45167=CARTESIAN_POINT('Ctrl Pts',(-0.198241608709373,0.00264201182077982,
0.00882694238263359));
#45168=CARTESIAN_POINT('Ctrl Pts',(-0.198270526973544,0.00261533210442332,
0.0088220795568075));
#45169=CARTESIAN_POINT('Ctrl Pts',(-0.19828458157657,0.00260448296114289,
0.00881606909428004));
#45170=CARTESIAN_POINT('Ctrl Pts',(-0.198289191848955,0.00260135615922656,
0.00881437505335988));
#45171=CARTESIAN_POINT('Ctrl Pts',(-0.198289866723518,0.00260070421971694,
0.00881400226185802));
#45172=CARTESIAN_POINT('Ctrl Pts',(-0.198290773684868,0.00259983144512114,
0.00881349978351456));
#45173=CARTESIAN_POINT('Ctrl Pts',(-0.198291531830531,0.00259926033540328,
0.00881316668848207));
#45174=CARTESIAN_POINT('Origin',(-0.197012620205462,0.0123453294618211,
0.00870476452362944));
#45175=CARTESIAN_POINT('Ctrl Pts',(-0.198174121550572,0.0122590158781096,
0.00878068088066938));
#45176=CARTESIAN_POINT('Ctrl Pts',(-0.198174094633242,0.012262978212402,
0.0087871132810639));
#45177=CARTESIAN_POINT('Ctrl Pts',(-0.198175038857425,0.0122675950228917,
0.00879299782819372));
#45178=CARTESIAN_POINT('Ctrl Pts',(-0.198179006095641,0.0122788340702126,
0.00880455626725186));
#45179=CARTESIAN_POINT('Ctrl Pts',(-0.198182326296455,0.0122854833920715,
0.00880978080657457));
#45180=CARTESIAN_POINT('Ctrl Pts',(-0.198192988871284,0.0123032595928686,
0.00882077167374966));
#45181=CARTESIAN_POINT('Ctrl Pts',(-0.198201945539821,0.0123153606316044,
0.00882542376076332));
#45182=CARTESIAN_POINT('Ctrl Pts',(-0.198222665756589,0.0123393976026421,
0.00882977557378687));
#45183=CARTESIAN_POINT('Ctrl Pts',(-0.198233470933688,0.0123505370415491,
0.00882978651421305));
#45184=CARTESIAN_POINT('Ctrl Pts',(-0.198258231999181,0.0123738810923607,
0.00882628789418516));
#45185=CARTESIAN_POINT('Ctrl Pts',(-0.19827047719199,0.0123839022446484,
0.00882218439658351));
#45186=CARTESIAN_POINT('Ctrl Pts',(-0.198279479382352,0.0123910906192307,
0.00881861094792741));
#45187=CARTESIAN_POINT('Ctrl Pts',(-0.198282242019807,0.0123932064780831,
0.00881753555986399));
#45188=CARTESIAN_POINT('Ctrl Pts',(-0.198285010804024,0.0123952581516283,
0.00881637615689229));
#45189=CARTESIAN_POINT('Ctrl Pts',(-0.198286011292521,0.0123960137502511,
0.00881593605607644));
#45190=CARTESIAN_POINT('Ctrl Pts',(-0.198263015582683,0.00221100833647082,
0.00844046058749481));
#45191=CARTESIAN_POINT('Ctrl Pts',(-0.198260617033187,0.00215267264060678,
0.00852519920881164));
#45192=CARTESIAN_POINT('Ctrl Pts',(-0.198362711813689,0.00216348282904155,
0.00853210786931248));
#45193=CARTESIAN_POINT('Ctrl Pts',(-0.198125466898689,0.00304557461821688,
0.00901447908689848));
#45194=CARTESIAN_POINT('Ctrl Pts',(-0.198122819594458,0.00299631796672872,
0.00910552077863998));
#45195=CARTESIAN_POINT('Ctrl Pts',(-0.198224571337662,0.00301073675780382,
0.00911272370854456));
#45196=CARTESIAN_POINT('Ctrl Pts',(-0.197849391405799,0.00493093979824749,
0.00989615351262796));
#45197=CARTESIAN_POINT('Ctrl Pts',(-0.197846378014324,0.00490274745865633,
0.00999699175877014));
#45198=CARTESIAN_POINT('Ctrl Pts',(-0.197950095003213,0.00490255268693708,
0.00999415547963392));
#45199=CARTESIAN_POINT('Ctrl Pts',(-0.198062615765221,0.00700335854996127,
0.0101264491950313));
#45200=CARTESIAN_POINT('Ctrl Pts',(-0.198059475798075,0.00699774833958211,
0.0102297907905905));
#45201=CARTESIAN_POINT('Ctrl Pts',(-0.198161840565047,0.00698765712520676,
0.0102294964296498));
#45202=CARTESIAN_POINT('Ctrl Pts',(-0.198145063363228,0.00802177486531964,
0.01007026479514));
#45203=CARTESIAN_POINT('Ctrl Pts',(-0.198141947620127,0.00802757715642436,
0.0101729638783758));
#45204=CARTESIAN_POINT('Ctrl Pts',(-0.198244536051857,0.00801926856690324,
0.0101736154882906));
#45205=CARTESIAN_POINT('Ctrl Pts',(-0.198101337934465,0.00749782688006727,
0.0100848682832439));
#45206=CARTESIAN_POINT('Ctrl Pts',(-0.198101190049774,0.00749782537457631,
0.010091411792284));
#45207=CARTESIAN_POINT('Ctrl Pts',(-0.198101687271057,0.00749782413947803,
0.0100979536440257));
#45208=CARTESIAN_POINT('Ctrl Pts',(-0.198104029073436,0.0074978221853558,
0.0101112549096639));
#45209=CARTESIAN_POINT('Ctrl Pts',(-0.198105950618229,0.00749782150952789,
0.0101179645588641));
#45210=CARTESIAN_POINT('Ctrl Pts',(-0.198113373509982,0.00749782055821905,
0.0101363654365789));
#45211=CARTESIAN_POINT('Ctrl Pts',(-0.198120458831957,0.0074978211208926,
0.0101472650224001));
#45212=CARTESIAN_POINT('Ctrl Pts',(-0.198138372856713,0.00749782454491441,
0.0101657877107848));
#45213=CARTESIAN_POINT('Ctrl Pts',(-0.19814903548975,0.00749782737340509,
0.0101732365777307));
#45214=CARTESIAN_POINT('Ctrl Pts',(-0.198172666729056,0.00749783500127251,
0.0101837369998498));
#45215=CARTESIAN_POINT('Ctrl Pts',(-0.198185793394253,0.0074977794521,0.0101867201386191));
#45216=CARTESIAN_POINT('Ctrl Pts',(-0.198198977094684,0.00749784953224362,
0.010187103726467));
#45217=CARTESIAN_POINT('Ctrl Pts',(-0.19819941389096,0.00749784541675471,
0.0101871143080195));
#45218=CARTESIAN_POINT('Ctrl Pts',(-0.198355693142376,0.0128319883322708,
0.0085350931304057));
#45219=CARTESIAN_POINT('Ctrl Pts',(-0.198253902786949,0.0128424016903643,
0.00852802812650304));
#45220=CARTESIAN_POINT('Ctrl Pts',(-0.198256323072633,0.0127843040832604,
0.00844353196650278));
#45221=CARTESIAN_POINT('Ctrl Pts',(-0.198219976457811,0.0119843975857885,
0.00911525593693403));
#45222=CARTESIAN_POINT('Ctrl Pts',(-0.198118520413737,0.0119983691518567,
0.00910787819325317));
#45223=CARTESIAN_POINT('Ctrl Pts',(-0.198121188461898,0.0119493251148045,
0.00901710497314409));
#45224=CARTESIAN_POINT('Ctrl Pts',(-0.197948583145872,0.0100922420607575,
0.00999549380886804));
#45225=CARTESIAN_POINT('Ctrl Pts',(-0.197845215243418,0.0100919920353229,
0.00999793656072922));
#45226=CARTESIAN_POINT('Ctrl Pts',(-0.197848249040959,0.0100639502008642,
0.00989740899395634));
#45227=CARTESIAN_POINT('Ctrl Pts',(-0.198160910579588,0.00800779606522802,
0.0102296858131739));
#45228=CARTESIAN_POINT('Ctrl Pts',(-0.19805888569194,0.00799760825584394,
0.0102296242114142));
#45229=CARTESIAN_POINT('Ctrl Pts',(-0.198062044056392,0.0079920701657748,
0.0101266163930227));
#45230=CARTESIAN_POINT('Ctrl Pts',(-0.198244657667604,0.00697658890091374,
0.0101733935029984));
#45231=CARTESIAN_POINT('Ctrl Pts',(-0.198142410611714,0.00696824631768505,
0.0101723721389504));
#45232=CARTESIAN_POINT('Ctrl Pts',(-0.198145544916776,0.00697407769767305,
0.0100700094381033));
#45233=CARTESIAN_POINT('Ctrl Pts',(-0.195151474094836,0.0021581839665313,
0.00846785476566089));
#45234=CARTESIAN_POINT('Ctrl Pts',(-0.19525748673727,0.00216438162946169,
0.00848230606819899));
#45235=CARTESIAN_POINT('Ctrl Pts',(-0.19525840470211,0.00222466604303826,
0.00839370419046678));
#45236=CARTESIAN_POINT('Ctrl Pts',(-0.195013516634162,0.00300817193503215,
0.00904611630303382));
#45237=CARTESIAN_POINT('Ctrl Pts',(-0.195119173493743,0.00301878746404222,
0.00906137595421988));
#45238=CARTESIAN_POINT('Ctrl Pts',(-0.195120345017048,0.00306957996306731,
0.00896625564857248));
#45239=CARTESIAN_POINT('Ctrl Pts',(-0.194744239513626,0.00490645046054183,
0.00992449906340472));
#45240=CARTESIAN_POINT('Ctrl Pts',(-0.194851902096146,0.00490363285336936,
0.00993020117251484));
#45241=CARTESIAN_POINT('Ctrl Pts',(-0.194853488851879,0.00493280240147255,
0.00982516951400271));
#45242=CARTESIAN_POINT('Ctrl Pts',(-0.194954744898083,0.00699491874387549,
0.0101570965807732));
#45243=CARTESIAN_POINT('Ctrl Pts',(-0.195060972979,0.00698403600339864,
0.0101657685812465));
#45244=CARTESIAN_POINT('Ctrl Pts',(-0.195062662204119,0.00698991992030242,
0.0100581059040497));
#45245=CARTESIAN_POINT('Ctrl Pts',(-0.195038044064419,0.00802772507301438,
0.0101005930890543));
#45246=CARTESIAN_POINT('Ctrl Pts',(-0.195144496335863,0.00801952667954973,
0.0101101565321198));
#45247=CARTESIAN_POINT('Ctrl Pts',(-0.195146167232292,0.0080135677939633,
0.0100031613552704));
#45248=CARTESIAN_POINT('Ctrl Pts',(-0.195088807996151,0.00259613933341528,
0.00874861478558778));
#45249=CARTESIAN_POINT('Ctrl Pts',(-0.195089568324798,0.00259688621242362,
0.00874908133152229));
#45250=CARTESIAN_POINT('Ctrl Pts',(-0.195091737536302,0.00259896565877408,
0.00875034712361913));
#45251=CARTESIAN_POINT('Ctrl Pts',(-0.195093898259448,0.00260110526380068,
0.00875152411652745));
#45252=CARTESIAN_POINT('Ctrl Pts',(-0.195100715212568,0.00260818642304804,
0.00875532749998801));
#45253=CARTESIAN_POINT('Ctrl Pts',(-0.195110287808044,0.00261827529366409,
0.00875994272695168));
#45254=CARTESIAN_POINT('Ctrl Pts',(-0.195130224176016,0.00264239001717091,
0.00876430394263768));
#45255=CARTESIAN_POINT('Ctrl Pts',(-0.195138802238907,0.00265369079223031,
0.00876455232971158));
#45256=CARTESIAN_POINT('Ctrl Pts',(-0.1951551844026,0.00267774154735868,
0.00876068640337326));
#45257=CARTESIAN_POINT('Ctrl Pts',(-0.195162304784493,0.00268976245709861,
0.00875624883714372));
#45258=CARTESIAN_POINT('Ctrl Pts',(-0.195170952608934,0.00270742477528601,
0.00874548965920323));
#45259=CARTESIAN_POINT('Ctrl Pts',(-0.195173638543081,0.00271391111696078,
0.00874039389129896));
#45260=CARTESIAN_POINT('Ctrl Pts',(-0.195177116914226,0.00272511226812696,
0.0087288969971338));
#45261=CARTESIAN_POINT('Ctrl Pts',(-0.195178036555258,0.00272982522991645,
0.00872279506055263));
#45262=CARTESIAN_POINT('Ctrl Pts',(-0.195178162823842,0.00273381293378166,
0.00871612270254606));
#45263=CARTESIAN_POINT('Ctrl Pts',(-0.195102853656511,0.00749647337670453,
0.0100174036489879));
#45264=CARTESIAN_POINT('Ctrl Pts',(-0.195102688430028,0.00749647092519468,
0.0100238445717337));
#45265=CARTESIAN_POINT('Ctrl Pts',(-0.19510189888294,0.0074964684868887,
0.0100302542422684));
#45266=CARTESIAN_POINT('Ctrl Pts',(-0.195098980964152,0.00749646351205413,
0.0100433365704581));
#45267=CARTESIAN_POINT('Ctrl Pts',(-0.195096758536737,0.00749646099736017,
0.0100499522302527));
#45268=CARTESIAN_POINT('Ctrl Pts',(-0.195088512706634,0.00749645413866188,
0.0100679986980086));
#45269=CARTESIAN_POINT('Ctrl Pts',(-0.195080942680449,0.00749645012399971,
0.0100785671796805));
#45270=CARTESIAN_POINT('Ctrl Pts',(-0.195062211056929,0.00749644338711119,
0.0100962620160301));
#45271=CARTESIAN_POINT('Ctrl Pts',(-0.195051223236752,0.00749644073745807,
0.0101032218231675));
#45272=CARTESIAN_POINT('Ctrl Pts',(-0.195019263724858,0.00749643580110644,
0.0101157274017836));
#45273=CARTESIAN_POINT('Ctrl Pts',(-0.195002697944291,0.00749646333374549,
0.0101148515365255));
#45274=CARTESIAN_POINT('Ctrl Pts',(-0.195000719135785,0.00749641518058753,
0.0101148199248467));
#45275=CARTESIAN_POINT('Ctrl Pts',(-0.195000276360688,0.00749643658133645,
0.0101148106853962));
#45276=CARTESIAN_POINT('Ctrl Pts',(-0.195258464889861,0.0127716222143721,
0.00839609631068042));
#45277=CARTESIAN_POINT('Ctrl Pts',(-0.195257661598623,0.0128320002529834,
0.00848495188464948));
#45278=CARTESIAN_POINT('Ctrl Pts',(-0.195151404514474,0.0128381542818839,
0.008470338536568));
#45279=CARTESIAN_POINT('Ctrl Pts',(-0.195119985170156,0.0119260586777307,
0.0089685011811852));
#45280=CARTESIAN_POINT('Ctrl Pts',(-0.195118927457144,0.0119769105830198,
0.00906388973756854));
#45281=CARTESIAN_POINT('Ctrl Pts',(-0.195013028416401,0.0119875277897504,
0.00904845632888441));
#45282=CARTESIAN_POINT('Ctrl Pts',(-0.194853120499905,0.0100615551736861,
0.00982677140189363));
#45283=CARTESIAN_POINT('Ctrl Pts',(-0.194851649079398,0.0100907329171985,
0.00993207689887392));
#45284=CARTESIAN_POINT('Ctrl Pts',(-0.19474373346643,0.0100878065962746,
0.00992624268005921));
#45285=CARTESIAN_POINT('Ctrl Pts',(-0.195062697269868,0.00800323442767928,
0.0100584301848728));
#45286=CARTESIAN_POINT('Ctrl Pts',(-0.195061122180014,0.0080090637473043,
0.0101663618724557));
#45287=CARTESIAN_POINT('Ctrl Pts',(-0.194954647414871,0.00799816636004166,
0.0101575142891252));
#45288=CARTESIAN_POINT('Ctrl Pts',(-0.195146171428379,0.00697914415917188,
0.0100026415787786));
#45289=CARTESIAN_POINT('Ctrl Pts',(-0.195144615154365,0.00697309723419385,
0.0101098951507728));
#45290=CARTESIAN_POINT('Ctrl Pts',(-0.195037915324914,0.00696489230979399,
0.0101001621065224));
#45291=CARTESIAN_POINT('Ctrl Pts',(-0.195178017022907,0.0122621355963516,
0.00871851959969473));
#45292=CARTESIAN_POINT('Ctrl Pts',(-0.195177580509937,0.0122758282388325,
0.00874146027159947));
#45293=CARTESIAN_POINT('Ctrl Pts',(-0.195163460529544,0.012307420071114,
0.00876039280475504));
#45294=CARTESIAN_POINT('Ctrl Pts',(-0.195146437813832,0.0123308055228815,
0.00876514629123138));
#45295=CARTESIAN_POINT('Ctrl Pts',(-0.195131119021796,0.0123518501598455,
0.00876942396772028));
#45296=CARTESIAN_POINT('Ctrl Pts',(-0.195119235232368,0.0123684243934701,
0.00876737961119782));
#45297=CARTESIAN_POINT('Ctrl Pts',(-0.195096603924478,0.0123918748609315,
0.00875552780766066));
#45298=CARTESIAN_POINT('Ctrl Pts',(-0.195094086595983,0.0123944833062879,
0.00875420950635378));
#45299=CARTESIAN_POINT('Ctrl Pts',(-0.19509144745469,0.0123971472448317,
0.00875272329131383));
#45300=CARTESIAN_POINT('Ctrl Pts',(-0.195088692557014,0.012399858493754,
0.00875103165054581));
#45301=CARTESIAN_POINT('Origin',(-0.196341530644781,0.00264910622819491,
0.00868825771150032));
#45302=CARTESIAN_POINT('Ctrl Pts',(-0.196178605749969,0.00273416037407678,
0.00873731991783359));
#45303=CARTESIAN_POINT('Ctrl Pts',(-0.196178579860494,0.00273009299958139,
0.00874394353981102));
#45304=CARTESIAN_POINT('Ctrl Pts',(-0.196179583205907,0.00272533404646618,
0.00874998493616834));
#45305=CARTESIAN_POINT('Ctrl Pts',(-0.196183787973507,0.00271371373445172,
0.00876182314931958));
#45306=CARTESIAN_POINT('Ctrl Pts',(-0.196187307070579,0.00270682499517073,
0.0087671365420531));
#45307=CARTESIAN_POINT('Ctrl Pts',(-0.196198455940222,0.00268861365389419,
0.00877810476957485));
#45308=CARTESIAN_POINT('Ctrl Pts',(-0.196207711713408,0.00267630899606189,
0.00878264090943895));
#45309=CARTESIAN_POINT('Ctrl Pts',(-0.196229260457889,0.0026516694477696,
0.00878669559224456));
#45310=CARTESIAN_POINT('Ctrl Pts',(-0.196240624737327,0.00264014354081433,
0.00878645001839778));
#45311=CARTESIAN_POINT('Ctrl Pts',(-0.1962692611573,0.00261366083176474,
0.00878172908321917));
#45312=CARTESIAN_POINT('Ctrl Pts',(-0.196283191869981,0.00260288006357014,
0.00877586776937855));
#45313=CARTESIAN_POINT('Ctrl Pts',(-0.196287978139581,0.00259953252469863,
0.0087740737788129));
#45314=CARTESIAN_POINT('Ctrl Pts',(-0.196288756787266,0.00259881568571221,
0.0087736695208446));
#45315=CARTESIAN_POINT('Ctrl Pts',(-0.196289802132512,0.00259785720803007,
0.00877312348153903));
#45316=CARTESIAN_POINT('Ctrl Pts',(-0.196290653689677,0.00259721438487426,
0.00877275027888147));
#45317=CARTESIAN_POINT('Origin',(-0.195016314063637,0.0123482798341224,
0.00866394192729312));
#45318=CARTESIAN_POINT('Ctrl Pts',(-0.196177629385444,0.0122611626189316,
0.00874006375723914));
#45319=CARTESIAN_POINT('Ctrl Pts',(-0.196177604684899,0.0122650166111309,
0.00874634656815966));
#45320=CARTESIAN_POINT('Ctrl Pts',(-0.196178505761057,0.0122694952960258,
0.00875211144220574));
#45321=CARTESIAN_POINT('Ctrl Pts',(-0.196182296395684,0.0122803850364228,
0.00876347360160108));
#45322=CARTESIAN_POINT('Ctrl Pts',(-0.196185470343792,0.0122868251469942,
0.0087686457365702));
#45323=CARTESIAN_POINT('Ctrl Pts',(-0.196195776348067,0.0123042086992948,
0.00877970743094284));
#45324=CARTESIAN_POINT('Ctrl Pts',(-0.196204518680032,0.0123161242904747,
0.00878449099801561));
#45325=CARTESIAN_POINT('Ctrl Pts',(-0.196225148046997,0.0123402424928695,
0.00878927088270124));
#45326=CARTESIAN_POINT('Ctrl Pts',(-0.19623615481724,0.0123516331750604,
0.00878941853515255));
#45327=CARTESIAN_POINT('Ctrl Pts',(-0.196261828351012,0.0123758886765458,
0.00878601069113465));
#45328=CARTESIAN_POINT('Ctrl Pts',(-0.196274345460426,0.0123860640870079,
0.00878176003385096));
#45329=CARTESIAN_POINT('Ctrl Pts',(-0.19628311218831,0.0123930638981874,
0.0087782975856912));
#45330=CARTESIAN_POINT('Ctrl Pts',(-0.196285923619682,0.0123952124629935,
0.00877721360122813));
#45331=CARTESIAN_POINT('Ctrl Pts',(-0.196288741215603,0.0123972935671941,
0.00877604129610507));
#45332=CARTESIAN_POINT('Ctrl Pts',(-0.196289697990218,0.0123980152811994,
0.00877562292559277));
#45333=CARTESIAN_POINT('Ctrl Pts',(-0.196261761273723,0.00220825086283849,
0.00840092612408506));
#45334=CARTESIAN_POINT('Ctrl Pts',(-0.196259359103124,0.00215010776402942,
0.00848578996319967));
#45335=CARTESIAN_POINT('Ctrl Pts',(-0.196361456778984,0.0021608707734272,
0.00849264249435443));
#45336=CARTESIAN_POINT('Ctrl Pts',(-0.196124935041166,0.00304408419344697,
0.00897303747973618));
#45337=CARTESIAN_POINT('Ctrl Pts',(-0.196122283249963,0.00299500238841375,
0.00906416088238421));
#45338=CARTESIAN_POINT('Ctrl Pts',(-0.19622404056787,0.00300935915833106,
0.00907131055929637));
#45339=CARTESIAN_POINT('Ctrl Pts',(-0.195850357502235,0.00493054266441542,
0.00985151168271769));
#45340=CARTESIAN_POINT('Ctrl Pts',(-0.195847337738017,0.0049024516121403,
0.00995235738966955));
#45341=CARTESIAN_POINT('Ctrl Pts',(-0.195951044646213,0.0049022109327829,
0.00994954044800188));
#45342=CARTESIAN_POINT('Ctrl Pts',(-0.196063682956604,0.00700246999388266,
0.0100810223901609));
#45343=CARTESIAN_POINT('Ctrl Pts',(-0.196060536777505,0.00699687455558653,
0.0101843537059636));
#45344=CARTESIAN_POINT('Ctrl Pts',(-0.196162895346769,0.00698677679606697,
0.0101840722583427));
#45345=CARTESIAN_POINT('Ctrl Pts',(-0.19614623552346,0.00802067462636459,
0.0100252039093978));
#45346=CARTESIAN_POINT('Ctrl Pts',(-0.196143113583024,0.00802644166365842,
0.0101278989422097));
#45347=CARTESIAN_POINT('Ctrl Pts',(-0.196245695189478,0.00801812145293573,
0.0101285601406757));
#45348=CARTESIAN_POINT('Ctrl Pts',(-0.196102458894692,0.00749683730988234,
0.0100396916414689));
#45349=CARTESIAN_POINT('Ctrl Pts',(-0.196102311008966,0.00749683509874942,
0.0100462351503637));
#45350=CARTESIAN_POINT('Ctrl Pts',(-0.196102808227049,0.00749683305950545,
0.0100527770024187));
#45351=CARTESIAN_POINT('Ctrl Pts',(-0.196105150018785,0.00749682926719129,
0.0100660782667755));
#45352=CARTESIAN_POINT('Ctrl Pts',(-0.196107071555501,0.00749682755110485,
0.010072787915366));
#45353=CARTESIAN_POINT('Ctrl Pts',(-0.196114494416142,0.00749682341853911,
0.0100911887837042));
#45354=CARTESIAN_POINT('Ctrl Pts',(-0.196121579709176,0.00749682168655211,
0.0101020883679008));
#45355=CARTESIAN_POINT('Ctrl Pts',(-0.196139493665661,0.00749682031724726,
0.0101206110477672));
#45356=CARTESIAN_POINT('Ctrl Pts',(-0.196150156255171,0.00749682068764585,
0.0101280599128218));
#45357=CARTESIAN_POINT('Ctrl Pts',(-0.196181811356627,0.0074968245635932,
0.0101421257479467));
#45358=CARTESIAN_POINT('Ctrl Pts',(-0.196198651212673,0.00749682018921974,
0.0101418849547825));
#45359=CARTESIAN_POINT('Ctrl Pts',(-0.196200096295123,0.0074968426416852,
0.0101419270317423));
#45360=CARTESIAN_POINT('Ctrl Pts',(-0.196200203314133,0.00749682939312149,
0.0101419301637073));
#45361=CARTESIAN_POINT('Ctrl Pts',(-0.196200533508802,0.00749682933724156,
0.0101419376171861));
#45362=CARTESIAN_POINT('Ctrl Pts',(-0.19636080552077,0.0128345631145169,
0.00849574728918621));
#45363=CARTESIAN_POINT('Ctrl Pts',(-0.196258557059731,0.0128454370666705,
0.0084889752095364));
#45364=CARTESIAN_POINT('Ctrl Pts',(-0.19626099705554,0.0127872520572483,
0.00840395151994793));
#45365=CARTESIAN_POINT('Ctrl Pts',(-0.196223005201044,0.0119856357125536,
0.00907398755842464));
#45366=CARTESIAN_POINT('Ctrl Pts',(-0.196121099622317,0.0120001214234957,
0.00906692248765129));
#45367=CARTESIAN_POINT('Ctrl Pts',(-0.196123789273586,0.0119510144111196,
0.00897563473339434));
#45368=CARTESIAN_POINT('Ctrl Pts',(-0.195949420026854,0.0100919430838383,
0.0099511818246222));
#45369=CARTESIAN_POINT('Ctrl Pts',(-0.195845548801905,0.0100916748893939,
0.00995415151336621));
#45370=CARTESIAN_POINT('Ctrl Pts',(-0.195848607042909,0.0100636041876074,
0.0098531341357168));
#45371=CARTESIAN_POINT('Ctrl Pts',(-0.196162792162144,0.00800692503941795,
0.0101844280639557));
#45372=CARTESIAN_POINT('Ctrl Pts',(-0.196060284308471,0.00799676411255229,
0.0101848280330257));
#45373=CARTESIAN_POINT('Ctrl Pts',(-0.196063468158884,0.00799123551783281,
0.010081336579869));
#45374=CARTESIAN_POINT('Ctrl Pts',(-0.196246080332815,0.00697549324604494,
0.0101282087141702));
#45375=CARTESIAN_POINT('Ctrl Pts',(-0.196143346637859,0.00696709994606931,
0.0101276618554586));
#45376=CARTESIAN_POINT('Ctrl Pts',(-0.196146506172932,0.00697294832614626,
0.0100248157795735));
#45377=CARTESIAN_POINT('Ctrl Pts',(-0.221150461937767,0.00811962085575298,
0.0105825552134681));
#45378=CARTESIAN_POINT('Ctrl Pts',(-0.2211495396963,0.00812732088454214,
0.0106927229483897));
#45379=CARTESIAN_POINT('Ctrl Pts',(-0.221040101821991,0.00813555022692369,
0.0106801850925946));
#45380=CARTESIAN_POINT('Ctrl Pts',(-0.221032677065535,0.00689153715468521,
0.0106668145952798));
#45381=CARTESIAN_POINT('Ctrl Pts',(-0.22103172824819,0.00688383601422594,
0.0107780583691776));
#45382=CARTESIAN_POINT('Ctrl Pts',(-0.220922567010128,0.00689630991786673,
0.0107669036634824));
#45383=CARTESIAN_POINT('Ctrl Pts',(-0.220896608196396,0.0050972250828522,
0.0104177246389459));
#45384=CARTESIAN_POINT('Ctrl Pts',(-0.220895752802238,0.00506778132256289,
0.0105259415777043));
#45385=CARTESIAN_POINT('Ctrl Pts',(-0.220785305656289,0.00507181257794575,
0.0105169696830634));
#45386=CARTESIAN_POINT('Ctrl Pts',(-0.221099672568277,0.00282025323552542,
0.00935943618997168));
#45387=CARTESIAN_POINT('Ctrl Pts',(-0.221099319942786,0.00276243769422579,
0.00945448593572196));
#45388=CARTESIAN_POINT('Ctrl Pts',(-0.220990565430845,0.00275247842578777,
0.00943635408645135));
#45389=CARTESIAN_POINT('Ctrl Pts',(-0.22139514771026,0.00185666417523725,
0.00864445166450529));
#45390=CARTESIAN_POINT('Ctrl Pts',(-0.22139511152028,0.00178727927747294,
0.00873084239674152));
#45391=CARTESIAN_POINT('Ctrl Pts',(-0.221288280479528,0.00177389461696801,
0.00870594947214869));
#45392=CARTESIAN_POINT('Ctrl Pts',(-0.221544108200661,0.00133248767187958,
0.00815434837593592));
#45393=CARTESIAN_POINT('Ctrl Pts',(-0.221544269965813,0.00125651031431327,
0.00823458355479384));
#45394=CARTESIAN_POINT('Ctrl Pts',(-0.221436545998082,0.00124802503912297,
0.00821143217143996));
#45395=CARTESIAN_POINT('Ctrl Pts',(-0.221311628769438,0.00171848642413581,
0.00862619824224493));
#45396=CARTESIAN_POINT('Ctrl Pts',(-0.221335049690428,0.00174110173044518,
0.00864534820546848));
#45397=CARTESIAN_POINT('Ctrl Pts',(-0.221348766211921,0.00175797442052312,
0.00864927269533899));
#45398=CARTESIAN_POINT('Ctrl Pts',(-0.221361583393583,0.0017796554992303,
0.00865009179604268));
#45399=CARTESIAN_POINT('Ctrl Pts',(-0.221362743032725,0.00178161710266088,
0.00865016590447483));
#45400=CARTESIAN_POINT('Ctrl Pts',(-0.221363895896245,0.00178363088934365,
0.00865018385643546));
#45401=CARTESIAN_POINT('Ctrl Pts',(-0.221365048880398,0.00178570794336532,
0.00865013521475478));
#45402=CARTESIAN_POINT('Ctrl Pts',(-0.221378945476116,0.00181074209492944,
0.0086495489501735));
#45403=CARTESIAN_POINT('Ctrl Pts',(-0.221392953879523,0.00184293580361415,
0.00863455712906129));
#45404=CARTESIAN_POINT('Ctrl Pts',(-0.22139331361059,0.0018597065642107,
0.00861406379669157));
#45405=CARTESIAN_POINT('Ctrl Pts',(-0.221093378117463,0.00749708146235502,
0.0106049495976336));
#45406=CARTESIAN_POINT('Ctrl Pts',(-0.221093205142074,0.00749707938042166,
0.0106113459163336));
#45407=CARTESIAN_POINT('Ctrl Pts',(-0.221092416367657,0.00749707747540696,
0.010617710754281));
#45408=CARTESIAN_POINT('Ctrl Pts',(-0.221089506457863,0.00749707392137382,
0.0106307519256261));
#45409=CARTESIAN_POINT('Ctrl Pts',(-0.221087282431476,0.00749707231971561,
0.0106373694403386));
#45410=CARTESIAN_POINT('Ctrl Pts',(-0.221079032172649,0.00749706854074414,
0.0106554173015107));
#45411=CARTESIAN_POINT('Ctrl Pts',(-0.221071459539386,0.00749706706830675,
0.0106659849606413));
#45412=CARTESIAN_POINT('Ctrl Pts',(-0.221052722966754,0.00749706622792382,
0.0106836774393237));
#45413=CARTESIAN_POINT('Ctrl Pts',(-0.221041732788639,0.00749706687881053,
0.0106906356764216));
#45414=CARTESIAN_POINT('Ctrl Pts',(-0.221016370204857,0.00749707029332032,
0.010700554781231));
#45415=CARTESIAN_POINT('Ctrl Pts',(-0.221003692357774,0.00749708761297438,
0.0107022186490283));
#45416=CARTESIAN_POINT('Ctrl Pts',(-0.220992859660385,0.00749707123864509,
0.0107022443220174));
#45417=CARTESIAN_POINT('Ctrl Pts',(-0.220992434802756,0.00749707047723624,
0.0107022424122139));
#45418=CARTESIAN_POINT('Ctrl Pts',(-0.220991842577576,0.00749706643585074,
0.0107022363855843));
#45419=CARTESIAN_POINT('Ctrl Pts',(-0.2209915935623,0.00749706431881418,
0.0107022330643159));
#45420=CARTESIAN_POINT('Ctrl Pts',(-0.220991241417974,0.00749705445135643,
0.010702227262308));
#45421=CARTESIAN_POINT('Ctrl Pts',(-0.220990864889388,0.00749696165836036,
0.0107022195991458));
#45422=CARTESIAN_POINT('Ctrl Pts',(-0.221039491002263,0.00685968436868825,
0.0106798040221069));
#45423=CARTESIAN_POINT('Ctrl Pts',(-0.2211492365355,0.00686784362818015,
0.0106927234678917));
#45424=CARTESIAN_POINT('Ctrl Pts',(-0.221150162182504,0.00687562622327931,
0.0105822167718128));
#45425=CARTESIAN_POINT('Ctrl Pts',(-0.220922250319514,0.0080967120552641,
0.0107670355630445));
#45426=CARTESIAN_POINT('Ctrl Pts',(-0.221031721906841,0.00810919801080945,
0.0107785744055876));
#45427=CARTESIAN_POINT('Ctrl Pts',(-0.221032674276105,0.00810155969385244,
0.0106669825539216));
#45428=CARTESIAN_POINT('Ctrl Pts',(-0.220788218290202,0.00991813533979832,
0.0105192170441643));
#45429=CARTESIAN_POINT('Ctrl Pts',(-0.220898965091819,0.00992213316049332,
0.0105286086746672));
#45430=CARTESIAN_POINT('Ctrl Pts',(-0.220899825135949,0.00989272597187494,
0.0104200247978636));
#45431=CARTESIAN_POINT('Ctrl Pts',(-0.220993366234941,0.0122349103118159,
0.00944376699900189));
#45432=CARTESIAN_POINT('Ctrl Pts',(-0.221102422349815,0.0122250398274275,
0.00946224918086765));
#45433=CARTESIAN_POINT('Ctrl Pts',(-0.221102779185047,0.0121671951175703,
0.00936681518662684));
#45434=CARTESIAN_POINT('Ctrl Pts',(-0.221293686408273,0.0132125520200273,
0.00871678626296279));
#45435=CARTESIAN_POINT('Ctrl Pts',(-0.221400740809213,0.0131990319642865,
0.00874220143421774));
#45436=CARTESIAN_POINT('Ctrl Pts',(-0.221400781399722,0.0131295984931284,
0.00865540763741799));
#45437=CARTESIAN_POINT('Ctrl Pts',(-0.221443349927793,0.0137382361695334,
0.00822458347293278));
#45438=CARTESIAN_POINT('Ctrl Pts',(-0.221551332642022,0.0137297760742548,
0.0082481846551935));
#45439=CARTESIAN_POINT('Ctrl Pts',(-0.221551177097651,0.013653735905962,
0.00816753405499274));
#45440=CARTESIAN_POINT('Ctrl Pts',(-0.221398994600239,0.0131267929917585,
0.00862507463528867));
#45441=CARTESIAN_POINT('Ctrl Pts',(-0.221398891939579,0.0131316229516505,
0.00863100166036205));
#45442=CARTESIAN_POINT('Ctrl Pts',(-0.221398088470179,0.0131370777877344,
0.00863629298538617));
#45443=CARTESIAN_POINT('Ctrl Pts',(-0.22139502985258,0.0131495873621591,
0.00864593890691218));
#45444=CARTESIAN_POINT('Ctrl Pts',(-0.221392666461445,0.0131566114257431,
0.00865003283544232));
#45445=CARTESIAN_POINT('Ctrl Pts',(-0.221384721392673,0.0131760488259407,
0.00865847676490165));
#45446=CARTESIAN_POINT('Ctrl Pts',(-0.221378157530941,0.0131886255371438,
0.00866101697794908));
#45447=CARTESIAN_POINT('Ctrl Pts',(-0.221363533028657,0.0132126585780711,
0.00866158988192774));
#45448=CARTESIAN_POINT('Ctrl Pts',(-0.221355517305592,0.0132241274980054,
0.00865973056392319));
#45449=CARTESIAN_POINT('Ctrl Pts',(-0.221335852230188,0.0132492406714318,
0.00865134678022098));
#45450=CARTESIAN_POINT('Ctrl Pts',(-0.221326472378544,0.0132589786142125,
0.0086444552679184));
#45451=CARTESIAN_POINT('Ctrl Pts',(-0.221321893750534,0.0132634897311423,
0.0086410835650841));
#45452=CARTESIAN_POINT('Ctrl Pts',(-0.221319816394641,0.0132656643245537,
0.00863943976353927));
#45453=CARTESIAN_POINT('Ctrl Pts',(-0.221317746469157,0.0132677508018423,
0.00863769213611541));
#45454=CARTESIAN_POINT('Ctrl Pts',(-0.221317509604566,0.0132679808638495,
0.0086374981209002));
#45455=CARTESIAN_POINT('Origin',(-0.222557040593836,0.00178348666403939,
0.0085734100013149));
#45456=CARTESIAN_POINT('Ctrl Pts',(-0.222392821469384,0.00185976161919177,
0.00863469597942385));
#45457=CARTESIAN_POINT('Ctrl Pts',(-0.222392851665228,0.00185471841683084,
0.00864067695413965));
#45458=CARTESIAN_POINT('Ctrl Pts',(-0.2223940171567,0.00184908923740676,
0.00864595328592874));
#45459=CARTESIAN_POINT('Ctrl Pts',(-0.222398791623032,0.00183568068451202,
0.00865603804918068));
#45460=CARTESIAN_POINT('Ctrl Pts',(-0.222402792716745,0.001827955969436,
0.00866029353481253));
#45461=CARTESIAN_POINT('Ctrl Pts',(-0.222415271837931,0.00180816896025231,
0.00866840805978246));
#45462=CARTESIAN_POINT('Ctrl Pts',(-0.22242559622064,0.00179522568857694,
0.00867101548583902));
#45463=CARTESIAN_POINT('Ctrl Pts',(-0.222448811324784,0.00177087556880312,
0.00867117726491881));
#45464=CARTESIAN_POINT('Ctrl Pts',(-0.222460500420385,0.0017601953052336,
0.00866936374343137));
#45465=CARTESIAN_POINT('Ctrl Pts',(-0.222488934943182,0.0017368874233403,
0.00866177871632728));
#45466=CARTESIAN_POINT('Ctrl Pts',(-0.222502563560879,0.00172781843157747,
0.00865561058774906));
#45467=CARTESIAN_POINT('Ctrl Pts',(-0.222508821481566,0.00172382527717114,
0.00865277338878037));
#45468=CARTESIAN_POINT('Ctrl Pts',(-0.222511943488237,0.00172173990045585,
0.00865127231333268));
#45469=CARTESIAN_POINT('Ctrl Pts',(-0.222515286760213,0.00171959773431523,
0.00864956320157879));
#45470=CARTESIAN_POINT('Origin',(-0.221237455096366,0.0132044515326223,
0.00855877605601754));
#45471=CARTESIAN_POINT('Ctrl Pts',(-0.22239855467333,0.013126959871322,
0.00864556967094923));
#45472=CARTESIAN_POINT('Ctrl Pts',(-0.222398693734901,0.0131508497456262,
0.00867409420882899));
#45473=CARTESIAN_POINT('Ctrl Pts',(-0.222421879764434,0.0131819804421261,
0.00868215664988287));
#45474=CARTESIAN_POINT('Ctrl Pts',(-0.22244667526595,0.0132098804246437,
0.00867921869573823));
#45475=CARTESIAN_POINT('Ctrl Pts',(-0.222467868815537,0.0132337274786178,
0.00867670752746002));
#45476=CARTESIAN_POINT('Ctrl Pts',(-0.222493016945457,0.0132565629439438,
0.00866887354856461));
#45477=CARTESIAN_POINT('Ctrl Pts',(-0.222521349609231,0.0132671009264466,
0.00866069085884597));
#45478=CARTESIAN_POINT('Ctrl Pts',(-0.222249879452339,0.00812452848998182,
0.010708612169071));
#45479=CARTESIAN_POINT('Ctrl Pts',(-0.222147518448448,0.00813291623381584,
0.0107075640119653));
#45480=CARTESIAN_POINT('Ctrl Pts',(-0.222150626988561,0.00812566746543201,
0.0106051733469215));
#45481=CARTESIAN_POINT('Ctrl Pts',(-0.222133026314569,0.00688653200057354,
0.0107938566452843));
#45482=CARTESIAN_POINT('Ctrl Pts',(-0.222030952328141,0.00689749083265872,
0.0107941909562852));
#45483=CARTESIAN_POINT('Ctrl Pts',(-0.222034092623134,0.0069045120619468,
0.0106907926699249));
#45484=CARTESIAN_POINT('Ctrl Pts',(-0.22199453534553,0.00506519692361534,
0.0105419098967548));
#45485=CARTESIAN_POINT('Ctrl Pts',(-0.221891198357135,0.00506624553307757,
0.0105441068399897));
#45486=CARTESIAN_POINT('Ctrl Pts',(-0.221894228499143,0.00509371640154661,
0.0104434958915309));
#45487=CARTESIAN_POINT('Ctrl Pts',(-0.222202898757155,0.00275215309907751,
0.00946096055553374));
#45488=CARTESIAN_POINT('Ctrl Pts',(-0.222101363550626,0.00273655987836659,
0.00945278298769915));
#45489=CARTESIAN_POINT('Ctrl Pts',(-0.222103946704122,0.0027907538603155,
0.00936468088853639));
#45490=CARTESIAN_POINT('Ctrl Pts',(-0.222502984837095,0.0017766303999828,
0.00873137796397993));
#45491=CARTESIAN_POINT('Ctrl Pts',(-0.222403127086071,0.00175761006895396,
0.00871654143776575));
#45492=CARTESIAN_POINT('Ctrl Pts',(-0.222405448098085,0.00182264005112638,
0.00863665510434452));
#45493=CARTESIAN_POINT('Ctrl Pts',(-0.222649516124785,0.00125128420842517,
0.00823635580503606));
#45494=CARTESIAN_POINT('Ctrl Pts',(-0.222548875458837,0.00123596872506605,
0.00822244965460723));
#45495=CARTESIAN_POINT('Ctrl Pts',(-0.222550999194757,0.00130702015936901,
0.00814827332314741));
#45496=CARTESIAN_POINT('Ctrl Pts',(-0.222093144978732,0.00749648852186606,
0.0106271018238363));
#45497=CARTESIAN_POINT('Ctrl Pts',(-0.222092997107659,0.00749648591386968,
0.0106336443875128));
#45498=CARTESIAN_POINT('Ctrl Pts',(-0.222093494220433,0.00749648312939007,
0.0106401852870836));
#45499=CARTESIAN_POINT('Ctrl Pts',(-0.222095835536279,0.00749647710304743,
0.010653484677253));
#45500=CARTESIAN_POINT('Ctrl Pts',(-0.222097756689006,0.00749647386023141,
0.0106601933989456));
#45501=CARTESIAN_POINT('Ctrl Pts',(-0.222105178870428,0.00749646437817162,
0.0106785939630422));
#45502=CARTESIAN_POINT('Ctrl Pts',(-0.222112264289149,0.00749645802673394,
0.0106894939842665));
#45503=CARTESIAN_POINT('Ctrl Pts',(-0.222130179059406,0.00749644565024443,
0.0107080180341044));
#45504=CARTESIAN_POINT('Ctrl Pts',(-0.222140842483058,0.00749643973517114,
0.0107154676427388));
#45505=CARTESIAN_POINT('Ctrl Pts',(-0.222172400273181,0.00749642562068748,
0.0107294912223153));
#45506=CARTESIAN_POINT('Ctrl Pts',(-0.222189155075009,0.00749640861672746,
0.0107292902671688));
#45507=CARTESIAN_POINT('Ctrl Pts',(-0.222190773040506,0.00749643501029294,
0.0107293377107985));
#45508=CARTESIAN_POINT('Ctrl Pts',(-0.222190885265316,0.00749642040198078,
0.0107293409891968));
#45509=CARTESIAN_POINT('Ctrl Pts',(-0.222191215574431,0.00749642030964181,
0.0107293485047956));
#45510=CARTESIAN_POINT('Ctrl Pts',(-0.22215039542817,0.00686823386554683,
0.0106047411261954));
#45511=CARTESIAN_POINT('Ctrl Pts',(-0.222147291245924,0.00686090299773189,
0.0107073006204878));
#45512=CARTESIAN_POINT('Ctrl Pts',(-0.222249829666163,0.00686926077332403,
0.0107081718176659));
#45513=CARTESIAN_POINT('Ctrl Pts',(-0.222033882153739,0.00808751688966911,
0.0106910818583913));
#45514=CARTESIAN_POINT('Ctrl Pts',(-0.222030746230797,0.00809445663738906,
0.0107946576004359));
#45515=CARTESIAN_POINT('Ctrl Pts',(-0.222133001056444,0.00810538495115661,
0.0107941436327104));
#45516=CARTESIAN_POINT('Ctrl Pts',(-0.22189809572205,0.00989579664481618,
0.0104460000225152));
#45517=CARTESIAN_POINT('Ctrl Pts',(-0.221895068156802,0.00992318971953597,
0.0105468118004952));
#45518=CARTESIAN_POINT('Ctrl Pts',(-0.221998571699939,0.00992407913617585,
0.0105444854422989));
#45519=CARTESIAN_POINT('Ctrl Pts',(-0.222106552859369,0.0121968557973979,
0.00937209506599623));
#45520=CARTESIAN_POINT('Ctrl Pts',(-0.222103972397347,0.0122510011058486,
0.0094604296734285));
#45521=CARTESIAN_POINT('Ctrl Pts',(-0.222205682870112,0.012235266783474,
0.00946843760091433));
#45522=CARTESIAN_POINT('Ctrl Pts',(-0.222411459865652,0.0131644409687035,
0.00864713334535926));
#45523=CARTESIAN_POINT('Ctrl Pts',(-0.222409139563845,0.0132294340807041,
0.0087272747710823));
#45524=CARTESIAN_POINT('Ctrl Pts',(-0.222509083672908,0.0132099447880335,
0.00874218337616711));
#45525=CARTESIAN_POINT('Ctrl Pts',(-0.222558486991795,0.0136798443822662,
0.00816098211452363));
#45526=CARTESIAN_POINT('Ctrl Pts',(-0.222556362475417,0.0137508603207363,
0.00823543380177068));
#45527=CARTESIAN_POINT('Ctrl Pts',(-0.222657130762485,0.013735231609234,
0.00824934739737568));
#45528=CARTESIAN_POINT('Ctrl Pts',(-0.219148404100077,0.00808836362885957,
0.0105397408946697));
#45529=CARTESIAN_POINT('Ctrl Pts',(-0.219147286260384,0.00809560494432423,
0.0106488954886024));
#45530=CARTESIAN_POINT('Ctrl Pts',(-0.219038810118551,0.00810395989687771,
0.0106373208135017));
#45531=CARTESIAN_POINT('Ctrl Pts',(-0.219036260639061,0.00692355290527283,
0.0106150424470077));
#45532=CARTESIAN_POINT('Ctrl Pts',(-0.219035119802892,0.00691634871689329,
0.0107251414266647));
#45533=CARTESIAN_POINT('Ctrl Pts',(-0.218926885305538,0.00692862928927927,
0.0107149222445564));
#45534=CARTESIAN_POINT('Ctrl Pts',(-0.218905493367159,0.00522543643497804,
0.0103925587148312));
#45535=CARTESIAN_POINT('Ctrl Pts',(-0.218904431859709,0.00519797604222467,
0.010500029300181));
#45536=CARTESIAN_POINT('Ctrl Pts',(-0.218795072781458,0.00520197616056926,
0.0104916549790139));
#45537=CARTESIAN_POINT('Ctrl Pts',(-0.219069945774343,0.00304060262385979,
0.00944022647325578));
#45538=CARTESIAN_POINT('Ctrl Pts',(-0.219069332996938,0.00298616501663537,
0.00953594714440858));
#45539=CARTESIAN_POINT('Ctrl Pts',(-0.218961240632144,0.00297739205618275,
0.00951996720256591));
#45540=CARTESIAN_POINT('Ctrl Pts',(-0.219322800899811,0.00209990025679052,
0.00879058344321244));
#45541=CARTESIAN_POINT('Ctrl Pts',(-0.219322481672864,0.00203429555214399,
0.00887852267246854));
#45542=CARTESIAN_POINT('Ctrl Pts',(-0.219216100504328,0.00202134997278713,
0.00885622517805967));
#45543=CARTESIAN_POINT('Ctrl Pts',(-0.219451770062291,0.00158485407297901,
0.00834673001569572));
#45544=CARTESIAN_POINT('Ctrl Pts',(-0.219451626127622,0.00151291782239926,
0.00842920614775955));
#45545=CARTESIAN_POINT('Ctrl Pts',(-0.219344450923872,0.00150470339121809,
0.0084085948337711));
#45546=CARTESIAN_POINT('Ctrl Pts',(-0.219329643945211,0.00206973899609492,
0.00873934399098496));
#45547=CARTESIAN_POINT('Ctrl Pts',(-0.21932954767613,0.00206564252185154,
0.00874469986786621));
#45548=CARTESIAN_POINT('Ctrl Pts',(-0.219328831198008,0.00206126786037065,
0.00874979857642302));
#45549=CARTESIAN_POINT('Ctrl Pts',(-0.219326098049909,0.00205177977988729,
0.00875966351192551));
#45550=CARTESIAN_POINT('Ctrl Pts',(-0.219324006068103,0.00204667681545294,
0.00876433959539986));
#45551=CARTESIAN_POINT('Ctrl Pts',(-0.219316297145377,0.00203190722576044,
0.00877620076329959));
#45552=CARTESIAN_POINT('Ctrl Pts',(-0.219309292282347,0.00202216812127946,
0.00878207855087985));
#45553=CARTESIAN_POINT('Ctrl Pts',(-0.2192921175356,0.00200325932998677,
0.00878988793020369));
#45554=CARTESIAN_POINT('Ctrl Pts',(-0.219282057436856,0.00199427474463678,
0.00879168528662207));
#45555=CARTESIAN_POINT('Ctrl Pts',(-0.219259249035481,0.00197748116797533,
0.00879101814240679));
#45556=CARTESIAN_POINT('Ctrl Pts',(-0.219249069113353,0.00197189892749821,
0.00878821256821367));
#45557=CARTESIAN_POINT('Ctrl Pts',(-0.219242270579201,0.00196834740913877,
0.00878599194012615));
#45558=CARTESIAN_POINT('Ctrl Pts',(-0.219240172952592,0.00196731085858162,
0.00878530517930024));
#45559=CARTESIAN_POINT('Ctrl Pts',(-0.219238073822237,0.00196633000923113,
0.00878455699842097));
#45560=CARTESIAN_POINT('Ctrl Pts',(-0.219237124510089,0.00196588311043685,
0.0087841963906634));
#45561=CARTESIAN_POINT('Ctrl Pts',(-0.219093939821662,0.00749806050132961,
0.010559781147994));
#45562=CARTESIAN_POINT('Ctrl Pts',(-0.219093765728207,0.00749805919151256,
0.0105661708589535));
#45563=CARTESIAN_POINT('Ctrl Pts',(-0.21909297706098,0.00749805803365454,
0.0105725290512502));
#45564=CARTESIAN_POINT('Ctrl Pts',(-0.219090068280447,0.00749805597621986,
0.0105855639856694));
#45565=CARTESIAN_POINT('Ctrl Pts',(-0.219087843995007,0.00749805511454117,
0.0105921816327154));
#45566=CARTESIAN_POINT('Ctrl Pts',(-0.21907959284429,0.00749805332442967,
0.0106102297141528));
#45567=CARTESIAN_POINT('Ctrl Pts',(-0.219072019489481,0.00749805296861923,
0.0106207972909321));
#45568=CARTESIAN_POINT('Ctrl Pts',(-0.2190532813129,0.00749805415624955,
0.0106384896244247));
#45569=CARTESIAN_POINT('Ctrl Pts',(-0.219042290189228,0.00749805556350332,
0.0106454477078487));
#45570=CARTESIAN_POINT('Ctrl Pts',(-0.219019950092807,0.00749806122118377,
0.0106541837873464));
#45571=CARTESIAN_POINT('Ctrl Pts',(-0.219009039840112,0.00749804440964752,
0.0106564778252645));
#45572=CARTESIAN_POINT('Ctrl Pts',(-0.218995817113753,0.00749809073883346,
0.0106570547372539));
#45573=CARTESIAN_POINT('Ctrl Pts',(-0.218993530063054,0.00749806237148593,
0.0106570788650823));
#45574=CARTESIAN_POINT('Ctrl Pts',(-0.218991338855106,0.00749806287369093,
0.0106570293466482));
#45575=CARTESIAN_POINT('Ctrl Pts',(-0.219458972439161,0.0134081066407698,
0.00835293645932442));
#45576=CARTESIAN_POINT('Ctrl Pts',(-0.219458332634967,0.0134799305966825,
0.00843531702472389));
#45577=CARTESIAN_POINT('Ctrl Pts',(-0.219351364553155,0.0134880627422249,
0.00841432815581591));
#45578=CARTESIAN_POINT('Ctrl Pts',(-0.219330919335611,0.0129021834400454,
0.00878997306616953));
#45579=CARTESIAN_POINT('Ctrl Pts',(-0.219330111991264,0.0129678170383922,
0.00887771930160673));
#45580=CARTESIAN_POINT('Ctrl Pts',(-0.219223960476356,0.0129807630116758,
0.00885498650689457));
#45581=CARTESIAN_POINT('Ctrl Pts',(-0.21907217366948,0.0119507491293741,
0.00944613164313236));
#45582=CARTESIAN_POINT('Ctrl Pts',(-0.219071061787161,0.0120050759109758,
0.00954176136696198));
#45583=CARTESIAN_POINT('Ctrl Pts',(-0.218963148115845,0.0120137476734168,
0.00952545967271347));
#45584=CARTESIAN_POINT('Ctrl Pts',(-0.218908878443448,0.00977018641413983,
0.0103930111689677));
#45585=CARTESIAN_POINT('Ctrl Pts',(-0.218907313830057,0.00979754952644692,
0.010500350610888));
#45586=CARTESIAN_POINT('Ctrl Pts',(-0.218798131116708,0.00979356929641045,
0.0104915911911937));
#45587=CARTESIAN_POINT('Ctrl Pts',(-0.21903560702607,0.0080761058161286,
0.0106160018814049));
#45588=CARTESIAN_POINT('Ctrl Pts',(-0.219033968343184,0.00808324228078203,
0.0107259654053647));
#45589=CARTESIAN_POINT('Ctrl Pts',(-0.218925901646514,0.00807099086232866,
0.0107153948463322));
#45590=CARTESIAN_POINT('Ctrl Pts',(-0.219148501134292,0.00690552738431865,
0.0105398630894422));
#45591=CARTESIAN_POINT('Ctrl Pts',(-0.219146884619599,0.00689818019381566,
0.0106488663910279));
#45592=CARTESIAN_POINT('Ctrl Pts',(-0.219038578450512,0.00688992144780411,
0.0106369402406613));
#45593=CARTESIAN_POINT('Ctrl Pts',(-0.219334447815789,0.0129187822150905,
0.00874810840271639));
#45594=CARTESIAN_POINT('Ctrl Pts',(-0.219334349313406,0.0129229875332314,
0.00875361950638557));
#45595=CARTESIAN_POINT('Ctrl Pts',(-0.219333611885487,0.0129275458909777,
0.00875880523042341));
#45596=CARTESIAN_POINT('Ctrl Pts',(-0.219330800131034,0.0129375763567918,
0.00876872890637208));
#45597=CARTESIAN_POINT('Ctrl Pts',(-0.219328645180264,0.0129430363384887,
0.00877334976205868));
#45598=CARTESIAN_POINT('Ctrl Pts',(-0.219320864830539,0.0129587194547766,
0.00878463247984444));
#45599=CARTESIAN_POINT('Ctrl Pts',(-0.219313950560981,0.0129690726824846,
0.00878985601767334));
#45600=CARTESIAN_POINT('Ctrl Pts',(-0.219297070769606,0.012989588910634,
0.00879623291603491));
#45601=CARTESIAN_POINT('Ctrl Pts',(-0.219287139859611,0.0129995534686749,
0.0087971642880923));
#45602=CARTESIAN_POINT('Ctrl Pts',(-0.219268011982728,0.0130157461221668,
0.00879493805234113));
#45603=CARTESIAN_POINT('Ctrl Pts',(-0.219259084995648,0.0130222780130516,
0.00879255390199529));
#45604=CARTESIAN_POINT('Ctrl Pts',(-0.219248202110861,0.0130291638450967,
0.00878810745217938));
#45605=CARTESIAN_POINT('Ctrl Pts',(-0.219246191884804,0.013030361992373,
0.00878724563927881));
#45606=CARTESIAN_POINT('Ctrl Pts',(-0.219244237320854,0.0130315050188546,
0.00878633307433836));
#45607=CARTESIAN_POINT('Ctrl Pts',(-0.220652621774988,0.00171860875021885,
0.00861403983191908));
#45608=CARTESIAN_POINT('Ctrl Pts',(-0.22065070898904,0.00179715124586783,
0.00868074893703625));
#45609=CARTESIAN_POINT('Ctrl Pts',(-0.220652186979373,0.00186150990883231,
0.00860050117613837));
#45610=CARTESIAN_POINT('Ctrl Pts',(-0.22038156151548,0.00172153788266806,
0.00861139809863215));
#45611=CARTESIAN_POINT('Ctrl Pts',(-0.220379331631024,0.0017994467145094,
0.0086774643645163));
#45612=CARTESIAN_POINT('Ctrl Pts',(-0.220380902934705,0.00186376460487148,
0.00859721360678668));
#45613=CARTESIAN_POINT('Ctrl Pts',(-0.219997085557986,0.00169755239672656,
0.00858453373495456));
#45614=CARTESIAN_POINT('Ctrl Pts',(-0.219993559109339,0.00177816495585469,
0.00865325916554496));
#45615=CARTESIAN_POINT('Ctrl Pts',(-0.219994933861779,0.00184264803256065,
0.00857302038288794));
#45616=CARTESIAN_POINT('Ctrl Pts',(-0.219457398216233,0.0018050393200918,
0.00866289593480801));
#45617=CARTESIAN_POINT('Ctrl Pts',(-0.21950512140762,0.00187792237709183,
0.00872395721311587));
#45618=CARTESIAN_POINT('Ctrl Pts',(-0.219505746247963,0.00194139912405486,
0.00864325897028411));
#45619=CARTESIAN_POINT('Ctrl Pts',(-0.219252194129174,0.00195596694160954,
0.00877794624534211));
#45620=CARTESIAN_POINT('Ctrl Pts',(-0.219324471820114,0.00201229795546534,
0.00882429986098872));
#45621=CARTESIAN_POINT('Ctrl Pts',(-0.219325359194532,0.00207418376706999,
0.00874287956348477));
#45622=CARTESIAN_POINT('Ctrl Pts',(-0.219129805649029,0.00203517720513716,
0.0088345274762402));
#45623=CARTESIAN_POINT('Ctrl Pts',(-0.219189125076113,0.00210065585944006,
0.00888677249466793));
#45624=CARTESIAN_POINT('Ctrl Pts',(-0.219190162076039,0.00216143160586825,
0.00880428766836637));
#45625=CARTESIAN_POINT('Ctrl Pts',(-0.220393521722421,0.00185901092063506,
0.00859658671256956));
#45626=CARTESIAN_POINT('Ctrl Pts',(-0.220393545683691,0.00185536086192936,
0.00860093418665886));
#45627=CARTESIAN_POINT('Ctrl Pts',(-0.220394166592933,0.00185139129769321,
0.00860493128106815));
#45628=CARTESIAN_POINT('Ctrl Pts',(-0.220397494433511,0.00183939323794458,
0.00861522365214686));
#45629=CARTESIAN_POINT('Ctrl Pts',(-0.22040142365534,0.00183106621657628,
0.00862036967205643));
#45630=CARTESIAN_POINT('Ctrl Pts',(-0.220413421988607,0.00181115837561913,
0.00862944761777806));
#45631=CARTESIAN_POINT('Ctrl Pts',(-0.220422944779313,0.00179879060235556,
0.00863252660109762));
#45632=CARTESIAN_POINT('Ctrl Pts',(-0.220446693838697,0.00177307264120848,
0.00863403325035388));
#45633=CARTESIAN_POINT('Ctrl Pts',(-0.220460216415066,0.00176067973120046,
0.00863218189800322));
#45634=CARTESIAN_POINT('Ctrl Pts',(-0.220480884415075,0.00174394626121798,
0.00862668378645218));
#45635=CARTESIAN_POINT('Ctrl Pts',(-0.220487970824601,0.00173858167731576,
0.00862434869605683));
#45636=CARTESIAN_POINT('Ctrl Pts',(-0.220498562066858,0.0017310627344125,
0.00862024819021514));
#45637=CARTESIAN_POINT('Ctrl Pts',(-0.220502054976112,0.00172866352663628,
0.00861879861371333));
#45638=CARTESIAN_POINT('Ctrl Pts',(-0.220507287796832,0.00172517941353552,
0.00861647938973381));
#45639=CARTESIAN_POINT('Ctrl Pts',(-0.220509010984543,0.00172405157047886,
0.00861569195890217));
#45640=CARTESIAN_POINT('Ctrl Pts',(-0.220511587454697,0.00172237856914534,
0.00861447017639169));
#45641=CARTESIAN_POINT('Ctrl Pts',(-0.220512494461661,0.00172179370048413,
0.00861403209497913));
#45642=CARTESIAN_POINT('Ctrl Pts',(-0.22051388248347,0.00172087463848556,
0.00861332861068179));
#45643=CARTESIAN_POINT('Ctrl Pts',(-0.220514289505427,0.00172059226538401,
0.00861310745220749));
#45644=CARTESIAN_POINT('Ctrl Pts',(-0.220514747001341,0.00172022865110598,
0.00861282031082267));
#45645=CARTESIAN_POINT('Ctrl Pts',(-0.220514873167071,0.00172010829936638,
0.00861272412883551));
#45646=CARTESIAN_POINT('Ctrl Pts',(-0.220515057375285,0.00171980899790886,
0.00861248132013813));
#45647=CARTESIAN_POINT('Ctrl Pts',(-0.220504895339338,0.0131091095836261,
0.00862176289898313));
#45648=CARTESIAN_POINT('Ctrl Pts',(-0.220503204519676,0.013172278658427,
0.00870065757297661));
#45649=CARTESIAN_POINT('Ctrl Pts',(-0.220524686999525,0.0132489243928214,
0.00863835592833102));
#45650=CARTESIAN_POINT('Ctrl Pts',(-0.220393730780806,0.0131269580310319,
0.00860539375055619));
#45651=CARTESIAN_POINT('Ctrl Pts',(-0.220392045709976,0.0131903179698247,
0.0086841360040918));
#45652=CARTESIAN_POINT('Ctrl Pts',(-0.22041353202268,0.0132668117899861,
0.00862164844129692));
#45653=CARTESIAN_POINT('Ctrl Pts',(-0.220184614434698,0.0131663208471479,
0.00856955272821915));
#45654=CARTESIAN_POINT('Ctrl Pts',(-0.220183091286059,0.0132300952247244,
0.00864807418559056));
#45655=CARTESIAN_POINT('Ctrl Pts',(-0.220190375822233,0.0133093870456292,
0.00858224595417015));
#45656=CARTESIAN_POINT('Ctrl Pts',(-0.219784302265126,0.0131135141202054,
0.00860522420992131));
#45657=CARTESIAN_POINT('Ctrl Pts',(-0.219783539999466,0.0131767153162485,
0.00868397549414707));
#45658=CARTESIAN_POINT('Ctrl Pts',(-0.219739129146227,0.0132501816669398,
0.00862323219516294));
#45659=CARTESIAN_POINT('Ctrl Pts',(-0.219485674564641,0.0129837568423567,
0.00870181479506232));
#45660=CARTESIAN_POINT('Ctrl Pts',(-0.219484575843822,0.0130454250762007,
0.0087816185864055));
#45661=CARTESIAN_POINT('Ctrl Pts',(-0.219437547728755,0.013115180181397,
0.00872598545329776));
#45662=CARTESIAN_POINT('Ctrl Pts',(-0.219285266042446,0.0128973209402166,
0.00876279522307528));
#45663=CARTESIAN_POINT('Ctrl Pts',(-0.219284139925531,0.0129580035698831,
0.00884334030755273));
#45664=CARTESIAN_POINT('Ctrl Pts',(-0.21923709929106,0.0130284151484448,
0.00878856304375625));
#45665=CARTESIAN_POINT('Ctrl Pts',(-0.220398946890659,0.0131276359028523,
0.00860743040991009));
#45666=CARTESIAN_POINT('Ctrl Pts',(-0.220398971642014,0.0131321314775003,
0.00861284084588095));
#45667=CARTESIAN_POINT('Ctrl Pts',(-0.220399881495722,0.013137006554187,
0.00861781950952909));
#45668=CARTESIAN_POINT('Ctrl Pts',(-0.220403652945788,0.0131482971438847,
0.00862767263867194));
#45669=CARTESIAN_POINT('Ctrl Pts',(-0.220406804708496,0.0131546746445743,
0.00863220881639067));
#45670=CARTESIAN_POINT('Ctrl Pts',(-0.220417285354963,0.0131715709114628,
0.00864208462491169));
#45671=CARTESIAN_POINT('Ctrl Pts',(-0.220426267100991,0.0131825846100448,
0.0086463614567408));
#45672=CARTESIAN_POINT('Ctrl Pts',(-0.220451830128197,0.0132080184642301,
0.00865141595330123));
#45673=CARTESIAN_POINT('Ctrl Pts',(-0.220469419124149,0.0132219431230173,
0.00865059776196831));
#45674=CARTESIAN_POINT('Ctrl Pts',(-0.22049334815256,0.0132371769667726,
0.00864495572013383));
#45675=CARTESIAN_POINT('Ctrl Pts',(-0.220498115179498,0.0132400462236785,
0.00864362986672573));
#45676=CARTESIAN_POINT('Ctrl Pts',(-0.220505238671295,0.0132441039903126,
0.00864135545795626));
#45677=CARTESIAN_POINT('Ctrl Pts',(-0.220507582366072,0.0132454010942176,
0.00864056065067561));
#45678=CARTESIAN_POINT('Ctrl Pts',(-0.220511137605847,0.0132473236276702,
0.00863927732404243));
#45679=CARTESIAN_POINT('Ctrl Pts',(-0.220512314305617,0.013247950397367,
0.00863883918371931));
#45680=CARTESIAN_POINT('Ctrl Pts',(-0.220513986335453,0.0132488496923406,
0.00863818618337553));
#45681=CARTESIAN_POINT('Ctrl Pts',(-0.220514656898247,0.0132492117024941,
0.00863791682953718));
#45682=CARTESIAN_POINT('Ctrl Pts',(-0.220515400278411,0.0132496510473206,
0.00863758226858773));
#45683=CARTESIAN_POINT('Ctrl Pts',(-0.220515602204728,0.0132497815996683,
0.00863748127580821));
#45684=CARTESIAN_POINT('Ctrl Pts',(-0.220515865363209,0.0132499845085129,
0.00863732249765459));
#45685=CARTESIAN_POINT('Ctrl Pts',(-0.220515947525014,0.0132500624648397,
0.00863726079027726));
#45686=CARTESIAN_POINT('Ctrl Pts',(-0.220516099934179,0.0132503125103766,
0.00863705970261241));
#45687=CARTESIAN_POINT('Ctrl Pts',(-0.2202504135532,0.00812534913742659,
0.0106634322264908));
#45688=CARTESIAN_POINT('Ctrl Pts',(-0.220147977225147,0.00813374905043262,
0.0106623784596957));
#45689=CARTESIAN_POINT('Ctrl Pts',(-0.220151169572582,0.00812650208014952,
0.010559914278616));
#45690=CARTESIAN_POINT('Ctrl Pts',(-0.220133573386841,0.00688792809120517,
0.0107484830823553));
#45691=CARTESIAN_POINT('Ctrl Pts',(-0.220031425127958,0.0068989046609728,
0.010748807990965));
#45692=CARTESIAN_POINT('Ctrl Pts',(-0.220034649032527,0.00690588109330772,
0.0106453391107511));
#45693=CARTESIAN_POINT('Ctrl Pts',(-0.219994804021819,0.00506747611300468,
0.0104977512748514));
#45694=CARTESIAN_POINT('Ctrl Pts',(-0.219891389349097,0.00506853282168791,
0.010499938160873));
#45695=CARTESIAN_POINT('Ctrl Pts',(-0.219894504064411,0.00509592002633516,
0.0103992372092036));
#45696=CARTESIAN_POINT('Ctrl Pts',(-0.220203419609321,0.00275378968309817,
0.00942103991272318));
#45697=CARTESIAN_POINT('Ctrl Pts',(-0.220101811139137,0.00273816330361558,
0.00941287454677868));
#45698=CARTESIAN_POINT('Ctrl Pts',(-0.220104476366608,0.00279222836967903,
0.00932461133402498));
#45699=CARTESIAN_POINT('Ctrl Pts',(-0.220503433261061,0.00177703780097305,
0.00869404760028399));
#45700=CARTESIAN_POINT('Ctrl Pts',(-0.220403503423106,0.00175796626419382,
0.00867923883869439));
#45701=CARTESIAN_POINT('Ctrl Pts',(-0.22040590406413,0.00182286455694324,
0.00859915204344728));
#45702=CARTESIAN_POINT('Ctrl Pts',(-0.220649949295114,0.00125070731346161,
0.0082007135299242));
#45703=CARTESIAN_POINT('Ctrl Pts',(-0.220549235546056,0.00123534032793399,
0.00818683084179405));
#45704=CARTESIAN_POINT('Ctrl Pts',(-0.220551438904638,0.00130625601097892,
0.00811242254542717));
#45705=CARTESIAN_POINT('Ctrl Pts',(-0.220093674791071,0.0074975850117286,
0.0105819125063979));
#45706=CARTESIAN_POINT('Ctrl Pts',(-0.220093526920449,0.00749758320628809,
0.0105884551073401));
#45707=CARTESIAN_POINT('Ctrl Pts',(-0.220094024045747,0.007497581232436,
0.0105949960431337));
#45708=CARTESIAN_POINT('Ctrl Pts',(-0.220096365411539,0.00749757686947963,
0.0106082955073979));
#45709=CARTESIAN_POINT('Ctrl Pts',(-0.220098286603548,0.00749757447419758,
0.0106150042638252));
#45710=CARTESIAN_POINT('Ctrl Pts',(-0.220105708909756,0.00749756733743141,
0.0106334048657344));
#45711=CARTESIAN_POINT('Ctrl Pts',(-0.220112794418493,0.00749756240258949,
0.0106443048720408));
#45712=CARTESIAN_POINT('Ctrl Pts',(-0.220130709373825,0.00749755245577472,
0.0106628288801252));
#45713=CARTESIAN_POINT('Ctrl Pts',(-0.220141372895899,0.00749754755040115,
0.0106702784560354));
#45714=CARTESIAN_POINT('Ctrl Pts',(-0.220172671231308,0.00749753517796745,
0.0106841865494111));
#45715=CARTESIAN_POINT('Ctrl Pts',(-0.220189205266996,0.00749757396411134,
0.0106840868768587));
#45716=CARTESIAN_POINT('Ctrl Pts',(-0.220191303401166,0.00749750031916177,
0.0106841483771092));
#45717=CARTESIAN_POINT('Ctrl Pts',(-0.220191746640651,0.00749753084563371,
0.0106841591947775));
#45718=CARTESIAN_POINT('Ctrl Pts',(-0.220150708821755,0.00687195702680685,
0.010559884303056));
#45719=CARTESIAN_POINT('Ctrl Pts',(-0.22014759399109,0.00686468413303138,
0.0106625473046195));
#45720=CARTESIAN_POINT('Ctrl Pts',(-0.220250229267773,0.0068730627295562,
0.0106633257059033));
#45721=CARTESIAN_POINT('Ctrl Pts',(-0.220034720928684,0.00808612268880879,
0.0106450343427239));
#45722=CARTESIAN_POINT('Ctrl Pts',(-0.220031574719443,0.00809303072895467,
0.0107486971037965));
#45723=CARTESIAN_POINT('Ctrl Pts',(-0.220133932562721,0.00810398139678503,
0.0107480825139144));
#45724=CARTESIAN_POINT('Ctrl Pts',(-0.219898939957643,0.00988609461928639,
0.0104026796240758));
#45725=CARTESIAN_POINT('Ctrl Pts',(-0.219895900748701,0.00991331796087509,
0.0105036180132768));
#45726=CARTESIAN_POINT('Ctrl Pts',(-0.219999481369186,0.0099141547094306,
0.0105012650911866));
#45727=CARTESIAN_POINT('Ctrl Pts',(-0.220104216028228,0.0121807920431273,
0.00934034778981266));
#45728=CARTESIAN_POINT('Ctrl Pts',(-0.220101623005436,0.0122346429002561,
0.00942896565106837));
#45729=CARTESIAN_POINT('Ctrl Pts',(-0.220203474394453,0.0122190459273884,
0.00943671421502881));
#45730=CARTESIAN_POINT('Ctrl Pts',(-0.220406547486447,0.0131480054901679,
0.00862237289776044));
#45731=CARTESIAN_POINT('Ctrl Pts',(-0.220404214515825,0.0132126844151198,
0.00870289002102647));
#45732=CARTESIAN_POINT('Ctrl Pts',(-0.220504233003487,0.0131929487356747,
0.00871771614458468));
#45733=CARTESIAN_POINT('Ctrl Pts',(-0.220553604100269,0.0136631541416016,
0.00814156304176045));
#45734=CARTESIAN_POINT('Ctrl Pts',(-0.220551464853133,0.0137338357445961,
0.00821646744183325));
#45735=CARTESIAN_POINT('Ctrl Pts',(-0.22065234139264,0.0137181149325072,
0.00823021086189709));
#45736=CARTESIAN_POINT('Ctrl Pts',(-0.217137874468735,0.008030785389101,
0.0104987600271184));
#45737=CARTESIAN_POINT('Ctrl Pts',(-0.217135999376533,0.00803730846625089,
0.010607296817054));
#45738=CARTESIAN_POINT('Ctrl Pts',(-0.217028124738702,0.00804529143374969,
0.0105958336575828));
#45739=CARTESIAN_POINT('Ctrl Pts',(-0.217053923565904,0.00696476469087671,
0.0105605954778132));
#45740=CARTESIAN_POINT('Ctrl Pts',(-0.217052029443782,0.00695824947239747,
0.0106699234267572));
#45741=CARTESIAN_POINT('Ctrl Pts',(-0.216944400117764,0.00696910854709431,
0.0106593295604461));
#45742=CARTESIAN_POINT('Ctrl Pts',(-0.216834795596937,0.0048122033769108,
0.0102961809446762));
#45743=CARTESIAN_POINT('Ctrl Pts',(-0.216833012543114,0.00478002238563605,
0.010402360493829));
#45744=CARTESIAN_POINT('Ctrl Pts',(-0.216723776467451,0.00478370698650778,
0.0103954490239756));
#45745=CARTESIAN_POINT('Ctrl Pts',(-0.217137701377203,0.00290143240652124,
0.00932526468848566));
#45746=CARTESIAN_POINT('Ctrl Pts',(-0.217136369590972,0.00284578989718424,
0.00941959858197015));
#45747=CARTESIAN_POINT('Ctrl Pts',(-0.217029631656927,0.00283459991226262,
0.00940110164852008));
#45748=CARTESIAN_POINT('Ctrl Pts',(-0.217300533120515,0.00206565219928745,
0.00869660496702258));
#45749=CARTESIAN_POINT('Ctrl Pts',(-0.217299461055391,0.00200015998946544,
0.00878340995987883));
#45750=CARTESIAN_POINT('Ctrl Pts',(-0.21719227419963,0.00199426821917551,
0.0087660056028655));
#45751=CARTESIAN_POINT('Ctrl Pts',(-0.217213240235122,0.00253454644557544,
0.00902670532692319));
#45752=CARTESIAN_POINT('Ctrl Pts',(-0.217213132107947,0.00253076598515692,
0.00903238191218357));
#45753=CARTESIAN_POINT('Ctrl Pts',(-0.217212380884729,0.0025266614085604,
0.00903779101041478));
#45754=CARTESIAN_POINT('Ctrl Pts',(-0.217209531777293,0.00251761914705192,
0.00904828662234579));
#45755=CARTESIAN_POINT('Ctrl Pts',(-0.217207353950518,0.00251268911402758,
0.00905326629660996));
#45756=CARTESIAN_POINT('Ctrl Pts',(-0.217199347813401,0.00249824154810511,
0.0090659359008687));
#45757=CARTESIAN_POINT('Ctrl Pts',(-0.217192101359339,0.00248855360873053,
0.0090722069176123));
#45758=CARTESIAN_POINT('Ctrl Pts',(-0.217174446526582,0.00246944770445475,
0.00908065823763552));
#45759=CARTESIAN_POINT('Ctrl Pts',(-0.217164116546706,0.00246020276307118,
0.00908266823978674));
#45760=CARTESIAN_POINT('Ctrl Pts',(-0.217144135035235,0.00244514628396083,
0.00908235046140921));
#45761=CARTESIAN_POINT('Ctrl Pts',(-0.217134775069224,0.00243902751563067,
0.00908076767243162));
#45762=CARTESIAN_POINT('Ctrl Pts',(-0.217123400409096,0.00243272926083712,
0.0090773181822219));
#45763=CARTESIAN_POINT('Ctrl Pts',(-0.217121274018224,0.00243155301768911,
0.00907658389939519));
#45764=CARTESIAN_POINT('Ctrl Pts',(-0.217119277829696,0.00243052048892982,
0.0090758545613406));
#45765=CARTESIAN_POINT('Ctrl Pts',(-0.217094602388958,0.00749884757784041,
0.0105144330190784));
#45766=CARTESIAN_POINT('Ctrl Pts',(-0.21709443736718,0.0074988465877603,
0.0105208742316926));
#45767=CARTESIAN_POINT('Ctrl Pts',(-0.217093648086457,0.00749884575649302,
0.0105272842319109));
#45768=CARTESIAN_POINT('Ctrl Pts',(-0.217090731117228,0.00749884434847888,
0.0105403659619601));
#45769=CARTESIAN_POINT('Ctrl Pts',(-0.217088509644837,0.00749884380187818,
0.0105469808193619));
#45770=CARTESIAN_POINT('Ctrl Pts',(-0.217080266789553,0.00749884271946781,
0.0105650264924206));
#45771=CARTESIAN_POINT('Ctrl Pts',(-0.217072698879009,0.00749884263169673,
0.0105755954190497));
#45772=CARTESIAN_POINT('Ctrl Pts',(-0.2170539717794,0.00749884292283719,
0.0105932912156081));
#45773=CARTESIAN_POINT('Ctrl Pts',(-0.21704298650683,0.0074988437000847,
0.0106002517588459));
#45774=CARTESIAN_POINT('Ctrl Pts',(-0.217019111256083,0.00749884076347341,
0.0106095973639871));
#45775=CARTESIAN_POINT('Ctrl Pts',(-0.217008118866313,0.00749888689621046,
0.0106113615914812));
#45776=CARTESIAN_POINT('Ctrl Pts',(-0.216997761731594,0.0074987818105982,
0.0106118145058692));
#45777=CARTESIAN_POINT('Ctrl Pts',(-0.216995371561048,0.00749881704992926,
0.0106118871769746));
#45778=CARTESIAN_POINT('Ctrl Pts',(-0.216992988389039,0.00749886191827281,
0.0106118645637799));
#45779=CARTESIAN_POINT('Ctrl Pts',(-0.216992039555683,0.0074988622638103,
0.0106118431559742));
#45780=CARTESIAN_POINT('Ctrl Pts',(-0.217307543356349,0.0129460293259321,
0.00868783863166776));
#45781=CARTESIAN_POINT('Ctrl Pts',(-0.217306819903283,0.013011671669317,
0.00877462975554483));
#45782=CARTESIAN_POINT('Ctrl Pts',(-0.217199541099427,0.0130177509641774,
0.00875739725535199));
#45783=CARTESIAN_POINT('Ctrl Pts',(-0.217142206976129,0.0120960223538591,
0.00932778214574832));
#45784=CARTESIAN_POINT('Ctrl Pts',(-0.217141217622965,0.0121516216063133,
0.00942224602098435));
#45785=CARTESIAN_POINT('Ctrl Pts',(-0.217034385733589,0.0121629501148438,
0.00940397474918907));
#45786=CARTESIAN_POINT('Ctrl Pts',(-0.216836257913023,0.010185646463759,
0.0102967050880177));
#45787=CARTESIAN_POINT('Ctrl Pts',(-0.216834826013361,0.010217830511706,
0.0104029574503101));
#45788=CARTESIAN_POINT('Ctrl Pts',(-0.216725490864702,0.0102144787022243,
0.0103962399214122));
#45789=CARTESIAN_POINT('Ctrl Pts',(-0.217054853915967,0.00802435938547715,
0.0105612587075268));
#45790=CARTESIAN_POINT('Ctrl Pts',(-0.217053305388005,0.00803077937328534,
0.0106706759148725));
#45791=CARTESIAN_POINT('Ctrl Pts',(-0.216945574819892,0.00801993045571461,
0.0106603452175849));
#45792=CARTESIAN_POINT('Ctrl Pts',(-0.217138149622957,0.00696060513773728,
0.0104977725037612));
#45793=CARTESIAN_POINT('Ctrl Pts',(-0.217136621510629,0.00695400059961224,
0.010606380722123));
#45794=CARTESIAN_POINT('Ctrl Pts',(-0.217028641347721,0.00694608024100671,
0.0105951772770944));
#45795=CARTESIAN_POINT('Ctrl Pts',(-0.217217404929227,0.0124620146248922,
0.00902905891344479));
#45796=CARTESIAN_POINT('Ctrl Pts',(-0.217217292950013,0.0124659537352925,
0.00903497088109792));
#45797=CARTESIAN_POINT('Ctrl Pts',(-0.217216495254757,0.0124703056948511,
0.00904054042042587));
#45798=CARTESIAN_POINT('Ctrl Pts',(-0.217213467856878,0.0124800507372417,
0.00905123743169844));
#45799=CARTESIAN_POINT('Ctrl Pts',(-0.217211148470925,0.0124854342259932,
0.00905622188096938));
#45800=CARTESIAN_POINT('Ctrl Pts',(-0.21720293947776,0.0125008317760289,
0.00906822295320578));
#45801=CARTESIAN_POINT('Ctrl Pts',(-0.217195796422827,0.0125110476227904,
0.00907375635273045));
#45802=CARTESIAN_POINT('Ctrl Pts',(-0.217178399375296,0.0125317585520276,
0.00908079249600287));
#45803=CARTESIAN_POINT('Ctrl Pts',(-0.217168102183229,0.0125420742072453,
0.0090819563423573));
#45804=CARTESIAN_POINT('Ctrl Pts',(-0.217140656078641,0.0125658047878956,
0.00907922929733444));
#45805=CARTESIAN_POINT('Ctrl Pts',(-0.217127225849111,0.0125741931915602,
0.00907284312855735));
#45806=CARTESIAN_POINT('Ctrl Pts',(-0.217125518265942,0.012575247500853,
0.00907211843792538));
#45807=CARTESIAN_POINT('Ctrl Pts',(-0.217125430481138,0.0125753249905193,
0.00907206576885612));
#45808=CARTESIAN_POINT('Ctrl Pts',(-0.217125136225254,0.0125755132818,0.00907193395437536));
#45809=CARTESIAN_POINT('Ctrl Pts',(-0.218505927384742,0.00219420861527787,
0.00893903540143742));
#45810=CARTESIAN_POINT('Ctrl Pts',(-0.218506576680989,0.00227829750388311,
0.00900996719729256));
#45811=CARTESIAN_POINT('Ctrl Pts',(-0.218508231183922,0.00234104950524819,
0.00892018804324298));
#45812=CARTESIAN_POINT('Ctrl Pts',(-0.218245421085756,0.0022043243771477,
0.0089411823686304));
#45813=CARTESIAN_POINT('Ctrl Pts',(-0.2182472119187,0.0022867159623372,
0.00901075868610424));
#45814=CARTESIAN_POINT('Ctrl Pts',(-0.218249117191188,0.00234931542687908,
0.00892093265387189));
#45815=CARTESIAN_POINT('Ctrl Pts',(-0.217712828506656,0.00217687540292711,
0.00891143052286725));
#45816=CARTESIAN_POINT('Ctrl Pts',(-0.217704611098061,0.00226956574195701,
0.00898827016224622));
#45817=CARTESIAN_POINT('Ctrl Pts',(-0.217705766229126,0.0023324873031235,
0.0088983393941371));
#45818=CARTESIAN_POINT('Ctrl Pts',(-0.217210903661233,0.00234921543953796,
0.00902402719766558));
#45819=CARTESIAN_POINT('Ctrl Pts',(-0.217284478791233,0.00241352385102592,
0.00907980326016165));
#45820=CARTESIAN_POINT('Ctrl Pts',(-0.217285575413226,0.0024746238390022,
0.00898952645001293));
#45821=CARTESIAN_POINT('Ctrl Pts',(-0.217008784931119,0.00249299341869297,
0.00911473622767726));
#45822=CARTESIAN_POINT('Ctrl Pts',(-0.217066036533421,0.00256425859926955,
0.00917304859362285));
#45823=CARTESIAN_POINT('Ctrl Pts',(-0.217067500167738,0.00262345357409097,
0.00908135538656866));
#45824=CARTESIAN_POINT('Ctrl Pts',(-0.218256634048459,0.00234470650638891,
0.00891994458535368));
#45825=CARTESIAN_POINT('Ctrl Pts',(-0.218256626639177,0.00234040530459759,
0.00892588558602306));
#45826=CARTESIAN_POINT('Ctrl Pts',(-0.218257578582534,0.00233552000606212,
0.0089312472304899));
#45827=CARTESIAN_POINT('Ctrl Pts',(-0.218261540417236,0.00232380224523273,
0.00894167585285985));
#45828=CARTESIAN_POINT('Ctrl Pts',(-0.218264856613629,0.00231697352292472,
0.00894629386253098));
#45829=CARTESIAN_POINT('Ctrl Pts',(-0.218275580156686,0.00229875209470095,
0.00895589403300023));
#45830=CARTESIAN_POINT('Ctrl Pts',(-0.218284702888905,0.00228640941556886,
0.00895969840013095));
#45831=CARTESIAN_POINT('Ctrl Pts',(-0.218306314313981,0.00226165582803696,
0.00896251059574449));
#45832=CARTESIAN_POINT('Ctrl Pts',(-0.218317875037794,0.00225009136726339,
0.00896169726079228));
#45833=CARTESIAN_POINT('Ctrl Pts',(-0.218341505795055,0.00222871318891932,
0.00895689458922));
#45834=CARTESIAN_POINT('Ctrl Pts',(-0.218353842689428,0.00221868141491273,
0.00895283427796545));
#45835=CARTESIAN_POINT('Ctrl Pts',(-0.218368730666572,0.00220769525572976,
0.0089463082783215));
#45836=CARTESIAN_POINT('Ctrl Pts',(-0.218371385735275,0.00220579459015017,
0.00894509374435352));
#45837=CARTESIAN_POINT('Ctrl Pts',(-0.218374005680645,0.00220395032896211,
0.00894382649250058));
#45838=CARTESIAN_POINT('Ctrl Pts',(-0.218489629254318,0.012611151918198,
0.00895310221279096));
#45839=CARTESIAN_POINT('Ctrl Pts',(-0.218487674841287,0.0126745742874925,
0.00904502916129814));
#45840=CARTESIAN_POINT('Ctrl Pts',(-0.218504904302657,0.0127576089696995,
0.00897317862838708));
#45841=CARTESIAN_POINT('Ctrl Pts',(-0.218222750307536,0.012661502377565,
0.00891280999119246));
#45842=CARTESIAN_POINT('Ctrl Pts',(-0.218220592929847,0.0127255073996101,
0.00900432897252887));
#45843=CARTESIAN_POINT('Ctrl Pts',(-0.218253673945024,0.0128079644187064,
0.00893229925480229));
#45844=CARTESIAN_POINT('Ctrl Pts',(-0.217766142708494,0.0126829340915357,
0.00888986543619831));
#45845=CARTESIAN_POINT('Ctrl Pts',(-0.217765157221868,0.0127472329221916,
0.00898121583622291));
#45846=CARTESIAN_POINT('Ctrl Pts',(-0.217717535145496,0.0128304182181186,
0.00890691214413009));
#45847=CARTESIAN_POINT('Ctrl Pts',(-0.217283803131409,0.0124821711351596,
0.00901759047954861));
#45848=CARTESIAN_POINT('Ctrl Pts',(-0.217282399769762,0.0125439262817006,
0.00911041470209943));
#45849=CARTESIAN_POINT('Ctrl Pts',(-0.217240271304298,0.012620944820576,
0.009044103947773));
#45850=CARTESIAN_POINT('Ctrl Pts',(-0.217043935029806,0.0124005232817256,
0.00906509087384854));
#45851=CARTESIAN_POINT('Ctrl Pts',(-0.217042471015379,0.012461219665155,
0.0091586465875576));
#45852=CARTESIAN_POINT('Ctrl Pts',(-0.217000060226919,0.0125405600879245,
0.00909203027864609));
#45853=CARTESIAN_POINT('Ctrl Pts',(-0.218253210572638,0.0126493218644601,
0.00892398112026186));
#45854=CARTESIAN_POINT('Ctrl Pts',(-0.218255261351961,0.0126731190888775,
0.00895794646059297));
#45855=CARTESIAN_POINT('Ctrl Pts',(-0.218298695621072,0.0127283794650483,
0.00899134738316015));
#45856=CARTESIAN_POINT('Ctrl Pts',(-0.218374738263889,0.0127707341741232,
0.0089594649654453));
#45857=CARTESIAN_POINT('Ctrl Pts',(-0.218370607902533,0.00180941438383972,
0.00851604478529543));
#45858=CARTESIAN_POINT('Ctrl Pts',(-0.218368285855028,0.00174473477363733,
0.00859546721180872));
#45859=CARTESIAN_POINT('Ctrl Pts',(-0.218469416891288,0.00175757178993804,
0.00860579739743824));
#45860=CARTESIAN_POINT('Ctrl Pts',(-0.218268644565581,0.00230105693080552,
0.00891381537685727));
#45861=CARTESIAN_POINT('Ctrl Pts',(-0.218266160139693,0.00224200310180626,
0.00899779099512986));
#45862=CARTESIAN_POINT('Ctrl Pts',(-0.218366775119483,0.00225777155667148,
0.00900884727234041));
#45863=CARTESIAN_POINT('Ctrl Pts',(-0.218048286160621,0.00322871717535582,
0.00951870881413451));
#45864=CARTESIAN_POINT('Ctrl Pts',(-0.218045567620402,0.00317998919478594,
0.00960947751407076));
#45865=CARTESIAN_POINT('Ctrl Pts',(-0.21814730176867,0.00319244194660178,
0.00961555565315444));
#45866=CARTESIAN_POINT('Ctrl Pts',(-0.217912216784612,0.0053435724410554,
0.0103893198794707));
#45867=CARTESIAN_POINT('Ctrl Pts',(-0.217909140610329,0.00531923057262254,
0.0104901173983572));
#45868=CARTESIAN_POINT('Ctrl Pts',(-0.218012029342262,0.00531695415747033,
0.0104884940391751));
#45869=CARTESIAN_POINT('Ctrl Pts',(-0.218040501648908,0.00696434230067764,
0.0105877544423164));
#45870=CARTESIAN_POINT('Ctrl Pts',(-0.218037334717472,0.00695806260383963,
0.0106907323437167));
#45871=CARTESIAN_POINT('Ctrl Pts',(-0.218139167571268,0.00694719575757316,
0.0106907713966397));
#45872=CARTESIAN_POINT('Ctrl Pts',(-0.218146972284269,0.00806696358112366,
0.0105188716989655));
#45873=CARTESIAN_POINT('Ctrl Pts',(-0.218143831668603,0.00807348051114177,
0.0106210514411844));
#45874=CARTESIAN_POINT('Ctrl Pts',(-0.218245905616467,0.00806488518621087,
0.0106223363913482));
#45875=CARTESIAN_POINT('Ctrl Pts',(-0.218192328422137,0.00749852093264668,
0.0106389711280447));
#45876=CARTESIAN_POINT('Ctrl Pts',(-0.218154305198807,0.00749977351117825,
0.0106381083927364));
#45877=CARTESIAN_POINT('Ctrl Pts',(-0.218121877726077,0.0075010566023537,
0.0106133985656208));
#45878=CARTESIAN_POINT('Ctrl Pts',(-0.218107640643032,0.00750094174584491,
0.0105885860309675));
#45879=CARTESIAN_POINT('Ctrl Pts',(-0.218097197572745,0.00750085749722526,
0.0105703857407404));
#45880=CARTESIAN_POINT('Ctrl Pts',(-0.218094029662777,0.0075002408200837,
0.0105524183613623));
#45881=CARTESIAN_POINT('Ctrl Pts',(-0.218094302901274,0.00749931921466459,
0.0105367255362189));
#45882=CARTESIAN_POINT('Origin',(-0.22171405081414,0.00791637279634685,
0.00318516322693479));
#45883=CARTESIAN_POINT('Ctrl Pts',(-0.215138270481614,0.00801653871855295,
0.0104545941803276));
#45884=CARTESIAN_POINT('Ctrl Pts',(-0.215136339530633,0.00802279480318382,
0.0105617554450719));
#45885=CARTESIAN_POINT('Ctrl Pts',(-0.215029738537428,0.0080309281096567,
0.0105517178004985));
#45886=CARTESIAN_POINT('Ctrl Pts',(-0.215054199654782,0.00697916618023934,
0.01051252586723));
#45887=CARTESIAN_POINT('Ctrl Pts',(-0.21505225151283,0.00697293458855082,
0.0106204169830234));
#45888=CARTESIAN_POINT('Ctrl Pts',(-0.214945874857355,0.00698382690371717,
0.0106113028447007));
#45889=CARTESIAN_POINT('Ctrl Pts',(-0.214841833023336,0.0048911525456576,
0.010264819707883));
#45890=CARTESIAN_POINT('Ctrl Pts',(-0.214839984604383,0.00486043155357993,
0.0103698241720069));
#45891=CARTESIAN_POINT('Ctrl Pts',(-0.214732132555284,0.00486330753472638,
0.0103638864488541));
#45892=CARTESIAN_POINT('Ctrl Pts',(-0.215123102029791,0.00301006841920348,
0.00934454242151527));
#45893=CARTESIAN_POINT('Ctrl Pts',(-0.215121678625563,0.00295659535466086,
0.00943847740912549));
#45894=CARTESIAN_POINT('Ctrl Pts',(-0.215015965458248,0.0029460175374489,
0.00942222581375646));
#45895=CARTESIAN_POINT('Ctrl Pts',(-0.215268667797406,0.00217542510416371,
0.00873918816030454));
#45896=CARTESIAN_POINT('Ctrl Pts',(-0.215267493810616,0.00211227092821834,
0.008825991556164));
#45897=CARTESIAN_POINT('Ctrl Pts',(-0.215161402439874,0.0021063441397646,
0.0088106397707087));
#45898=CARTESIAN_POINT('Ctrl Pts',(-0.215095387779062,0.00254083911603525,
0.00910817608666392));
#45899=CARTESIAN_POINT('Ctrl Pts',(-0.21512037463289,0.00256400002101044,
0.00912360420379185));
#45900=CARTESIAN_POINT('Ctrl Pts',(-0.215133745878006,0.00258169558032891,
0.00912601392496322));
#45901=CARTESIAN_POINT('Ctrl Pts',(-0.215148676560894,0.00260130634252768,
0.00912383356325065));
#45902=CARTESIAN_POINT('Ctrl Pts',(-0.215150273563903,0.00260340393220061,
0.00912360034925493));
#45903=CARTESIAN_POINT('Ctrl Pts',(-0.215151889432577,0.00260554977826508,
0.0091232734480787));
#45904=CARTESIAN_POINT('Ctrl Pts',(-0.215153528948729,0.00260776901397922,
0.00912283471210183));
#45905=CARTESIAN_POINT('Ctrl Pts',(-0.215170496594165,0.00263073628068582,
0.0091182941551298));
#45906=CARTESIAN_POINT('Ctrl Pts',(-0.215184361861634,0.00266180392841244,
0.00909996890792453));
#45907=CARTESIAN_POINT('Ctrl Pts',(-0.21518479796162,0.00267607596988323,
0.00907755560002423));
#45908=CARTESIAN_POINT('Ctrl Pts',(-0.215095211620886,0.00749946305213359,
0.0104691619661793));
#45909=CARTESIAN_POINT('Ctrl Pts',(-0.215095051270524,0.00749946252715341,
0.0104756317925372));
#45910=CARTESIAN_POINT('Ctrl Pts',(-0.215094261018183,0.00749946210845811,
0.0104820704988108));
#45911=CARTESIAN_POINT('Ctrl Pts',(-0.215091337124818,0.00749946144379272,
0.0104951805243167));
#45912=CARTESIAN_POINT('Ctrl Pts',(-0.215089114951798,0.00749946121552005,
0.0105017959519679));
#45913=CARTESIAN_POINT('Ctrl Pts',(-0.215080869890318,0.00749946084296753,
0.0105198422392518));
#45914=CARTESIAN_POINT('Ctrl Pts',(-0.215073300383325,0.00749946096680242,
0.0105304108795332));
#45915=CARTESIAN_POINT('Ctrl Pts',(-0.215054569912047,0.00749946128003418,
0.0105481059791543));
#45916=CARTESIAN_POINT('Ctrl Pts',(-0.21504358277679,0.00749946180673463,
0.0105550659716542));
#45917=CARTESIAN_POINT('Ctrl Pts',(-0.215018712085791,0.00749945861210784,
0.0105647986730059));
#45918=CARTESIAN_POINT('Ctrl Pts',(-0.215007312676018,0.00749948519567766,
0.0105662336960224));
#45919=CARTESIAN_POINT('Ctrl Pts',(-0.214998324007091,0.00749940758554542,
0.0105666280985719));
#45920=CARTESIAN_POINT('Ctrl Pts',(-0.21499598086407,0.00749943731930172,
0.010566697535465));
#45921=CARTESIAN_POINT('Ctrl Pts',(-0.214993636732782,0.00749947573716579,
0.0105666778348444));
#45922=CARTESIAN_POINT('Ctrl Pts',(-0.214992640535139,0.00749947588860775,
0.0105666554240425));
#45923=CARTESIAN_POINT('Ctrl Pts',(-0.215271612902418,0.0128241679430378,
0.00873958050001579));
#45924=CARTESIAN_POINT('Ctrl Pts',(-0.215270600712745,0.0128872591163074,
0.00882634285591854));
#45925=CARTESIAN_POINT('Ctrl Pts',(-0.215164566564404,0.0128933475034878,
0.00881117707783499));
#45926=CARTESIAN_POINT('Ctrl Pts',(-0.215125346805473,0.0119839960519677,
0.00934778460885941));
#45927=CARTESIAN_POINT('Ctrl Pts',(-0.215124083651265,0.0120373410606281,
0.0094417082717187));
#45928=CARTESIAN_POINT('Ctrl Pts',(-0.215018426721982,0.0120480293424221,
0.00942567701482509));
#45929=CARTESIAN_POINT('Ctrl Pts',(-0.214843451277587,0.010112463684472,
0.0102630293596174));
#45930=CARTESIAN_POINT('Ctrl Pts',(-0.214841768792085,0.0101432088582359,
0.0103679387850742));
#45931=CARTESIAN_POINT('Ctrl Pts',(-0.214733973527544,0.0101405822780667,
0.0103621781245389));
#45932=CARTESIAN_POINT('Ctrl Pts',(-0.215054297296728,0.00801821343807021,
0.0105127492974011));
#45933=CARTESIAN_POINT('Ctrl Pts',(-0.215052511950845,0.00802442511231975,
0.0106205721752317));
#45934=CARTESIAN_POINT('Ctrl Pts',(-0.214946184595913,0.00801356394386956,
0.0106117052262838));
#45935=CARTESIAN_POINT('Ctrl Pts',(-0.215138103483795,0.00698312146912351,
0.0104542920384517));
#45936=CARTESIAN_POINT('Ctrl Pts',(-0.215136335928839,0.00697687891345948,
0.0105613808476118));
#45937=CARTESIAN_POINT('Ctrl Pts',(-0.215029785457826,0.0069687779079764,
0.0105515847686282));
#45938=CARTESIAN_POINT('Ctrl Pts',(-0.21518738632965,0.0123215256882542,
0.00907911767190286));
#45939=CARTESIAN_POINT('Ctrl Pts',(-0.215186958732144,0.0123358311960233,
0.00910150651904035));
#45940=CARTESIAN_POINT('Ctrl Pts',(-0.215173114189427,0.0123669940601415,
0.00911976197539705));
#45941=CARTESIAN_POINT('Ctrl Pts',(-0.215156188916878,0.0123899124403107,
0.00912431683714909));
#45942=CARTESIAN_POINT('Ctrl Pts',(-0.215141006736465,0.0124104705129507,
0.00912840260490722));
#45943=CARTESIAN_POINT('Ctrl Pts',(-0.215129055078211,0.0124265747862727,
0.00912637222642325));
#45944=CARTESIAN_POINT('Ctrl Pts',(-0.215106250017454,0.0124489868903362,
0.00911441803181024));
#45945=CARTESIAN_POINT('Ctrl Pts',(-0.215103631701308,0.0124515600899674,
0.00911304553554294));
#45946=CARTESIAN_POINT('Ctrl Pts',(-0.215100882380107,0.0124541833998731,
0.00911149354874494));
#45947=CARTESIAN_POINT('Ctrl Pts',(-0.215098009459442,0.0124568456463797,
0.00910972113216459));
#45948=CARTESIAN_POINT('Origin',(-0.216343132180981,0.00254791657843158,
0.0090181005548472));
#45949=CARTESIAN_POINT('Ctrl Pts',(-0.216191667803065,0.0026370176797586,
0.00907415689238714));
#45950=CARTESIAN_POINT('Ctrl Pts',(-0.216191796566365,0.00262309746236483,
0.00909510774781046));
#45951=CARTESIAN_POINT('Ctrl Pts',(-0.216210204957318,0.00259351228337774,
0.00911334041689735));
#45952=CARTESIAN_POINT('Ctrl Pts',(-0.216228349712416,0.00256888190445406,
0.00911727926076771));
#45953=CARTESIAN_POINT('Ctrl Pts',(-0.21622997958263,0.00256666945679458,
0.00911763307123604));
#45954=CARTESIAN_POINT('Ctrl Pts',(-0.216231607982164,0.00256450993898164,
0.0091179055386048));
#45955=CARTESIAN_POINT('Ctrl Pts',(-0.216233221666543,0.00256242089040709,
0.00911810802884885));
#45956=CARTESIAN_POINT('Ctrl Pts',(-0.216251067152262,0.00253931842564724,
0.00912034733710838));
#45957=CARTESIAN_POINT('Ctrl Pts',(-0.216267135569045,0.00252489955735048,
0.00911810893501753));
#45958=CARTESIAN_POINT('Ctrl Pts',(-0.216295512027883,0.00250229745532596,
0.00910638817612955));
#45959=CARTESIAN_POINT('Ctrl Pts',(-0.216298673982971,0.00249977892995521,
0.00910508214589432));
#45960=CARTESIAN_POINT('Ctrl Pts',(-0.216301989265945,0.00249717858831983,
0.00910360948776118));
#45961=CARTESIAN_POINT('Ctrl Pts',(-0.216305478212088,0.00249450055261697,
0.0091019248989092));
#45962=CARTESIAN_POINT('Origin',(-0.215029763026557,0.0124000795960937,
0.00902581809007369));
#45963=CARTESIAN_POINT('Ctrl Pts',(-0.216308818597444,0.0125017236340575,
0.00910474588717665));
#45964=CARTESIAN_POINT('Ctrl Pts',(-0.216277529676922,0.0124777449670039,
0.00911980894330316));
#45965=CARTESIAN_POINT('Ctrl Pts',(-0.216259955722432,0.0124623601332724,
0.00912198910373754));
#45966=CARTESIAN_POINT('Ctrl Pts',(-0.216242122224109,0.0124407253367735,
0.00912127527717495));
#45967=CARTESIAN_POINT('Ctrl Pts',(-0.21624027025839,0.0124384786154227,
0.0091212011480109));
#45968=CARTESIAN_POINT('Ctrl Pts',(-0.216238415756952,0.0124361530299236,
0.00912105345816178));
#45969=CARTESIAN_POINT('Ctrl Pts',(-0.21623654299763,0.0124337307492349,
0.00912081197832088));
#45970=CARTESIAN_POINT('Ctrl Pts',(-0.21621848869826,0.0124103787999494,
0.00911848399666931));
#45971=CARTESIAN_POINT('Ctrl Pts',(-0.216198675184547,0.0123793078462243,
0.00910311913336652));
#45972=CARTESIAN_POINT('Ctrl Pts',(-0.216195447172136,0.0123631989134075,
0.00908219261644899));
#45973=CARTESIAN_POINT('Ctrl Pts',(-0.216195162186071,0.0123617767313345,
0.00908034511248652));
#45974=CARTESIAN_POINT('Ctrl Pts',(-0.2161950072882,0.012360451903129,0.00907848426629928));
#45975=CARTESIAN_POINT('Ctrl Pts',(-0.216194995682923,0.0123592255510163,
0.0090766289839036));
#45976=CARTESIAN_POINT('Ctrl Pts',(-0.216282811305448,0.00210699698509605,
0.00870789405373815));
#45977=CARTESIAN_POINT('Ctrl Pts',(-0.216280515760285,0.00204578096542595,
0.0087903315284613));
#45978=CARTESIAN_POINT('Ctrl Pts',(-0.216382322956288,0.00205681455673375,
0.00879811835758324));
#45979=CARTESIAN_POINT('Ctrl Pts',(-0.2161336968756,0.00294260178677836,
0.00932798061931376));
#45980=CARTESIAN_POINT('Ctrl Pts',(-0.216131148003743,0.00289072230453424,
0.00941741795418149));
#45981=CARTESIAN_POINT('Ctrl Pts',(-0.216232583643101,0.00290558261026826,
0.00942551757946072));
#45982=CARTESIAN_POINT('Ctrl Pts',(-0.21583544487376,0.00485581975852901,
0.0102857719853994));
#45983=CARTESIAN_POINT('Ctrl Pts',(-0.21583252840372,0.0048259645110555,
0.010386157855722));
#45984=CARTESIAN_POINT('Ctrl Pts',(-0.215936095167298,0.00482604039136546,
0.0103832490778077));
#45985=CARTESIAN_POINT('Ctrl Pts',(-0.216055652321081,0.00699289556514365,
0.0105372650696793));
#45986=CARTESIAN_POINT('Ctrl Pts',(-0.216052599771092,0.00698696979358537,
0.0106404709262405));
#45987=CARTESIAN_POINT('Ctrl Pts',(-0.216154764015332,0.00697690020144171,
0.010640271432368));
#45988=CARTESIAN_POINT('Ctrl Pts',(-0.216139423474306,0.00803607929674203,
0.0104756027513544));
#45989=CARTESIAN_POINT('Ctrl Pts',(-0.216136396349725,0.00804222090374004,
0.0105780850791528));
#45990=CARTESIAN_POINT('Ctrl Pts',(-0.216238791819397,0.00803398924503048,
0.010578878627741));
#45991=CARTESIAN_POINT('Ctrl Pts',(-0.216094905541403,0.00749916574467118,
0.0104915386727778));
#45992=CARTESIAN_POINT('Ctrl Pts',(-0.216094757687043,0.0074991648329644,
0.010498081812457));
#45993=CARTESIAN_POINT('Ctrl Pts',(-0.216095254807929,0.00749916380265483,
0.0105046233037114));
#45994=CARTESIAN_POINT('Ctrl Pts',(-0.216097596140649,0.00749916144150093,
0.0105179238150449));
#45995=CARTESIAN_POINT('Ctrl Pts',(-0.216099517294234,0.00749916010265018,
0.0105246331063143));
#45996=CARTESIAN_POINT('Ctrl Pts',(-0.216106938902494,0.007499155955148,
0.0105430335441308));
#45997=CARTESIAN_POINT('Ctrl Pts',(-0.216114023258208,0.00749915292472183,
0.01055393325295));
#45998=CARTESIAN_POINT('Ctrl Pts',(-0.2161319352607,0.00749914604860085,
0.010572456286503));
#45999=CARTESIAN_POINT('Ctrl Pts',(-0.216142596797795,0.00749914251354345,
0.0105799054483358));
#46000=CARTESIAN_POINT('Ctrl Pts',(-0.216165306353742,0.00749913251202104,
0.0105899977046191));
#46001=CARTESIAN_POINT('Ctrl Pts',(-0.216176121942762,0.00749916225956268,
0.0105925056055666));
#46002=CARTESIAN_POINT('Ctrl Pts',(-0.216187363138591,0.00749908779708458,
0.0105935062401521));
#46003=CARTESIAN_POINT('Ctrl Pts',(-0.216189644461058,0.00749910866675623,
0.0105936746436355));
#46004=CARTESIAN_POINT('Ctrl Pts',(-0.216191923222015,0.00749913622058534,
0.0105937606861201));
#46005=CARTESIAN_POINT('Ctrl Pts',(-0.216192971542667,0.00749913607619458,
0.0105937843838612));
#46006=CARTESIAN_POINT('Ctrl Pts',(-0.216139271434847,0.00696167292438563,
0.0104754199577516));
#46007=CARTESIAN_POINT('Ctrl Pts',(-0.216136032556292,0.0069554754642468,
0.0105781262309377));
#46008=CARTESIAN_POINT('Ctrl Pts',(-0.216238661874465,0.00696368361581323,
0.0105788967963663));
#46009=CARTESIAN_POINT('Ctrl Pts',(-0.216055749080497,0.00800701645360984,
0.0105367407275864));
#46010=CARTESIAN_POINT('Ctrl Pts',(-0.216052485301961,0.00801293344084057,
0.0106401701354799));
#46011=CARTESIAN_POINT('Ctrl Pts',(-0.216154883799805,0.00802300632093563,
0.0106399421743868));
#46012=CARTESIAN_POINT('Ctrl Pts',(-0.215836723914711,0.0101351578949112,
0.010288615649846));
#46013=CARTESIAN_POINT('Ctrl Pts',(-0.215833592413248,0.0101649786171273,
0.0103892619918857));
#46014=CARTESIAN_POINT('Ctrl Pts',(-0.215937391379544,0.010164739474805,
0.0103863667566106));
#46015=CARTESIAN_POINT('Ctrl Pts',(-0.216137685088785,0.0120577995594403,
0.0093274156971316));
#46016=CARTESIAN_POINT('Ctrl Pts',(-0.216134927581704,0.0121098292957299,
0.0094170278487481));
#46017=CARTESIAN_POINT('Ctrl Pts',(-0.216236585824584,0.0120949081867636,
0.00942513537855531));
#46018=CARTESIAN_POINT('Ctrl Pts',(-0.216285885406936,0.0128864817321484,
0.00871227969984319));
#46019=CARTESIAN_POINT('Ctrl Pts',(-0.216283378885618,0.0129477820406068,
0.00879493367149495));
#46020=CARTESIAN_POINT('Ctrl Pts',(-0.216385410595137,0.0129366667576193,
0.00880273281431371));
#46021=CARTESIAN_POINT('Ctrl Pts',(-0.192428879980893,0.0120843945331614,
0.0087649457194958));
#46022=CARTESIAN_POINT('Ctrl Pts',(-0.192427684894032,0.0121357661329368,
0.00885788569507324));
#46023=CARTESIAN_POINT('Ctrl Pts',(-0.192388028297364,0.0122187879722831,
0.00880424655434642));
#46024=CARTESIAN_POINT('Ctrl Pts',(-0.192151323086433,0.0119795060504334,
0.00881770899823756));
#46025=CARTESIAN_POINT('Ctrl Pts',(-0.192149856911976,0.0120295605951977,
0.00891133291804273));
#46026=CARTESIAN_POINT('Ctrl Pts',(-0.192109296359608,0.0121115249848374,
0.00885952921437927));
#46027=CARTESIAN_POINT('Ctrl Pts',(-0.191564603142634,0.0117903694463313,
0.00890698930513747));
#46028=CARTESIAN_POINT('Ctrl Pts',(-0.191564013677017,0.0118387145052195,
0.00900174454816317));
#46029=CARTESIAN_POINT('Ctrl Pts',(-0.191530667510288,0.0119326676422929,
0.00894707674718653));
#46030=CARTESIAN_POINT('Ctrl Pts',(-0.191125489451457,0.0114918545236309,
0.00904483726167067));
#46031=CARTESIAN_POINT('Ctrl Pts',(-0.191124463101182,0.0115367200971647,
0.00914043416370774));
#46032=CARTESIAN_POINT('Ctrl Pts',(-0.191036060600173,0.0115898425845301,
0.00910830917324193));
#46033=CARTESIAN_POINT('Ctrl Pts',(-0.190937349462523,0.0112538014290112,
0.00914481642408066));
#46034=CARTESIAN_POINT('Ctrl Pts',(-0.190936022194301,0.0112957769699949,
0.00924184994069289));
#46035=CARTESIAN_POINT('Ctrl Pts',(-0.190858698051812,0.0113582174074258,
0.0092072657414013));
#46036=CARTESIAN_POINT('Ctrl Pts',(-0.190965604317401,0.0114699046751051,
0.00915921566447933));
#46037=CARTESIAN_POINT('Ctrl Pts',(-0.190965712140185,0.0114693256191559,
0.00915945856588905));
#46038=CARTESIAN_POINT('Ctrl Pts',(-0.19096584960052,0.0114687652071312,
0.00915968912157385));
#46039=CARTESIAN_POINT('Ctrl Pts',(-0.190966623351059,0.0114662430478265,
0.00916070319296896));
#46040=CARTESIAN_POINT('Ctrl Pts',(-0.190967620055349,0.0114644811373346,
0.00916134408901796));
#46041=CARTESIAN_POINT('Ctrl Pts',(-0.190971301001675,0.0114599299463686,
0.00916272534006976));
#46042=CARTESIAN_POINT('Ctrl Pts',(-0.190974434960915,0.011457573567264,
0.00916308429216945));
#46043=CARTESIAN_POINT('Ctrl Pts',(-0.19098349851718,0.0114511312613147,
0.0091634866949268));
#46044=CARTESIAN_POINT('Ctrl Pts',(-0.190993053421979,0.0114456390258318,
0.00916252708498545));
#46045=CARTESIAN_POINT('Ctrl Pts',(-0.191014186860149,0.0114318448089166,
0.00915493967903766));
#46046=CARTESIAN_POINT('Ctrl Pts',(-0.191023959965254,0.0114246414658966,
0.00914875819715902));
#46047=CARTESIAN_POINT('Ctrl Pts',(-0.191038704796521,0.0114114486010586,
0.00913371410696604));
#46048=CARTESIAN_POINT('Ctrl Pts',(-0.191044101370854,0.0114055487134585,
0.00912550309845127));
#46049=CARTESIAN_POINT('Ctrl Pts',(-0.191051294287109,0.0113950265549819,
0.00910780083128093));
#46050=CARTESIAN_POINT('Ctrl Pts',(-0.191053300655896,0.0113904207832051,
0.00909861234382404));
#46051=CARTESIAN_POINT('Ctrl Pts',(-0.191053800278385,0.0113864428152143,
0.00908899053291756));
#46052=CARTESIAN_POINT('Ctrl Pts',(-0.1921323840585,0.0119768370000007,
0.00882020102336473));
#46053=CARTESIAN_POINT('Ctrl Pts',(-0.192132364786965,0.0119786721251219,
0.00882344223574507));
#46054=CARTESIAN_POINT('Ctrl Pts',(-0.192132589966708,0.0119807741225516,
0.0088264991122001));
#46055=CARTESIAN_POINT('Ctrl Pts',(-0.192133582901725,0.0119858894502443,
0.00883275520009954));
#46056=CARTESIAN_POINT('Ctrl Pts',(-0.1921344320636,0.011988948143783,0.00883581682223052));
#46057=CARTESIAN_POINT('Ctrl Pts',(-0.192138118929948,0.0119998831934135,
0.00884502631740865));
#46058=CARTESIAN_POINT('Ctrl Pts',(-0.192142050074175,0.0120085802053719,
0.0088496863821559));
#46059=CARTESIAN_POINT('Ctrl Pts',(-0.192154401339469,0.0120327292412066,
0.00885878096165628));
#46060=CARTESIAN_POINT('Ctrl Pts',(-0.192165255403088,0.0120508336147267,
0.00886133147853749));
#46061=CARTESIAN_POINT('Ctrl Pts',(-0.192196350964399,0.0120972880751649,
0.00885918763376293));
#46062=CARTESIAN_POINT('Ctrl Pts',(-0.192217846207761,0.0121258988100782,
0.00885155820539949));
#46063=CARTESIAN_POINT('Ctrl Pts',(-0.192243109585965,0.0121561496495416,
0.00883674354182499));
#46064=CARTESIAN_POINT('Ctrl Pts',(-0.192245681482551,0.0121592070619706,
0.00883516361505474));
#46065=CARTESIAN_POINT('Ctrl Pts',(-0.192248250704815,0.0121622138291422,
0.00883352725727037));
#46066=CARTESIAN_POINT('Ctrl Pts',(-0.192146287432863,0.007001445991187,
0.00993616740742011));
#46067=CARTESIAN_POINT('Ctrl Pts',(-0.192143234360962,0.0069960223197089,
0.0100379092428061));
#46068=CARTESIAN_POINT('Ctrl Pts',(-0.192244826903568,0.00700429955503233,
0.0100394799668714));
#46069=CARTESIAN_POINT('Ctrl Pts',(-0.192066737897779,0.00796348467110267,
0.00998615353633715));
#46070=CARTESIAN_POINT('Ctrl Pts',(-0.192063663567035,0.00796862002590671,
0.0100884509595953));
#46071=CARTESIAN_POINT('Ctrl Pts',(-0.192165062872102,0.00797874334461845,
0.0100891007288684));
#46072=CARTESIAN_POINT('Ctrl Pts',(-0.191868623073859,0.00992132327542535,
0.00978412510994995));
#46073=CARTESIAN_POINT('Ctrl Pts',(-0.191865654370179,0.00994730546079022,
0.00988429983653193));
#46074=CARTESIAN_POINT('Ctrl Pts',(-0.191968225046628,0.00994788503575821,
0.00988283229722599));
#46075=CARTESIAN_POINT('Ctrl Pts',(-0.192097500947389,0.011726822685467,
0.00900328990038117));
#46076=CARTESIAN_POINT('Ctrl Pts',(-0.192094870340512,0.0117725876792211,
0.00909494068949507));
#46077=CARTESIAN_POINT('Ctrl Pts',(-0.192195977838082,0.0117608643675088,
0.00910140164182352));
#46078=CARTESIAN_POINT('Ctrl Pts',(-0.192204910903453,0.0125394508655713,
0.00849025004975171));
#46079=CARTESIAN_POINT('Ctrl Pts',(-0.192202503077705,0.0125938763574182,
0.00857639379684929));
#46080=CARTESIAN_POINT('Ctrl Pts',(-0.192303866003295,0.0125851484834753,
0.00858255214977472));
#46081=CARTESIAN_POINT('Ctrl Pts',(-0.192104389150085,0.00749606093322131,
0.00994933148053198));
#46082=CARTESIAN_POINT('Ctrl Pts',(-0.192103965966015,0.00749467760198495,
0.00997324747001774));
#46083=CARTESIAN_POINT('Ctrl Pts',(-0.192111877116073,0.00749406236498253,
0.010004922477519));
#46084=CARTESIAN_POINT('Ctrl Pts',(-0.192141205886966,0.00749486189663908,
0.0100289347544931));
#46085=CARTESIAN_POINT('Ctrl Pts',(-0.192157026284705,0.00749529317651977,
0.0100418873522594));
#46086=CARTESIAN_POINT('Ctrl Pts',(-0.192179289265701,0.00749615081568364,
0.010051053680766));
#46087=CARTESIAN_POINT('Ctrl Pts',(-0.192202394110733,0.00749688548776383,
0.0100515763031989));
#46088=CARTESIAN_POINT('Origin',(-0.194644697133607,0.00789563648975762,
0.00208891925293578));
#46089=CARTESIAN_POINT('Ctrl Pts',(-0.191108295474911,0.00749762843016989,
0.00992693903429683));
#46090=CARTESIAN_POINT('Ctrl Pts',(-0.191106599644801,0.00749466645656951,
0.00996733235007675));
#46091=CARTESIAN_POINT('Ctrl Pts',(-0.191068850231782,0.00749416418348105,
0.010026720270591));
#46092=CARTESIAN_POINT('Ctrl Pts',(-0.191002065707968,0.00749708279836953,
0.0100253807384898));
#46093=CARTESIAN_POINT('Origin',(-0.195907470514249,0.00706161748354586,
0.00229602172434024));
#46094=CARTESIAN_POINT('Ctrl Pts',(-0.19224449469211,0.0028417662121083,
0.00883510047266706));
#46095=CARTESIAN_POINT('Ctrl Pts',(-0.192244116214055,0.00284188625041017,
0.00883516237725147));
#46096=CARTESIAN_POINT('Ctrl Pts',(-0.192243945000766,0.00284194509216338,
0.00883519239511538));
#46097=CARTESIAN_POINT('Ctrl Pts',(-0.19224376737675,0.00284200983416614,
0.00883522517817115));
#46098=CARTESIAN_POINT('Ctrl Pts',(-0.192243759668759,0.0028420126509833,
0.00883522660404886));
#46099=CARTESIAN_POINT('Ctrl Pts',(-0.192243661274495,0.00284204870176666,
0.0088352448471908));
#46100=CARTESIAN_POINT('Ctrl Pts',(-0.19224357098158,0.0028420827986193,
0.00883526203851272));
#46101=CARTESIAN_POINT('Ctrl Pts',(-0.192243259650548,0.00284220376464917,
0.00883532282286752));
#46102=CARTESIAN_POINT('Ctrl Pts',(-0.192243040657529,0.00284229483416492,
0.00883536823330852));
#46103=CARTESIAN_POINT('Ctrl Pts',(-0.19224234559644,0.00284260145477907,
0.00883552013874578));
#46104=CARTESIAN_POINT('Ctrl Pts',(-0.192241878182314,0.00284283467675889,
0.0088356342547113));
#46105=CARTESIAN_POINT('Ctrl Pts',(-0.192232081281346,0.00284818838957794,
0.00883822897286899));
#46106=CARTESIAN_POINT('Ctrl Pts',(-0.192217537131995,0.00286541958630876,
0.0088462686043001));
#46107=CARTESIAN_POINT('Ctrl Pts',(-0.192183195336512,0.00290883611484725,
0.00885719354998073));
#46108=CARTESIAN_POINT('Ctrl Pts',(-0.192167532798987,0.00293086406224391,
0.00885906951994799));
#46109=CARTESIAN_POINT('Ctrl Pts',(-0.192144790319268,0.00296657424698169,
0.00885489827767933));
#46110=CARTESIAN_POINT('Ctrl Pts',(-0.192136926370917,0.00298050245508833,
0.00885062267327234));
#46111=CARTESIAN_POINT('Ctrl Pts',(-0.192128608339638,0.00299808673321409,
0.00884076917177549));
#46112=CARTESIAN_POINT('Ctrl Pts',(-0.192126244627568,0.0030037842653694,
0.00883666173174214));
#46113=CARTESIAN_POINT('Ctrl Pts',(-0.192123326144348,0.0030129383334435,
0.00882759558586231));
#46114=CARTESIAN_POINT('Ctrl Pts',(-0.192122534580363,0.00301651956758922,
0.00882306590260883));
#46115=CARTESIAN_POINT('Ctrl Pts',(-0.192122335498293,0.00301948148814979,
0.00881802786499082));
#46116=CARTESIAN_POINT('Origin',(-0.194610820040351,0.00711537823747164,
0.00203978596199847));
#46117=CARTESIAN_POINT('Ctrl Pts',(-0.191053242553077,0.00360271141258139,
0.00908428820748653));
#46118=CARTESIAN_POINT('Ctrl Pts',(-0.191052569970049,0.00359318967230302,
0.00910573763815595));
#46119=CARTESIAN_POINT('Ctrl Pts',(-0.191043275012929,0.00357822482286264,
0.00913268910298602));
#46120=CARTESIAN_POINT('Ctrl Pts',(-0.191014962710414,0.00355712033360826,
0.00914835516048045));
#46121=CARTESIAN_POINT('Ctrl Pts',(-0.190999318265651,0.0035454586887731,
0.00915701170725896));
#46122=CARTESIAN_POINT('Ctrl Pts',(-0.190977649332568,0.00353243205832534,
0.00916064451185934));
#46123=CARTESIAN_POINT('Ctrl Pts',(-0.190954534254184,0.00352393167612197,
0.00915627380277794));
#46124=CARTESIAN_POINT('Ctrl Pts',(-0.190934183649427,0.0037372444874487,
0.00914086988152931));
#46125=CARTESIAN_POINT('Ctrl Pts',(-0.190932852889833,0.00369517829876202,
0.00923782622115866));
#46126=CARTESIAN_POINT('Ctrl Pts',(-0.190855734892733,0.00363259200256237,
0.00920313590394181));
#46127=CARTESIAN_POINT('Ctrl Pts',(-0.191122446529827,0.0035006976223372,
0.00904127409012918));
#46128=CARTESIAN_POINT('Ctrl Pts',(-0.191121414789953,0.00345576162697059,
0.00913680019546882));
#46129=CARTESIAN_POINT('Ctrl Pts',(-0.191033257028283,0.0034024260949739,
0.00910455083415403));
#46130=CARTESIAN_POINT('Ctrl Pts',(-0.191561608589598,0.00320278619904903,
0.00890344310116076));
#46131=CARTESIAN_POINT('Ctrl Pts',(-0.191561013525955,0.00315437706644305,
0.00899812271039178));
#46132=CARTESIAN_POINT('Ctrl Pts',(-0.191527722358912,0.00306053710433882,
0.00894344562862373));
#46133=CARTESIAN_POINT('Ctrl Pts',(-0.192148771194034,0.00301412826261319,
0.00881422045040244));
#46134=CARTESIAN_POINT('Ctrl Pts',(-0.192147303763206,0.00296401287835609,
0.00890776993720604));
#46135=CARTESIAN_POINT('Ctrl Pts',(-0.192106853669778,0.0028820556788135,
0.00885592463034678));
#46136=CARTESIAN_POINT('Ctrl Pts',(-0.192426303994506,0.00290954717981133,
0.00876152705466917));
#46137=CARTESIAN_POINT('Ctrl Pts',(-0.192425106237976,0.00285811942618207,
0.00885439357611185));
#46138=CARTESIAN_POINT('Ctrl Pts',(-0.192385551248651,0.00277512108865769,
0.00880072184303747));
#46139=CARTESIAN_POINT('Origin',(-0.22505940669331,0.00262788566134477,
-0.00925282722029539));
#46140=CARTESIAN_POINT('Ctrl Pts',(-0.225017273462258,0.00228350670705836,
-0.00900753387751742));
#46141=CARTESIAN_POINT('Ctrl Pts',(-0.225016618997253,0.00226753903385881,
-0.00902807321753408));
#46142=CARTESIAN_POINT('Ctrl Pts',(-0.224995064422474,0.00223443663122194,
-0.0090512478955521));
#46143=CARTESIAN_POINT('Ctrl Pts',(-0.224957173953608,0.00220011152757988,
-0.00905137780072061));
#46144=CARTESIAN_POINT('Ctrl Pts',(-0.224939696469926,0.00218427861611907,
-0.00905143772121066));
#46145=CARTESIAN_POINT('Ctrl Pts',(-0.224918567789863,0.00216920129523207,
-0.00904681991919557));
#46146=CARTESIAN_POINT('Ctrl Pts',(-0.224895681452505,0.00215874544783754,
-0.00903810107358197));
#46147=CARTESIAN_POINT('Ctrl Pts',(-0.225202513398594,0.00215390640396955,
-0.00904067530421461));
#46148=CARTESIAN_POINT('Ctrl Pts',(-0.225222962285849,0.0021853939560013,
-0.00906395019002407));
#46149=CARTESIAN_POINT('Ctrl Pts',(-0.225251193905704,0.00223630020952242,
-0.00907966627427055));
#46150=CARTESIAN_POINT('Ctrl Pts',(-0.225265203386337,0.00227752916182422,
-0.00907232786917598));
#46151=CARTESIAN_POINT('Ctrl Pts',(-0.22527246641627,0.0022989037668184,
-0.00906852337011824));
#46152=CARTESIAN_POINT('Ctrl Pts',(-0.225277058816433,0.00231715688114545,
-0.00905899968495788));
#46153=CARTESIAN_POINT('Ctrl Pts',(-0.225277037624834,0.00232818316358624,
-0.009044627616207));
#46154=CARTESIAN_POINT('Origin',(-0.226664408832371,0.00780583959346437,
-0.00183869293915824));
#46155=CARTESIAN_POINT('Ctrl Pts',(-0.225398032236364,0.00187965741570819,
-0.00870574455337625));
#46156=CARTESIAN_POINT('Ctrl Pts',(-0.225397670102207,0.00186284156270298,
-0.00872622281070892));
#46157=CARTESIAN_POINT('Ctrl Pts',(-0.225383677532918,0.00183056037380823,
-0.00874116199336752));
#46158=CARTESIAN_POINT('Ctrl Pts',(-0.225369807377174,0.00180549564236411,
-0.00874167732286142));
#46159=CARTESIAN_POINT('Ctrl Pts',(-0.225357067469305,0.00178247337965452,
-0.00874215065931098));
#46160=CARTESIAN_POINT('Ctrl Pts',(-0.225344270584155,0.00176631228172648,
-0.00873834609751508));
#46161=CARTESIAN_POINT('Ctrl Pts',(-0.225322589017758,0.00174427895566282,
-0.00872225830951696));
#46162=CARTESIAN_POINT('Ctrl Pts',(-0.225320665464812,0.0017423241951762,
-0.00872083102739873));
#46163=CARTESIAN_POINT('Ctrl Pts',(-0.225318672542542,0.00174034173716805,
-0.00871927766735267));
#46164=CARTESIAN_POINT('Ctrl Pts',(-0.225316604397166,0.0017383399119561,
-0.0087175758055758));
#46165=CARTESIAN_POINT('Origin',(-0.221413443561174,0.00402141110915759,
-0.00795211642683932));
#46166=CARTESIAN_POINT('Ctrl Pts',(-0.22512329647086,0.00302740120073959,
-0.0094920048930922));
#46167=CARTESIAN_POINT('Ctrl Pts',(-0.225122829997078,0.00301427597960748,
-0.00951459329922939));
#46168=CARTESIAN_POINT('Ctrl Pts',(-0.225112043106003,0.00299810554080808,
-0.00954228597437161));
#46169=CARTESIAN_POINT('Ctrl Pts',(-0.225080306438971,0.0029854217871898,
-0.00956043404639643));
#46170=CARTESIAN_POINT('Ctrl Pts',(-0.22506440406025,0.00297906630400566,
-0.00956952755057898));
#46171=CARTESIAN_POINT('Ctrl Pts',(-0.225043136430339,0.00297421075602464,
-0.00957511746433099));
#46172=CARTESIAN_POINT('Ctrl Pts',(-0.225021220651722,0.00297339553324741,
-0.00957419359245674));
#46173=CARTESIAN_POINT('Origin',(-0.225236920251344,0.00180210050578165,
-0.00863903021502896));
#46174=CARTESIAN_POINT('Ctrl Pts',(-0.22652065160046,0.00174023860749072,
-0.00874178828015322));
#46175=CARTESIAN_POINT('Ctrl Pts',(-0.226487204106126,0.00176069370205139,
-0.00875884229287255));
#46176=CARTESIAN_POINT('Ctrl Pts',(-0.226470246988884,0.00177636799853321,
-0.0087638065890931));
#46177=CARTESIAN_POINT('Ctrl Pts',(-0.226449412389476,0.00179560312689298,
-0.00876408887588995));
#46178=CARTESIAN_POINT('Ctrl Pts',(-0.226447161748294,0.00179768098647492,
-0.00876411936969872));
#46179=CARTESIAN_POINT('Ctrl Pts',(-0.226444880102038,0.00179983146927284,
-0.00876406231823839));
#46180=CARTESIAN_POINT('Ctrl Pts',(-0.226442559673134,0.00180208740374035,
-0.00876390573224407));
#46181=CARTESIAN_POINT('Ctrl Pts',(-0.226421164393966,0.00182288801850279,
-0.0087624619469782));
#46182=CARTESIAN_POINT('Ctrl Pts',(-0.226399628888184,0.00185516923677106,
-0.00875058152146249));
#46183=CARTESIAN_POINT('Ctrl Pts',(-0.226396806525128,0.00187493136781516,
-0.0087321638437343));
#46184=CARTESIAN_POINT('Ctrl Pts',(-0.226396489163485,0.00187715352784392,
-0.00873009286124872));
#46185=CARTESIAN_POINT('Ctrl Pts',(-0.226396357073774,0.00187919374951108,
-0.00872795259181485));
#46186=CARTESIAN_POINT('Ctrl Pts',(-0.226396396172104,0.00188100664625559,
-0.00872574966728709));
#46187=CARTESIAN_POINT('Ctrl Pts',(-0.225204446336403,0.0026266116901076,
-0.00924432147987809));
#46188=CARTESIAN_POINT('Ctrl Pts',(-0.225204186385791,0.00256699386850615,
-0.0093357214718889));
#46189=CARTESIAN_POINT('Ctrl Pts',(-0.225097536665866,0.00255469103811688,
-0.0093160140711595));
#46190=CARTESIAN_POINT('Ctrl Pts',(-0.224843954512892,0.0041869607368055,
-0.0102625319434793));
#46191=CARTESIAN_POINT('Ctrl Pts',(-0.224843308353265,0.00414600493747456,
-0.010366055089662));
#46192=CARTESIAN_POINT('Ctrl Pts',(-0.224732922386792,0.00414683281156139,
-0.010359908500413));
#46193=CARTESIAN_POINT('Ctrl Pts',(-0.224960782705356,0.00611227388836029,
-0.0107818802397));
#46194=CARTESIAN_POINT('Ctrl Pts',(-0.224959834766411,0.00609508919934752,
-0.0108921774109498));
#46195=CARTESIAN_POINT('Ctrl Pts',(-0.224851943717515,0.00610784388063427,
-0.0108832416000841));
#46196=CARTESIAN_POINT('Ctrl Pts',(-0.225134764212758,0.00797670854236963,
-0.0106811162212081));
#46197=CARTESIAN_POINT('Ctrl Pts',(-0.225133867458967,0.00798256516491125,
-0.0107900411429812));
#46198=CARTESIAN_POINT('Ctrl Pts',(-0.225025636845997,0.00799125572483553,
-0.0107791637264416));
#46199=CARTESIAN_POINT('Ctrl Pts',(-0.225092276670026,0.00750489649772228,
-0.01069488405633));
#46200=CARTESIAN_POINT('Ctrl Pts',(-0.225092128720339,0.00750490060436441,
-0.010701428529533));
#46201=CARTESIAN_POINT('Ctrl Pts',(-0.225091336119301,0.00750490447888119,
-0.010707942167662));
#46202=CARTESIAN_POINT('Ctrl Pts',(-0.225088394527797,0.00750491197011461,
-0.0107211259016258));
#46203=CARTESIAN_POINT('Ctrl Pts',(-0.225086170863583,0.00750491553257603,
-0.0107277427406404));
#46204=CARTESIAN_POINT('Ctrl Pts',(-0.225077921390693,0.00750492486451957,
-0.0107457902190495));
#46205=CARTESIAN_POINT('Ctrl Pts',(-0.225070348970769,0.00750492976174552,
-0.0107563581170778));
#46206=CARTESIAN_POINT('Ctrl Pts',(-0.225051612800588,0.00750493867065022,
-0.0107740510630533));
#46207=CARTESIAN_POINT('Ctrl Pts',(-0.225040622831016,0.00750494157171742,
-0.0107810095606538));
#46208=CARTESIAN_POINT('Ctrl Pts',(-0.225011480672544,0.00750496211207701,
-0.0107924079104823));
#46209=CARTESIAN_POINT('Ctrl Pts',(-0.224997203143753,0.00750484457550957,
-0.0107925677269123));
#46210=CARTESIAN_POINT('Ctrl Pts',(-0.22499236923333,0.00750532531593724,
-0.0107926204687227));
#46211=CARTESIAN_POINT('Ctrl Pts',(-0.224991813978919,0.00750541957447757,
-0.0107926197981443));
#46212=CARTESIAN_POINT('Ctrl Pts',(-0.224991176190761,0.00750565492711975,
-0.0107926161397585));
#46213=CARTESIAN_POINT('Ctrl Pts',(-0.224990994648027,0.00750575025996745,
-0.0107926144173287));
#46214=CARTESIAN_POINT('Ctrl Pts',(-0.224990699885213,0.00750599070999525,
-0.0107926109188229));
#46215=CARTESIAN_POINT('Origin',(-0.228248406260441,0.00774941156494066,
-0.00207700075378771));
#46216=CARTESIAN_POINT('Ctrl Pts',(-0.226399236752868,0.00218270468350247,
-0.00908497199103555));
#46217=CARTESIAN_POINT('Ctrl Pts',(-0.226365903759496,0.0022077025998989,
-0.0091023416857952));
#46218=CARTESIAN_POINT('Ctrl Pts',(-0.226347961427136,0.00222302783543612,
-0.00910602669584673));
#46219=CARTESIAN_POINT('Ctrl Pts',(-0.226329441624569,0.00224518588862393,
-0.00910807014497639));
#46220=CARTESIAN_POINT('Ctrl Pts',(-0.226327076128619,0.00224801609077578,
-0.00910833115049321));
#46221=CARTESIAN_POINT('Ctrl Pts',(-0.226324703650294,0.00225098073497979,
-0.00910850424177511));
#46222=CARTESIAN_POINT('Ctrl Pts',(-0.226322290680913,0.00225412156710692,
-0.00910855561276932));
#46223=CARTESIAN_POINT('Ctrl Pts',(-0.226303524544785,0.00227854843457011,
-0.0091089551350667));
#46224=CARTESIAN_POINT('Ctrl Pts',(-0.226281641731344,0.00231268229690328,
-0.00909758541846404));
#46225=CARTESIAN_POINT('Ctrl Pts',(-0.22627679619897,0.0023306356395595,
-0.0090785542339953));
#46226=CARTESIAN_POINT('Ctrl Pts',(-0.226276140780917,0.00233306405071963,
-0.00907598003142816));
#46227=CARTESIAN_POINT('Ctrl Pts',(-0.226275806586992,0.00233523498560651,
-0.00907334009471901));
#46228=CARTESIAN_POINT('Ctrl Pts',(-0.226275854855421,0.00233713586297991,
-0.0090706994431196));
#46229=CARTESIAN_POINT('Ctrl Pts',(-0.225133508843075,0.0070426021535604,
-0.0106822844475311));
#46230=CARTESIAN_POINT('Ctrl Pts',(-0.225132851123412,0.00703714641402199,
-0.0107876109477567));
#46231=CARTESIAN_POINT('Ctrl Pts',(-0.225027954928167,0.00702870940870006,
-0.0107808140229128));
#46232=CARTESIAN_POINT('Ctrl Pts',(-0.22505071331137,0.00795538372590099,
-0.0107280453401897));
#46233=CARTESIAN_POINT('Ctrl Pts',(-0.225050042044769,0.00796099163518786,
-0.0108339164285507));
#46234=CARTESIAN_POINT('Ctrl Pts',(-0.224945248577277,0.00794989075010101,
-0.0108283334006842));
#46235=CARTESIAN_POINT('Ctrl Pts',(-0.224891592789171,0.0098189938545337,
-0.0105337716279733));
#46236=CARTESIAN_POINT('Ctrl Pts',(-0.224890988885346,0.00984605488963252,
-0.0106374837459184));
#46237=CARTESIAN_POINT('Ctrl Pts',(-0.224785486085702,0.00984549125624428,
-0.0106327018871958));
#46238=CARTESIAN_POINT('Ctrl Pts',(-0.225018871785121,0.0115441087398936,
-0.00977372250019193));
#46239=CARTESIAN_POINT('Ctrl Pts',(-0.225018607206713,0.0115921107104299,
-0.0098682361745316));
#46240=CARTESIAN_POINT('Ctrl Pts',(-0.224913292664793,0.01159740002097,
-0.00985985852773063));
#46241=CARTESIAN_POINT('Ctrl Pts',(-0.225178663464904,0.0122963651375774,
-0.00929332951627353));
#46242=CARTESIAN_POINT('Ctrl Pts',(-0.225178596738866,0.0123530193226692,
-0.00938229566958859));
#46243=CARTESIAN_POINT('Ctrl Pts',(-0.225075076993298,0.0123667363075108,
-0.0093669049292091));
#46244=CARTESIAN_POINT('Ctrl Pts',(-0.22500367450264,0.0119594504746824,
-0.00961245894030661));
#46245=CARTESIAN_POINT('Ctrl Pts',(-0.225042476908726,0.0119588072618708,
-0.00961362081736056));
#46246=CARTESIAN_POINT('Ctrl Pts',(-0.225075686348922,0.0119457864636921,
-0.00959384445542012));
#46247=CARTESIAN_POINT('Ctrl Pts',(-0.225090894665548,0.011933491925558,
-0.00957280406153543));
#46248=CARTESIAN_POINT('Ctrl Pts',(-0.225101658275347,0.0119247905278699,
-0.00955791282831388));
#46249=CARTESIAN_POINT('Ctrl Pts',(-0.22510571623242,0.011916204305882,
-0.00954259735527654));
#46250=CARTESIAN_POINT('Ctrl Pts',(-0.225106005940227,0.0119082516245216,
-0.00952863752848153));
#46251=CARTESIAN_POINT('Origin',(-0.226795305644497,0.00512875096591446,
-0.0111302531463925));
#46252=CARTESIAN_POINT('Ctrl Pts',(-0.227126281596587,0.00216860077931266,
-0.00908887685446537));
#46253=CARTESIAN_POINT('Ctrl Pts',(-0.227103468837074,0.00219179982118522,
-0.00910550310580199));
#46254=CARTESIAN_POINT('Ctrl Pts',(-0.22709216978019,0.00220949873293601,
-0.00910753311530889));
#46255=CARTESIAN_POINT('Ctrl Pts',(-0.227080571285647,0.00222769884615225,
-0.00910656554082502));
#46256=CARTESIAN_POINT('Ctrl Pts',(-0.227078774217523,0.00223051876758185,
-0.0091064156250531));
#46257=CARTESIAN_POINT('Ctrl Pts',(-0.227076958950209,0.00223341391934925,
-0.00910611361219578));
#46258=CARTESIAN_POINT('Ctrl Pts',(-0.22707510700407,0.00223645998904377,
-0.00910561814509268));
#46259=CARTESIAN_POINT('Ctrl Pts',(-0.227061302369607,0.00225916576746203,
-0.00910192487232323));
#46260=CARTESIAN_POINT('Ctrl Pts',(-0.22705025226088,0.0022883868956522,
-0.00908773493242626));
#46261=CARTESIAN_POINT('Ctrl Pts',(-0.22705075587212,0.00230593082281523,
-0.00906364037858624));
#46262=CARTESIAN_POINT('Origin',(-0.220737639952009,0.0101645710188458,
-0.00705086064850374));
#46263=CARTESIAN_POINT('Ctrl Pts',(-0.224973343469933,0.0127081065850716,
-0.00901241391075122));
#46264=CARTESIAN_POINT('Ctrl Pts',(-0.224972867526866,0.0127230932238013,
-0.00903178146774925));
#46265=CARTESIAN_POINT('Ctrl Pts',(-0.224954069874002,0.0127463242050564,
-0.00905044998856422));
#46266=CARTESIAN_POINT('Ctrl Pts',(-0.224920022767307,0.0127792324768161,
-0.00905480033347338));
#46267=CARTESIAN_POINT('Ctrl Pts',(-0.224901830748141,0.0127968159947325,
-0.00905712480581916));
#46268=CARTESIAN_POINT('Ctrl Pts',(-0.224878894299268,0.0128172384444568,
-0.00905462517503522));
#46269=CARTESIAN_POINT('Ctrl Pts',(-0.22485135503735,0.0128342630404597,
-0.00904243198075601));
#46270=CARTESIAN_POINT('Ctrl Pts',(-0.227001241570868,0.00180642850357482,
-0.0088047000233499));
#46271=CARTESIAN_POINT('Ctrl Pts',(-0.226900506181097,0.00183019171535291,
-0.00882613840246201));
#46272=CARTESIAN_POINT('Ctrl Pts',(-0.226904412758277,0.00189655459570073,
-0.00874393346586029));
#46273=CARTESIAN_POINT('Ctrl Pts',(-0.227153448032914,0.0022110448391632,
-0.00914043886458957));
#46274=CARTESIAN_POINT('Ctrl Pts',(-0.227049842562979,0.00222790739901197,
-0.00915517224639843));
#46275=CARTESIAN_POINT('Ctrl Pts',(-0.227053893271391,0.00228956405612877,
-0.00906920714343653));
#46276=CARTESIAN_POINT('Ctrl Pts',(-0.227365349818599,0.00297531408401169,
-0.00966050279634506));
#46277=CARTESIAN_POINT('Ctrl Pts',(-0.227267539357192,0.00301108431445871,
-0.00968461017188333));
#46278=CARTESIAN_POINT('Ctrl Pts',(-0.227271547008689,0.00306306528267084,
-0.00959208981312559));
#46279=CARTESIAN_POINT('Ctrl Pts',(-0.228325656075677,0.00449820905690461,
-0.0104150080377229));
#46280=CARTESIAN_POINT('Ctrl Pts',(-0.228240062671686,0.00455763333783317,
-0.0104388268493249));
#46281=CARTESIAN_POINT('Ctrl Pts',(-0.22824408912365,0.00459088144197996,
-0.0103373670073668));
#46282=CARTESIAN_POINT('Ctrl Pts',(-0.229161619106937,0.00554785569106383,
-0.0107000249104784));
#46283=CARTESIAN_POINT('Ctrl Pts',(-0.229078979149685,0.00561257757990715,
-0.0107161200036778));
#46284=CARTESIAN_POINT('Ctrl Pts',(-0.229083451610345,0.00563384010371639,
-0.0106119667335707));
#46285=CARTESIAN_POINT('Ctrl Pts',(-0.229777994677051,0.00626685681131663,
-0.0108152446626343));
#46286=CARTESIAN_POINT('Ctrl Pts',(-0.229697325445588,0.00633494067670393,
-0.0108264360914299));
#46287=CARTESIAN_POINT('Ctrl Pts',(-0.22970183524063,0.00634769058836431,
-0.0107211605684957));
#46288=CARTESIAN_POINT('Ctrl Pts',(-0.229392048724075,0.00598507781155818,
-0.0106610739775155));
#46289=CARTESIAN_POINT('Ctrl Pts',(-0.229390542419233,0.00597321450034639,
-0.0107280577062599));
#46290=CARTESIAN_POINT('Ctrl Pts',(-0.229392105759804,0.00588226597872448,
-0.0107445713598933));
#46291=CARTESIAN_POINT('Ctrl Pts',(-0.229393975477449,0.00581660464796607,
-0.0107320544081558));
#46292=CARTESIAN_POINT('Origin',(-0.225014917424223,0.0121976159450981,
-0.00937785723393056));
#46293=CARTESIAN_POINT('Ctrl Pts',(-0.225267117543399,0.0126690414880847,
-0.00904616167166099));
#46294=CARTESIAN_POINT('Ctrl Pts',(-0.22526707803216,0.0126827612232737,
-0.00906407729233419));
#46295=CARTESIAN_POINT('Ctrl Pts',(-0.225249780251561,0.012753996211984,
-0.00910717479492578));
#46296=CARTESIAN_POINT('Ctrl Pts',(-0.225189992040237,0.012835362403236,
-0.00904829323284222));
#46297=CARTESIAN_POINT('Ctrl Pts',(-0.224396676139726,-0.00142332076525291,
0.00171535545036799));
#46298=CARTESIAN_POINT('Ctrl Pts',(-0.22440262397633,-0.00152767275903206,
0.0017228806849109));
#46299=CARTESIAN_POINT('Ctrl Pts',(-0.224301788788553,-0.00153188245866574,
0.00169183918866943));
#46300=CARTESIAN_POINT('Ctrl Pts',(-0.224886223773115,-0.00150538358571777,
0.000505008790366226));
#46301=CARTESIAN_POINT('Ctrl Pts',(-0.224888895735799,-0.00161018065377861,
0.000505692381198935));
#46302=CARTESIAN_POINT('Ctrl Pts',(-0.224791190497898,-0.00160705300214277,
0.000469981952361821));
#46303=CARTESIAN_POINT('Ctrl Pts',(-0.225312479549641,-0.00146449675102691,
-0.00113756146524579));
#46304=CARTESIAN_POINT('Ctrl Pts',(-0.225317589847797,-0.00156890719457313,
-0.00113693061187638));
#46305=CARTESIAN_POINT('Ctrl Pts',(-0.225215903592698,-0.00157050028691277,
-0.00116612020660587));
#46306=CARTESIAN_POINT('Ctrl Pts',(-0.226180826034794,-0.00134425411844392,
-0.00294330696628029));
#46307=CARTESIAN_POINT('Ctrl Pts',(-0.226184344417459,-0.00144865223190297,
-0.00295560123666401));
#46308=CARTESIAN_POINT('Ctrl Pts',(-0.226091759329284,-0.00144114023446119,
-0.00300491641135075));
#46309=CARTESIAN_POINT('Ctrl Pts',(-0.226933085082599,-0.00110947784190311,
-0.00418900462821542));
#46310=CARTESIAN_POINT('Ctrl Pts',(-0.226935809002347,-0.00121135843081841,
-0.00421601234379386));
#46311=CARTESIAN_POINT('Ctrl Pts',(-0.226849103899972,-0.00119375720027678,
-0.00427331043439446));
#46312=CARTESIAN_POINT('Ctrl Pts',(-0.227852338361138,-0.00071336136482749,
-0.0053200366555796));
#46313=CARTESIAN_POINT('Ctrl Pts',(-0.227854799933957,-0.000811012846727041,
-0.00535991228805838));
#46314=CARTESIAN_POINT('Ctrl Pts',(-0.227774403608196,-0.000782339329089386,
-0.00542196422418219));
#46315=CARTESIAN_POINT('Ctrl Pts',(-0.228870818459826,-0.000230238301254827,
-0.00627315584430081));
#46316=CARTESIAN_POINT('Ctrl Pts',(-0.228872528896894,-0.000322624060608064,
-0.0063238210346253));
#46317=CARTESIAN_POINT('Ctrl Pts',(-0.228798516093321,-0.000283020163498878,
-0.00638754543715099));
#46318=CARTESIAN_POINT('Ctrl Pts',(-0.229685021388832,0.00016983281225574,
-0.00692536606282476));
#46319=CARTESIAN_POINT('Ctrl Pts',(-0.229686436788066,8.18761831818451E-5,
-0.0069834750083683));
#46320=CARTESIAN_POINT('Ctrl Pts',(-0.229616247601761,0.000128826935045281,
-0.00704653030251611));
#46321=CARTESIAN_POINT('Ctrl Pts',(-0.230541713269828,0.000600161250818714,
-0.00751902719524027));
#46322=CARTESIAN_POINT('Ctrl Pts',(-0.230542692670766,0.000516956443363417,
-0.00758381901479241));
#46323=CARTESIAN_POINT('Ctrl Pts',(-0.230474718780796,0.000570314407031533,
-0.00764432333491235));
#46324=CARTESIAN_POINT('Ctrl Pts',(-0.231240730721998,0.00101586856032313,
-0.00800875883378466));
#46325=CARTESIAN_POINT('Ctrl Pts',(-0.231241596006655,0.000937600164170982,
-0.00807926470697491));
#46326=CARTESIAN_POINT('Ctrl Pts',(-0.231167251978618,0.000991127187817129,
-0.00813130972012129));
#46327=CARTESIAN_POINT('Ctrl Pts',(-0.231746311087107,0.00141861438610773,
-0.00842042128462309));
#46328=CARTESIAN_POINT('Ctrl Pts',(-0.231747138074993,0.00134534692439856,
-0.00849585660741608));
#46329=CARTESIAN_POINT('Ctrl Pts',(-0.231664594865682,0.00139585162906457,
-0.0085381855415369));
#46330=CARTESIAN_POINT('Ctrl Pts',(-0.232056074667116,0.00178920573458372,
-0.00876109936472852));
#46331=CARTESIAN_POINT('Ctrl Pts',(-0.232056921580141,0.00172079157747844,
-0.00884057353990152));
#46332=CARTESIAN_POINT('Ctrl Pts',(-0.231958886560654,0.00175583914593751,
-0.00886433751250737));
#46333=CARTESIAN_POINT('Ctrl Pts',(-0.232193077929066,0.0022593348110294,
-0.00913722136145496));
#46334=CARTESIAN_POINT('Ctrl Pts',(-0.232193895416839,0.00219728065587455,
-0.00922146917010263));
#46335=CARTESIAN_POINT('Ctrl Pts',(-0.232086297599378,0.00220194228853664,
-0.00921877403283003));
#46336=CARTESIAN_POINT('Ctrl Pts',(-0.232069159882949,0.00275709221639288,
-0.00947418078662092));
#46337=CARTESIAN_POINT('Ctrl Pts',(-0.232069760611005,0.00270143516070841,
-0.00956299654933791));
#46338=CARTESIAN_POINT('Ctrl Pts',(-0.231971241371772,0.00267077028039009,
-0.00953798268856777));
#46339=CARTESIAN_POINT('Ctrl Pts',(-0.231817071059768,0.00320367822680323,
-0.009733687825506));
#46340=CARTESIAN_POINT('Ctrl Pts',(-0.23181751007782,0.00315337366854661,
-0.00982578095251141));
#46341=CARTESIAN_POINT('Ctrl Pts',(-0.231726075148213,0.00311073478768687,
-0.00979708818873018));
#46342=CARTESIAN_POINT('Ctrl Pts',(-0.231406108401932,0.0037813454740335,
-0.0100253031754078));
#46343=CARTESIAN_POINT('Ctrl Pts',(-0.231406285019437,0.00373820127523732,
-0.0101212130320277));
#46344=CARTESIAN_POINT('Ctrl Pts',(-0.231322534976874,0.00368204180968578,
-0.0100900101324168));
#46345=CARTESIAN_POINT('Ctrl Pts',(-0.230820435181291,0.00445368016899616,
-0.0102948098424759));
#46346=CARTESIAN_POINT('Ctrl Pts',(-0.230820492564017,0.00441870338655471,
-0.0103941115079675));
#46347=CARTESIAN_POINT('Ctrl Pts',(-0.230741020352473,0.00435575367357216,
-0.0103663664226606));
#46348=CARTESIAN_POINT('Ctrl Pts',(-0.229705029163254,0.00565307708557098,
-0.0106446791912509));
#46349=CARTESIAN_POINT('Ctrl Pts',(-0.229704860572995,0.00563255866281126,
-0.0107483485835331));
#46350=CARTESIAN_POINT('Ctrl Pts',(-0.229628571771374,0.00556235013793471,
-0.0107286444532703));
#46351=CARTESIAN_POINT('Ctrl Pts',(-0.22880521178587,0.00660766312397794,
-0.0107567659866438));
#46352=CARTESIAN_POINT('Ctrl Pts',(-0.228805149664529,0.00659816138019425,
-0.0108617688099226));
#46353=CARTESIAN_POINT('Ctrl Pts',(-0.228727395906984,0.00652825978395869,
-0.0108504227547395));
#46354=CARTESIAN_POINT('Ctrl Pts',(-0.228204402529689,0.00728967204301217,
-0.0107607843627637));
#46355=CARTESIAN_POINT('Ctrl Pts',(-0.228204231002405,0.00728845450009763,
-0.0108659909308064));
#46356=CARTESIAN_POINT('Ctrl Pts',(-0.228126736912477,0.00721732932302992,
-0.0108591494756485));
#46357=CARTESIAN_POINT('Ctrl Pts',(-0.225010408220381,-0.001474251923458,
-8.66933507069693E-8));
#46358=CARTESIAN_POINT('Ctrl Pts',(-0.225010513130272,-0.00148096461986653,
-8.60291771540735E-8));
#46359=CARTESIAN_POINT('Ctrl Pts',(-0.2250099051443,-0.00148766394680708,
-8.63326333322152E-8));
#46360=CARTESIAN_POINT('Ctrl Pts',(-0.225007201134807,-0.00150128853343724,
-8.88873034778271E-8));
#46361=CARTESIAN_POINT('Ctrl Pts',(-0.225005016374328,-0.00150814265758981,
-9.12616443811379E-8));
#46362=CARTESIAN_POINT('Ctrl Pts',(-0.224996743541649,-0.0015267190689707,
-1.00688159401524E-7));
#46363=CARTESIAN_POINT('Ctrl Pts',(-0.224989020434532,-0.00153751939434098,
-1.09921160579431E-7));
#46364=CARTESIAN_POINT('Ctrl Pts',(-0.224969774277744,-0.00155577474558815,
-1.32360595393897E-7));
#46365=CARTESIAN_POINT('Ctrl Pts',(-0.224958379470597,-0.00156301015807106,
-1.46031598591108E-7));
#46366=CARTESIAN_POINT('Ctrl Pts',(-0.224932296005058,-0.00157349211018854,
-1.68872337400542E-7));
#46367=CARTESIAN_POINT('Ctrl Pts',(-0.224920543955411,-0.00157502458955791,
-2.06100960647531E-7));
#46368=CARTESIAN_POINT('Ctrl Pts',(-0.224912805021654,-0.00157563989864377,
-1.09230025696975E-7));
#46369=CARTESIAN_POINT('Ctrl Pts',(-0.22491012475841,-0.00157582454580539,
-1.61765696956859E-7));
#46370=CARTESIAN_POINT('Ctrl Pts',(-0.224907438932167,-0.00157589361967845,
-2.25179927914984E-7));
#46371=CARTESIAN_POINT('Ctrl Pts',(-0.22490660358187,-0.00157590691521979,
-2.26286434986113E-7));
#46372=CARTESIAN_POINT('Origin',(-0.226660317458695,0.00720499143128829,
-0.00184762445713072));
#46373=CARTESIAN_POINT('Ctrl Pts',(-0.225309820211856,0.0132780515765434,
-0.00870378491731464));
#46374=CARTESIAN_POINT('Ctrl Pts',(-0.225310270518267,0.0132776177035617,
-0.00870415552087384));
#46375=CARTESIAN_POINT('Ctrl Pts',(-0.225311023382707,0.0132779301043826,
-0.00870389963108353));
#46376=CARTESIAN_POINT('Ctrl Pts',(-0.225311232192588,0.0132772106330284,
-0.00870449657790214));
#46377=CARTESIAN_POINT('Ctrl Pts',(-0.225311553950656,0.0132767496254951,
-0.00870488159341767));
#46378=CARTESIAN_POINT('Ctrl Pts',(-0.225312613380327,0.0132755573730371,
-0.0087058439119948));
#46379=CARTESIAN_POINT('Ctrl Pts',(-0.225313051364385,0.013275092055929,
-0.00870621364083127));
#46380=CARTESIAN_POINT('Ctrl Pts',(-0.225314209362679,0.0132738730043072,
-0.00870716690654188));
#46381=CARTESIAN_POINT('Ctrl Pts',(-0.225315037951984,0.0132730168765924,
-0.00870781670795182));
#46382=CARTESIAN_POINT('Ctrl Pts',(-0.225317483670858,0.0132704706091192,
-0.00870968427436419));
#46383=CARTESIAN_POINT('Ctrl Pts',(-0.225319113893644,0.0132687539642296,
-0.00871086506368553));
#46384=CARTESIAN_POINT('Ctrl Pts',(-0.225323972395015,0.0132635216454238,
-0.00871422988017993));
#46385=CARTESIAN_POINT('Ctrl Pts',(-0.225327194760367,0.0132599069287703,
-0.00871625565991771));
#46386=CARTESIAN_POINT('Ctrl Pts',(-0.225342320259782,0.0132421739271964,
-0.00872479923956172));
#46387=CARTESIAN_POINT('Ctrl Pts',(-0.225353424218474,0.0132268946822168,
-0.00872819403241251));
#46388=CARTESIAN_POINT('Ctrl Pts',(-0.225370281092151,0.0131993265799017,
-0.00872784051699747));
#46389=CARTESIAN_POINT('Ctrl Pts',(-0.22537689223205,0.0131867227470534,
-0.00872543917842188));
#46390=CARTESIAN_POINT('Ctrl Pts',(-0.225385934802891,0.0131647319127703,
-0.00871617296164978));
#46391=CARTESIAN_POINT('Ctrl Pts',(-0.225388851873419,0.013155420922425,
-0.00871039322749511));
#46392=CARTESIAN_POINT('Ctrl Pts',(-0.225390991697131,0.0131433715023081,
-0.0086996018357167));
#46393=CARTESIAN_POINT('Ctrl Pts',(-0.225391353704068,0.0131399272886964,
-0.00869601173353095));
#46394=CARTESIAN_POINT('Ctrl Pts',(-0.225391419217255,0.0131367695105258,
-0.0086921820518181));
#46395=CARTESIAN_POINT('Ctrl Pts',(-0.228163515612994,0.00733515508811961,
0.0107625774342653));
#46396=CARTESIAN_POINT('Ctrl Pts',(-0.228163459199396,0.00733469307617318,
0.0108687650146076));
#46397=CARTESIAN_POINT('Ctrl Pts',(-0.228085015691996,0.0072631586172991,
0.0108613593351734));
#46398=CARTESIAN_POINT('Ctrl Pts',(-0.228743649451567,0.00665278436300879,
0.0107581182094424));
#46399=CARTESIAN_POINT('Ctrl Pts',(-0.228743828274746,0.00664383782840776,
0.0108640874686174));
#46400=CARTESIAN_POINT('Ctrl Pts',(-0.228664959938252,0.00657387845985657,
0.0108524569587656));
#46401=CARTESIAN_POINT('Ctrl Pts',(-0.22963210211456,0.00571569401386139,
0.0106555484427694));
#46402=CARTESIAN_POINT('Ctrl Pts',(-0.229632061465273,0.00569595006967033,
0.0107603333381804));
#46403=CARTESIAN_POINT('Ctrl Pts',(-0.22955520323395,0.00562499939819525,
0.0107401577457921));
#46404=CARTESIAN_POINT('Ctrl Pts',(-0.230724245638906,0.00451099638068745,
0.0103135525699589));
#46405=CARTESIAN_POINT('Ctrl Pts',(-0.230724478352774,0.00447655937784655,
0.010414023536827));
#46406=CARTESIAN_POINT('Ctrl Pts',(-0.230643166808046,0.00441441049208174,
0.0103862385728284));
#46407=CARTESIAN_POINT('Ctrl Pts',(-0.231293450457664,0.0038259590991092,
0.0100434420479585));
#46408=CARTESIAN_POINT('Ctrl Pts',(-0.231293848628935,0.00378306605575638,
0.0101404566930396));
#46409=CARTESIAN_POINT('Ctrl Pts',(-0.23120738031312,0.00372893782348863,
0.0101097087117905));
#46410=CARTESIAN_POINT('Ctrl Pts',(-0.231667282960074,0.00323956433154689,
0.00975046297908365));
#46411=CARTESIAN_POINT('Ctrl Pts',(-0.231667951722417,0.00318932082472952,
0.00984359953359723));
#46412=CARTESIAN_POINT('Ctrl Pts',(-0.23157290806973,0.00315106112455292,
0.0098166551560102));
#46413=CARTESIAN_POINT('Ctrl Pts',(-0.231878171710574,0.00277621374154605,
0.00948262239106185));
#46414=CARTESIAN_POINT('Ctrl Pts',(-0.231879062889777,0.00272020523476094,
0.00957221388849241));
#46415=CARTESIAN_POINT('Ctrl Pts',(-0.231775237663013,0.00269967656492334,
0.0095526871407656));
#46416=CARTESIAN_POINT('Ctrl Pts',(-0.231911081200316,0.0022771945351161,
0.00914372039368585));
#46417=CARTESIAN_POINT('Ctrl Pts',(-0.231912143168076,0.00221451729150512,
0.00922872354247918));
#46418=CARTESIAN_POINT('Ctrl Pts',(-0.23180532211203,0.00223182547592494,
0.0092344894905382));
#46419=CARTESIAN_POINT('Ctrl Pts',(-0.231724190086194,0.00183722198742645,
0.00879379616530824));
#46420=CARTESIAN_POINT('Ctrl Pts',(-0.231725223949959,0.00176861677599736,
0.0088744276874275));
#46421=CARTESIAN_POINT('Ctrl Pts',(-0.231629985856898,0.00180875294582294,
0.00890135004891185));
#46422=CARTESIAN_POINT('Ctrl Pts',(-0.231408286783581,0.00147669052636452,
0.00846836905126042));
#46423=CARTESIAN_POINT('Ctrl Pts',(-0.231409336524876,0.00140344626307841,
0.00854510935254151));
#46424=CARTESIAN_POINT('Ctrl Pts',(-0.231325538660294,0.00145450447662584,
0.00858614430807182));
#46425=CARTESIAN_POINT('Ctrl Pts',(-0.230925990974879,0.0010718808526038,
0.00806298588782171));
#46426=CARTESIAN_POINT('Ctrl Pts',(-0.230927069716664,0.000993566663471985,
0.00813479332567291));
#46427=CARTESIAN_POINT('Ctrl Pts',(-0.230849955200748,0.00104704858832882,
0.0081846698003006));
#46428=CARTESIAN_POINT('Ctrl Pts',(-0.230261991331419,0.000642679936980595,
0.00756775583408155));
#46429=CARTESIAN_POINT('Ctrl Pts',(-0.230263231713554,0.000559265972955093,
0.0076337316989568));
#46430=CARTESIAN_POINT('Ctrl Pts',(-0.230191098868531,0.000612031842833926,
0.00769135709643061));
#46431=CARTESIAN_POINT('Ctrl Pts',(-0.22919233226498,4.57818412561549E-5,
0.0067574639823101));
#46432=CARTESIAN_POINT('Ctrl Pts',(-0.229194129960548,-4.4281278233945E-5,
0.00681420798335808));
#46433=CARTESIAN_POINT('Ctrl Pts',(-0.229119133350779,1.08743265013897E-8,
0.00687532298388693));
#46434=CARTESIAN_POINT('Ctrl Pts',(-0.227932685841537,-0.000625271979417362,
0.00557903136162669));
#46435=CARTESIAN_POINT('Ctrl Pts',(-0.227935460994856,-0.000722688106822415,
0.00562244279410726));
#46436=CARTESIAN_POINT('Ctrl Pts',(-0.227852889082099,-0.000692019389878893,
0.00568252489260457));
#46437=CARTESIAN_POINT('Ctrl Pts',(-0.226870498362358,-0.00111144671474683,
0.00418396327020359));
#46438=CARTESIAN_POINT('Ctrl Pts',(-0.226873447749571,-0.00121426192939155,
0.00421110560023027));
#46439=CARTESIAN_POINT('Ctrl Pts',(-0.226784623034336,-0.00119640615038005,
0.00426665238329828));
#46440=CARTESIAN_POINT('Ctrl Pts',(-0.226141786432928,-0.00134786885158213,
0.00291774568293432));
#46441=CARTESIAN_POINT('Ctrl Pts',(-0.226145556131887,-0.00145321997732708,
0.0029296788274651));
#46442=CARTESIAN_POINT('Ctrl Pts',(-0.226051217691109,-0.00144536866999242,
0.00297752009225177));
#46443=CARTESIAN_POINT('Ctrl Pts',(-0.225309314238018,-0.00146331986333167,
0.00111118276018021));
#46444=CARTESIAN_POINT('Ctrl Pts',(-0.225314574440745,-0.00156865189798677,
0.00111063356664893));
#46445=CARTESIAN_POINT('Ctrl Pts',(-0.225212189039601,-0.00156924905290015,
0.00113991809877219));
#46446=CARTESIAN_POINT('Ctrl Pts',(-0.224886529385567,-0.0015053586236984,
-0.00049391139130483));
#46447=CARTESIAN_POINT('Ctrl Pts',(-0.224889615321908,-0.00161108241616776,
-0.00049465971725397));
#46448=CARTESIAN_POINT('Ctrl Pts',(-0.224790799753559,-0.00160751596957962,
-0.000458880758028573));
#46449=CARTESIAN_POINT('Ctrl Pts',(-0.224413778106133,-0.0014231156766575,
-0.00169196883250104));
#46450=CARTESIAN_POINT('Ctrl Pts',(-0.224419774485945,-0.00152837716757349,
-0.0016996429168911));
#46451=CARTESIAN_POINT('Ctrl Pts',(-0.224318111707952,-0.00153157542826408,
-0.00166863240918668));
#46452=CARTESIAN_POINT('Ctrl Pts',(-0.229322728421253,0.00603936961279809,
0.0106687798113575));
#46453=CARTESIAN_POINT('Ctrl Pts',(-0.229321217780042,0.0060278782329308,
0.0107359585066643));
#46454=CARTESIAN_POINT('Ctrl Pts',(-0.229322620684285,0.00593681079674449,
0.0107528602121019));
#46455=CARTESIAN_POINT('Ctrl Pts',(-0.229324382301549,0.00587096534799219,
0.0107407249786847));
#46456=CARTESIAN_POINT('Origin',(-0.226555118506608,0.0132132840185884,
-0.00865094685306489));
#46457=CARTESIAN_POINT('Ctrl Pts',(-0.226391100214881,0.0131362729098227,
-0.00871148492904484));
#46458=CARTESIAN_POINT('Ctrl Pts',(-0.22639099939902,0.0131408916001344,
-0.00871707599316609));
#46459=CARTESIAN_POINT('Ctrl Pts',(-0.226391877522066,0.0131460464250971,
-0.00872209676525605));
#46460=CARTESIAN_POINT('Ctrl Pts',(-0.226396241089665,0.0131597801495802,
-0.00873297084794114));
#46461=CARTESIAN_POINT('Ctrl Pts',(-0.226400631403011,0.0131684509980104,
-0.00873781356047663));
#46462=CARTESIAN_POINT('Ctrl Pts',(-0.22641373138063,0.0131891685691253,
-0.00874613941805954));
#46463=CARTESIAN_POINT('Ctrl Pts',(-0.226424048697701,0.0132020838590036,
-0.00874865540428968));
#46464=CARTESIAN_POINT('Ctrl Pts',(-0.226454171535271,0.0132336318450819,
-0.00874868449941933));
#46465=CARTESIAN_POINT('Ctrl Pts',(-0.226475314459197,0.0132515451103633,
-0.00874360856911665));
#46466=CARTESIAN_POINT('Ctrl Pts',(-0.226504389347222,0.0132715457543843,
-0.00873146777518632));
#46467=CARTESIAN_POINT('Ctrl Pts',(-0.226509609320238,0.013274891856478,
-0.00872888455161681));
#46468=CARTESIAN_POINT('Ctrl Pts',(-0.226512544837996,0.0132762772382622,
-0.00872782692749136));
#46469=CARTESIAN_POINT('Ctrl Pts',(-0.226512607671518,0.0132767688794727,
-0.00872741805619649));
#46470=CARTESIAN_POINT('Ctrl Pts',(-0.226513565707048,0.0132773985794685,
-0.0087269091281644));
#46471=CARTESIAN_POINT('Ctrl Pts',(-0.22691449864251,0.00188912409957078,
0.00874101187538417));
#46472=CARTESIAN_POINT('Ctrl Pts',(-0.226912882541645,0.00182380187236744,
0.00882075610471368));
#46473=CARTESIAN_POINT('Ctrl Pts',(-0.227011968494547,0.00180258160872482,
0.00880179656685173));
#46474=CARTESIAN_POINT('Ctrl Pts',(-0.227052876055634,0.00228681646168442,
0.00907019845969648));
#46475=CARTESIAN_POINT('Ctrl Pts',(-0.227051157818039,0.00222625156923484,
0.00915378807385768));
#46476=CARTESIAN_POINT('Ctrl Pts',(-0.227152592109862,0.00221147656246655,
0.00914106091400232));
#46477=CARTESIAN_POINT('Ctrl Pts',(-0.227243827191478,0.00306830791249711,
0.00959853048103973));
#46478=CARTESIAN_POINT('Ctrl Pts',(-0.227242027555894,0.00301688618314614,
0.0096883671492618));
#46479=CARTESIAN_POINT('Ctrl Pts',(-0.227338827573701,0.00298480159953571,
0.0096668734289546));
#46480=CARTESIAN_POINT('Ctrl Pts',(-0.228154605500681,0.00459990079405723,
0.0103395772456444));
#46481=CARTESIAN_POINT('Ctrl Pts',(-0.228152531261446,0.00456632614965043,
0.0104381318959621));
#46482=CARTESIAN_POINT('Ctrl Pts',(-0.228237400064536,0.00450986270607348,
0.0104157331075302));
#46483=CARTESIAN_POINT('Ctrl Pts',(-0.228964082156122,0.00562823913086061,
0.0106085667885485));
#46484=CARTESIAN_POINT('Ctrl Pts',(-0.228961542575069,0.00560606514916299,
0.0107098744596661));
#46485=CARTESIAN_POINT('Ctrl Pts',(-0.229042444109394,0.00554326214965241,
0.0106944729792509));
#46486=CARTESIAN_POINT('Ctrl Pts',(-0.229559203666659,0.00631640552755159,
0.0107158903392713));
#46487=CARTESIAN_POINT('Ctrl Pts',(-0.229556533468569,0.00630212175177429,
0.0108183699092633));
#46488=CARTESIAN_POINT('Ctrl Pts',(-0.229635305092869,0.00623583857093286,
0.0108075661196736));
#46489=CARTESIAN_POINT('Ctrl Pts',(-0.227048969078908,0.00230603179210533,
0.00906366400351058));
#46490=CARTESIAN_POINT('Ctrl Pts',(-0.227048487225699,0.00228917960945197,
0.00908680953759018));
#46491=CARTESIAN_POINT('Ctrl Pts',(-0.22705976561457,0.00225915926815955,
0.00910191473859165));
#46492=CARTESIAN_POINT('Ctrl Pts',(-0.227074094125804,0.00223632626390423,
0.00910567066208655));
#46493=CARTESIAN_POINT('Ctrl Pts',(-0.227086502500316,0.00221655306741396,
0.00910892326136944));
#46494=CARTESIAN_POINT('Ctrl Pts',(-0.227096119022736,0.00220123369184519,
0.00910711704019592));
#46495=CARTESIAN_POINT('Ctrl Pts',(-0.227116358685445,0.00217914689185743,
0.00909540149177823));
#46496=CARTESIAN_POINT('Ctrl Pts',(-0.227119490693188,0.00217572904692728,
0.00909358855700337));
#46497=CARTESIAN_POINT('Ctrl Pts',(-0.227122863556042,0.00217221506441309,
0.00909145502818572));
#46498=CARTESIAN_POINT('Ctrl Pts',(-0.227126457702988,0.00216864736443003,
0.00908889965119285));
#46499=CARTESIAN_POINT('Origin',(-0.2278013545925,0.0072019569842425,-0.00186521002294653));
#46500=CARTESIAN_POINT('Ctrl Pts',(-0.22626372473152,0.0126609453232516,
-0.00907137440433446));
#46501=CARTESIAN_POINT('Ctrl Pts',(-0.226263573629508,0.0126654614507829,
-0.00907770987697118));
#46502=CARTESIAN_POINT('Ctrl Pts',(-0.226264580331983,0.0126707561268844,
-0.00908325776756278));
#46503=CARTESIAN_POINT('Ctrl Pts',(-0.226269247059774,0.0126845083276505,
-0.00909440199537926));
#46504=CARTESIAN_POINT('Ctrl Pts',(-0.226273586565231,0.0126930823229516,
-0.00909907503057873));
#46505=CARTESIAN_POINT('Ctrl Pts',(-0.226286568425147,0.0127144805599102,
-0.00910735204035213));
#46506=CARTESIAN_POINT('Ctrl Pts',(-0.226297082359114,0.0127286147065889,
-0.0091097655807238));
#46507=CARTESIAN_POINT('Ctrl Pts',(-0.226334765361614,0.0127720987460258,
-0.00910910869015226));
#46508=CARTESIAN_POINT('Ctrl Pts',(-0.226362067829375,0.012795480515493,
-0.00909854469517186));
#46509=CARTESIAN_POINT('Ctrl Pts',(-0.226381826363649,0.0128112801451954,
-0.00908888771940711));
#46510=CARTESIAN_POINT('Ctrl Pts',(-0.22638412128973,0.0128130883201525,
-0.00908769467773142));
#46511=CARTESIAN_POINT('Ctrl Pts',(-0.226385866678303,0.0128146615116663,
-0.00908662433726843));
#46512=CARTESIAN_POINT('Ctrl Pts',(-0.226386262576521,0.0128150458650998,
-0.00908635898063884));
#46513=CARTESIAN_POINT('Ctrl Pts',(-0.226386768472206,0.0128156694119735,
-0.00908592114511766));
#46514=CARTESIAN_POINT('Ctrl Pts',(-0.22638699037668,0.0128161318494855,
-0.00908558925922971));
#46515=CARTESIAN_POINT('Origin',(-0.226785760559816,0.00535801911423735,
0.0112988545290219));
#46516=CARTESIAN_POINT('Ctrl Pts',(-0.226387677522943,0.00218135007292164,
0.00908374645919642));
#46517=CARTESIAN_POINT('Ctrl Pts',(-0.226387517829732,0.00218169450496916,
0.00908399406881082));
#46518=CARTESIAN_POINT('Ctrl Pts',(-0.226387348413078,0.00218193204633596,
0.00908416247407508));
#46519=CARTESIAN_POINT('Ctrl Pts',(-0.226386693227517,0.00218265984835474,
0.00908467088690384));
#46520=CARTESIAN_POINT('Ctrl Pts',(-0.2263860557642,0.00218323697421753,
0.00908506930642161));
#46521=CARTESIAN_POINT('Ctrl Pts',(-0.226381957964186,0.00218662050727849,
0.00908732217272258));
#46522=CARTESIAN_POINT('Ctrl Pts',(-0.226374795136826,0.00219209340473146,
0.00909086571165971));
#46523=CARTESIAN_POINT('Ctrl Pts',(-0.226342638124601,0.00221913347866911,
0.00910384797271027));
#46524=CARTESIAN_POINT('Ctrl Pts',(-0.226321383091947,0.00224036162316775,
0.00910819378426068));
#46525=CARTESIAN_POINT('Ctrl Pts',(-0.226293023697157,0.00227450048798041,
0.00910644145231066));
#46526=CARTESIAN_POINT('Ctrl Pts',(-0.226283795653164,0.00228749349753115,
0.00910340025700874));
#46527=CARTESIAN_POINT('Ctrl Pts',(-0.226272433519139,0.00230732054682446,
0.00909450550810068));
#46528=CARTESIAN_POINT('Ctrl Pts',(-0.226268703397229,0.00231530414933038,
0.00908960317565377));
#46529=CARTESIAN_POINT('Ctrl Pts',(-0.226265146545548,0.00232737965992297,
0.00907890647267523));
#46530=CARTESIAN_POINT('Ctrl Pts',(-0.226264467950038,0.00233171333312063,
0.00907412667988085));
#46531=CARTESIAN_POINT('Ctrl Pts',(-0.226264593786723,0.00233548626079879,
0.00906884045917144));
#46532=CARTESIAN_POINT('Origin',(-0.226777858818941,0.00989529916463247,
-0.0111105690553547));
#46533=CARTESIAN_POINT('Ctrl Pts',(-0.227006489040078,0.0126931492004507,
-0.00906333669283264));
#46534=CARTESIAN_POINT('Ctrl Pts',(-0.227006359658267,0.0126975068624466,
-0.00906933365124984));
#46535=CARTESIAN_POINT('Ctrl Pts',(-0.227006857270868,0.0127024672528347,
-0.00907482462423548));
#46536=CARTESIAN_POINT('Ctrl Pts',(-0.227009147112344,0.0127138818625653,
-0.00908508685135224));
#46537=CARTESIAN_POINT('Ctrl Pts',(-0.227011034309181,0.0127203292004405,
-0.00908965220311262));
#46538=CARTESIAN_POINT('Ctrl Pts',(-0.227017721423457,0.0127385730039939,
-0.00909978676830201));
#46539=CARTESIAN_POINT('Ctrl Pts',(-0.22702353660833,0.0127506850584017,
-0.0091036725767193));
#46540=CARTESIAN_POINT('Ctrl Pts',(-0.227037909708246,0.0127758982765603,
-0.00910714103478806));
#46541=CARTESIAN_POINT('Ctrl Pts',(-0.227046637460994,0.0127888529052407,
-0.00910619248230766));
#46542=CARTESIAN_POINT('Ctrl Pts',(-0.227064691972426,0.0128122260649919,
-0.00909983643384995));
#46543=CARTESIAN_POINT('Ctrl Pts',(-0.227072059174435,0.0128202275894214,
-0.00909532632992795));
#46544=CARTESIAN_POINT('Ctrl Pts',(-0.22707636600345,0.0128249181393595,
-0.00909243574350203));
#46545=CARTESIAN_POINT('Ctrl Pts',(-0.227078486743332,0.0128270744437461,
-0.00909109745054717));
#46546=CARTESIAN_POINT('Ctrl Pts',(-0.227080622192005,0.0128291400139368,
-0.0090896437656076));
#46547=CARTESIAN_POINT('Ctrl Pts',(-0.227081057780342,0.0128295770214247,
-0.00908933084235787));
#46548=CARTESIAN_POINT('Origin',(-0.227796834054845,0.00779833113437804,
0.001863412373519));
#46549=CARTESIAN_POINT('Ctrl Pts',(-0.226391079628494,0.00186369918642903,
0.00871144032132472));
#46550=CARTESIAN_POINT('Ctrl Pts',(-0.226390978660276,0.00185907532151077,
0.00871703755041187));
#46551=CARTESIAN_POINT('Ctrl Pts',(-0.226391858808544,0.00185391430762597,
0.00872206300839274));
#46552=CARTESIAN_POINT('Ctrl Pts',(-0.226396229435358,0.00184017066974772,
0.00873293975251571));
#46553=CARTESIAN_POINT('Ctrl Pts',(-0.226400623541884,0.00183149690541248,
0.00873778102458434));
#46554=CARTESIAN_POINT('Ctrl Pts',(-0.22641373311484,0.00181077232703316,
0.00874610285334654));
#46555=CARTESIAN_POINT('Ctrl Pts',(-0.226424057461933,0.0017978525598305,
0.00874861517548048));
#46556=CARTESIAN_POINT('Ctrl Pts',(-0.226454202151599,0.00176629171031552,
0.00874863186234132));
#46557=CARTESIAN_POINT('Ctrl Pts',(-0.226475356568348,0.00174837615164434,
0.00874354332882413));
#46558=CARTESIAN_POINT('Ctrl Pts',(-0.226504398614371,0.00172840715421356,
0.00873140694530539));
#46559=CARTESIAN_POINT('Ctrl Pts',(-0.226509593825756,0.00172507720736087,
0.00872883644315529));
#46560=CARTESIAN_POINT('Ctrl Pts',(-0.226512524128562,0.0017236946270086,
0.00872778095183921));
#46561=CARTESIAN_POINT('Ctrl Pts',(-0.226512586716719,0.00172320269411854,
0.00872737181745011));
#46562=CARTESIAN_POINT('Ctrl Pts',(-0.226513544924145,0.00172257286242674,
0.00872686276718726));
#46563=CARTESIAN_POINT('Ctrl Pts',(-0.226844203584844,0.0131107712181138,
-0.00873939524392954));
#46564=CARTESIAN_POINT('Ctrl Pts',(-0.226842621902213,0.0131746060428305,
-0.00881739135542764));
#46565=CARTESIAN_POINT('Ctrl Pts',(-0.226938629422854,0.0131992305333852,
-0.00879836193580715));
#46566=CARTESIAN_POINT('Ctrl Pts',(-0.227013983078059,0.0127097047938499,
-0.00907297714742843));
#46567=CARTESIAN_POINT('Ctrl Pts',(-0.227012239789711,0.0127690078022699,
-0.00915470391965529));
#46568=CARTESIAN_POINT('Ctrl Pts',(-0.227109707645705,0.0127899788532772,
-0.00914054786865483));
#46569=CARTESIAN_POINT('Ctrl Pts',(-0.227247196171394,0.0119136086184864,
-0.00960839126399033));
#46570=CARTESIAN_POINT('Ctrl Pts',(-0.22724548833278,0.0119636176376727,
-0.00969634779479045));
#46571=CARTESIAN_POINT('Ctrl Pts',(-0.227340402437741,0.0119956557482216,
-0.00967769841531056));
#46572=CARTESIAN_POINT('Ctrl Pts',(-0.227934521197248,0.0108226289252953,
-0.0101349612257964));
#46573=CARTESIAN_POINT('Ctrl Pts',(-0.227932339489337,0.0108606492245814,
-0.0102288267212789));
#46574=CARTESIAN_POINT('Ctrl Pts',(-0.228016200220304,0.0109137714728394,
-0.0102076384847793));
#46575=CARTESIAN_POINT('Ctrl Pts',(-0.22871448845887,0.00979872364412934,
-0.0104964529615865));
#46576=CARTESIAN_POINT('Ctrl Pts',(-0.22871201473603,0.00982522763215701,
-0.0105942771404052));
#46577=CARTESIAN_POINT('Ctrl Pts',(-0.228792016848652,0.00988517379494635,
-0.0105788098693705));
#46578=CARTESIAN_POINT('Ctrl Pts',(-0.229293042529654,0.00909568586137089,
-0.0106532464722863));
#46579=CARTESIAN_POINT('Ctrl Pts',(-0.229290470784652,0.00911432520868509,
-0.010752734650283));
#46580=CARTESIAN_POINT('Ctrl Pts',(-0.229369210267429,0.00917698075244273,
-0.0107418335978009));
#46581=CARTESIAN_POINT('Ctrl Pts',(-0.229615819717098,0.00869617259597773,
-0.0107153935627931));
#46582=CARTESIAN_POINT('Ctrl Pts',(-0.229613213780719,0.00871029853769483,
-0.0108155121778463));
#46583=CARTESIAN_POINT('Ctrl Pts',(-0.229692353173153,0.00877277078058718,
-0.0108076154274616));
#46584=CARTESIAN_POINT('Ctrl Pts',(-0.229386006289235,0.00897973788217584,
-0.0106669693656825));
#46585=CARTESIAN_POINT('Ctrl Pts',(-0.229385834316954,0.00898106101767042,
-0.0106746123133356));
#46586=CARTESIAN_POINT('Ctrl Pts',(-0.229385712152104,0.00898372565412568,
-0.0106818666110971));
#46587=CARTESIAN_POINT('Ctrl Pts',(-0.229385551882414,0.00899195445542397,
-0.0106963846629467));
#46588=CARTESIAN_POINT('Ctrl Pts',(-0.229385531656438,0.00899774869796057,
-0.0107032419010174));
#46589=CARTESIAN_POINT('Ctrl Pts',(-0.229385610858662,0.00901508036564382,
-0.0107186785449647));
#46590=CARTESIAN_POINT('Ctrl Pts',(-0.229385792041169,0.00902866472857107,
-0.0107264500956539));
#46591=CARTESIAN_POINT('Ctrl Pts',(-0.229386386722512,0.00905943807325047,
-0.0107374076859636));
#46592=CARTESIAN_POINT('Ctrl Pts',(-0.229386768105326,0.00907540386138489,
-0.0107404657857017));
#46593=CARTESIAN_POINT('Ctrl Pts',(-0.229387633511884,0.00910728634568047,
-0.0107428879162213));
#46594=CARTESIAN_POINT('Ctrl Pts',(-0.229388121567382,0.00912354354792321,
-0.0107422591777074));
#46595=CARTESIAN_POINT('Ctrl Pts',(-0.229388775079068,0.00914282080369923,
-0.0107395367729916));
#46596=CARTESIAN_POINT('Ctrl Pts',(-0.229388881801912,0.00914623216986349,
-0.0107389781526564));
#46597=CARTESIAN_POINT('Ctrl Pts',(-0.229388998216237,0.00914960349487052,
-0.0107383496584743));
#46598=CARTESIAN_POINT('Origin',(-0.226555098762114,0.00178668839685616,
0.00865090131818249));
#46599=CARTESIAN_POINT('Ctrl Pts',(-0.225309797184906,0.00172192161890831,
0.00870374066956656));
#46600=CARTESIAN_POINT('Ctrl Pts',(-0.225310247209972,0.00172235519632964,
0.00870411103008553));
#46601=CARTESIAN_POINT('Ctrl Pts',(-0.225311002611275,0.00172203997768199,
0.00870385280409576));
#46602=CARTESIAN_POINT('Ctrl Pts',(-0.225311208914087,0.0017227600167316,
0.00870445023600111));
#46603=CARTESIAN_POINT('Ctrl Pts',(-0.225311530294346,0.00172322144104357,
0.00870483562786732));
#46604=CARTESIAN_POINT('Ctrl Pts',(-0.225312590214738,0.00172441475890014,
0.00870579884762694));
#46605=CARTESIAN_POINT('Ctrl Pts',(-0.225313028186745,0.0017248801472261,
0.00870616864922502));
#46606=CARTESIAN_POINT('Ctrl Pts',(-0.225314185750255,0.00172609889403774,
0.00870712172336859));
#46607=CARTESIAN_POINT('Ctrl Pts',(-0.225315014254334,0.00172695494933646,
0.00870777150728844));
#46608=CARTESIAN_POINT('Ctrl Pts',(-0.225317459383959,0.00172950059423514,
0.00870963873423945));
#46609=CARTESIAN_POINT('Ctrl Pts',(-0.225319089298796,0.00173121682918185,
0.00871081933948459));
#46610=CARTESIAN_POINT('Ctrl Pts',(-0.225323946891331,0.00173644787754945,
0.00871418366037928));
#46611=CARTESIAN_POINT('Ctrl Pts',(-0.22532716864885,0.00174006163539265,
0.00871620917519089));
#46612=CARTESIAN_POINT('Ctrl Pts',(-0.225342294487028,0.00175779352469263,
0.00872475379468167));
#46613=CARTESIAN_POINT('Ctrl Pts',(-0.225353399479346,0.00177307296761273,
0.00872814969225069));
#46614=CARTESIAN_POINT('Ctrl Pts',(-0.225370257987112,0.00180064171972645,
0.00872779781635509));
#46615=CARTESIAN_POINT('Ctrl Pts',(-0.225376869823117,0.00181324593478133,
0.00872539716034856));
#46616=CARTESIAN_POINT('Ctrl Pts',(-0.225385913454783,0.00183523752526527,
0.00871613199201331));
#46617=CARTESIAN_POINT('Ctrl Pts',(-0.225388830957791,0.00184454886515225,
0.00871035273326283));
#46618=CARTESIAN_POINT('Ctrl Pts',(-0.225390971525641,0.00185659996340586,
0.00869956095985846));
#46619=CARTESIAN_POINT('Ctrl Pts',(-0.225391333711933,0.0018600452739431,
0.00869596993208362));
#46620=CARTESIAN_POINT('Ctrl Pts',(-0.225391399224265,0.00186320399461255,
0.00869213917474686));
#46621=CARTESIAN_POINT('Ctrl Pts',(-0.224314879611255,0.0165309527154701,
0.00169539118491105));
#46622=CARTESIAN_POINT('Ctrl Pts',(-0.224412832453008,0.0165261318210616,
0.0017283511372909));
#46623=CARTESIAN_POINT('Ctrl Pts',(-0.22440807336887,0.0164236964218974,
0.00172137583111113));
#46624=CARTESIAN_POINT('Ctrl Pts',(-0.224796453732221,0.0166076184506538,
0.000471064888113262));
#46625=CARTESIAN_POINT('Ctrl Pts',(-0.224893455689256,0.016609717003541,
0.000502793734545124));
#46626=CARTESIAN_POINT('Ctrl Pts',(-0.224891878603847,0.0165069023284093,
0.000502434681482319));
#46627=CARTESIAN_POINT('Ctrl Pts',(-0.225201428568935,0.0165700272266111,
-0.00117029070511372));
#46628=CARTESIAN_POINT('Ctrl Pts',(-0.225300625050002,0.0165676556420741,
-0.00114004230938044));
#46629=CARTESIAN_POINT('Ctrl Pts',(-0.225296650208344,0.0164651958368812,
-0.00114023248766775));
#46630=CARTESIAN_POINT('Ctrl Pts',(-0.226095507126995,0.0164417448751073,
-0.00299946840558335));
#46631=CARTESIAN_POINT('Ctrl Pts',(-0.226186142905089,0.0164482910388427,
-0.00295072881265121));
#46632=CARTESIAN_POINT('Ctrl Pts',(-0.226183670844414,0.0163459084325657,
-0.00293822423704356));
#46633=CARTESIAN_POINT('Ctrl Pts',(-0.226658272402392,0.016256772552681,
-0.00395106792067057));
#46634=CARTESIAN_POINT('Ctrl Pts',(-0.226745240907684,0.0162705352409148,
-0.00389734512079282));
#46635=CARTESIAN_POINT('Ctrl Pts',(-0.226743379782759,0.0161700948643406,
-0.00387393372333392));
#46636=CARTESIAN_POINT('Ctrl Pts',(-0.227309431860278,0.0159880923504392,
-0.00485196380139293));
#46637=CARTESIAN_POINT('Ctrl Pts',(-0.227391181903299,0.0160099755008125,
-0.00479277052584003));
#46638=CARTESIAN_POINT('Ctrl Pts',(-0.227389517585843,0.015912267948463,
-0.00475943666660673));
#46639=CARTESIAN_POINT('Ctrl Pts',(-0.228028119018682,0.0156603845179188,
-0.00565588952548107));
#46640=CARTESIAN_POINT('Ctrl Pts',(-0.228105108350196,0.0156905302113713,
-0.00559393310834394));
#46641=CARTESIAN_POINT('Ctrl Pts',(-0.228103863210623,0.0155962483295275,
-0.00555167686899847));
#46642=CARTESIAN_POINT('Ctrl Pts',(-0.228802757285458,0.0152823868470796,
-0.00638961457773919));
#46643=CARTESIAN_POINT('Ctrl Pts',(-0.228875533245265,0.0153203957783105,
-0.00632681833521576));
#46644=CARTESIAN_POINT('Ctrl Pts',(-0.228874614212836,0.0152301844971178,
-0.00627636725223939));
#46645=CARTESIAN_POINT('Ctrl Pts',(-0.229627994727228,0.0148670422144861,
-0.00705276295927651));
#46646=CARTESIAN_POINT('Ctrl Pts',(-0.229696602632231,0.0149126078655,-0.00699024645412036));
#46647=CARTESIAN_POINT('Ctrl Pts',(-0.229695993342631,0.0148268265883492,
-0.00693249486514969));
#46648=CARTESIAN_POINT('Ctrl Pts',(-0.230481878170306,0.01442369053443,
-0.00765169618674575));
#46649=CARTESIAN_POINT('Ctrl Pts',(-0.230549279564022,0.0144748984918072,
-0.00759242459387856));
#46650=CARTESIAN_POINT('Ctrl Pts',(-0.230549019547242,0.014393931285933,
-0.00752807881257224));
#46651=CARTESIAN_POINT('Ctrl Pts',(-0.231177467493998,0.014003890473077,
-0.00813697751827833));
#46652=CARTESIAN_POINT('Ctrl Pts',(-0.231249685385162,0.0140565675637169,
-0.00808465444694161));
#46653=CARTESIAN_POINT('Ctrl Pts',(-0.231249658084979,0.0139803452106898,
-0.00801487102447448));
#46654=CARTESIAN_POINT('Ctrl Pts',(-0.231670728309359,0.0135947224063574,
-0.00854712336180957));
#46655=CARTESIAN_POINT('Ctrl Pts',(-0.231752619804048,0.0136426772192251,
-0.00850601156601645));
#46656=CARTESIAN_POINT('Ctrl Pts',(-0.231752693652761,0.0135714697124679,
-0.00843141437557248));
#46657=CARTESIAN_POINT('Ctrl Pts',(-0.231966406597232,0.0132362082644641,
-0.00887116443097536));
#46658=CARTESIAN_POINT('Ctrl Pts',(-0.232062273088291,0.0132709718533777,
-0.00884649553010581));
#46659=CARTESIAN_POINT('Ctrl Pts',(-0.232062481656899,0.0132042914499902,
-0.0087681741575853));
#46660=CARTESIAN_POINT('Ctrl Pts',(-0.232089783925324,0.0127867877948663,
-0.00922721017894486));
#46661=CARTESIAN_POINT('Ctrl Pts',(-0.232195444754471,0.0127888549173578,
-0.00923064524789568));
#46662=CARTESIAN_POINT('Ctrl Pts',(-0.232195795965022,0.0127281581789461,
-0.00914789582704976));
#46663=CARTESIAN_POINT('Ctrl Pts',(-0.231968971356067,0.0123157844703992,
-0.00954672899977835));
#46664=CARTESIAN_POINT('Ctrl Pts',(-0.232065675411668,0.012285771447896,
-0.00957008688076997));
#46665=CARTESIAN_POINT('Ctrl Pts',(-0.232066144322818,0.0122309820328145,
-0.00948309977348297));
#46666=CARTESIAN_POINT('Ctrl Pts',(-0.231720771626718,0.0118689957268499,
-0.00980836544689196));
#46667=CARTESIAN_POINT('Ctrl Pts',(-0.231809935349982,0.0118256369660778,
-0.00983624870656414));
#46668=CARTESIAN_POINT('Ctrl Pts',(-0.231810485252569,0.0117760634407629,
-0.00974603498528647));
#46669=CARTESIAN_POINT('Ctrl Pts',(-0.231315018306534,0.0113053865717837,
-0.0100956259794169));
#46670=CARTESIAN_POINT('Ctrl Pts',(-0.231397271592812,0.0112501747778728,
-0.0101251515102169));
#46671=CARTESIAN_POINT('Ctrl Pts',(-0.23139798144253,0.011207353978372,
-0.0100313194005554));
#46672=CARTESIAN_POINT('Ctrl Pts',(-0.23072504796845,0.010615585256532,
-0.0103774887010382));
#46673=CARTESIAN_POINT('Ctrl Pts',(-0.230803651447536,0.0105540854545879,
-0.0104034766730699));
#46674=CARTESIAN_POINT('Ctrl Pts',(-0.230804445927653,0.0105194090449751,
-0.0103062150531577));
#46675=CARTESIAN_POINT('Ctrl Pts',(-0.229647060853282,0.00942256760179786,
-0.0107297449576376));
#46676=CARTESIAN_POINT('Ctrl Pts',(-0.229722099652704,0.00935373083032424,
-0.0107480730605707));
#46677=CARTESIAN_POINT('Ctrl Pts',(-0.229723102517257,0.00933302452585627,
-0.0106465471042351));
#46678=CARTESIAN_POINT('Ctrl Pts',(-0.228778830421403,0.00850199841465629,
-0.0108449553313066));
#46679=CARTESIAN_POINT('Ctrl Pts',(-0.228855210405385,0.00843344082546064,
-0.0108554634871318));
#46680=CARTESIAN_POINT('Ctrl Pts',(-0.228856077356639,0.00842299482164084,
-0.0107526226063158));
#46681=CARTESIAN_POINT('Ctrl Pts',(-0.228206393600378,0.00780936869860245,
-0.0108644994342279));
#46682=CARTESIAN_POINT('Ctrl Pts',(-0.228284049039534,0.00774147764959962,
-0.0108702768244508));
#46683=CARTESIAN_POINT('Ctrl Pts',(-0.228285021567739,0.00773913782172368,
-0.010767089034139));
#46684=CARTESIAN_POINT('Ctrl Pts',(-0.225009750798511,0.0164742919676833,
-2.94234935793932E-7));
#46685=CARTESIAN_POINT('Ctrl Pts',(-0.225009853509087,0.0164809894657856,
-2.94108435594111E-7));
#46686=CARTESIAN_POINT('Ctrl Pts',(-0.225009248162902,0.0164876738465301,
-2.94985003331512E-7));
#46687=CARTESIAN_POINT('Ctrl Pts',(-0.225006557138774,0.0165012782295379,
-2.98820133665149E-7));
#46688=CARTESIAN_POINT('Ctrl Pts',(-0.225004381157442,0.0165081277083827,
-3.01905547296842E-7));
#46689=CARTESIAN_POINT('Ctrl Pts',(-0.224996139283575,0.0165266941161087,
-3.13528887012115E-7));
#46690=CARTESIAN_POINT('Ctrl Pts',(-0.224988442162309,0.0165374948473636,
-3.24342008419143E-7));
#46691=CARTESIAN_POINT('Ctrl Pts',(-0.224969252270092,0.016555753366864,
-3.5089401941877E-7));
#46692=CARTESIAN_POINT('Ctrl Pts',(-0.224957889791733,0.0165629935330378,
-3.66636042736974E-7));
#46693=CARTESIAN_POINT('Ctrl Pts',(-0.224933916678097,0.0165726615164696,
-3.97335259411207E-7));
#46694=CARTESIAN_POINT('Ctrl Pts',(-0.224922798675663,0.0165748188773007,
-4.30993709014285E-7));
#46695=CARTESIAN_POINT('Ctrl Pts',(-0.224910907505475,0.0165757632925934,
-3.97281805675274E-7));
#46696=CARTESIAN_POINT('Ctrl Pts',(-0.224908458936007,0.0165758792333304,
-4.40024533364447E-7));
#46697=CARTESIAN_POINT('Ctrl Pts',(-0.224906181933197,0.0165759154128579,
-4.43226285311814E-7));
#46698=CARTESIAN_POINT('Origin',(-0.226648799791358,0.00779550107807324,
0.0018430762351178));
#46699=CARTESIAN_POINT('Ctrl Pts',(-0.225192864155308,0.00215336583509703,
0.00904010670453624));
#46700=CARTESIAN_POINT('Ctrl Pts',(-0.225204706288654,0.00216933111886313,
0.00905188432053952));
#46701=CARTESIAN_POINT('Ctrl Pts',(-0.225224728767847,0.00220285845149844,
0.00906873009866757));
#46702=CARTESIAN_POINT('Ctrl Pts',(-0.225240738467706,0.00223802863421344,
0.00907116763090578));
#46703=CARTESIAN_POINT('Ctrl Pts',(-0.22525674809356,0.00227319865435349,
0.00907360515187645));
#46704=CARTESIAN_POINT('Ctrl Pts',(-0.225269616920643,0.00230901002534829,
0.00906077332273702));
#46705=CARTESIAN_POINT('Ctrl Pts',(-0.225269618511371,0.00232397812765925,
0.00904117190417335));
#46706=CARTESIAN_POINT('Ctrl Pts',(-0.224423102415366,0.0164240572405408,
-0.0017009526594877));
#46707=CARTESIAN_POINT('Ctrl Pts',(-0.22442753931816,0.0165274809959018,
-0.00170826230446446));
#46708=CARTESIAN_POINT('Ctrl Pts',(-0.224328623267926,0.0165310813381061,
-0.00167531627545616));
#46709=CARTESIAN_POINT('Ctrl Pts',(-0.224888576396618,0.0165068622639915,
-0.000507779096031469));
#46710=CARTESIAN_POINT('Ctrl Pts',(-0.224890080375599,0.0166106061384932,
-0.000507850690853431));
#46711=CARTESIAN_POINT('Ctrl Pts',(-0.224792054255541,0.0166074069025231,
-0.000476013916690959));
#46712=CARTESIAN_POINT('Ctrl Pts',(-0.225297934651115,0.0164656143571788,
0.00113605080611901));
#46713=CARTESIAN_POINT('Ctrl Pts',(-0.22530166511579,0.0165690618324774,
0.00113577106828663));
#46714=CARTESIAN_POINT('Ctrl Pts',(-0.225201608773796,0.0165702170608381,
0.00116603472722438));
#46715=CARTESIAN_POINT('Ctrl Pts',(-0.226160156840923,0.0163464165517524,
0.00293824900518469));
#46716=CARTESIAN_POINT('Ctrl Pts',(-0.226162443178585,0.0164497276877427,
0.00295095984804816));
#46717=CARTESIAN_POINT('Ctrl Pts',(-0.226070274722855,0.0164421273393253,
0.00299861916200696));
#46718=CARTESIAN_POINT('Ctrl Pts',(-0.226875182678137,0.0161110455835552,
0.00419057100130972));
#46719=CARTESIAN_POINT('Ctrl Pts',(-0.226876732829769,0.0162117033653627,
0.00421805256419852));
#46720=CARTESIAN_POINT('Ctrl Pts',(-0.226788904849661,0.016194807216906,
0.00427157151275447));
#46721=CARTESIAN_POINT('Ctrl Pts',(-0.227956254663923,0.0156144693913653,
0.00560704096080674));
#46722=CARTESIAN_POINT('Ctrl Pts',(-0.227957828737694,0.0157095212737186,
0.00565098557902036));
#46723=CARTESIAN_POINT('Ctrl Pts',(-0.227877264381436,0.0156793865260549,
0.00571072697276061));
#46724=CARTESIAN_POINT('Ctrl Pts',(-0.229210309208534,0.0149506460476673,
0.00676589468964074));
#46725=CARTESIAN_POINT('Ctrl Pts',(-0.229210872891863,0.0150384255713987,
0.00682253731830502));
#46726=CARTESIAN_POINT('Ctrl Pts',(-0.229137956318801,0.0149947728795728,
0.00688320487905378));
#46727=CARTESIAN_POINT('Ctrl Pts',(-0.230287556148017,0.0143461956309686,
0.00758447983064182));
#46728=CARTESIAN_POINT('Ctrl Pts',(-0.230287717729031,0.01442714587865,
0.0076503219879991));
#46729=CARTESIAN_POINT('Ctrl Pts',(-0.23021627985812,0.0143760462362006,
0.00770647349494255));
#46730=CARTESIAN_POINT('Ctrl Pts',(-0.230951348226825,0.0139153574913946,
0.00807928185038737));
#46731=CARTESIAN_POINT('Ctrl Pts',(-0.230951233983676,0.0139913315871583,
0.00815069361700217));
#46732=CARTESIAN_POINT('Ctrl Pts',(-0.230876037824531,0.0139384580487563,
0.00820029147724192));
#46733=CARTESIAN_POINT('Ctrl Pts',(-0.231432809970025,0.0135059184053885,
0.00848700995994168));
#46734=CARTESIAN_POINT('Ctrl Pts',(-0.231432584554041,0.0135768401502669,
0.00856317562692272));
#46735=CARTESIAN_POINT('Ctrl Pts',(-0.231349537669097,0.0135278627464521,
0.00860273139657538));
#46736=CARTESIAN_POINT('Ctrl Pts',(-0.231745465211004,0.0131461000136674,
0.00881019374563095));
#46737=CARTESIAN_POINT('Ctrl Pts',(-0.231745063580486,0.013212670154277,
0.00888993882945493));
#46738=CARTESIAN_POINT('Ctrl Pts',(-0.231651625200096,0.0131728945446976,
0.00891695333527741));
#46739=CARTESIAN_POINT('Ctrl Pts',(-0.231924372807378,0.0126958161713031,
0.0091657531528894));
#46740=CARTESIAN_POINT('Ctrl Pts',(-0.231923809183617,0.0127567627508423,
0.00924952970467843));
#46741=CARTESIAN_POINT('Ctrl Pts',(-0.231818227394473,0.0127436564621929,
0.00925272722690912));
#46742=CARTESIAN_POINT('Ctrl Pts',(-0.231871582732807,0.0121954486342374,
0.00950210157316456));
#46743=CARTESIAN_POINT('Ctrl Pts',(-0.231870910432785,0.012250396442285,
0.00959002308213435));
#46744=CARTESIAN_POINT('Ctrl Pts',(-0.231769686742723,0.012271888694355,
0.00957067213786439));
#46745=CARTESIAN_POINT('Ctrl Pts',(-0.231655490809696,0.0117298373815043,
0.00976870709561953));
#46746=CARTESIAN_POINT('Ctrl Pts',(-0.231654730412008,0.0117793811745959,
0.00985996820273655));
#46747=CARTESIAN_POINT('Ctrl Pts',(-0.231561990926401,0.0118183205410903,
0.00983340751634403));
#46748=CARTESIAN_POINT('Ctrl Pts',(-0.231272911021964,0.0111462630541763,
0.0100571125220447));
#46749=CARTESIAN_POINT('Ctrl Pts',(-0.231272010484576,0.011188849482947,
0.0101520756394755));
#46750=CARTESIAN_POINT('Ctrl Pts',(-0.23118753117075,0.0112425848166589,
0.0101223341433138));
#46751=CARTESIAN_POINT('Ctrl Pts',(-0.230703596413716,0.0104641706532134,
0.010323445088338));
#46752=CARTESIAN_POINT('Ctrl Pts',(-0.230702628925254,0.0104986298412639,
0.0104217843528756));
#46753=CARTESIAN_POINT('Ctrl Pts',(-0.230622791844109,0.0105598058105489,
0.0103951096952851));
#46754=CARTESIAN_POINT('Ctrl Pts',(-0.229654376601397,0.00928919713295885,
0.0106537304156924));
#46755=CARTESIAN_POINT('Ctrl Pts',(-0.229653231650024,0.00930975120703328,
0.0107562426244593));
#46756=CARTESIAN_POINT('Ctrl Pts',(-0.229576535600367,0.00937798854178594,
0.0107371719305779));
#46757=CARTESIAN_POINT('Ctrl Pts',(-0.22880130602491,0.00837465238807093,
0.0107570024335721));
#46758=CARTESIAN_POINT('Ctrl Pts',(-0.228800187139004,0.00838466046235115,
0.0108608767335588));
#46759=CARTESIAN_POINT('Ctrl Pts',(-0.228723594842368,0.00845424764654016,
0.0108493022767735));
#46760=CARTESIAN_POINT('Ctrl Pts',(-0.228220153777608,0.00770395662147991,
0.010764867331218));
#46761=CARTESIAN_POINT('Ctrl Pts',(-0.228219244623913,0.00770629588168661,
0.0108689369194601));
#46762=CARTESIAN_POINT('Ctrl Pts',(-0.228139692445573,0.00777347521877263,
0.0108625950646913));
#46763=CARTESIAN_POINT('Ctrl Pts',(-0.229319785018526,0.00893281966668023,
0.0106733205234826));
#46764=CARTESIAN_POINT('Ctrl Pts',(-0.229318259485533,0.00894418630796205,
0.0107410766231035));
#46765=CARTESIAN_POINT('Ctrl Pts',(-0.229320209696457,0.00903641302211148,
0.0107575141350037));
#46766=CARTESIAN_POINT('Ctrl Pts',(-0.229322271958198,0.00910280340307577,
0.0107454877379686));
#46767=CARTESIAN_POINT('Origin',(-0.22504807827475,0.00267369066304345,
0.00928633187534054));
#46768=CARTESIAN_POINT('Ctrl Pts',(-0.224893951312673,0.00215954182917785,
0.00903842305818316));
#46769=CARTESIAN_POINT('Ctrl Pts',(-0.224911141103877,0.00216992176564713,
0.00904603151524389));
#46770=CARTESIAN_POINT('Ctrl Pts',(-0.224951134219812,0.00219064274957742,
0.0090535915278308));
#46771=CARTESIAN_POINT('Ctrl Pts',(-0.22497913921113,0.00221947895890837,
0.00904507092145141));
#46772=CARTESIAN_POINT('Ctrl Pts',(-0.225002380419073,0.00224340999069353,
0.00903799971109383));
#46773=CARTESIAN_POINT('Ctrl Pts',(-0.225014260642788,0.00227143120128385,
0.00902261128732804));
#46774=CARTESIAN_POINT('Ctrl Pts',(-0.225014720871232,0.00228334524727118,
0.0090072968842552));
#46775=CARTESIAN_POINT('Ctrl Pts',(-0.229620207397339,0.00855813827595884,
0.0107332969856487));
#46776=CARTESIAN_POINT('Ctrl Pts',(-0.229616538665817,0.00857090518029757,
0.0108412348410576));
#46777=CARTESIAN_POINT('Ctrl Pts',(-0.229701615329559,0.00863731696429406,
0.0108269786528085));
#46778=CARTESIAN_POINT('Ctrl Pts',(-0.22903299248322,0.00930406829717384,
0.0106244444186668));
#46779=CARTESIAN_POINT('Ctrl Pts',(-0.229029268207648,0.00932610885666542,
0.0107311427610987));
#46780=CARTESIAN_POINT('Ctrl Pts',(-0.229113325739694,0.00939167115900597,
0.0107118574650714));
#46781=CARTESIAN_POINT('Ctrl Pts',(-0.228116908040458,0.0103192133070879,
0.0103716166304235));
#46782=CARTESIAN_POINT('Ctrl Pts',(-0.228113961793712,0.010352440661458,
0.0104760412785541));
#46783=CARTESIAN_POINT('Ctrl Pts',(-0.228201379265707,0.0104150729421031,
0.0104460896936027));
#46784=CARTESIAN_POINT('Ctrl Pts',(-0.22728197906512,0.0119325496639152,
0.00959955446290684));
#46785=CARTESIAN_POINT('Ctrl Pts',(-0.227279031174141,0.0119862717024164,
0.00969406047754389));
#46786=CARTESIAN_POINT('Ctrl Pts',(-0.227383186150131,0.0120112033292314,
0.00967194223499914));
#46787=CARTESIAN_POINT('Ctrl Pts',(-0.227034169568235,0.0127020208624721,
0.00907567277747115));
#46788=CARTESIAN_POINT('Ctrl Pts',(-0.227031194864248,0.0127655060260149,
0.00916367976789601));
#46789=CARTESIAN_POINT('Ctrl Pts',(-0.227134428282106,0.0127877316141476,
0.00914076544299377));
#46790=CARTESIAN_POINT('Ctrl Pts',(-0.226856974623676,0.0131107264396041,
0.00873962932632364));
#46791=CARTESIAN_POINT('Ctrl Pts',(-0.226854228559386,0.013178989557894,
0.00882371307415828));
#46792=CARTESIAN_POINT('Ctrl Pts',(-0.226957558425783,0.0132004200200363,
0.00879837917996526));
#46793=CARTESIAN_POINT('Ctrl Pts',(-0.22709761102,0.0128296959531864,0.00908953899803701));
#46794=CARTESIAN_POINT('Ctrl Pts',(-0.227097896903337,0.0128293463272935,
0.00908980452749194));
#46795=CARTESIAN_POINT('Ctrl Pts',(-0.227097980985701,0.0128291697025301,
0.00908993637037429));
#46796=CARTESIAN_POINT('Ctrl Pts',(-0.22709798906973,0.0128291516969385,
0.00908994979281978));
#46797=CARTESIAN_POINT('Ctrl Pts',(-0.227097999108598,0.0128291278282252,
0.0090899675611068));
#46798=CARTESIAN_POINT('Ctrl Pts',(-0.227098001470723,0.012829122091011,
0.00908997183012093));
#46799=CARTESIAN_POINT('Ctrl Pts',(-0.227098006026732,0.0128291107783129,
0.0090899802440751));
#46800=CARTESIAN_POINT('Ctrl Pts',(-0.2270980082234,0.0128291052041497,
0.00908998438815479));
#46801=CARTESIAN_POINT('Ctrl Pts',(-0.227098013190528,0.0128290923132555,
0.00908999396767163));
#46802=CARTESIAN_POINT('Ctrl Pts',(-0.227098015929209,0.0128290849890549,
0.00908999940738772));
#46803=CARTESIAN_POINT('Ctrl Pts',(-0.227098021113615,0.0128290706815099,
0.00909001002758949));
#46804=CARTESIAN_POINT('Ctrl Pts',(-0.227098023566733,0.0128290637014166,
0.00909001520597644));
#46805=CARTESIAN_POINT('Ctrl Pts',(-0.227098030839428,0.0128290423360304,
0.00909003104784491));
#46806=CARTESIAN_POINT('Ctrl Pts',(-0.227098035427359,0.01282902790273,
0.00909004173781594));
#46807=CARTESIAN_POINT('Ctrl Pts',(-0.227098087132581,0.012828852541214,
0.00909017147004589));
#46808=CARTESIAN_POINT('Ctrl Pts',(-0.227098092975546,0.012828693757072,
0.00909028745450568));
#46809=CARTESIAN_POINT('Ctrl Pts',(-0.227098036381531,0.0128283795127757,
0.00909051412772828));
#46810=CARTESIAN_POINT('Ctrl Pts',(-0.227097981119594,0.0128282316182478,
0.00909061957142001));
#46811=CARTESIAN_POINT('Ctrl Pts',(-0.22709781509159,0.0128278855864363,
0.00909086411088216));
#46812=CARTESIAN_POINT('Ctrl Pts',(-0.22709768022983,0.0128276751102533,
0.00909101080013109));
#46813=CARTESIAN_POINT('Ctrl Pts',(-0.227097330399864,0.0128271776743247,
0.00909135402846317));
#46814=CARTESIAN_POINT('Ctrl Pts',(-0.22709706096517,0.0128268448743511,
0.00909157963435271));
#46815=CARTESIAN_POINT('Ctrl Pts',(-0.227096353084741,0.0128260014481448,
0.00909214351272337));
#46816=CARTESIAN_POINT('Ctrl Pts',(-0.227095796735987,0.0128253813011885,
0.00909254670859746));
#46817=CARTESIAN_POINT('Ctrl Pts',(-0.227093819503803,0.0128231928490514,
0.00909393301778212));
#46818=CARTESIAN_POINT('Ctrl Pts',(-0.227092192667826,0.0128214263144734,
0.00909497481582912));
#46819=CARTESIAN_POINT('Ctrl Pts',(-0.22708508832393,0.0128134962161041,
0.00909924848525208));
#46820=CARTESIAN_POINT('Ctrl Pts',(-0.227079680338992,0.0128070270610738,
0.00910182504888053));
#46821=CARTESIAN_POINT('Ctrl Pts',(-0.227065324825336,0.0127883677251284,
0.00910683477824836));
#46822=CARTESIAN_POINT('Ctrl Pts',(-0.22705668742453,0.0127754892527389,
0.0091077276220021));
#46823=CARTESIAN_POINT('Ctrl Pts',(-0.227042441902929,0.0127503795925126,
0.00910418707108994));
#46824=CARTESIAN_POINT('Ctrl Pts',(-0.227036677809703,0.0127382988866502,
0.00910026136023822));
#46825=CARTESIAN_POINT('Ctrl Pts',(-0.227030063463232,0.012720118593403,
0.00909009366612189));
#46826=CARTESIAN_POINT('Ctrl Pts',(-0.227028200856115,0.0127136996055961,
0.00908552597126478));
#46827=CARTESIAN_POINT('Ctrl Pts',(-0.227025944415882,0.012702340715504,
0.00907528610289493));
#46828=CARTESIAN_POINT('Ctrl Pts',(-0.227025454709595,0.0126974045244964,
0.00906981769686516));
#46829=CARTESIAN_POINT('Ctrl Pts',(-0.22702558160064,0.0126930625462286,
0.0090638516120818));
#46830=CARTESIAN_POINT('Origin',(-0.221493379745634,0.00394271703026399,
0.00803042653342771));
#46831=CARTESIAN_POINT('Ctrl Pts',(-0.225016038306626,0.00296527640567411,
0.00956936262132929));
#46832=CARTESIAN_POINT('Ctrl Pts',(-0.225054837504787,0.00296676909900014,
0.0095710276794746));
#46833=CARTESIAN_POINT('Ctrl Pts',(-0.225088091302381,0.00298068453682126,
0.0095516424980561));
#46834=CARTESIAN_POINT('Ctrl Pts',(-0.225103269221005,0.00299367647273647,
0.0095306661184691));
#46835=CARTESIAN_POINT('Ctrl Pts',(-0.225113739935693,0.00300263915448291,
0.00951619524856506));
#46836=CARTESIAN_POINT('Ctrl Pts',(-0.225117785239288,0.00301142193691076,
0.00950115649627434));
#46837=CARTESIAN_POINT('Ctrl Pts',(-0.225118071269482,0.00301949283818061,
0.00948729957575529));
#46838=CARTESIAN_POINT('Origin',(-0.226780511856133,0.0100405374416167,
0.0110051741771939));
#46839=CARTESIAN_POINT('Ctrl Pts',(-0.226273558818709,0.0126615507097427,
0.00907157974325745));
#46840=CARTESIAN_POINT('Ctrl Pts',(-0.226273018871854,0.0126830229129793,
0.00910141756778122));
#46841=CARTESIAN_POINT('Ctrl Pts',(-0.226298864402728,0.0127209315695524,
0.00910908677761961));
#46842=CARTESIAN_POINT('Ctrl Pts',(-0.226321295777411,0.0127454310152486,
0.00910934848928192));
#46843=CARTESIAN_POINT('Ctrl Pts',(-0.226340598417199,0.0127665132708808,
0.00910957369732274));
#46844=CARTESIAN_POINT('Ctrl Pts',(-0.226353873932747,0.0127801920629709,
0.00910660552022882));
#46845=CARTESIAN_POINT('Ctrl Pts',(-0.226383304101992,0.0128042931570195,
0.0090932051586158));
#46846=CARTESIAN_POINT('Ctrl Pts',(-0.22638807437404,0.0128081996508736,
0.00909103312318123));
#46847=CARTESIAN_POINT('Ctrl Pts',(-0.226393292302312,0.0128123158788516,
0.0090885067005233));
#46848=CARTESIAN_POINT('Ctrl Pts',(-0.226399047297907,0.0128166255196227,
0.00908546833389411));
#46849=CARTESIAN_POINT('Ctrl Pts',(-0.225133546245736,0.0079572727413433,
0.0106839114428361));
#46850=CARTESIAN_POINT('Ctrl Pts',(-0.225131202582991,0.00796280010051278,
0.0107879669222465));
#46851=CARTESIAN_POINT('Ctrl Pts',(-0.225027565196397,0.00797114141935883,
0.0107807941497949));
#46852=CARTESIAN_POINT('Ctrl Pts',(-0.225049122764504,0.00703055902368649,
0.0107304119903276));
#46853=CARTESIAN_POINT('Ctrl Pts',(-0.225046767464602,0.00702503046949575,
0.0108350360113988));
#46854=CARTESIAN_POINT('Ctrl Pts',(-0.224943244930424,0.00703596129787379,
0.0108290232843219));
#46855=CARTESIAN_POINT('Ctrl Pts',(-0.224889836960112,0.00513717572956065,
0.0105283887484728));
#46856=CARTESIAN_POINT('Ctrl Pts',(-0.224887538335525,0.00510991286636644,
0.0106307975956611));
#46857=CARTESIAN_POINT('Ctrl Pts',(-0.224783218214591,0.0051108634611282,
0.0106258911999091));
#46858=CARTESIAN_POINT('Ctrl Pts',(-0.225023719104184,0.00339280049023757,
0.00974486159724177));
#46859=CARTESIAN_POINT('Ctrl Pts',(-0.225021774812465,0.00334449320283454,
0.00983783365658757));
#46860=CARTESIAN_POINT('Ctrl Pts',(-0.224917880936671,0.0033382150606942,
0.00982841550280784));
#46861=CARTESIAN_POINT('Ctrl Pts',(-0.225194501068205,0.00263332843217836,
0.00925026456232951));
#46862=CARTESIAN_POINT('Ctrl Pts',(-0.225192783985461,0.00257626916693201,
0.00933748070290354));
#46863=CARTESIAN_POINT('Ctrl Pts',(-0.22509059122008,0.00256284175228321,
0.00932156835961672));
#46864=CARTESIAN_POINT('Ctrl Pts',(-0.225092271993048,0.0074950696415353,
0.0106948847060478));
#46865=CARTESIAN_POINT('Ctrl Pts',(-0.225092124042334,0.00749506551951806,
0.0107014292645462));
#46866=CARTESIAN_POINT('Ctrl Pts',(-0.225091331424227,0.00749506162327073,
0.0107079429871891));
#46867=CARTESIAN_POINT('Ctrl Pts',(-0.225088389756039,0.00749505407695255,
0.0107211269286868));
#46868=CARTESIAN_POINT('Ctrl Pts',(-0.225086166021754,0.00749505048060983,
0.0107277438866657));
#46869=CARTESIAN_POINT('Ctrl Pts',(-0.225077916451027,0.00749504104297401,
0.0107457912927371));
#46870=CARTESIAN_POINT('Ctrl Pts',(-0.225070344089698,0.00749503606449245,
0.0107563590318577));
#46871=CARTESIAN_POINT('Ctrl Pts',(-0.225051607693862,0.00749502702891778,
0.0107740521520703));
#46872=CARTESIAN_POINT('Ctrl Pts',(-0.225040617287013,0.0074950240544077,
0.0107810108087723));
#46873=CARTESIAN_POINT('Ctrl Pts',(-0.225011582445515,0.00749500389423601,
0.0107923667013775));
#46874=CARTESIAN_POINT('Ctrl Pts',(-0.224997392673719,0.00749510403851621,
0.0107925601345168));
#46875=CARTESIAN_POINT('Ctrl Pts',(-0.224992643923633,0.00749468154582047,
0.010792618809641));
#46876=CARTESIAN_POINT('Ctrl Pts',(-0.224992118552164,0.00749461327975819,
0.0107926204901728));
#46877=CARTESIAN_POINT('Ctrl Pts',(-0.224991378287202,0.00749441910071412,
0.0107926185236326));
#46878=CARTESIAN_POINT('Ctrl Pts',(-0.224991133735545,0.00749431857707768,
0.0107926165100084));
#46879=CARTESIAN_POINT('Ctrl Pts',(-0.224990604703868,0.00749391093596826,
0.0107926104063756));
#46880=CARTESIAN_POINT('Origin',(-0.227808378362649,0.00719112862353373,
0.00185696123111253));
#46881=CARTESIAN_POINT('Ctrl Pts',(-0.226520627867466,0.0132597435976571,
0.00874175744832851));
#46882=CARTESIAN_POINT('Ctrl Pts',(-0.226487176491317,0.0132389482725006,
0.0087584114230379));
#46883=CARTESIAN_POINT('Ctrl Pts',(-0.226470495664087,0.0132231203056123,
0.00876329055696138));
#46884=CARTESIAN_POINT('Ctrl Pts',(-0.226449937155245,0.0132037737465187,
0.00876353000619182));
#46885=CARTESIAN_POINT('Ctrl Pts',(-0.226447721306919,0.0132016885252163,
0.00876355581463836));
#46886=CARTESIAN_POINT('Ctrl Pts',(-0.226445475166781,0.0131995315973307,
0.00876349525475088));
#46887=CARTESIAN_POINT('Ctrl Pts',(-0.226443190924595,0.0131972703049045,
0.0087633363683377));
#46888=CARTESIAN_POINT('Ctrl Pts',(-0.226421963144674,0.013176255800291,
0.00876185981483047));
#46889=CARTESIAN_POINT('Ctrl Pts',(-0.226400801825894,0.0131437796706972,
0.00875009709576872));
#46890=CARTESIAN_POINT('Ctrl Pts',(-0.226398183046263,0.0131243802924447,
0.008731911942556));
#46891=CARTESIAN_POINT('Ctrl Pts',(-0.226397905532036,0.0131223245244056,
0.00872998484694108));
#46892=CARTESIAN_POINT('Ctrl Pts',(-0.226397790265506,0.013120436131916,
0.00872799650275696));
#46893=CARTESIAN_POINT('Ctrl Pts',(-0.226397825284883,0.0131187534369297,
0.00872595188639632));
#46894=CARTESIAN_POINT('Ctrl Pts',(-0.225190041859337,0.0123109312972237,
0.00928452960023628));
#46895=CARTESIAN_POINT('Ctrl Pts',(-0.225189716453424,0.0123699621157433,
0.00937667255010711));
#46896=CARTESIAN_POINT('Ctrl Pts',(-0.225082687608397,0.012381811054789,
0.00935700919890517));
#46897=CARTESIAN_POINT('Ctrl Pts',(-0.224849534335206,0.0107686015790774,
0.0102729844456006));
#46898=CARTESIAN_POINT('Ctrl Pts',(-0.224848828147693,0.0108091195061921,
0.0103769377881753));
#46899=CARTESIAN_POINT('Ctrl Pts',(-0.224738109563861,0.0108069665241362,
0.0103708724457372));
#46900=CARTESIAN_POINT('Ctrl Pts',(-0.224962173305664,0.00887287258771333,
0.0107780555327175));
#46901=CARTESIAN_POINT('Ctrl Pts',(-0.224961178899313,0.00888991514828659,
0.0108886125707888));
#46902=CARTESIAN_POINT('Ctrl Pts',(-0.224853022929204,0.00887733942185127,
0.0108791940235274));
#46903=CARTESIAN_POINT('Ctrl Pts',(-0.225133451501574,0.00703771621441337,
0.0106819139847117));
#46904=CARTESIAN_POINT('Ctrl Pts',(-0.225132505084545,0.00703201791455483,
0.0107911553449083));
#46905=CARTESIAN_POINT('Ctrl Pts',(-0.225024003315464,0.00702327394296394,
0.0107799226729097));
#46906=CARTESIAN_POINT('Ctrl Pts',(-0.22511470191617,0.0119224377252866,
0.00952072100618005));
#46907=CARTESIAN_POINT('Ctrl Pts',(-0.225114237492274,0.0119352596408989,
0.00954312606581834));
#46908=CARTESIAN_POINT('Ctrl Pts',(-0.2251037365202,0.011950952820735,0.00957078918542189));
#46909=CARTESIAN_POINT('Ctrl Pts',(-0.225072256833985,0.0119632244350986,
0.00958934476625811));
#46910=CARTESIAN_POINT('Ctrl Pts',(-0.225056268536952,0.0119694570961923,
0.00959876900689375));
#46911=CARTESIAN_POINT('Ctrl Pts',(-0.225034719043819,0.0119741726577803,
0.00960469177404778));
#46912=CARTESIAN_POINT('Ctrl Pts',(-0.225012478416595,0.0119747498425115,
0.00960390435316071));
#46913=CARTESIAN_POINT('Origin',(-0.225236894197425,0.0131978724148554,
0.00863903100067282));
#46914=CARTESIAN_POINT('Ctrl Pts',(-0.225398010193384,0.013120318400212,
0.00870574369815946));
#46915=CARTESIAN_POINT('Ctrl Pts',(-0.22539764807259,0.0131371343383082,
0.00872622181582472));
#46916=CARTESIAN_POINT('Ctrl Pts',(-0.225383644932907,0.0131694250657152,
0.00874116107965085));
#46917=CARTESIAN_POINT('Ctrl Pts',(-0.225369785250098,0.0131944797608948,
0.00874167639760945));
#46918=CARTESIAN_POINT('Ctrl Pts',(-0.225357073815439,0.0132174587226127,
0.00874214902246313));
#46919=CARTESIAN_POINT('Ctrl Pts',(-0.225344323092837,0.0132335688478599,
0.00873837016524198));
#46920=CARTESIAN_POINT('Ctrl Pts',(-0.225322671626811,0.0132555887805521,
0.00872233569144969));
#46921=CARTESIAN_POINT('Ctrl Pts',(-0.225320715789482,0.0132575779025037,
0.00872088725269888));
#46922=CARTESIAN_POINT('Ctrl Pts',(-0.225318687903922,0.0132595961215726,
0.0087193083418805));
#46923=CARTESIAN_POINT('Ctrl Pts',(-0.225316581766884,0.0132616346613913,
0.00871757524912672));
#46924=CARTESIAN_POINT('Origin',(-0.22097494585212,0.0105087759000406,0.00743958985954961));
#46925=CARTESIAN_POINT('Ctrl Pts',(-0.224871009513959,0.0128386119989575,
0.00903955781216604));
#46926=CARTESIAN_POINT('Ctrl Pts',(-0.224916241833165,0.0128120209719476,
0.00906116586928584));
#46927=CARTESIAN_POINT('Ctrl Pts',(-0.224949040953459,0.0127765826465377,
0.00905521952879191));
#46928=CARTESIAN_POINT('Ctrl Pts',(-0.224969134043051,0.0127528695470433,
0.00904336442625093));
#46929=CARTESIAN_POINT('Ctrl Pts',(-0.224983890367304,0.0127354546948581,
0.00903465806298362));
#46930=CARTESIAN_POINT('Ctrl Pts',(-0.224992190595086,0.0127224256089223,
0.0090226133050689));
#46931=CARTESIAN_POINT('Ctrl Pts',(-0.22499258838655,0.0127125317992707,
0.00900988833309594));
#46932=CARTESIAN_POINT('Origin',(-0.226669448078697,0.00719407473391473,
0.00184050621984594));
#46933=CARTESIAN_POINT('Ctrl Pts',(-0.225275995996774,0.0126688942355271,
0.00904667010172663));
#46934=CARTESIAN_POINT('Ctrl Pts',(-0.225275996142043,0.0126847257901777,
0.00906724967341423));
#46935=CARTESIAN_POINT('Ctrl Pts',(-0.225262378782242,0.0127238511465841,
0.00907909399293944));
#46936=CARTESIAN_POINT('Ctrl Pts',(-0.225248326149835,0.0127563741278717,
0.00907641831404782));
#46937=CARTESIAN_POINT('Ctrl Pts',(-0.225234256379279,0.012788936773166,
0.00907373937198225));
#46938=CARTESIAN_POINT('Ctrl Pts',(-0.225217670901798,0.0128145451972767,
0.00906372431565276));
#46939=CARTESIAN_POINT('Ctrl Pts',(-0.225201030506077,0.0128404758197692,
0.0090447303940509));
#46940=CARTESIAN_POINT('Origin',(-0.225040472131482,0.0123086179887162,
0.00929799673594919));
#46941=CARTESIAN_POINT('Ctrl Pts',(-0.226460323864687,0.0164849848685168,
-0.00182542491256227));
#46942=CARTESIAN_POINT('Ctrl Pts',(-0.226357855404146,0.0164899166391132,
-0.00178775040261278));
#46943=CARTESIAN_POINT('Ctrl Pts',(-0.22636169061375,0.0163828437721616,
-0.00178569503389344));
#46944=CARTESIAN_POINT('Ctrl Pts',(-0.226928626615793,0.0165540683490847,
-0.000945327665866397));
#46945=CARTESIAN_POINT('Ctrl Pts',(-0.226829588972375,0.0165622085538829,
-0.00090622765606428));
#46946=CARTESIAN_POINT('Ctrl Pts',(-0.2268300202053,0.0164544928037623,
-0.000903811545142425));
#46947=CARTESIAN_POINT('Ctrl Pts',(-0.22732376166117,0.0165471381897995,
0.000459404657520975));
#46948=CARTESIAN_POINT('Ctrl Pts',(-0.227219857669224,0.0165519175322698,
0.00049097703221346));
#46949=CARTESIAN_POINT('Ctrl Pts',(-0.22722202781326,0.0164443490933984,
0.00048688368879839));
#46950=CARTESIAN_POINT('Ctrl Pts',(-0.228087003030431,0.0164796571711842,
0.00211169858914439));
#46951=CARTESIAN_POINT('Ctrl Pts',(-0.227992577930613,0.0164840917454652,
0.00216345181702484));
#46952=CARTESIAN_POINT('Ctrl Pts',(-0.227993997265494,0.0163765955727232,
0.00215882659204883));
#46953=CARTESIAN_POINT('Ctrl Pts',(-0.228710023259209,0.0164019593689328,
0.00316442782941463));
#46954=CARTESIAN_POINT('Ctrl Pts',(-0.228619671146624,0.0163991049219305,
0.0032241214340768));
#46955=CARTESIAN_POINT('Ctrl Pts',(-0.228621805321824,0.0162921981879355,
0.00320625921131432));
#46956=CARTESIAN_POINT('Ctrl Pts',(-0.229657567732581,0.0161254558637834,
0.0044874505494743));
#46957=CARTESIAN_POINT('Ctrl Pts',(-0.229574718139383,0.0161107313516101,
0.00455611627440692));
#46958=CARTESIAN_POINT('Ctrl Pts',(-0.229577504909484,0.016007399298503,
0.0045232489857868));
#46959=CARTESIAN_POINT('Ctrl Pts',(-0.230782492911356,0.0157135844815065,
0.00559630641179901));
#46960=CARTESIAN_POINT('Ctrl Pts',(-0.230706701936257,0.0156864648997765,
0.00566911350638642));
#46961=CARTESIAN_POINT('Ctrl Pts',(-0.230709555108569,0.0155883751293595,
0.00562241066007922));
#46962=CARTESIAN_POINT('Ctrl Pts',(-0.231954884548777,0.0151726511086173,
0.00661364144351075));
#46963=CARTESIAN_POINT('Ctrl Pts',(-0.231879927645458,0.0151359104217408,
0.00668269343885589));
#46964=CARTESIAN_POINT('Ctrl Pts',(-0.231883490729645,0.0150444879907642,
0.00662454319409727));
#46965=CARTESIAN_POINT('Ctrl Pts',(-0.232812135329546,0.0146956231411079,
0.00734628897413812));
#46966=CARTESIAN_POINT('Ctrl Pts',(-0.232730280256018,0.0146560965832439,
0.00740574769828582));
#46967=CARTESIAN_POINT('Ctrl Pts',(-0.23273445915703,0.0145703447276702,
0.00733970090416684));
#46968=CARTESIAN_POINT('Ctrl Pts',(-0.233526760469644,0.014056171381814,
0.00814319080840423));
#46969=CARTESIAN_POINT('Ctrl Pts',(-0.233430966824543,0.0140223502084935,
0.00818325695970401));
#46970=CARTESIAN_POINT('Ctrl Pts',(-0.233435828983806,0.0139438644997202,
0.00810904310707394));
#46971=CARTESIAN_POINT('Ctrl Pts',(-0.233963240632296,0.0132087652045752,
0.00896223768026468));
#46972=CARTESIAN_POINT('Ctrl Pts',(-0.233855630854944,0.0131932739624839,
0.00897664245241558));
#46973=CARTESIAN_POINT('Ctrl Pts',(-0.233860658240855,0.0131247144347458,
0.0088934990969508));
#46974=CARTESIAN_POINT('Ctrl Pts',(-0.233990673499441,0.0121849661189448,
0.00969801941997673));
#46975=CARTESIAN_POINT('Ctrl Pts',(-0.233882385854836,0.01219960051827,
0.00969004641588171));
#46976=CARTESIAN_POINT('Ctrl Pts',(-0.233887663559822,0.0121428785160235,
0.00959846506542782));
#46977=CARTESIAN_POINT('Ctrl Pts',(-0.233608550440856,0.0111179473338957,
0.0102465362016285));
#46978=CARTESIAN_POINT('Ctrl Pts',(-0.233510341012519,0.0111613510123303,
0.0102290029036576));
#46979=CARTESIAN_POINT('Ctrl Pts',(-0.233515957859729,0.0111166032784907,
0.0101308151772016));
#46980=CARTESIAN_POINT('Ctrl Pts',(-0.232973388139519,0.010116162533787,
0.0106005529114346));
#46981=CARTESIAN_POINT('Ctrl Pts',(-0.232885165283324,0.0101768275513439,
0.0105844086579605));
#46982=CARTESIAN_POINT('Ctrl Pts',(-0.232890700139198,0.0101433743507589,
0.0104816507674126));
#46983=CARTESIAN_POINT('Ctrl Pts',(-0.23159038031528,0.00836951725233097,
0.0109948951822117));
#46984=CARTESIAN_POINT('Ctrl Pts',(-0.231511257002863,0.00844418452103866,
0.0109893103432351));
#46985=CARTESIAN_POINT('Ctrl Pts',(-0.231517202802167,0.0084315211648833,
0.0108808883898792));
#46986=CARTESIAN_POINT('Ctrl Pts',(-0.230293417632758,0.00705158142584348,
0.0109556442486425));
#46987=CARTESIAN_POINT('Ctrl Pts',(-0.230215203379315,0.00712643592335552,
0.0109628407060781));
#46988=CARTESIAN_POINT('Ctrl Pts',(-0.230220372577151,0.00712874403259708,
0.010854144651623));
#46989=CARTESIAN_POINT('Ctrl Pts',(-0.229386810800953,0.0059251590909317,
0.0107665255249345));
#46990=CARTESIAN_POINT('Ctrl Pts',(-0.229301654948061,0.00599069017573065,
0.0107812705223676));
#46991=CARTESIAN_POINT('Ctrl Pts',(-0.229306186219208,0.00600670522370337,
0.0106743424323745));
#46992=CARTESIAN_POINT('Ctrl Pts',(-0.227105547431042,0.0164416356533416,
-1.96367242225517E-8));
#46993=CARTESIAN_POINT('Ctrl Pts',(-0.227106271411155,0.0164869558406628,
-1.56753936214819E-8));
#46994=CARTESIAN_POINT('Ctrl Pts',(-0.227142754365489,0.0165269328020988,
-7.87961297604824E-8));
#46995=CARTESIAN_POINT('Ctrl Pts',(-0.227186338350779,0.0165370366065652,
1.51447635016797E-7));
#46996=CARTESIAN_POINT('Ctrl Pts',(-0.227195260295749,0.0165391049256242,
1.9858013530413E-7));
#46997=CARTESIAN_POINT('Ctrl Pts',(-0.22720444130248,0.0165400702997432,
2.43952579346465E-7));
#46998=CARTESIAN_POINT('Ctrl Pts',(-0.22721356409307,0.0165399273072623,
2.64138495236366E-7));
#46999=CARTESIAN_POINT('Ctrl Pts',(-0.23059831458869,0.00749150590459184,
0.0108190894733326));
#47000=CARTESIAN_POINT('Ctrl Pts',(-0.230598147360955,0.00749149939828456,
0.0108265200709065));
#47001=CARTESIAN_POINT('Ctrl Pts',(-0.230599102175073,0.00749149541385465,
0.0108338813048351));
#47002=CARTESIAN_POINT('Ctrl Pts',(-0.230603304621065,0.00749149238562031,
0.0108489776967078));
#47003=CARTESIAN_POINT('Ctrl Pts',(-0.230606737271225,0.00749149395180183,
0.0108564893413419));
#47004=CARTESIAN_POINT('Ctrl Pts',(-0.230618362153178,0.00749150550463007,
0.0108749535226858));
#47005=CARTESIAN_POINT('Ctrl Pts',(-0.230628423413568,0.00749152031944393,
0.0108853640995515));
#47006=CARTESIAN_POINT('Ctrl Pts',(-0.23065496699676,0.00749157064776889,
0.0109041826329793));
#47007=CARTESIAN_POINT('Ctrl Pts',(-0.230671138540069,0.00749160344961521,
0.0109114284322365));
#47008=CARTESIAN_POINT('Ctrl Pts',(-0.230694761031536,0.00749168275194574,
0.0109179699756364));
#47009=CARTESIAN_POINT('Ctrl Pts',(-0.230701775839829,0.00749170704004545,
0.0109194442755902));
#47010=CARTESIAN_POINT('Ctrl Pts',(-0.230712384818665,0.00749178450294742,
0.0109210202406609));
#47011=CARTESIAN_POINT('Ctrl Pts',(-0.230715905182152,0.00749181293946376,
0.010921433226754));
#47012=CARTESIAN_POINT('Ctrl Pts',(-0.230721064742677,0.0074919198014703,
0.0109218917459213));
#47013=CARTESIAN_POINT('Ctrl Pts',(-0.230722841815142,0.0074919663207982,
0.0109220228385434));
#47014=CARTESIAN_POINT('Ctrl Pts',(-0.230725231630399,0.00749210732536436,
0.0109221676238527));
#47015=CARTESIAN_POINT('Ctrl Pts',(-0.23072618476541,0.00749217893940242,
0.0109222187380797));
#47016=CARTESIAN_POINT('Ctrl Pts',(-0.230727492126692,0.00749237315537678,
0.0109222792098174));
#47017=CARTESIAN_POINT('Ctrl Pts',(-0.230727934235603,0.00749246408382049,
0.0109222975651963));
#47018=CARTESIAN_POINT('Ctrl Pts',(-0.230728668324687,0.00749269378485217,
0.0109223256573981));
#47019=CARTESIAN_POINT('Ctrl Pts',(-0.230728965398421,0.00749282531917022,
0.0109223358742854));
#47020=CARTESIAN_POINT('Ctrl Pts',(-0.230729583032033,0.00749328310367994,
0.0109223542496217));
#47021=CARTESIAN_POINT('Ctrl Pts',(-0.22939971429741,0.00902231898868095,
0.0107696055271206));
#47022=CARTESIAN_POINT('Ctrl Pts',(-0.229317236826403,0.0089464276852763,
0.0107826523435916));
#47023=CARTESIAN_POINT('Ctrl Pts',(-0.229327136398156,0.00893435685226059,
0.0106710273104172));
#47024=CARTESIAN_POINT('Ctrl Pts',(-0.23028282524575,0.00794079935763272,
0.0109577498892055));
#47025=CARTESIAN_POINT('Ctrl Pts',(-0.230198785803285,0.00786578121681689,
0.010963523886201));
#47026=CARTESIAN_POINT('Ctrl Pts',(-0.230208806930841,0.00786787364958645,
0.0108505771393227));
#47027=CARTESIAN_POINT('Ctrl Pts',(-0.231597063345844,0.00661001185322147,
0.0109902582614569));
#47028=CARTESIAN_POINT('Ctrl Pts',(-0.231516131837863,0.00653048941558155,
0.0109820740545611));
#47029=CARTESIAN_POINT('Ctrl Pts',(-0.231526964171442,0.00654839740201362,
0.0108702093496403));
#47030=CARTESIAN_POINT('Ctrl Pts',(-0.232965808562566,0.00488992308630332,
0.0106020892738249));
#47031=CARTESIAN_POINT('Ctrl Pts',(-0.232873579300101,0.00482771019810843,
0.0105836762826241));
#47032=CARTESIAN_POINT('Ctrl Pts',(-0.232884605773775,0.00486582449374799,
0.0104782074384069));
#47033=CARTESIAN_POINT('Ctrl Pts',(-0.233605220528918,0.0038840291080987,
0.0102473328805686));
#47034=CARTESIAN_POINT('Ctrl Pts',(-0.233503283699538,0.00383871726872211,
0.0102270182108335));
#47035=CARTESIAN_POINT('Ctrl Pts',(-0.233514916837305,0.0038876872738603,
0.0101264028421645));
#47036=CARTESIAN_POINT('Ctrl Pts',(-0.233980537332444,0.00282437387879693,
0.0097033931294933));
#47037=CARTESIAN_POINT('Ctrl Pts',(-0.233867530792116,0.0028108286421166,
0.00969394810388323));
#47038=CARTESIAN_POINT('Ctrl Pts',(-0.233879460305132,0.00287024877252639,
0.009599479752749));
#47039=CARTESIAN_POINT('Ctrl Pts',(-0.23395842524631,0.00179682516051009,
0.00896703580133416));
#47040=CARTESIAN_POINT('Ctrl Pts',(-0.233846367591842,0.00181382176323882,
0.00898039582417626));
#47041=CARTESIAN_POINT('Ctrl Pts',(-0.233857974495682,0.00188386343549592,
0.00889339615048512));
#47042=CARTESIAN_POINT('Ctrl Pts',(-0.233525319503738,0.000950916333047615,
0.00815049547091419));
#47043=CARTESIAN_POINT('Ctrl Pts',(-0.233425241575143,0.000987309445839432,
0.00819063695809306));
#47044=CARTESIAN_POINT('Ctrl Pts',(-0.233436000330147,0.00106648365210777,
0.00811134827503141));
#47045=CARTESIAN_POINT('Ctrl Pts',(-0.232815357496005,0.000312535379510872,
0.00735780536508385));
#47046=CARTESIAN_POINT('Ctrl Pts',(-0.232729912996603,0.000355240759461433,
0.00741848169680565));
#47047=CARTESIAN_POINT('Ctrl Pts',(-0.232739152296681,0.000441578432710503,
0.00734645441856656));
#47048=CARTESIAN_POINT('Ctrl Pts',(-0.231951736654993,-0.000171158652928347,
0.0066165523630098));
#47049=CARTESIAN_POINT('Ctrl Pts',(-0.23187366145612,-0.000131220286198218,
0.00668759534496474));
#47050=CARTESIAN_POINT('Ctrl Pts',(-0.231881821261106,-3.87834252174242E-5,
0.00662323404316121));
#47051=CARTESIAN_POINT('Ctrl Pts',(-0.230785589044538,-0.000709423264214162,
0.00560435737523353));
#47052=CARTESIAN_POINT('Ctrl Pts',(-0.230706537242168,-0.000679412943678259,
0.0056793959267812));
#47053=CARTESIAN_POINT('Ctrl Pts',(-0.230714035519574,-0.00057952778959745,
0.00562665136337194));
#47054=CARTESIAN_POINT('Ctrl Pts',(-0.229659631065858,-0.00112259134770437,
0.00450042681701567));
#47055=CARTESIAN_POINT('Ctrl Pts',(-0.229573488553691,-0.00110522274085626,
0.00457169571489191));
#47056=CARTESIAN_POINT('Ctrl Pts',(-0.229581284792486,-0.000999176418349601,
0.00453324254178003));
#47057=CARTESIAN_POINT('Ctrl Pts',(-0.228704830832439,-0.00140318368076378,
0.00315941395843816));
#47058=CARTESIAN_POINT('Ctrl Pts',(-0.228610654986378,-0.00139852405540933,
0.00322143708123328));
#47059=CARTESIAN_POINT('Ctrl Pts',(-0.228618237517232,-0.0012879748082025,
0.00319964145512532));
#47060=CARTESIAN_POINT('Ctrl Pts',(-0.227556561243924,-0.00154241565951436,
0.0012329595537125));
#47061=CARTESIAN_POINT('Ctrl Pts',(-0.227456077166232,-0.00155052303720059,
0.00128236480914283));
#47062=CARTESIAN_POINT('Ctrl Pts',(-0.227460355524764,-0.0014385066227586,
0.00128071762255347));
#47063=CARTESIAN_POINT('Ctrl Pts',(-0.227067475401737,-0.00156364911782018,
-0.000543776460822949));
#47064=CARTESIAN_POINT('Ctrl Pts',(-0.226954628187393,-0.00156468311793233,
-0.000524073299869157));
#47065=CARTESIAN_POINT('Ctrl Pts',(-0.226966244999462,-0.00145297979334359,
-0.000526745240384302));
#47066=CARTESIAN_POINT('Ctrl Pts',(-0.226499467790203,-0.00150465501127181,
-0.00186941076976256));
#47067=CARTESIAN_POINT('Ctrl Pts',(-0.226406444017648,-0.00151556901664699,
-0.00180216089269515));
#47068=CARTESIAN_POINT('Ctrl Pts',(-0.226407377277794,-0.00140350174937455,
-0.001803497060247));
#47069=CARTESIAN_POINT('Ctrl Pts',(-0.227106039951076,-0.00144162797772285,
-1.96352411817887E-8));
#47070=CARTESIAN_POINT('Ctrl Pts',(-0.227106764003939,-0.00148696123572356,
-1.58531560466822E-8));
#47071=CARTESIAN_POINT('Ctrl Pts',(-0.227143294427859,-0.00152691654689948,
-1.05861461769103E-7));
#47072=CARTESIAN_POINT('Ctrl Pts',(-0.22718689352733,-0.00153702230304076,
8.6620036555294E-8));
#47073=CARTESIAN_POINT('Ctrl Pts',(-0.227195833594342,-0.00153909450494876,
1.26088684176056E-7));
#47074=CARTESIAN_POINT('Ctrl Pts',(-0.227205033194746,-0.00154006152936436,
1.63587269727728E-7));
#47075=CARTESIAN_POINT('Ctrl Pts',(-0.227214174219929,-0.00153991824305303,
1.76093623814383E-7));
#47076=CARTESIAN_POINT('Ctrl Pts',(-0.226392113206532,0.0163918999727596,
0.00168503949271779));
#47077=CARTESIAN_POINT('Ctrl Pts',(-0.226391019396591,0.0164937656877913,
0.00168965763500863));
#47078=CARTESIAN_POINT('Ctrl Pts',(-0.226488180900027,0.0164909418855625,
0.00172671497106663));
#47079=CARTESIAN_POINT('Ctrl Pts',(-0.226852777892721,0.0164582707631305,
0.000831312067351));
#47080=CARTESIAN_POINT('Ctrl Pts',(-0.226855540364924,0.0165604646886994,
0.00083395588090366));
#47081=CARTESIAN_POINT('Ctrl Pts',(-0.226949543911946,0.0165548900333955,
0.00087119979331494));
#47082=CARTESIAN_POINT('Ctrl Pts',(-0.227237968586075,0.0164450763319647,
-0.000539645166208353));
#47083=CARTESIAN_POINT('Ctrl Pts',(-0.227238798227237,0.0165473213837703,
-0.000542455601089969));
#47084=CARTESIAN_POINT('Ctrl Pts',(-0.227337590667714,0.0165449321176619,
-0.000511810717256663));
#47085=CARTESIAN_POINT('Ctrl Pts',(-0.228035000539669,0.0163790222318258,
-0.00217959547214826));
#47086=CARTESIAN_POINT('Ctrl Pts',(-0.228036534639494,0.016481137218235,
-0.00218239346647812));
#47087=CARTESIAN_POINT('Ctrl Pts',(-0.22812497432452,0.0164790173149829,
-0.00213090379182275));
#47088=CARTESIAN_POINT('Ctrl Pts',(-0.228708921333346,0.0162902569986761,
-0.00323431581776797));
#47089=CARTESIAN_POINT('Ctrl Pts',(-0.22870963661687,0.0163920559157401,
-0.00325001291976414));
#47090=CARTESIAN_POINT('Ctrl Pts',(-0.228793564308444,0.0163974242481985,
-0.00319058715685894));
#47091=CARTESIAN_POINT('Ctrl Pts',(-0.229730987265362,0.0160079041094603,
-0.00452203445052858));
#47092=CARTESIAN_POINT('Ctrl Pts',(-0.229730769949974,0.01610670436963,
-0.00455111205785709));
#47093=CARTESIAN_POINT('Ctrl Pts',(-0.229805911713532,0.0161237707411685,
-0.00448235671725372));
#47094=CARTESIAN_POINT('Ctrl Pts',(-0.230935134430229,0.0156120089346621,
-0.00557070752495235));
#47095=CARTESIAN_POINT('Ctrl Pts',(-0.230934670361149,0.0157064984816925,
-0.00561229511004819));
#47096=CARTESIAN_POINT('Ctrl Pts',(-0.231002371233807,0.0157353050227464,
-0.00554004179593496));
#47097=CARTESIAN_POINT('Ctrl Pts',(-0.232177744180245,0.0151028200699603,
-0.00653547490843776));
#47098=CARTESIAN_POINT('Ctrl Pts',(-0.232176588665142,0.0151916192466989,
-0.00658760783579178));
#47099=CARTESIAN_POINT('Ctrl Pts',(-0.232244981206936,0.0152287657678068,
-0.00652027966165211));
#47100=CARTESIAN_POINT('Ctrl Pts',(-0.233054633763043,0.0146485714867585,
-0.00724293745904123));
#47101=CARTESIAN_POINT('Ctrl Pts',(-0.233053075526623,0.0147322907208735,
-0.00730274052660402));
#47102=CARTESIAN_POINT('Ctrl Pts',(-0.233129281923515,0.0147718879604937,
-0.00724522074812763));
#47103=CARTESIAN_POINT('Ctrl Pts',(-0.233780549323432,0.0140296693618124,
-0.00802833810437384));
#47104=CARTESIAN_POINT('Ctrl Pts',(-0.233778793651804,0.0141064055513379,
-0.00809659254281335));
#47105=CARTESIAN_POINT('Ctrl Pts',(-0.233870885754837,0.0141387792230417,
-0.00806053199685345));
#47106=CARTESIAN_POINT('Ctrl Pts',(-0.23417681319712,0.0131895359915029,
-0.00885217079243862));
#47107=CARTESIAN_POINT('Ctrl Pts',(-0.234175306972833,0.0132559030196369,
-0.00893028824280225));
#47108=CARTESIAN_POINT('Ctrl Pts',(-0.234278422455447,0.0132689423938031,
-0.00892070199865507));
#47109=CARTESIAN_POINT('Ctrl Pts',(-0.234152670783076,0.0121914679424191,
-0.00957792241659341));
#47110=CARTESIAN_POINT('Ctrl Pts',(-0.23415083916279,0.0122454565740586,
-0.00966504377078786));
#47111=CARTESIAN_POINT('Ctrl Pts',(-0.23425279196153,0.0122284519300089,
-0.00967704060679076));
#47112=CARTESIAN_POINT('Ctrl Pts',(-0.233726044807365,0.0111642828582113,
-0.0101174976232404));
#47113=CARTESIAN_POINT('Ctrl Pts',(-0.233723596210825,0.0112061357531395,
-0.0102112243167655));
#47114=CARTESIAN_POINT('Ctrl Pts',(-0.233815358570609,0.0111632233286248,
-0.0102310405426672));
#47115=CARTESIAN_POINT('Ctrl Pts',(-0.233061858989254,0.0101827622716988,
-0.0104764728820601));
#47116=CARTESIAN_POINT('Ctrl Pts',(-0.233059226207355,0.0102132546913798,
-0.0105746029191505));
#47117=CARTESIAN_POINT('Ctrl Pts',(-0.23314194681633,0.0101548706247753,
-0.0105925793018587));
#47118=CARTESIAN_POINT('Ctrl Pts',(-0.231683602236085,0.00851585290564029,
-0.0108729492449486));
#47119=CARTESIAN_POINT('Ctrl Pts',(-0.231680434000005,0.00852679029691534,
-0.0109760864334407));
#47120=CARTESIAN_POINT('Ctrl Pts',(-0.231755479841859,0.0084561911036003,
-0.0109838889155731));
#47121=CARTESIAN_POINT('Ctrl Pts',(-0.230418420088248,0.00719112093427334,
-0.0108666061778807));
#47122=CARTESIAN_POINT('Ctrl Pts',(-0.230415842999401,0.00718736729446149,
-0.0109698519447955));
#47123=CARTESIAN_POINT('Ctrl Pts',(-0.230492085334579,0.00711822388992815,
-0.0109659055259879));
#47124=CARTESIAN_POINT('Ctrl Pts',(-0.229525698879995,0.00614771790123177,
-0.0106946346144635));
#47125=CARTESIAN_POINT('Ctrl Pts',(-0.22952334834197,0.00613160474304804,
-0.0107960792076886));
#47126=CARTESIAN_POINT('Ctrl Pts',(-0.229599955864645,0.00606416878077252,
-0.0107848368047938));
#47127=CARTESIAN_POINT('Ctrl Pts',(-0.230713742406189,0.00748906369436089,
-0.010821683971079));
#47128=CARTESIAN_POINT('Ctrl Pts',(-0.230713574584272,0.00748905436859433,
-0.0108291148800308));
#47129=CARTESIAN_POINT('Ctrl Pts',(-0.230714527471167,0.00748904745953601,
-0.0108364768338736));
#47130=CARTESIAN_POINT('Ctrl Pts',(-0.23071872359061,0.00748903792811973,
-0.0108515735632303));
#47131=CARTESIAN_POINT('Ctrl Pts',(-0.230722151247374,0.0074890359577174,
-0.0108590855100948));
#47132=CARTESIAN_POINT('Ctrl Pts',(-0.23073376178249,0.00748903765108982,
-0.0108775512731657));
#47133=CARTESIAN_POINT('Ctrl Pts',(-0.230743810553506,0.0074890458653673,
-0.0108879615646477));
#47134=CARTESIAN_POINT('Ctrl Pts',(-0.230770302348385,0.00748907690128229,
-0.0109067656321191));
#47135=CARTESIAN_POINT('Ctrl Pts',(-0.230786433005652,0.00748910168902196,
-0.0109140058410522));
#47136=CARTESIAN_POINT('Ctrl Pts',(-0.230810323644408,0.00748913267026307,
-0.0109206355722776));
#47137=CARTESIAN_POINT('Ctrl Pts',(-0.230817653411284,0.00748914304852623,
-0.0109221578060995));
#47138=CARTESIAN_POINT('Ctrl Pts',(-0.230828641240643,0.00748914067964123,
-0.0109237318478977));
#47139=CARTESIAN_POINT('Ctrl Pts',(-0.23083224030065,0.00748914000390417,
-0.0109241347209408));
#47140=CARTESIAN_POINT('Ctrl Pts',(-0.230837645742019,0.00748910265615934,
-0.010924578658873));
#47141=CARTESIAN_POINT('Ctrl Pts',(-0.230839444858523,0.0074890863471106,
-0.0109246969586367));
#47142=CARTESIAN_POINT('Ctrl Pts',(-0.23084194199522,0.00748900478020963,
-0.0109248290895748));
#47143=CARTESIAN_POINT('Ctrl Pts',(-0.230842846341935,0.00748896132912684,
-0.0109248694996749));
#47144=CARTESIAN_POINT('Ctrl Pts',(-0.230844078640512,0.00748881721420382,
-0.0109249173915236));
#47145=CARTESIAN_POINT('Ctrl Pts',(-0.230844469751936,0.00748873856186406,
-0.0109249304395881));
#47146=CARTESIAN_POINT('Ctrl Pts',(-0.230845032959145,0.00748854352309953,
-0.0109249479600377));
#47147=CARTESIAN_POINT('Ctrl Pts',(-0.230845459445073,0.00748823871023351,
-0.0109249589743604));
#47148=CARTESIAN_POINT('Ctrl Pts',(-0.226417776006695,-0.00148225140227062,
0.00185960662666182));
#47149=CARTESIAN_POINT('Ctrl Pts',(-0.226315901794499,-0.00148400327446099,
0.0018271058249673));
#47150=CARTESIAN_POINT('Ctrl Pts',(-0.226321596488582,-0.00138004225740634,
0.00182063316556843));
#47151=CARTESIAN_POINT('Ctrl Pts',(-0.226922704220666,-0.00155536550330681,
0.000950761709448938));
#47152=CARTESIAN_POINT('Ctrl Pts',(-0.226827971984197,-0.00156047124551848,
0.000910041917077747));
#47153=CARTESIAN_POINT('Ctrl Pts',(-0.226827215374829,-0.00145621045917323,
0.000908994318720162));
#47154=CARTESIAN_POINT('Ctrl Pts',(-0.22731937189759,-0.00154668628306353,
-0.000461986142874138));
#47155=CARTESIAN_POINT('Ctrl Pts',(-0.227217889493944,-0.00154838350965434,
-0.000491876202524546));
#47156=CARTESIAN_POINT('Ctrl Pts',(-0.227220115021664,-0.0014440291172182,
-0.000488620476369189));
#47157=CARTESIAN_POINT('Ctrl Pts',(-0.228125390529573,-0.00147896673645822,
-0.00213882311461267));
#47158=CARTESIAN_POINT('Ctrl Pts',(-0.228035127544321,-0.00148038441206057,
-0.00219126104933539));
#47159=CARTESIAN_POINT('Ctrl Pts',(-0.228035985439426,-0.00137628011913535,
-0.0021870094782073));
#47160=CARTESIAN_POINT('Ctrl Pts',(-0.228800442741132,-0.00139591234854455,
-0.00319848657186414));
#47161=CARTESIAN_POINT('Ctrl Pts',(-0.228714988735678,-0.00138956022407906,
-0.00325932429238547));
#47162=CARTESIAN_POINT('Ctrl Pts',(-0.228716584232433,-0.00128596080771844,
-0.00324145656436105));
#47163=CARTESIAN_POINT('Ctrl Pts',(-0.229802414559229,-0.00112488746796975,
-0.00447866062824715));
#47164=CARTESIAN_POINT('Ctrl Pts',(-0.22972550890945,-0.00110682459306145,
-0.00454832175455453));
#47165=CARTESIAN_POINT('Ctrl Pts',(-0.229727909135064,-0.0010065759274476,
-0.00451693236917198));
#47166=CARTESIAN_POINT('Ctrl Pts',(-0.23102492508135,-0.000727133402331402,
-0.00555987995846644));
#47167=CARTESIAN_POINT('Ctrl Pts',(-0.230955989651605,-0.000696808628886392,
-0.00563338908879835));
#47168=CARTESIAN_POINT('Ctrl Pts',(-0.230958341272015,-0.000601417291620782,
-0.00558870908358806));
#47169=CARTESIAN_POINT('Ctrl Pts',(-0.2322669550296,-0.000219169508655132,
-0.00653742651569375));
#47170=CARTESIAN_POINT('Ctrl Pts',(-0.232197149845059,-0.000180431312386987,
-0.00660566366607625));
#47171=CARTESIAN_POINT('Ctrl Pts',(-0.232200275963735,-9.10743939232668E-5,
-0.00655046594115202));
#47172=CARTESIAN_POINT('Ctrl Pts',(-0.233168284464011,0.000250847815714136,
-0.00727854722407495));
#47173=CARTESIAN_POINT('Ctrl Pts',(-0.233089769094286,0.00029173553377382,
-0.00733597722321239));
#47174=CARTESIAN_POINT('Ctrl Pts',(-0.233093540799596,0.000375715453733222,
-0.00727309367766053));
#47175=CARTESIAN_POINT('Ctrl Pts',(-0.233887901163237,0.00088893249295194,
-0.00809090747094352));
#47176=CARTESIAN_POINT('Ctrl Pts',(-0.233793447168666,0.000921951025758477,
-0.00812622297247575));
#47177=CARTESIAN_POINT('Ctrl Pts',(-0.233797813695556,0.000998937702461697,
-0.00805531832094409));
#47178=CARTESIAN_POINT('Ctrl Pts',(-0.2342833231198,0.00175231486175419,
-0.00893805236514278));
#47179=CARTESIAN_POINT('Ctrl Pts',(-0.234178058148385,0.00176584924761954,
-0.00894697349444574));
#47180=CARTESIAN_POINT('Ctrl Pts',(-0.234182479893669,0.00183287667611329,
-0.00886686230220629));
#47181=CARTESIAN_POINT('Ctrl Pts',(-0.234239736026175,0.00278957126582501,
-0.00968761331434967));
#47182=CARTESIAN_POINT('Ctrl Pts',(-0.234135862048126,0.0027716261589432,
-0.0096741294278813));
#47183=CARTESIAN_POINT('Ctrl Pts',(-0.234140599754382,0.00282694337281929,
-0.00958554148882367));
#47184=CARTESIAN_POINT('Ctrl Pts',(-0.233800163603698,0.00384612493495253,
-0.0102343465381826));
#47185=CARTESIAN_POINT('Ctrl Pts',(-0.233707082011014,0.00380181276785467,
-0.010213200060769));
#47186=CARTESIAN_POINT('Ctrl Pts',(-0.233712136747671,0.00384561342082835,
-0.010118178596806));
#47187=CARTESIAN_POINT('Ctrl Pts',(-0.233127412811296,0.0048454443045241,
-0.0105921689340489));
#47188=CARTESIAN_POINT('Ctrl Pts',(-0.233042619310187,0.00478663294724717,
-0.0105732614730382));
#47189=CARTESIAN_POINT('Ctrl Pts',(-0.233047623062891,0.00481933284931598,
-0.0104737473815675));
#47190=CARTESIAN_POINT('Ctrl Pts',(-0.23171980787036,0.00658675750707835,
-0.0109937670799221));
#47191=CARTESIAN_POINT('Ctrl Pts',(-0.231644109187706,0.00651358566164336,
-0.0109850576705971));
#47192=CARTESIAN_POINT('Ctrl Pts',(-0.231649556960457,0.00652610632374098,
-0.0108799788430654));
#47193=CARTESIAN_POINT('Ctrl Pts',(-0.230396057458204,0.00794487415788723,
-0.0109626141392042));
#47194=CARTESIAN_POINT('Ctrl Pts',(-0.230317899932501,0.00787480750145839,
-0.0109666566144382));
#47195=CARTESIAN_POINT('Ctrl Pts',(-0.230322554500073,0.00787234081934371,
-0.0108613201128976));
#47196=CARTESIAN_POINT('Ctrl Pts',(-0.229489510910491,0.00904713179573227,
-0.0107675268815905));
#47197=CARTESIAN_POINT('Ctrl Pts',(-0.229412653084916,0.00897672311594609,
-0.0107789166455273));
#47198=CARTESIAN_POINT('Ctrl Pts',(-0.229417095976447,0.00896089386946676,
-0.010675313992194));
#54553=UNCERTAINTY_MEASURE_WITH_UNIT(LENGTH_MEASURE(1.E-5),#54581,
'DISTANCE_ACCURACY_VALUE',
'Maximum model space distance between geometric entities at asserted c
onnectivities');
#54564=UNCERTAINTY_MEASURE_WITH_UNIT(LENGTH_MEASURE(1.E-5),#54581,
'DISTANCE_ACCURACY_VALUE',
'Maximum model space distance between geometric entities at asserted c
onnectivities');
#54569=(
GEOMETRIC_REPRESENTATION_CONTEXT(3)
GLOBAL_UNCERTAINTY_ASSIGNED_CONTEXT((#54553))
GLOBAL_UNIT_ASSIGNED_CONTEXT((#54581,#54582,#54583))
REPRESENTATION_CONTEXT('','3D')
);
#54580=(
GEOMETRIC_REPRESENTATION_CONTEXT(3)
GLOBAL_UNCERTAINTY_ASSIGNED_CONTEXT((#54564))
GLOBAL_UNIT_ASSIGNED_CONTEXT((#54581,#54582,#54583))
REPRESENTATION_CONTEXT('','3D')
);
#54581=(
LENGTH_UNIT()
NAMED_UNIT(*)
SI_UNIT($,.METRE.)
);
#54582=(
NAMED_UNIT(*)
PLANE_ANGLE_UNIT()
SI_UNIT($,.RADIAN.)
);
#54583=(
NAMED_UNIT(*)
SI_UNIT($,.STERADIAN.)
SOLID_ANGLE_UNIT()
);
#54588=SHAPE_DEFINITION_REPRESENTATION(#54603,#54633);
#54603=PRODUCT_DEFINITION_SHAPE('',$,#54649);
#54633=SHAPE_REPRESENTATION('',(#18520),#54569);
#54644=PRODUCT_DEFINITION_CONTEXT('part definition',#54691,'design');
#54649=PRODUCT_DEFINITION('Part_10','Part_10',#54664,#54644);
#54664=PRODUCT_DEFINITION_FORMATION('',$,#54697);
#54691=APPLICATION_CONTEXT(
'Core Data for Automotive Mechanical Design Process');
#54692=PRODUCT_CONTEXT('part definition',#54691,'mechanical');
#54697=PRODUCT('Part_10','Part_10','Part 1',(#54692));
#54714=PRESENTATION_STYLE_ASSIGNMENT((#54724));
#54724=SURFACE_STYLE_USAGE(.BOTH.,#54734);
#54734=SURFACE_SIDE_STYLE('',(#54744));
#54744=SURFACE_STYLE_FILL_AREA(#54754);
#54754=FILL_AREA_STYLE('Opaque(73,169,84)',(#54764));
#54764=FILL_AREA_STYLE_COLOUR('Opaque(73,169,84)',#54774);
#54774=COLOUR_RGB('Opaque(73,169,84)', 0.40784314, 0.44705882, 0.49803922);
ENDSEC;
END-ISO-10303-21;
